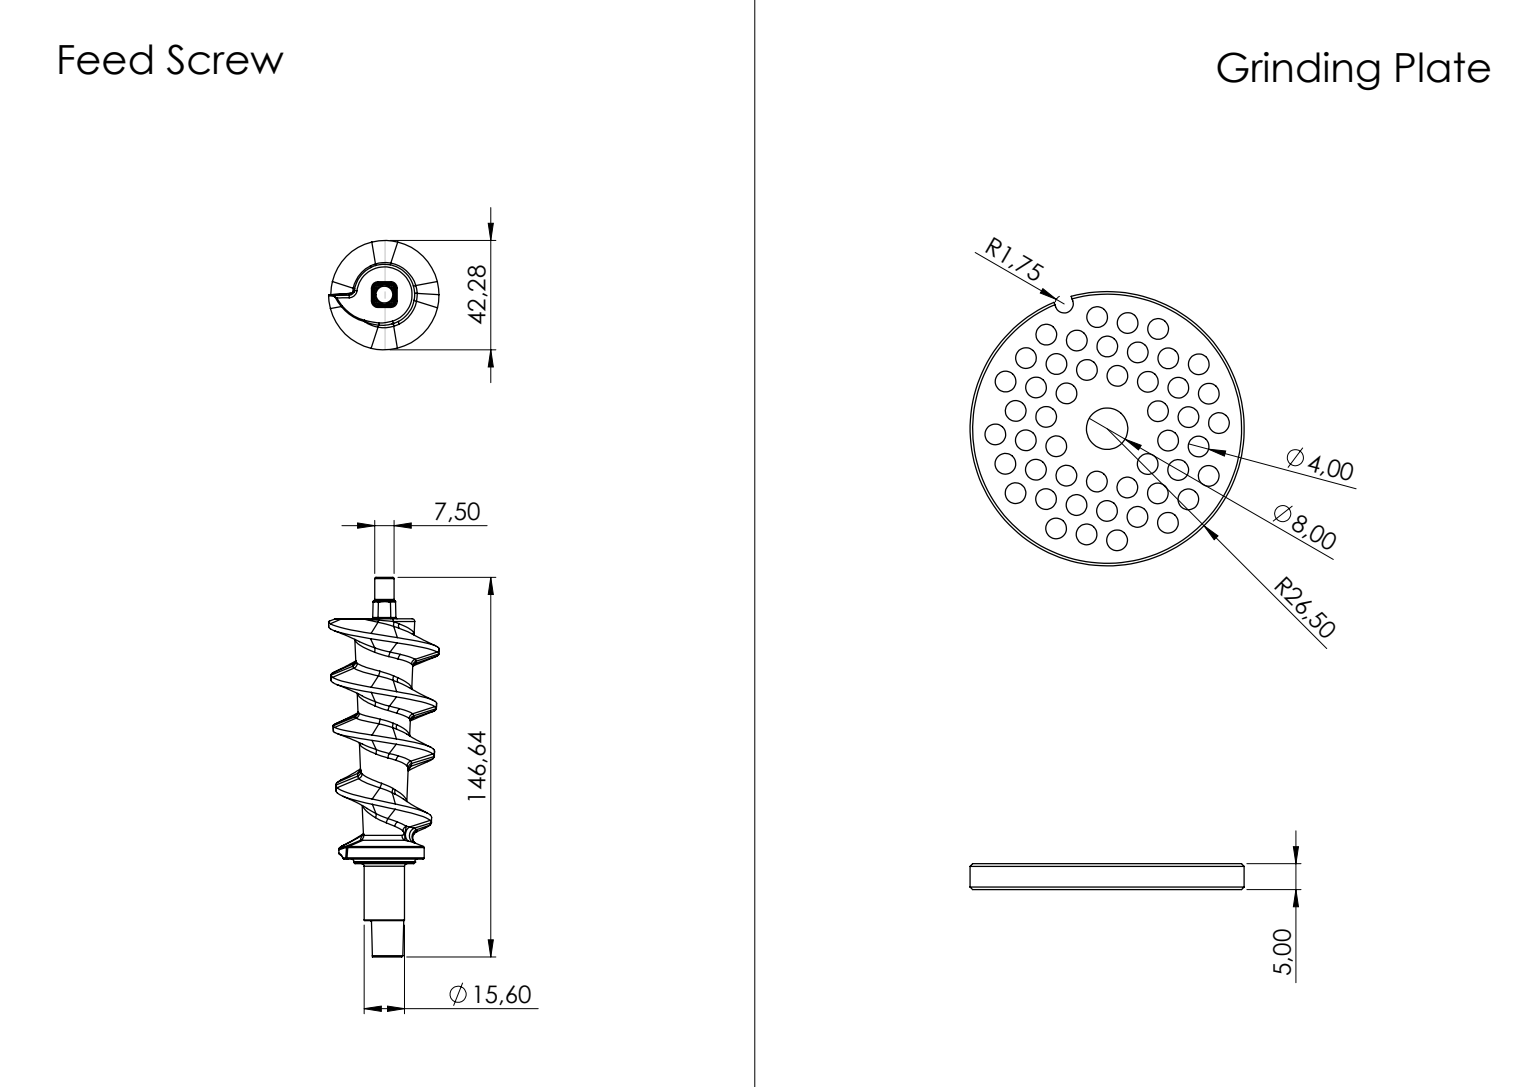
ISO-10303-21;
HEADER;
FILE_DESCRIPTION (('STEP AP214'),
    '1' );
FILE_NAME ('Feed Screw.step',
    '2026-10-06T09:49:54',
    ( '' ),
    ( '' ),
    'SwSTEP 2.0',
    'SolidWorks 2020',
    '' );
FILE_SCHEMA (( 'AUTOMOTIVE_DESIGN' ));
ENDSEC;

DATA;
#2=CIRCLE ( 'NONE', #35720, 101.7125698847119821 ) ;
#3=CARTESIAN_POINT ( 'NONE',  ( -1.842962214803815835, 1515.372048948338943, 213.3835825141717351 ) ) ;
#4=CARTESIAN_POINT ( 'NONE',  ( 9.183457267990059236, 1463.661210998930073, 215.2718514178839939 ) ) ;
#8=AXIS2_PLACEMENT_3D ( 'NONE', #3263, #37391, #36278 ) ;
#10=CARTESIAN_POINT ( 'NONE',  ( 0.5551898266394985626, 1477.809674746627479, 198.7211068470872135 ) ) ;
#12=CARTESIAN_POINT ( 'NONE',  ( -1.480872463509999903, 1515.456375364289897, 204.9462865469589872 ) ) ;
#15=CARTESIAN_POINT ( 'NONE',  ( 18.94656044352759849, 1455.761274322379904, 200.3458232381809694 ) ) ;
#17=CARTESIAN_POINT ( 'NONE',  ( -11.86274611122550127, 1422.387374207680068, 206.9860570071450070 ) ) ;
#28=CARTESIAN_POINT ( 'NONE',  ( -10.29516445159999982, 1471.669286221989978, 209.3797728120900103 ) ) ;
#29=DIRECTION ( 'NONE',  ( -3.697785493223495027E-32, -1.000000000000000000, 1.836970198721029688E-16 ) ) ;
#33=CARTESIAN_POINT ( 'NONE',  ( -4.766037424247389964, 1433.470086930039997, 216.3697912905370231 ) ) ;
#41=CARTESIAN_POINT ( 'NONE',  ( 11.68414648092010033, 1426.908524124409951, 207.1431733947370049 ) ) ;
#51=CARTESIAN_POINT ( 'NONE',  ( -6.833281637050000690, 1495.558145441189936, 200.1869151102389992 ) ) ;
#57=CARTESIAN_POINT ( 'NONE',  ( 5.798353088509999864, 1447.164911394289902, 201.8788308129090012 ) ) ;
#60=CARTESIAN_POINT ( 'NONE',  ( -2.894710226049999946, 1455.369075570189807, 200.0025452760189921 ) ) ;
#65=CARTESIAN_POINT ( 'NONE',  ( -1.064557613579999895, 1496.012454471690035, 220.6945835667989968 ) ) ;
#83=EDGE_CURVE ( 'NONE', #58839, #22042, #17431, .T. ) ;
#87=CARTESIAN_POINT ( 'NONE',  ( -4.994992778070000305, 1391.721842379389955, 214.6484993776389842 ) ) ;
#88=CARTESIAN_POINT ( 'NONE',  ( 15.23962836178434799, 1416.181292664740113, 211.4166089860522106 ) ) ;
#91=CARTESIAN_POINT ( 'NONE',  ( 9.827367186236088514, 1460.770885483560050, 206.7613957114989773 ) ) ;
#96=ORIENTED_EDGE ( 'NONE', *, *, #80068, .T. ) ;
#97=CARTESIAN_POINT ( 'NONE',  ( 2.803078862940000082, 1426.178365722219951, 191.2633630063989756 ) ) ;
#100=CARTESIAN_POINT ( 'NONE',  ( -12.21821484229520927, 1417.425190588804981, 199.7413714526001911 ) ) ;
#102=CARTESIAN_POINT ( 'NONE',  ( 4.324092179420000015, 1515.269353058490196, 209.1218459615519976 ) ) ;
#106=CARTESIAN_POINT ( 'NONE',  ( 9.417062327005512046, 1451.666586838229932, 209.4644760955090135 ) ) ;
#108=EDGE_CURVE ( 'NONE', #73608, #106056, #21407, .T. ) ;
#110=ORIENTED_EDGE ( 'NONE', *, *, #5630, .F. ) ;
#120=EDGE_CURVE ( 'NONE', #81793, #103948, #97600, .T. ) ;
#121=CARTESIAN_POINT ( 'NONE',  ( -9.628359219779209610, 1460.738556064009799, 208.1949697569470175 ) ) ;
#123=CARTESIAN_POINT ( 'NONE',  ( 10.94055631708340037, 1470.192781946979949, 206.9724510450730008 ) ) ;
#124=CARTESIAN_POINT ( 'NONE',  ( -3.048415848927723992, 1468.134006689671196, 219.8853015524805699 ) ) ;
#125=EDGE_CURVE ( 'NONE', #75164, #6066, #41467, .T. ) ;
#134=CARTESIAN_POINT ( 'NONE',  ( -17.39685236538799984, 1503.136637835580132, 222.8801028628849963 ) ) ;
#140=CARTESIAN_POINT ( 'NONE',  ( 0.7783252048321530614, 1515.125841190099891, 204.7939957918700316 ) ) ;
#144=CARTESIAN_POINT ( 'NONE',  ( -0.9578802547590020700, 1508.340034268889895, 220.7784182282989889 ) ) ;
#149=CARTESIAN_POINT ( 'NONE',  ( -5.649091365077420157, 1427.323616392150143, 201.6849725672220188 ) ) ;
#153=FACE_OUTER_BOUND ( 'NONE', #32956, .T. ) ;
#165=CARTESIAN_POINT ( 'NONE',  ( -14.80402621179999834, 1415.917690476640018, 204.7946628682890093 ) ) ;
#167=CARTESIAN_POINT ( 'NONE',  ( -4.911821946417970430, 1485.009740505319996, 198.2803573512069875 ) ) ;
#168=B_SPLINE_SURFACE_WITH_KNOTS ( 'NONE', 5, 5, ( 
 ( #106952, #71755, #28601, #29694, #97994, #64429 ),
 ( #81736, #88517, #89050, #98547, #97459, #20727 ),
 ( #54922, #21816, #107503, #56015, #12336, #105310 ),
 ( #90139, #13422, #62802, #46527, #11801, #45969 ),
 ( #80104, #37555, #80661, #98449, #4411, #47512 ),
 ( #96816, #3329, #28500, #89503, #82194, #106305 ),
 ( #97348, #37453, #12795, #72186, #90039, #21163 ),
 ( #90596, #62695, #38004, #13317, #4937, #12239 ),
 ( #72718, #45871, #80005, #29056, #106840, #63242 ) ),
 .UNSPECIFIED., .F., .F., .F.,
 ( 6, 3, 6 ),
 ( 6, 6 ),
 ( 14.29638737439180041, 25.07790639679999956, 35.02433850343369670 ),
 ( 0.000000000000000000, 2.000134677740009970 ),
 .UNSPECIFIED. ) ;
#169=CARTESIAN_POINT ( 'NONE',  ( -8.621279951388869378, 1436.974942194019832, 209.5887057810519991 ) ) ;
#170=CARTESIAN_POINT ( 'NONE',  ( -4.720696006799999900, 1497.300349750090163, 219.8012105612990013 ) ) ;
#172=CARTESIAN_POINT ( 'NONE',  ( 4.989246313819999834, 1471.909539260290103, 189.7082128665990126 ) ) ;
#175=CARTESIAN_POINT ( 'NONE',  ( -11.30102602861320094, 1508.425847713210032, 208.0120230822289784 ) ) ;
#193=CARTESIAN_POINT ( 'NONE',  ( 10.49733858283609855, 1480.659481621079976, 208.1380713321520091 ) ) ;
#195=CARTESIAN_POINT ( 'NONE',  ( -17.48499182319999790, 1442.494624508590050, 219.3180649765990040 ) ) ;
#197=CARTESIAN_POINT ( 'NONE',  ( -21.44637737161449920, 1506.412668956640118, 216.0243792029939982 ) ) ;
#202=CARTESIAN_POINT ( 'NONE',  ( 9.734438220109071338, 1436.124822200840072, 210.5259218765519620 ) ) ;
#203=CARTESIAN_POINT ( 'NONE',  ( -10.63028651890000020, 1491.023698122589849, 211.9405787866489845 ) ) ;
#204=CARTESIAN_POINT ( 'NONE',  ( 6.587579149753620023, 1448.214850730340004, 201.2521096501800173 ) ) ;
#214=ORIENTED_EDGE ( 'NONE', *, *, #74162, .T. ) ;
#220=CARTESIAN_POINT ( 'NONE',  ( -10.22078022364619976, 1448.827725899079724, 207.2905427559460065 ) ) ;
#221=CARTESIAN_POINT ( 'NONE',  ( -4.554962005479259446, 1508.731359867455467, 211.6097811027402713 ) ) ;
#230=CARTESIAN_POINT ( 'NONE',  ( 4.229167303610000594, 1436.983388288790138, 227.1518914930990150 ) ) ;
#234=VERTEX_POINT ( 'NONE', #57535 ) ;
#242=DIRECTION ( 'NONE',  ( -8.555280247707230573E-26, -1.000000000000000000, 1.836970198721029688E-16 ) ) ;
#245=EDGE_CURVE ( 'NONE', #43735, #91400, #105524, .T. ) ;
#249=ORIENTED_EDGE ( 'NONE', *, *, #87778, .F. ) ;
#257=CARTESIAN_POINT ( 'NONE',  ( 2.105736771246019767, 1423.442917612190058, 192.6277106367970191 ) ) ;
#258=EDGE_LOOP ( 'NONE', ( #43493, #77998, #28454, #11261 ) ) ;
#260=CARTESIAN_POINT ( 'NONE',  ( -17.51735096566159910, 1508.551704408389924, 210.4017072017840064 ) ) ;
#261=EDGE_CURVE ( 'NONE', #100109, #93900, #60124, .T. ) ;
#263=CARTESIAN_POINT ( 'NONE',  ( 5.082331142230000154, 1453.684120746589770, 217.0135184815189859 ) ) ;
#267=CARTESIAN_POINT ( 'NONE',  ( -2.999960124414019713, 1428.921094993090037, 200.2473963957619958 ) ) ;
#278=CARTESIAN_POINT ( 'NONE',  ( 10.93308164779909930, 1490.452501404730128, 209.9926135395130018 ) ) ;
#288=VERTEX_POINT ( 'NONE', #17119 ) ;
#290=CARTESIAN_POINT ( 'NONE',  ( -11.00800901137619903, 1508.439403004749920, 218.3132624233929846 ) ) ;
#293=CARTESIAN_POINT ( 'NONE',  ( -4.675540975309999681, 1462.620895424390028, 200.5633310686890241 ) ) ;
#301=CARTESIAN_POINT ( 'NONE',  ( 11.69460626421270000, 1479.933455554200009, 210.6357844716710019 ) ) ;
#302=CARTESIAN_POINT ( 'NONE',  ( 5.597778194180000888, 1506.679269386989972, 219.3685102149989916 ) ) ;
#308=EDGE_CURVE ( 'NONE', #12135, #84259, #7929, .T. ) ;
#312=CARTESIAN_POINT ( 'NONE',  ( 11.46319645939999887, 1501.893709296690076, 208.7006337201350163 ) ) ;
#318=DIRECTION ( 'NONE',  ( 0.000000000000000000, 1.000000000000000000, -1.836970198721029688E-16 ) ) ;
#320=CARTESIAN_POINT ( 'NONE',  ( -5.102340803919999779, 1483.010473641589897, 199.7820758705289848 ) ) ;
#328=VERTEX_POINT ( 'NONE', #27220 ) ;
#329=CARTESIAN_POINT ( 'NONE',  ( -2.217375791810000329, 1495.290970025190290, 217.2501089269190118 ) ) ;
#332=CARTESIAN_POINT ( 'NONE',  ( -0.6694169535389160597, 1457.182704574260015, 219.7360533319789795 ) ) ;
#336=CARTESIAN_POINT ( 'NONE',  ( 7.206186347910000123, 1424.944465238209887, 212.8420735846389960 ) ) ;
#337=CARTESIAN_POINT ( 'NONE',  ( -9.573037224950001089, 1423.427965722019962, 192.3355728592989919 ) ) ;
#345=VERTEX_POINT ( 'NONE', #33388 ) ;
#377=CARTESIAN_POINT ( 'NONE',  ( -3.070761075385165295, 1457.085219852218870, 218.1263196974262826 ) ) ;
#390=CARTESIAN_POINT ( 'NONE',  ( 10.73298406322840037, 1460.408024784029976, 207.0975327187530013 ) ) ;
#396=CARTESIAN_POINT ( 'NONE',  ( -18.69110324289999880, 1444.867398023490068, 206.3373603049990095 ) ) ;
#407=CARTESIAN_POINT ( 'NONE',  ( -10.75057650454519909, 1492.402834311169954, 203.1666067258980206 ) ) ;
#420=CARTESIAN_POINT ( 'NONE',  ( -16.94440841599999814, 1420.377411313550056, 203.4608118218089885 ) ) ;
#434=CARTESIAN_POINT ( 'NONE',  ( -13.41341432257899946, 1418.544055057069727, 200.5656092512240036 ) ) ;
#435=CARTESIAN_POINT ( 'NONE',  ( -5.015825127099213354, 1391.761757684846771, 203.5511880675617249 ) ) ;
#450=CARTESIAN_POINT ( 'NONE',  ( 10.56937681823290021, 1452.418559324240050, 209.1099374865879952 ) ) ;
#456=EDGE_LOOP ( 'NONE', ( #45426, #15333, #70007, #61987 ) ) ;
#458=FACE_OUTER_BOUND ( 'NONE', #93445, .T. ) ;
#462=CARTESIAN_POINT ( 'NONE',  ( 11.76667485211559949, 1479.372979666780111, 208.7507148262919827 ) ) ;
#470=CARTESIAN_POINT ( 'NONE',  ( -8.755578957433581166, 1424.773583938259890, 204.8410018134340191 ) ) ;
#475=CARTESIAN_POINT ( 'NONE',  ( 20.33642612138580219, 1475.138353456469986, 218.0161241308549904 ) ) ;
#479=DIRECTION ( 'NONE',  ( -1.699538841806929935E-33, 1.000000000000000000, -1.698192320643030073E-16 ) ) ;
#481=EDGE_CURVE ( 'NONE', #82285, #55990, #44994, .T. ) ;
#485=CARTESIAN_POINT ( 'NONE',  ( -2.314955559389999973, 1476.586284849689946, 199.0068122257989955 ) ) ;
#491=CARTESIAN_POINT ( 'NONE',  ( -7.514967970819999898, 1426.327999703259820, 205.9160403778789998 ) ) ;
#495=CARTESIAN_POINT ( 'NONE',  ( -7.863671303257509848, 1471.291298022706087, 215.5245834466820440 ) ) ;
#496=CARTESIAN_POINT ( 'NONE',  ( 7.537606959944939788, 1425.724147855899901, 212.1987702218239917 ) ) ;
#503=CARTESIAN_POINT ( 'NONE',  ( 1.205243432004479809, 1487.387165744484264, 219.8907050796039755 ) ) ;
#508=VERTEX_POINT ( 'NONE', #77503 ) ;
#515=ORIENTED_EDGE ( 'NONE', *, *, #31765, .T. ) ;
#529=CARTESIAN_POINT ( 'NONE',  ( -0.1150915766366530091, 1444.816874904579890, 199.0635159857669976 ) ) ;
#534=CARTESIAN_POINT ( 'NONE',  ( -3.384752634116700243, 1508.551704408389924, 213.9439043168609942 ) ) ;
#538=CARTESIAN_POINT ( 'NONE',  ( -3.774700670050000095, 1496.332844194289919, 198.4120365050989960 ) ) ;
#540=CARTESIAN_POINT ( 'NONE',  ( -1.514784269649715576, 1443.601484486217942, 218.3342104795610510 ) ) ;
#551=CARTESIAN_POINT ( 'NONE',  ( 9.575940986468468807, 1427.729431014379998, 211.3625234817539820 ) ) ;
#552=CARTESIAN_POINT ( 'NONE',  ( 1.154719254338330447, 1421.357514871522653, 193.7585151656728044 ) ) ;
#555=CARTESIAN_POINT ( 'NONE',  ( -9.252874484757731111, 1477.963449144112474, 214.0067384189093218 ) ) ;
#558=CARTESIAN_POINT ( 'NONE',  ( -11.02797255089159911, 1462.256692482700146, 209.5173753044250020 ) ) ;
#559=CARTESIAN_POINT ( 'NONE',  ( 18.24211828920000045, 1431.096497597789948, 200.8001355623590030 ) ) ;
#560=CARTESIAN_POINT ( 'NONE',  ( 10.45726464265210076, 1420.924558883679993, 198.4227429697920115 ) ) ;
#561=CARTESIAN_POINT ( 'NONE',  ( 4.780270616392929384, 1467.625973390280024, 217.8721612978610267 ) ) ;
#566=CARTESIAN_POINT ( 'NONE',  ( 0.3281250907512314741, 1477.756992672553451, 198.7115816712109506 ) ) ;
#568=CARTESIAN_POINT ( 'NONE',  ( -1.082449427729999858, 1515.225850744089939, 204.7966151436789914 ) ) ;
#570=CARTESIAN_POINT ( 'NONE',  ( -3.071477015947639888, 1470.850262397169899, 187.3986309147560121 ) ) ;
#572=CARTESIAN_POINT ( 'NONE',  ( -19.83550667398609946, 1418.664640197639983, 208.7685751368389901 ) ) ;
#578=DIRECTION ( 'NONE',  ( -0.000000000000000000, 1.836970198721029688E-16, 1.000000000000000000 ) ) ;
#582=CARTESIAN_POINT ( 'NONE',  ( -10.30263834680000024, 1471.732697784889979, 209.1299246244929861 ) ) ;
#583=B_SPLINE_CURVE_WITH_KNOTS ( 'NONE', 3,
 ( #94797, #754, #35441, #77995 ),
 .UNSPECIFIED., .F., .F.,
 ( 4, 4 ),
 ( 0.000000000000000000, 1.000000000000000000 ),
 .UNSPECIFIED. ) ;
#586=DIRECTION ( 'NONE',  ( -1.000000000000000000, 0.000000000000000000, 0.000000000000000000 ) ) ;
#587=CARTESIAN_POINT ( 'NONE',  ( -3.138770468918330003, 1433.097189459889933, 217.7316335566559928 ) ) ;
#589=CARTESIAN_POINT ( 'NONE',  ( 1.842963721827329815, 1515.551704300040001, 212.9514659606769840 ) ) ;
#594=CARTESIAN_POINT ( 'NONE',  ( 11.30421211722389963, 1422.134199828960163, 208.7798009037170175 ) ) ;
#599=CARTESIAN_POINT ( 'NONE',  ( 6.224950473385610472, 1466.920039123629977, 216.8753481341400118 ) ) ;
#601=CARTESIAN_POINT ( 'NONE',  ( 1.842962231260000028, 1515.064792882589927, 204.7923971856590128 ) ) ;
#603=CARTESIAN_POINT ( 'NONE',  ( -10.90040372089999998, 1492.525755917289871, 207.2558760794690045 ) ) ;
#608=CARTESIAN_POINT ( 'NONE',  ( 4.176540423850000572, 1446.483799824789912, 200.6257159222890039 ) ) ;
#611=CARTESIAN_POINT ( 'NONE',  ( -3.558358605100000016, 1455.955982659790152, 200.3550966547389862 ) ) ;
#615=CARTESIAN_POINT ( 'NONE',  ( -2.487213358930000062, 1495.883017016489930, 197.0235130655990190 ) ) ;
#616=CARTESIAN_POINT ( 'NONE',  ( -2.182814748220000212, 1496.366357223990008, 220.5334820124990074 ) ) ;
#618=CARTESIAN_POINT ( 'NONE',  ( -3.313501335607589748, 1397.551704408390151, 203.0565224509919915 ) ) ;
#633=EDGE_CURVE ( 'NONE', #14236, #26775, #48569, .T. ) ;
#635=CARTESIAN_POINT ( 'NONE',  ( 4.789026039587930050, 1508.551704408389924, 212.5881120909519950 ) ) ;
#639=CARTESIAN_POINT ( 'NONE',  ( 9.326151436081950408, 1460.944241195969880, 206.0386860876060098 ) ) ;
#640=CARTESIAN_POINT ( 'NONE',  ( -9.966727850805121136, 1439.480327375449860, 208.4309914983489875 ) ) ;
#642=VERTEX_POINT ( 'NONE', #25961 ) ;
#647=CARTESIAN_POINT ( 'NONE',  ( -11.16856291581570737, 1417.847332803086601, 198.5153517745319220 ) ) ;
#651=CARTESIAN_POINT ( 'NONE',  ( 9.418151193910370367, 1451.571079816670135, 209.2450735257419865 ) ) ;
#662=CARTESIAN_POINT ( 'NONE',  ( 6.537718912151950335, 1429.433188304760051, 215.9971499089490123 ) ) ;
#664=CARTESIAN_POINT ( 'NONE',  ( -8.182145408407338394, 1490.196931670758431, 216.4137635874354828 ) ) ;
#668=CARTESIAN_POINT ( 'NONE',  ( -8.211943818390000871, 1474.301007847190021, 202.7927141847590065 ) ) ;
#673=FACE_OUTER_BOUND ( 'NONE', #12560, .T. ) ;
#677=CARTESIAN_POINT ( 'NONE',  ( -19.73299507883049841, 1503.904988652430120, 218.6992329638289903 ) ) ;
#684=CARTESIAN_POINT ( 'NONE',  ( 0.4426438243888760060, 1515.147163425719782, 204.7945541343150069 ) ) ;
#690=CARTESIAN_POINT ( 'NONE',  ( -10.98255251702510016, 1462.120311678340158, 210.0436777776439783 ) ) ;
#692=FACE_OUTER_BOUND ( 'NONE', #109949, .T. ) ;
#694=CARTESIAN_POINT ( 'NONE',  ( 2.737811238710000428, 1478.658245750390051, 201.8858327187489863 ) ) ;
#696=CARTESIAN_POINT ( 'NONE',  ( -10.40955016854329962, 1480.514293831559826, 207.4814632850010128 ) ) ;
#703=EDGE_CURVE ( 'NONE', #94689, #56179, #31918, .T. ) ;
#707=CARTESIAN_POINT ( 'NONE',  ( -14.80403897610000108, 1417.086023134510015, 204.2975919913589848 ) ) ;
#710=CARTESIAN_POINT ( 'NONE',  ( -4.056355225345120274, 1485.204183987449824, 197.9328813784530041 ) ) ;
#712=CARTESIAN_POINT ( 'NONE',  ( 18.19395003950230105, 1429.625430537140119, 208.6624982699469797 ) ) ;
#713=CARTESIAN_POINT ( 'NONE',  ( -7.496170620820000075, 1497.189208763689976, 217.7743331409489826 ) ) ;
#714=VERTEX_POINT ( 'NONE', #62956 ) ;
#717=CARTESIAN_POINT ( 'NONE',  ( 10.57777681304790107, 1481.493442856720094, 209.1910062161780104 ) ) ;
#732=CARTESIAN_POINT ( 'NONE',  ( 3.609405579419999732, 1486.009611374690166, 219.2752556430990012 ) ) ;
#733=CARTESIAN_POINT ( 'NONE',  ( 10.89000033453339888, 1479.690907560379856, 208.0590789013299968 ) ) ;
#735=CARTESIAN_POINT ( 'NONE',  ( -17.57323599084560328, 1441.322512277789883, 219.0501625471149794 ) ) ;
#738=CARTESIAN_POINT ( 'NONE',  ( 20.56231132718039589, 1477.111355667389716, 217.7195232095880044 ) ) ;
#739=B_SPLINE_CURVE_WITH_KNOTS ( 'NONE', 5,
 ( #42585, #61612, #95745, #102472, #34730, #601 ),
 .UNSPECIFIED., .F., .F.,
 ( 6, 6 ),
 ( 0.000000000000000000, 1.000000000000000000 ),
 .UNSPECIFIED. ) ;
#744=CARTESIAN_POINT ( 'NONE',  ( -10.54543569900000044, 1491.422408008689899, 212.2964277208190254 ) ) ;
#745=CARTESIAN_POINT ( 'NONE',  ( 3.902982118626540320, 1446.676946215170119, 199.7493785281279770 ) ) ;
#751=CARTESIAN_POINT ( 'NONE',  ( 7.392112708435170099, 1434.232064116840093, 226.0537490036730048 ) ) ;
#753=CARTESIAN_POINT ( 'NONE',  ( 8.026470750289130152, 1504.708605097430109, 217.7675590729679982 ) ) ;
#754=CARTESIAN_POINT ( 'NONE',  ( -11.45094915626656018, 1505.046207261508243, 207.2314953572074785 ) ) ;
#761=ORIENTED_EDGE ( 'NONE', *, *, #76582, .F. ) ;
#763=CARTESIAN_POINT ( 'NONE',  ( -10.27580570860629905, 1448.659754571809799, 207.6397982481969962 ) ) ;
#764=CARTESIAN_POINT ( 'NONE',  ( 3.272146740929090303, 1515.551704204679936, 205.4774934054959772 ) ) ;
#769=CARTESIAN_POINT ( 'NONE',  ( 3.159262866049999730, 1466.676511916789877, 219.3004965968990234 ) ) ;
#777=VERTEX_POINT ( 'NONE', #27103 ) ;
#784=CARTESIAN_POINT ( 'NONE',  ( 20.96882344929999675, 1497.403700851489930, 212.2137616143489822 ) ) ;
#786=CARTESIAN_POINT ( 'NONE',  ( -0.9078489423485659460, 1465.209724574289794, 198.1556611775330055 ) ) ;
#788=CARTESIAN_POINT ( 'NONE',  ( 11.21656023086370091, 1422.137379126830183, 210.4074592674920154 ) ) ;
#791=ORIENTED_EDGE ( 'NONE', *, *, #108401, .F. ) ;
#795=DIRECTION ( 'NONE',  ( 0.9996573249755574819, 0.02617694830786557875, 0.000000000000000000 ) ) ;
#799=CARTESIAN_POINT ( 'NONE',  ( -1.400903968945880207, 1422.610669904860060, 192.5490106176209792 ) ) ;
#802=CARTESIAN_POINT ( 'NONE',  ( -17.67716118599750175, 1508.551704408389924, 210.4042409862270233 ) ) ;
#803=CARTESIAN_POINT ( 'NONE',  ( 1.779428963082609894, 1456.357349037730046, 198.6855221610310309 ) ) ;
#810=B_SPLINE_CURVE_WITH_KNOTS ( 'NONE', 3,
 ( #86877, #102007, #10171, #16338, #84662, #19666, #72306, #44910, #11292, #105900, #29721, #45460, #38124, #106437, #63371, #38670, #12366, #95830, #3999, #54953, #96390, #71782, #63906, #98021, #87442, #29180, #89079, #88010, #81220, #79601, #21293, #89626, #46553, #19098, #4536, #2905, #20755 ),
 .UNSPECIFIED., .F., .F.,
 ( 4, 3, 3, 3, 3, 3, 3, 3, 3, 3, 3, 3, 4 ),
 ( -12.02648877283809981, -11.71886065317380066, -11.10599023740059899, -10.45513282830309976, -9.768661030076680518, -9.016051782489549637, -8.113804059961630344, -7.249942693435659891, -6.491588414576360044, -5.633190057283429475, -4.895335684179899616, -4.254313181755179585, -3.650975912550000757 ),
 .UNSPECIFIED. ) ;
#811=FACE_OUTER_BOUND ( 'NONE', #80418, .T. ) ;
#818=ORIENTED_EDGE ( 'NONE', *, *, #64063, .F. ) ;
#820=CARTESIAN_POINT ( 'NONE',  ( 10.79932292162989960, 1490.768715835539979, 211.1233481957399931 ) ) ;
#839=B_SPLINE_CURVE_WITH_KNOTS ( 'NONE', 3,
 ( #94188, #26432, #95856, #96974, #60626, #95310, #44933, #10194, #44369, #79080, #712, #94749, #20238 ),
 .UNSPECIFIED., .F., .F.,
 ( 4, 3, 3, 3, 4 ),
 ( -1.599569173379999931, -0.7029132044934469636, 0.1891147555273189340, 1.073570521650659693, 1.599569173380000375 ),
 .UNSPECIFIED. ) ;
#840=CARTESIAN_POINT ( 'NONE',  ( 3.686065144790000137, 1468.106296616489999, 218.4108491294889802 ) ) ;
#841=CARTESIAN_POINT ( 'NONE',  ( 4.894570698429999922, 1447.010184225089915, 205.0316855332089858 ) ) ;
#847=CARTESIAN_POINT ( 'NONE',  ( 10.89269473999179993, 1480.433624861380167, 210.4306936963210148 ) ) ;
#849=CARTESIAN_POINT ( 'NONE',  ( -4.230955727593959104, 1446.180919742871311, 217.1469061245145724 ) ) ;
#857=CARTESIAN_POINT ( 'NONE',  ( 12.56213108819999924, 1501.082362947789989, 211.1229812159690198 ) ) ;
#861=CARTESIAN_POINT ( 'NONE',  ( 8.972723096110000185, 1427.878097284390151, 212.0837492402690145 ) ) ;
#866=CARTESIAN_POINT ( 'NONE',  ( -8.388361968899999965, 1483.465050472690109, 201.7385226000290004 ) ) ;
#874=ORIENTED_EDGE ( 'NONE', *, *, #74452, .T. ) ;
#876=CARTESIAN_POINT ( 'NONE',  ( -11.25637332900000054, 1500.624827952490023, 211.0037260121189888 ) ) ;
#877=CARTESIAN_POINT ( 'NONE',  ( -14.67979535943448255, 1416.151753477184002, 204.4125811959580972 ) ) ;
#880=CARTESIAN_POINT ( 'NONE',  ( -9.954564879586309090, 1438.994910147829842, 209.5496646517129875 ) ) ;
#881=EDGE_CURVE ( 'NONE', #44275, #39082, #97366, .T. ) ;
#884=CARTESIAN_POINT ( 'NONE',  ( 7.904651180169999236, 1423.075284537190100, 213.5785853047590024 ) ) ;
#885=CARTESIAN_POINT ( 'NONE',  ( -18.32377786700000399, 1464.077817829789865, 217.4721512913189940 ) ) ;
#890=CARTESIAN_POINT ( 'NONE',  ( 6.121126660120000729, 1455.402339941889750, 217.8370560331890147 ) ) ;
#894=CARTESIAN_POINT ( 'NONE',  ( -21.51338636340619814, 1505.551605034549766, 209.1218290568810119 ) ) ;
#896=CARTESIAN_POINT ( 'NONE',  ( 7.616929904139634999, 1500.300532160428247, 200.6431694768011482 ) ) ;
#898=CARTESIAN_POINT ( 'NONE',  ( -2.006862033407029955, 1475.288591552500066, 197.8580126313549954 ) ) ;
#925=B_SPLINE_SURFACE_WITH_KNOTS ( 'NONE', 5, 5, ( 
 ( #19475, #46376, #97294, #18912, #53676, #3824 ),
 ( #38484, #53110, #54765, #72133, #81042, #63188 ),
 ( #104039, #87819, #79951, #29002, #55317, #61517 ),
 ( #11106, #87247, #27891, #10538, #12182, #46923 ),
 ( #89449, #62074, #45268, #44712, #79406, #12741 ),
 ( #78863, #2717, #71032, #2170, #96760, #36285 ),
 ( #105153, #28445, #20030, #62639, #54224, #88351 ),
 ( #45818, #3268, #89993, #66483, #7097, #81581 ),
 ( #100045, #106789, #99478, #98393, #13268, #32299 ) ),
 .UNSPECIFIED., .F., .F., .F.,
 ( 6, 3, 6 ),
 ( 6, 6 ),
 ( 0.000000000000000000, 6.814644137399999302, 13.62928827480000038 ),
 ( 0.000000000000000000, 2.000000000000000000 ),
 .UNSPECIFIED. ) ;
#933=CARTESIAN_POINT ( 'NONE',  ( 5.983287317399999417, 1451.235340618889950, 210.0682002075799915 ) ) ;
#936=ADVANCED_FACE ( 'NONE', ( #76810 ), #40125, .T. ) ;
#940=CARTESIAN_POINT ( 'NONE',  ( -18.84544153430000080, 1444.454624232390188, 208.1911640471150235 ) ) ;
#950=EDGE_CURVE ( 'NONE', #36610, #45421, #18629, .T. ) ;
#951=CARTESIAN_POINT ( 'NONE',  ( -11.26811797368760004, 1492.006046055339993, 204.2379200572160016 ) ) ;
#961=CARTESIAN_POINT ( 'NONE',  ( -14.65245215464970130, 1420.119839417710182, 213.8659310620899987 ) ) ;
#964=ORIENTED_EDGE ( 'NONE', *, *, #29949, .T. ) ;
#966=CARTESIAN_POINT ( 'NONE',  ( 4.987078435459999071, 1509.051704408389924, 209.1218459616989946 ) ) ;
#971=CARTESIAN_POINT ( 'NONE',  ( 2.969165624449999541, 1442.252637987289972, 217.6050255308190060 ) ) ;
#976=EDGE_CURVE ( 'NONE', #32267, #2539, #49404, .T. ) ;
#978=CARTESIAN_POINT ( 'NONE',  ( 9253.086965755297570, 5182.654794667092574, 284.7734187413164477 ) ) ;
#980=CARTESIAN_POINT ( 'NONE',  ( -14.43176806938940082, 1417.361901689390152, 203.3004255274190086 ) ) ;
#983=CARTESIAN_POINT ( 'NONE',  ( -8.333035966500000669, 1508.478891882389917, 219.2689049391989897 ) ) ;
#991=CARTESIAN_POINT ( 'NONE',  ( -3.276363691050809823, 1486.691431019839911, 220.6577433852839931 ) ) ;
#992=CARTESIAN_POINT ( 'NONE',  ( -8.229021304010000648, 1439.448076410589920, 228.6152058856989697 ) ) ;
#998=CARTESIAN_POINT ( 'NONE',  ( 10.57159226293329901, 1452.549534872659933, 209.4522820094259714 ) ) ;
#1011=EDGE_CURVE ( 'NONE', #13254, #104898, #107740, .T. ) ;
#1020=CARTESIAN_POINT ( 'NONE',  ( 9.327660711791368797, 1434.415577812250149, 206.2244467992360057 ) ) ;
#1021=CARTESIAN_POINT ( 'NONE',  ( -15.14764113784119992, 1421.271689049209954, 203.4892272555310058 ) ) ;
#1024=ORIENTED_EDGE ( 'NONE', *, *, #4374, .T. ) ;
#1027=CARTESIAN_POINT ( 'NONE',  ( -4.249593083980000685, 1482.545674215690042, 231.1654941120989974 ) ) ;
#1034=CARTESIAN_POINT ( 'NONE',  ( -20.40544550950000158, 1484.240032026089921, 212.0770037828889940 ) ) ;
#1043=CARTESIAN_POINT ( 'NONE',  ( -7.987246895440000216, 1424.400859198919989, 210.3710278188289919 ) ) ;
#1048=CARTESIAN_POINT ( 'NONE',  ( 7.536498802507920480, 1425.740918852369987, 212.2034145707320079 ) ) ;
#1052=CARTESIAN_POINT ( 'NONE',  ( -10.95146640095969914, 1492.561632748999955, 207.2597909512799959 ) ) ;
#1055=CARTESIAN_POINT ( 'NONE',  ( -16.86741971048520128, 1508.492928484489994, 213.3340837003470085 ) ) ;
#1057=EDGE_LOOP ( 'NONE', ( #24193, #71471, #42216, #1770 ) ) ;
#1082=CARTESIAN_POINT ( 'NONE',  ( 4.303235405216580212, 1508.728291632010041, 205.3334392574930121 ) ) ;
#1085=CARTESIAN_POINT ( 'NONE',  ( -4.733838392061969991, 1508.551704408389924, 212.7087210097289756 ) ) ;
#1097=ORIENTED_EDGE ( 'NONE', *, *, #75681, .T. ) ;
#1102=CARTESIAN_POINT ( 'NONE',  ( 1.493039702043341022, 1421.445368576706869, 193.7871365012589706 ) ) ;
#1103=CARTESIAN_POINT ( 'NONE',  ( -4.326994892130199055, 1515.158502928330108, 209.0793308605450136 ) ) ;
#1106=CARTESIAN_POINT ( 'NONE',  ( -14.01525996361490023, 1415.677402202029953, 204.0303134510289738 ) ) ;
#1108=EDGE_CURVE ( 'NONE', #61133, #15891, #6544, .T. ) ;
#1110=FACE_OUTER_BOUND ( 'NONE', #108740, .T. ) ;
#1111=CARTESIAN_POINT ( 'NONE',  ( 18.25142110790000061, 1430.901022324190080, 200.8464198818790010 ) ) ;
#1113=CARTESIAN_POINT ( 'NONE',  ( 9.724852847713158610, 1462.948292999750265, 211.0616404486619899 ) ) ;
#1121=CARTESIAN_POINT ( 'NONE',  ( -1.448833437790000067, 1515.064791419390076, 204.7923971473389884 ) ) ;
#1122=CARTESIAN_POINT ( 'NONE',  ( -19.58884344854149973, 1465.811382644940068, 204.1485388013770148 ) ) ;
#1124=CARTESIAN_POINT ( 'NONE',  ( -13.94196614533020018, 1421.875924885620179, 203.6998106941310027 ) ) ;
#1125=CARTESIAN_POINT ( 'NONE',  ( 8.723134474349999223, 1451.781317889190177, 212.2855316608589931 ) ) ;
#1126=CARTESIAN_POINT ( 'NONE',  ( 17.96785475010000255, 1431.047211114990205, 205.7578563200790143 ) ) ;
#1130=CARTESIAN_POINT ( 'NONE',  ( -4.475591295720000140, 1474.980283356190057, 199.4186445563689745 ) ) ;
#1133=CARTESIAN_POINT ( 'NONE',  ( -5.469245208306690920, 1508.551704408389924, 219.5679309264459960 ) ) ;
#1135=FACE_OUTER_BOUND ( 'NONE', #76793, .T. ) ;
#1137=CARTESIAN_POINT ( 'NONE',  ( 5.104653541605128630, 1445.782371245855984, 201.6469468901138953 ) ) ;
#1148=ORIENTED_EDGE ( 'NONE', *, *, #73078, .F. ) ;
#1150=CARTESIAN_POINT ( 'NONE',  ( -4.378911555961889412, 1438.826708660780014, 227.2015615265439976 ) ) ;
#1151=ORIENTED_EDGE ( 'NONE', *, *, #27606, .F. ) ;
#1152=CARTESIAN_POINT ( 'NONE',  ( 5.622310450973170504, 1467.227804191469886, 217.3393949240599738 ) ) ;
#1155=CARTESIAN_POINT ( 'NONE',  ( 19.25039672899999843, 1455.004482529790039, 207.2621563279390102 ) ) ;
#1161=CARTESIAN_POINT ( 'NONE',  ( -10887.13479812350670, -2340.220200558883789, 7538.395907487779368 ) ) ;
#1165=CARTESIAN_POINT ( 'NONE',  ( 0.5801875626090010618, 1457.903154489290046, 199.5761716166789768 ) ) ;
#1169=CARTESIAN_POINT ( 'NONE',  ( -2.952024859200000240, 1496.639021482089902, 198.1365015686990034 ) ) ;
#1170=CARTESIAN_POINT ( 'NONE',  ( -2.178754852690000021, 1496.647359717190056, 220.9005516230989770 ) ) ;
#1185=CARTESIAN_POINT ( 'NONE',  ( -4.992439150849999230, 1391.624323207190173, 214.5505945479090144 ) ) ;
#1189=CARTESIAN_POINT ( 'NONE',  ( 10.02612625315829931, 1461.114985608630150, 207.7185774112350032 ) ) ;
#1191=ORIENTED_EDGE ( 'NONE', *, *, #89082, .F. ) ;
#1192=EDGE_LOOP ( 'NONE', ( #45908, #29426, #27970, #23465, #53686, #75685 ) ) ;
#1196=CARTESIAN_POINT ( 'NONE',  ( -7.680767148276910206, 1508.410451920919968, 219.5486563066939993 ) ) ;
#1197=CARTESIAN_POINT ( 'NONE',  ( -14.73343723154779994, 1508.551704405130067, 210.0752011545839935 ) ) ;
#1201=CARTESIAN_POINT ( 'NONE',  ( 9.592369369698889869, 1451.333035786799883, 207.7642936628679990 ) ) ;
#1202=CARTESIAN_POINT ( 'NONE',  ( 19.04547816490000045, 1456.669743087390088, 205.4226615881689781 ) ) ;
#1210=ORIENTED_EDGE ( 'NONE', *, *, #80921, .F. ) ;
#1214=CARTESIAN_POINT ( 'NONE',  ( -11.02689301977250125, 1462.508944275419935, 208.4529861560579889 ) ) ;
#1218=CARTESIAN_POINT ( 'NONE',  ( -7.027808362610000081, 1475.334978324289978, 201.5104037304890028 ) ) ;
#1219=CARTESIAN_POINT ( 'NONE',  ( 10.45331111600000185, 1492.246367015789929, 213.2054363916189743 ) ) ;
#1221=CARTESIAN_POINT ( 'NONE',  ( 8.995217975349083517, 1425.047741747077225, 195.6353441828489110 ) ) ;
#1222=CARTESIAN_POINT ( 'NONE',  ( -21.10523119420000171, 1505.940419546890098, 209.1830678612959957 ) ) ;
#1231=CARTESIAN_POINT ( 'NONE',  ( -14.75858115399999981, 1415.739699861750069, 212.8702772705990185 ) ) ;
#1232=CARTESIAN_POINT ( 'NONE',  ( -0.5056391281412709882, 1515.143808641139913, 204.7944662863439760 ) ) ;
#1234=CARTESIAN_POINT ( 'NONE',  ( -15.84297102958074532, 1415.885071821111978, 209.7209629398730328 ) ) ;
#1237=CARTESIAN_POINT ( 'NONE',  ( 19.96736869389999924, 1474.314440584889780, 212.0838811099789893 ) ) ;
#1238=CARTESIAN_POINT ( 'NONE',  ( -11.01732325727999928, 1462.230258711259921, 209.6174576145919843 ) ) ;
#1243=CARTESIAN_POINT ( 'NONE',  ( -11.63790511286740070, 1482.566214428189824, 206.5868431706369961 ) ) ;
#1255=CARTESIAN_POINT ( 'NONE',  ( -15.39978337890000049, 1415.475588077589919, 208.2578686251449938 ) ) ;
#1258=CARTESIAN_POINT ( 'NONE',  ( -3.792791800014749803, 1485.262872875560106, 197.8389773509790075 ) ) ;
#1260=DIRECTION ( 'NONE',  ( -0.1867376760110624201, -0.7251253628122718009, 0.6628138868222048785 ) ) ;
#1264=CARTESIAN_POINT ( 'NONE',  ( 14.60984432997775251, 1434.489065057944799, 221.3746616866943100 ) ) ;
#1277=CARTESIAN_POINT ( 'NONE',  ( 4.287908595200000228, 1515.369371658090131, 208.3885716294179815 ) ) ;
#1281=CARTESIAN_POINT ( 'NONE',  ( 5.027891267510000262, 1485.388390063490078, 218.6205902490090125 ) ) ;
#1282=CARTESIAN_POINT ( 'NONE',  ( 10.57494700539420052, 1480.041567197929908, 207.7444763255160183 ) ) ;
#1285=AXIS2_PLACEMENT_3D ( 'NONE', #34811, #68998, #94716 ) ;
#1286=CARTESIAN_POINT ( 'NONE',  ( 0.7066465098517540344, 1461.574489129789981, 230.4559209505140132 ) ) ;
#1288=CARTESIAN_POINT ( 'NONE',  ( 9.738308991446089635, 1493.400139332539993, 188.2659903719689680 ) ) ;
#1291=CARTESIAN_POINT ( 'NONE',  ( 9.815434228962379493, 1435.417726128900085, 208.8923042721449974 ) ) ;
#1292=CARTESIAN_POINT ( 'NONE',  ( -11.75194039070000152, 1490.261998080790136, 210.2102649680689979 ) ) ;
#1295=CARTESIAN_POINT ( 'NONE',  ( 4.180945349216710127, 1429.153325867737976, 216.2854025766479822 ) ) ;
#1299=CARTESIAN_POINT ( 'NONE',  ( 8.551703227357981163, 1503.794247392529996, 218.6779256640890026 ) ) ;
#1300=CARTESIAN_POINT ( 'NONE',  ( -10.04607665504151370, 1422.599490385782929, 210.6606566106900118 ) ) ;
#1315=CARTESIAN_POINT ( 'NONE',  ( 2.739535155620000051, 1466.840063050689878, 219.4352059655989819 ) ) ;
#1323=CARTESIAN_POINT ( 'NONE',  ( -18.26023438560000045, 1443.256148476890075, 213.5656046648789754 ) ) ;
#1331=CARTESIAN_POINT ( 'NONE',  ( -0.2723979594944390126, 1465.344599497509989, 198.1196121825180114 ) ) ;
#1336=CARTESIAN_POINT ( 'NONE',  ( 8.645456105984701267, 1437.915333935219905, 209.8214125568420059 ) ) ;
#1342=ORIENTED_EDGE ( 'NONE', *, *, #58015, .F. ) ;
#1346=CARTESIAN_POINT ( 'NONE',  ( -0.5495911971522959849, 1422.810403843149970, 192.5012090975810111 ) ) ;
#1355=CARTESIAN_POINT ( 'NONE',  ( -2.492811848245119588, 1429.200768276920144, 200.0866537460539973 ) ) ;
#1364=CARTESIAN_POINT ( 'NONE',  ( -4.987078442593329441, 1508.551704408389924, 211.6097810465890063 ) ) ;
#1377=AXIS2_PLACEMENT_3D ( 'NONE', #103027, #26324, #9531 ) ;
#1380=CARTESIAN_POINT ( 'NONE',  ( 3.466155636220000336, 1466.556171815189828, 219.1989959499990164 ) ) ;
#1387=CARTESIAN_POINT ( 'NONE',  ( 11.33822704553409899, 1479.770480605789999, 209.4503463167290249 ) ) ;
#1388=CARTESIAN_POINT ( 'NONE',  ( 3.529345253949999872, 1506.116810073189981, 220.6266478869990237 ) ) ;
#1396=CARTESIAN_POINT ( 'NONE',  ( 11.41988475489999999, 1502.185962516789914, 211.2997121632290032 ) ) ;
#1399=CARTESIAN_POINT ( 'NONE',  ( 8.877586941319998814, 1422.885318649510054, 212.4206501655689863 ) ) ;
#1404=ORIENTED_EDGE ( 'NONE', *, *, #13862, .F. ) ;
#1409=CARTESIAN_POINT ( 'NONE',  ( 1.850333291829999949, 1499.742999841690107, 230.3385376657990093 ) ) ;
#1410=CARTESIAN_POINT ( 'NONE',  ( -15.17407649454405139, 1416.062935498875049, 206.0915010440276660 ) ) ;
#1412=CARTESIAN_POINT ( 'NONE',  ( 0.2230871135786579862, 1456.931719161489809, 219.7455025295530220 ) ) ;
#1415=ADVANCED_FACE ( 'NONE', ( #58346 ), #55745, .F. ) ;
#1418=CARTESIAN_POINT ( 'NONE',  ( 7.494293556130000589, 1424.653638210349982, 212.2908972313289837 ) ) ;
#1419=CARTESIAN_POINT ( 'NONE',  ( 11.27339694790000024, 1433.557990534789951, 225.8166789514989716 ) ) ;
#1423=CARTESIAN_POINT ( 'NONE',  ( 6.708537208820000153, 1454.558820378589871, 216.3279882152490075 ) ) ;
#1432=CARTESIAN_POINT ( 'NONE',  ( 1.506981856204509862, 1476.106228118699846, 197.7392248870460207 ) ) ;
#1445=CARTESIAN_POINT ( 'NONE',  ( -4.060232945970000173, 1454.025412599190076, 199.8833095181790043 ) ) ;
#1457=EDGE_CURVE ( 'NONE', #35149, #76715, #34783, .T. ) ;
#1473=ORIENTED_EDGE ( 'NONE', *, *, #96056, .F. ) ;
#1483=CARTESIAN_POINT ( 'NONE',  ( -18.92739890465090014, 1503.345986874440086, 222.1981604764409894 ) ) ;
#1488=EDGE_CURVE ( 'NONE', #32360, #66058, #13266, .T. ) ;
#1492=CARTESIAN_POINT ( 'NONE',  ( -3.359680129360000045, 1429.147736159890201, 201.1390560926290050 ) ) ;
#1496=ADVANCED_FACE ( 'NONE', ( #9028 ), #7081, .T. ) ;
#1498=CARTESIAN_POINT ( 'NONE',  ( 3.830726099870000123, 1487.263094006890014, 197.7783884857990131 ) ) ;
#1510=VERTEX_POINT ( 'NONE', #35900 ) ;
#1511=EDGE_CURVE ( 'NONE', #61012, #77321, #48001, .T. ) ;
#1515=CARTESIAN_POINT ( 'NONE',  ( 2.613887865783830033, 1424.090078648330064, 191.3525227764439762 ) ) ;
#1522=CARTESIAN_POINT ( 'NONE',  ( -1.073559340110749938, 1444.993510080170154, 218.0402162255370229 ) ) ;
#1523=CARTESIAN_POINT ( 'NONE',  ( 10.57339846829999885, 1490.054618766489966, 202.8450963736189863 ) ) ;
#1526=ORIENTED_EDGE ( 'NONE', *, *, #72632, .T. ) ;
#1528=CARTESIAN_POINT ( 'NONE',  ( -4.833436873729840322, 1508.551704408090018, 212.3464058856069983 ) ) ;
#1532=CARTESIAN_POINT ( 'NONE',  ( 5.161277877375379575, 1424.205378946189967, 193.2953230041809718 ) ) ;
#1536=CARTESIAN_POINT ( 'NONE',  ( -2.731551787915110108, 1488.063880473559948, 219.6750998402769994 ) ) ;
#1537=CARTESIAN_POINT ( 'NONE',  ( 20.10527798697370017, 1430.877974082169885, 215.1856728963680041 ) ) ;
#1542=CARTESIAN_POINT ( 'NONE',  ( -5.034946147495399593, 1391.797004273162884, 214.6764752712134339 ) ) ;
#1544=CARTESIAN_POINT ( 'NONE',  ( 10.34950188612880062, 1451.639534178259964, 207.2650128704659949 ) ) ;
#1556=CARTESIAN_POINT ( 'NONE',  ( 8.983348777261449314, 1436.547473071500008, 210.1510915947499996 ) ) ;
#1565=CARTESIAN_POINT ( 'NONE',  ( -9.179291680683139276, 1449.804744045379948, 209.6468028662770280 ) ) ;
#1566=CARTESIAN_POINT ( 'NONE',  ( -10.52065382388829917, 1423.715440622650021, 204.4033256026779952 ) ) ;
#1571=CARTESIAN_POINT ( 'NONE',  ( 5.076297622210270255, 1469.790078878110080, 187.8425686012589892 ) ) ;
#1586=CARTESIAN_POINT ( 'NONE',  ( -9.227567128520000495, 1423.503386125029920, 208.4707392769450109 ) ) ;
#1587=ORIENTED_EDGE ( 'NONE', *, *, #48761, .T. ) ;
#1589=CARTESIAN_POINT ( 'NONE',  ( -9.088549428918609507, 1447.355647609609832, 212.1269012052750043 ) ) ;
#1592=CARTESIAN_POINT ( 'NONE',  ( 0.6958875083883689916, 1496.027399175239907, 221.4434803195429993 ) ) ;
#1602=CARTESIAN_POINT ( 'NONE',  ( -1.974748282550000011, 1461.153703759689961, 228.6317503212989948 ) ) ;
#1603=CARTESIAN_POINT ( 'NONE',  ( -8.888452916799840509, 1439.739375908359989, 206.8159864752560111 ) ) ;
#1604=ORIENTED_EDGE ( 'NONE', *, *, #54213, .T. ) ;
#1608=CARTESIAN_POINT ( 'NONE',  ( 2.157536728407479565, 1378.013060387289897, 207.9431782750405659 ) ) ;
#1611=ORIENTED_EDGE ( 'NONE', *, *, #77581, .F. ) ;
#1619=EDGE_CURVE ( 'NONE', #42338, #31705, #37819, .T. ) ;
#1626=ORIENTED_EDGE ( 'NONE', *, *, #36492, .T. ) ;
#1630=ORIENTED_EDGE ( 'NONE', *, *, #44015, .F. ) ;
#1637=CARTESIAN_POINT ( 'NONE',  ( -3.958123615280000784, 1496.263532292789932, 198.4814042619989891 ) ) ;
#1652=CARTESIAN_POINT ( 'NONE',  ( -9.414212789456051667, 1483.762164573529844, 201.8265950495219840 ) ) ;
#1653=CARTESIAN_POINT ( 'NONE',  ( 6.694559447547406172, 1420.584111001019892, 222.6458102056001565 ) ) ;
#1655=CARTESIAN_POINT ( 'NONE',  ( -4.329271545279450351, 1515.071561052280003, 207.5714932352460096 ) ) ;
#1661=CARTESIAN_POINT ( 'NONE',  ( -17.64133914897380251, 1419.302713979609962, 207.1869683601410088 ) ) ;
#1669=CARTESIAN_POINT ( 'NONE',  ( -15.57808073540140015, 1420.358152465259991, 210.5578313205389804 ) ) ;
#1672=CARTESIAN_POINT ( 'NONE',  ( 19.03958015586209740, 1453.804226984369734, 200.7927591122619901 ) ) ;
#1674=CARTESIAN_POINT ( 'NONE',  ( 1970.025574498409924, -8382.262153571269664, 413.0777247525010125 ) ) ;
#1675=( BOUNDED_SURFACE ( )  B_SPLINE_SURFACE ( 1, 2, ( 
 ( #51920, #17718, #978 ),
 ( #35102, #42398, #77665 ) ),
 .UNSPECIFIED., .F., .F., .F. ) 
 B_SPLINE_SURFACE_WITH_KNOTS ( ( 2, 2 ),
 ( 3, 3 ),
 ( -10000.00000000000000, 10000.00000000000000 ),
 ( 5.770213223686299742, 6.084699837289689661 ),
 .UNSPECIFIED. ) 
 GEOMETRIC_REPRESENTATION_ITEM ( )  RATIONAL_B_SPLINE_SURFACE ( (
 ( 0.8711730261270910214, 0.8915130006034900356, 0.9353332883307809986),
 ( 0.8711730261270910214, 0.8915130006034900356, 0.9353332883307809986) ) ) 
 REPRESENTATION_ITEM ( '' )  SURFACE ( )  );
#1678=VERTEX_POINT ( 'NONE', #59194 ) ;
#1679=DIRECTION ( 'NONE',  ( -6.922360974429999144E-17, -1.000000000000000000, 2.302693041820029802E-16 ) ) ;
#1681=CARTESIAN_POINT ( 'NONE',  ( -4.845900717560000182, 1475.703791084489922, 200.0054995007290017 ) ) ;
#1684=CARTESIAN_POINT ( 'NONE',  ( -5.312643570539870019, 1508.551704408389924, 219.6039287689250159 ) ) ;
#1686=B_SPLINE_SURFACE_WITH_KNOTS ( 'NONE', 5, 1, ( 
 ( #74996, #40266 ),
 ( #6664, #109145 ),
 ( #76630, #7225 ),
 ( #66606, #84478 ),
 ( #41384, #32960 ),
 ( #33500, #57097 ) ),
 .UNSPECIFIED., .F., .F., .F.,
 ( 6, 6 ),
 ( 2, 2 ),
 ( 0.000000000000000000, 3.644487327430000256 ),
 ( 0.000000000000000000, 14.00000000000000000 ),
 .UNSPECIFIED. ) ;
#1688=CARTESIAN_POINT ( 'NONE',  ( 7.124063054187752542, 1447.290098683538417, 203.4859220507082114 ) ) ;
#1692=CARTESIAN_POINT ( 'NONE',  ( 0.3570378922979989822, 1430.313573167290087, 217.4716923096189873 ) ) ;
#1693=CARTESIAN_POINT ( 'NONE',  ( -10.47820675957179937, 1471.893954719099838, 206.9970117854870182 ) ) ;
#1701=CARTESIAN_POINT ( 'NONE',  ( 11.15529992359070022, 1491.248582895630079, 209.3143910749519705 ) ) ;
#1704=CARTESIAN_POINT ( 'NONE',  ( 5.409313786005300884, 1467.330720308250193, 217.4825536316049863 ) ) ;
#1712=CARTESIAN_POINT ( 'NONE',  ( 11.41287573240554032, 1427.618782186570115, 209.6357587079445182 ) ) ;
#1716=CARTESIAN_POINT ( 'NONE',  ( 3.297786776830000210, 1446.227578061590066, 199.9593577526889874 ) ) ;
#1719=CARTESIAN_POINT ( 'NONE',  ( -17.04962538713110121, 1486.805668029350045, 197.2415639623459924 ) ) ;
#1724=B_SPLINE_SURFACE_WITH_KNOTS ( 'NONE', 5, 1, ( 
 ( #92066, #41669 ),
 ( #83658, #94260 ),
 ( #57933, #15338 ),
 ( #49533, #76934 ),
 ( #15879, #66891 ),
 ( #42221, #42773 ) ),
 .UNSPECIFIED., .F., .F., .F.,
 ( 6, 6 ),
 ( 2, 2 ),
 ( 0.000000000000000000, 3.703380931809999943 ),
 ( 0.000000000000000000, 14.00000000000000000 ),
 .UNSPECIFIED. ) ;
#1727=CARTESIAN_POINT ( 'NONE',  ( 0.1390463022569990159, 1495.976490991190076, 221.0825533988989946 ) ) ;
#1729=DIRECTION ( 'NONE',  ( 0.02091224828123159837, -0.9990482215818557998, 0.03827961371219689574 ) ) ;
#1742=CARTESIAN_POINT ( 'NONE',  ( 3.664296634863810187, 1508.551704408389924, 213.8143107331380008 ) ) ;
#1744=ORIENTED_EDGE ( 'NONE', *, *, #703, .T. ) ;
#1746=CARTESIAN_POINT ( 'NONE',  ( 10.57327070435720096, 1460.185313085440157, 206.4178343085929725 ) ) ;
#1752=CARTESIAN_POINT ( 'NONE',  ( 8.386023354940000729, 1423.866883236690001, 196.1572597689990118 ) ) ;
#1754=ORIENTED_EDGE ( 'NONE', *, *, #76872, .F. ) ;
#1758=EDGE_CURVE ( 'NONE', #70893, #20110, #58084, .T. ) ;
#1761=CARTESIAN_POINT ( 'NONE',  ( 10.12479509396839994, 1452.415778204070193, 209.5091751999849805 ) ) ;
#1770=ORIENTED_EDGE ( 'NONE', *, *, #81687, .F. ) ;
#1772=CARTESIAN_POINT ( 'NONE',  ( -7.764617407222809575, 1508.427764620530070, 219.4967056752809924 ) ) ;
#1774=CARTESIAN_POINT ( 'NONE',  ( -9.335957737771540366, 1471.828384389039911, 213.1700668700030121 ) ) ;
#1780=CARTESIAN_POINT ( 'NONE',  ( 10.26709333669999857, 1491.783873301489848, 213.2283046884589908 ) ) ;
#1788=VERTEX_POINT ( 'NONE', #48586 ) ;
#1793=CARTESIAN_POINT ( 'NONE',  ( 5.067689999509999765, 1506.887323632490052, 219.6537200326989989 ) ) ;
#1796=CARTESIAN_POINT ( 'NONE',  ( -1.107569330198709956, 1515.100382602269974, 204.7933291353800200 ) ) ;
#1798=CARTESIAN_POINT ( 'NONE',  ( -15.91585955922337980, 1416.028785253251044, 209.7484352619693198 ) ) ;
#1800=CARTESIAN_POINT ( 'NONE',  ( -16.16142260170000000, 1416.488921252410137, 208.6362116258320043 ) ) ;
#1801=CARTESIAN_POINT ( 'NONE',  ( 20.12874795999999833, 1473.837606016890049, 209.1218459616989946 ) ) ;
#1804=CARTESIAN_POINT ( 'NONE',  ( 1.124603181250000139, 1449.146011021990034, 189.9697284036990368 ) ) ;
#1805=FACE_OUTER_BOUND ( 'NONE', #29524, .T. ) ;
#1808=CARTESIAN_POINT ( 'NONE',  ( -10.50091854186509899, 1480.819183498580060, 208.0986103929409694 ) ) ;
#1818=CARTESIAN_POINT ( 'NONE',  ( 4.709520687179999499, 1480.407452823689937, 228.9869292435990076 ) ) ;
#1821=CARTESIAN_POINT ( 'NONE',  ( -15.39672782999999967, 1414.987016207339821, 208.1293397230249980 ) ) ;
#1847=CARTESIAN_POINT ( 'NONE',  ( 3.394586460100000203, 1484.752177863690122, 220.4731790066989845 ) ) ;
#1853=CARTESIAN_POINT ( 'NONE',  ( -9.960918163209999676, 1449.652119265389956, 190.8907471528989959 ) ) ;
#1855=CARTESIAN_POINT ( 'NONE',  ( 18.32583680416279748, 1473.764155899330035, 194.8973843979659932 ) ) ;
#1858=CARTESIAN_POINT ( 'NONE',  ( -5.076113882429999613, 1391.871667267490011, 203.5799967627289675 ) ) ;
#1861=CARTESIAN_POINT ( 'NONE',  ( -15.26258821600000104, 1420.451304246630116, 211.3041522489459965 ) ) ;
#1862=CARTESIAN_POINT ( 'NONE',  ( 9.538751646130227968, 1491.433371252692041, 189.9872483449992728 ) ) ;
#1869=CARTESIAN_POINT ( 'NONE',  ( 6.506813043129500151, 1504.727164751039936, 219.6746885927560129 ) ) ;
#1876=VERTEX_POINT ( 'NONE', #26095 ) ;
#1878=CARTESIAN_POINT ( 'NONE',  ( -10.29190872868499973, 1448.598814390959888, 207.7705778465489743 ) ) ;
#1881=CARTESIAN_POINT ( 'NONE',  ( 4.039020860156879777, 1467.562285101070074, 215.1688013428469901 ) ) ;
#1883=CARTESIAN_POINT ( 'NONE',  ( -1.713873510270000011, 1469.335086563190089, 219.0204275940589866 ) ) ;
#1885=ADVANCED_FACE ( 'NONE', ( #104481 ), #66090, .T. ) ;
#1888=CARTESIAN_POINT ( 'NONE',  ( -6.146133249640749696, 1425.318217922679878, 208.0573756490000221 ) ) ;
#1889=CARTESIAN_POINT ( 'NONE',  ( -20.61186923340000021, 1484.905403178689994, 208.1155942278690247 ) ) ;
#1892=DIRECTION ( 'NONE',  ( 0.4794255386042031719, 0.000000000000000000, 0.8775825618903726477 ) ) ;
#1901=CARTESIAN_POINT ( 'NONE',  ( 10.14837267200000070, 1461.673059420789968, 209.1843067467119965 ) ) ;
#1905=EDGE_CURVE ( 'NONE', #90721, #25072, #15288, .T. ) ;
#1907=VERTEX_POINT ( 'NONE', #61964 ) ;
#1909=ORIENTED_EDGE ( 'NONE', *, *, #65995, .T. ) ;
#1913=ORIENTED_EDGE ( 'NONE', *, *, #78321, .T. ) ;
#1922=CARTESIAN_POINT ( 'NONE',  ( -3.318767601309999815, 1508.056473026189906, 220.8617977084990116 ) ) ;
#1934=VERTEX_POINT ( 'NONE', #95529 ) ;
#1937=CARTESIAN_POINT ( 'NONE',  ( 5.939587785669203868, 1485.462588962051768, 218.1262196687094388 ) ) ;
#1940=CARTESIAN_POINT ( 'NONE',  ( -10.33299517979799909, 1447.717325788079961, 209.8084994951809961 ) ) ;
#1943=CARTESIAN_POINT ( 'NONE',  ( -9.135375560561769248, 1450.134946103599987, 207.9596124096709673 ) ) ;
#1952=CARTESIAN_POINT ( 'NONE',  ( 20.78416965899999980, 1496.368170310390042, 205.3334059301089951 ) ) ;
#1953=CARTESIAN_POINT ( 'NONE',  ( -0.3966884594078615711, 1469.475063426553106, 219.1656958591027831 ) ) ;
#1957=CARTESIAN_POINT ( 'NONE',  ( 1.248319727109999944, 1432.832940530890028, 200.7627304074090091 ) ) ;
#1959=CARTESIAN_POINT ( 'NONE',  ( 2.586184907469999850, 1507.324410716090142, 220.5577431766989775 ) ) ;
#1960=FACE_OUTER_BOUND ( 'NONE', #14772, .T. ) ;
#1965=CARTESIAN_POINT ( 'NONE',  ( -0.09132851563079860679, 1485.606224300089934, 197.9629336334990057 ) ) ;
#1966=CARTESIAN_POINT ( 'NONE',  ( 8.026943330234900031, 1467.154782912119799, 202.9971560891700051 ) ) ;
#1971=CARTESIAN_POINT ( 'NONE',  ( 8.528404547750000120, 1427.401138475999915, 211.7487601184689936 ) ) ;
#1976=CARTESIAN_POINT ( 'NONE',  ( -9.604374367299998383, 1481.821681780390008, 204.6246279580790031 ) ) ;
#1979=ORIENTED_EDGE ( 'NONE', *, *, #8655, .T. ) ;
#1980=CONICAL_SURFACE ( 'NONE', #64570, 0.9999999999999962252, 0.7853981633970000820 ) ;
#1984=CARTESIAN_POINT ( 'NONE',  ( -19.65008011549999978, 1466.825520213989876, 211.9829227778189988 ) ) ;
#1985=CARTESIAN_POINT ( 'NONE',  ( -15.29554544528689597, 1416.036841487845777, 206.5879621630117242 ) ) ;
#1988=CARTESIAN_POINT ( 'NONE',  ( -9.821317627027500663, 1438.502739476040233, 210.5947021706759870 ) ) ;
#1989=CARTESIAN_POINT ( 'NONE',  ( 0.1076058614650010070, 1458.116229757589963, 202.2619487776389917 ) ) ;
#1992=CARTESIAN_POINT ( 'NONE',  ( 7.540798545940000430, 1425.730109158910182, 212.1916703474689996 ) ) ;
#1993=CARTESIAN_POINT ( 'NONE',  ( 4.677562605459999467, 1434.889072344290071, 228.7640133631989841 ) ) ;
#1998=CARTESIAN_POINT ( 'NONE',  ( 5.588245553200000160, 1454.953086687389941, 217.2248557766390036 ) ) ;
#2008=CARTESIAN_POINT ( 'NONE',  ( -2.333876373187340203, 1475.197367001489965, 197.9245314158600024 ) ) ;
#2019=ORIENTED_EDGE ( 'NONE', *, *, #82259, .F. ) ;
#2021=CARTESIAN_POINT ( 'NONE',  ( -3.467945401910000225, 1455.040194281890081, 200.2251794624690149 ) ) ;
#2026=ORIENTED_EDGE ( 'NONE', *, *, #78076, .F. ) ;
#2036=CARTESIAN_POINT ( 'NONE',  ( 9.634908749268699779, 1462.534321465409903, 207.6260219664079898 ) ) ;
#2050=CARTESIAN_POINT ( 'NONE',  ( -21.46486317390879961, 1504.440058737759955, 215.6677353464210114 ) ) ;
#2056=ORIENTED_EDGE ( 'NONE', *, *, #95674, .T. ) ;
#2059=CARTESIAN_POINT ( 'NONE',  ( -4.858360392517085735, 1508.551704411667288, 206.6339107026657018 ) ) ;
#2080=CARTESIAN_POINT ( 'NONE',  ( 2.840612313169999847, 1441.622523712489965, 218.2291133001489811 ) ) ;
#2082=CARTESIAN_POINT ( 'NONE',  ( 740.1067050506055693, 11216.44053380570949, 2045.284436369865034 ) ) ;
#2086=CARTESIAN_POINT ( 'NONE',  ( -5.134146397328430922, 1464.447298219960203, 199.3723941709099847 ) ) ;
#2095=CARTESIAN_POINT ( 'NONE',  ( -2.205748714679999889, 1484.684221590389825, 198.4976517307989923 ) ) ;
#2096=CARTESIAN_POINT ( 'NONE',  ( -11.41675697748640061, 1482.775670443970057, 205.7339590229720159 ) ) ;
#2101=CARTESIAN_POINT ( 'NONE',  ( -11.28648375916229973, 1489.673514985999873, 212.4366478923779766 ) ) ;
#2102=CARTESIAN_POINT ( 'NONE',  ( 13.52267151192459949, 1497.923547478540286, 227.8730108396369758 ) ) ;
#2109=CARTESIAN_POINT ( 'NONE',  ( 10.56407631929999980, 1452.658139941989930, 209.7432180256290053 ) ) ;
#2116=EDGE_CURVE ( 'NONE', #42951, #41116, #80771, .T. ) ;
#2121=CARTESIAN_POINT ( 'NONE',  ( 9.001848782638129265, 1436.441033338579928, 209.9342506180670114 ) ) ;
#2127=CARTESIAN_POINT ( 'NONE',  ( -1.693092047772239983, 1443.235800395060096, 218.9922115469449864 ) ) ;
#2130=CARTESIAN_POINT ( 'NONE',  ( -9.184076889506968655, 1450.489465732099916, 208.2759141665609945 ) ) ;
#2131=CARTESIAN_POINT ( 'NONE',  ( -9.418568788532940772, 1424.364165527140131, 204.6686179336989824 ) ) ;
#2135=CARTESIAN_POINT ( 'NONE',  ( -3.176056732109739933, 1508.610720109290014, 213.8016369874950158 ) ) ;
#2136=CARTESIAN_POINT ( 'NONE',  ( 16.44572865500000347, 1495.267817486490003, 192.9050346917990169 ) ) ;
#2138=EDGE_CURVE ( 'NONE', #104484, #77864, #77374, .T. ) ;
#2143=CARTESIAN_POINT ( 'NONE',  ( 4.329407853939748918, 1515.066355634550064, 210.8164016152200020 ) ) ;
#2155=EDGE_CURVE ( 'NONE', #105726, #27470, #27209, .T. ) ;
#2162=CARTESIAN_POINT ( 'NONE',  ( -3.703568358935259930, 1497.311626042180023, 220.9591690318370070 ) ) ;
#2163=ORIENTED_EDGE ( 'NONE', *, *, #35189, .T. ) ;
#2168=CARTESIAN_POINT ( 'NONE',  ( 5.350728454891725328, 1427.748570762830695, 215.4189187839067188 ) ) ;
#2169=CARTESIAN_POINT ( 'NONE',  ( -17.00038391736149990, 1508.541898703860170, 212.8847129985989852 ) ) ;
#2170=CARTESIAN_POINT ( 'NONE',  ( 9.211869141260001115, 1471.980260610790083, 214.4234941383089961 ) ) ;
#2171=FACE_OUTER_BOUND ( 'NONE', #70001, .T. ) ;
#2175=FACE_OUTER_BOUND ( 'NONE', #89613, .T. ) ;
#2176=CARTESIAN_POINT ( 'NONE',  ( 8.468745670032260975, 1436.332250083529971, 207.5732686620520155 ) ) ;
#2195=VERTEX_POINT ( 'NONE', #5887 ) ;
#2196=CARTESIAN_POINT ( 'NONE',  ( 3.224549562455929941, 1508.551704408489968, 204.2884091523009999 ) ) ;
#2202=CARTESIAN_POINT ( 'NONE',  ( -3.983585865099999790, 1497.196993069489963, 198.5852023898990240 ) ) ;
#2208=CARTESIAN_POINT ( 'NONE',  ( 12.26870259150531872, 1428.415420825756428, 194.9349402552377057 ) ) ;
#2209=EDGE_CURVE ( 'NONE', #26627, #53103, #57965, .T. ) ;
#2213=CARTESIAN_POINT ( 'NONE',  ( -16.84534104709999980, 1417.257337058139910, 207.1240090553390019 ) ) ;
#2215=CARTESIAN_POINT ( 'NONE',  ( -6.267272736393399768, 1484.683887506470001, 198.9978965073320012 ) ) ;
#2216=CARTESIAN_POINT ( 'NONE',  ( -20.75777115397048433, 1507.865918544692931, 209.5048640109985172 ) ) ;
#2218=CARTESIAN_POINT ( 'NONE',  ( -4.327148319164989765, 1515.152643786279896, 208.8010119524350046 ) ) ;
#2225=CARTESIAN_POINT ( 'NONE',  ( -9.613516620566301185, 1460.231789534549989, 209.9813920803319718 ) ) ;
#2226=CARTESIAN_POINT ( 'NONE',  ( -9.292082803063870244, 1422.258564872340003, 192.2454125014830026 ) ) ;
#2231=CARTESIAN_POINT ( 'NONE',  ( -0.7790227543749990158, 1442.687262046989872, 200.2740145245590213 ) ) ;
#2232=CARTESIAN_POINT ( 'NONE',  ( -20.11385680769999951, 1487.601373209189887, 204.1067431612489997 ) ) ;
#2237=CARTESIAN_POINT ( 'NONE',  ( 8.454790733525280544, 1428.363638633589972, 213.4109935021670026 ) ) ;
#2239=EDGE_CURVE ( 'NONE', #10343, #12135, #19253, .T. ) ;
#2240=FACE_OUTER_BOUND ( 'NONE', #51460, .T. ) ;
#2243=CARTESIAN_POINT ( 'NONE',  ( 234.5897387251999930, 11221.53578756869865, -1757.702084499889907 ) ) ;
#2246=FACE_OUTER_BOUND ( 'NONE', #26866, .T. ) ;
#2253=CARTESIAN_POINT ( 'NONE',  ( -9.104767224130160486, 1421.478911732549932, 192.1853015429209961 ) ) ;
#2254=ORIENTED_EDGE ( 'NONE', *, *, #36492, .F. ) ;
#2260=CARTESIAN_POINT ( 'NONE',  ( -2.854504612459999979, 1433.072736100190014, 218.2391856586490064 ) ) ;
#2261=CARTESIAN_POINT ( 'NONE',  ( -10.39285233026310173, 1472.009416248819889, 207.0409344721679759 ) ) ;
#2266=CARTESIAN_POINT ( 'NONE',  ( 10.14173938847820189, 1422.829424262219845, 209.7691254332700055 ) ) ;
#2267=ORIENTED_EDGE ( 'NONE', *, *, #90513, .T. ) ;
#2269=CARTESIAN_POINT ( 'NONE',  ( 10.95672069168569962, 1490.579439969769965, 207.2253856564389878 ) ) ;
#2277=CARTESIAN_POINT ( 'NONE',  ( 12.32624855160359978, 1427.184147377119871, 207.2003428294259777 ) ) ;
#2288=CARTESIAN_POINT ( 'NONE',  ( 0.9541163229580019722, 1497.352948200390074, 197.4851080636989877 ) ) ;
#2289=CARTESIAN_POINT ( 'NONE',  ( -2.432658854300000062, 1495.143052030289937, 220.0417648853990045 ) ) ;
#2290=EDGE_CURVE ( 'NONE', #6066, #15508, #7175, .T. ) ;
#2293=DIRECTION ( 'NONE',  ( -9.152776640618289361E-47, 1.000000000000000000, -1.836970198721029688E-16 ) ) ;
#2303=CARTESIAN_POINT ( 'NONE',  ( -5.292247061280000331, 1391.913060387289988, 214.4361776263990009 ) ) ;
#2306=CARTESIAN_POINT ( 'NONE',  ( 6.225972109890000716, 1494.795958560490135, 219.7811165620990153 ) ) ;
#2310=VERTEX_POINT ( 'NONE', #53149 ) ;
#2311=CARTESIAN_POINT ( 'NONE',  ( 8.784510176764259270, 1452.237572000909950, 212.1743866200270077 ) ) ;
#2330=CARTESIAN_POINT ( 'NONE',  ( -2.188078410709979771, 1508.020976590390092, 220.9453026643990086 ) ) ;
#2333=CARTESIAN_POINT ( 'NONE',  ( -9.105445285308739756, 1471.726587830969947, 213.6544575909670129 ) ) ;
#2336=CARTESIAN_POINT ( 'NONE',  ( 9.221676543900459322, 1450.699204871009897, 209.5818517409399817 ) ) ;
#2337=CARTESIAN_POINT ( 'NONE',  ( -6.917540847650000657, 1474.438802919490172, 201.2803177021589818 ) ) ;
#2338=CARTESIAN_POINT ( 'NONE',  ( 9.489398001770000590, 1491.701139852389815, 214.8220554479490261 ) ) ;
#2340=CARTESIAN_POINT ( 'NONE',  ( 8.556778216962817041, 1424.669736104401181, 195.7159935075917474 ) ) ;
#2341=CARTESIAN_POINT ( 'NONE',  ( -20.26886524579999715, 1505.341425002289952, 209.1373927737770089 ) ) ;
#2355=CARTESIAN_POINT ( 'NONE',  ( -1.480922050758809894, 1515.075000927520023, 204.7926644938669938 ) ) ;
#2357=CARTESIAN_POINT ( 'NONE',  ( -15.87953847626955373, 1415.948856948393768, 209.7347139027639287 ) ) ;
#2361=CARTESIAN_POINT ( 'NONE',  ( 8.311307340579794811, 1438.191820051692957, 214.6582588010098220 ) ) ;
#2369=CARTESIAN_POINT ( 'NONE',  ( 9.756855720090040762, 1469.870621582290141, 211.6163541429820043 ) ) ;
#2382=CARTESIAN_POINT ( 'NONE',  ( -16.80421781410000293, 1416.570018552790089, 209.4889783200769955 ) ) ;
#2392=CARTESIAN_POINT ( 'NONE',  ( -12.56042467189510070, 1508.551704408300111, 210.1774334085390024 ) ) ;
#2396=CARTESIAN_POINT ( 'NONE',  ( -11.87618687435380060, 1481.834444412209905, 209.2076145084409973 ) ) ;
#2405=CARTESIAN_POINT ( 'NONE',  ( -10.06401538933667617, 1494.155344878688538, 204.3007335798515953 ) ) ;
#2408=CARTESIAN_POINT ( 'NONE',  ( 9.548870672246419389, 1470.075437067029952, 212.3439895025789781 ) ) ;
#2411=CARTESIAN_POINT ( 'NONE',  ( 3.296743891669999815, 1423.732652684919913, 192.8007254636989956 ) ) ;
#2414=CARTESIAN_POINT ( 'NONE',  ( 8.092055354027909431, 1461.514282906779954, 228.8774819441619854 ) ) ;
#2420=CARTESIAN_POINT ( 'NONE',  ( -15.57808073540140015, 1420.358152465259991, 210.5578313205389804 ) ) ;
#2433=VERTEX_POINT ( 'NONE', #33412 ) ;
#2448=CARTESIAN_POINT ( 'NONE',  ( -8.430248171497698451, 1423.638267348000227, 208.7623137433450040 ) ) ;
#2461=CARTESIAN_POINT ( 'NONE',  ( 10.95832423829999946, 1461.079497205190137, 209.0421603647289999 ) ) ;
#2466=VERTEX_POINT ( 'NONE', #101717 ) ;
#2478=CARTESIAN_POINT ( 'NONE',  ( 0.05881865638218039538, 1422.953928556980145, 192.4959481148550253 ) ) ;
#2493=VERTEX_POINT ( 'NONE', #74906 ) ;
#2497=CARTESIAN_POINT ( 'NONE',  ( -20.46002591053339970, 1487.323977817510013, 205.7581023369010040 ) ) ;
#2507=CARTESIAN_POINT ( 'NONE',  ( 1.448833437790000067, 1515.064791419390076, 213.4512947760589725 ) ) ;
#2515=CARTESIAN_POINT ( 'NONE',  ( -1.041670117440000043, 1431.845129037589913, 200.7519452021190034 ) ) ;
#2516=ADVANCED_FACE ( 'NONE', ( #76536 ), #83285, .T. ) ;
#2518=CARTESIAN_POINT ( 'NONE',  ( -1.441032304519999974, 1508.469141107589849, 220.8031696840990037 ) ) ;
#2523=CARTESIAN_POINT ( 'NONE',  ( 2.117784065689999995, 1485.870414137690204, 198.4209573190990170 ) ) ;
#2524=CARTESIAN_POINT ( 'NONE',  ( 5.461196333839980710, 1466.354709272569835, 200.5519884797059831 ) ) ;
#2530=EDGE_CURVE ( 'NONE', #53058, #98779, #37933, .T. ) ;
#2539=VERTEX_POINT ( 'NONE', #82737 ) ;
#2540=CARTESIAN_POINT ( 'NONE',  ( -11.38338690025777566, 1501.299005368582584, 207.9712302931637851 ) ) ;
#2541=CARTESIAN_POINT ( 'NONE',  ( -13.58182138314900023, 1508.547225165770215, 210.2471086096300041 ) ) ;
#2542=CARTESIAN_POINT ( 'NONE',  ( -19.67699484670000132, 1505.884115603990040, 219.0034652596590092 ) ) ;
#2544=CARTESIAN_POINT ( 'NONE',  ( -9.939836244837959356, 1438.908082076499795, 209.7414840783459908 ) ) ;
#2548=CARTESIAN_POINT ( 'NONE',  ( 7.508655101499999596, 1425.090260414829800, 212.1994906295190049 ) ) ;
#2549=CARTESIAN_POINT ( 'NONE',  ( -18.65941870309999828, 1468.219763198689861, 201.0822021908089994 ) ) ;
#2551=FACE_OUTER_BOUND ( 'NONE', #82195, .T. ) ;
#2554=EDGE_CURVE ( 'NONE', #73642, #32988, #47243, .T. ) ;
#2556=CARTESIAN_POINT ( 'NONE',  ( 4.492546581380000958, 1453.878649273890005, 217.3453973181289882 ) ) ;
#2558=ORIENTED_EDGE ( 'NONE', *, *, #1457, .F. ) ;
#2567=CARTESIAN_POINT ( 'NONE',  ( -2.765433514615380339, 1464.871865108300199, 198.4563297728979876 ) ) ;
#2579=CARTESIAN_POINT ( 'NONE',  ( -3.850432596239999672, 1454.142522157690109, 199.7891201249690027 ) ) ;
#2584=CARTESIAN_POINT ( 'NONE',  ( 7.892794852110000647, 1424.253103618490059, 211.9974886484589831 ) ) ;
#2605=CARTESIAN_POINT ( 'NONE',  ( 16.19637447162289945, 1427.902519050969886, 200.9814647519390007 ) ) ;
#2633=CARTESIAN_POINT ( 'NONE',  ( 3.255456066760000322, 1443.056962053689858, 217.4032295331390117 ) ) ;
#2641=CARTESIAN_POINT ( 'NONE',  ( 4.127868055549999582, 1487.366509936789953, 197.8725145131990075 ) ) ;
#2642=CARTESIAN_POINT ( 'NONE',  ( -4.996962189119175335, 1391.699467640956755, 203.5364589991260118 ) ) ;
#2647=CARTESIAN_POINT ( 'NONE',  ( -20.36287103150000277, 1507.711394158289977, 209.4617748114379765 ) ) ;
#2648=CARTESIAN_POINT ( 'NONE',  ( -2.721324782990000468, 1483.631500244790004, 198.7950877463990196 ) ) ;
#2649=CARTESIAN_POINT ( 'NONE',  ( -16.50171338560091883, 1417.502269239514590, 205.9477000315035582 ) ) ;
#2655=CARTESIAN_POINT ( 'NONE',  ( -11.02047842716129900, 1489.051096228969982, 214.3262357338399795 ) ) ;
#2656=CARTESIAN_POINT ( 'NONE',  ( 18.46111059403260057, 1471.786040807520067, 195.2229583357160152 ) ) ;
#2660=( BOUNDED_CURVE ( )  B_SPLINE_CURVE ( 3, ( #67670, #49211, #50851, #58160 ),
 .UNSPECIFIED., .F., .F. ) 
 B_SPLINE_CURVE_WITH_KNOTS ( ( 4, 4 ),
 ( 4.148177588089209777, 5.276600406385650643 ),
 .UNSPECIFIED. ) 
 CURVE ( )  GEOMETRIC_REPRESENTATION_ITEM ( )  RATIONAL_B_SPLINE_CURVE ( ( 1.000000000000000000, 0.8966737078530113703, 0.8966737078530113703, 1.000000000000000000 ) ) 
 REPRESENTATION_ITEM ( '' )  );
#2663=CARTESIAN_POINT ( 'NONE',  ( -18.65443362373700253, 1443.700676952599906, 211.5885854860179904 ) ) ;
#2669=ORIENTED_EDGE ( 'NONE', *, *, #55867, .F. ) ;
#2670=EDGE_LOOP ( 'NONE', ( #50814, #100737, #66353, #10024 ) ) ;
#2677=CARTESIAN_POINT ( 'NONE',  ( 9.820871455967859376, 1435.437962752369913, 208.9438784677120111 ) ) ;
#2679=CARTESIAN_POINT ( 'NONE',  ( 1.788309357509999975, 1480.920316621989969, 229.5180507505990022 ) ) ;
#2686=CARTESIAN_POINT ( 'NONE',  ( 1.959285310369999866, 1474.800623465989929, 220.3715843581990157 ) ) ;
#2687=CIRCLE ( 'NONE', #18699, 11.73843354579999954 ) ;
#2688=CARTESIAN_POINT ( 'NONE',  ( -10.99273638719279944, 1491.630725221910097, 209.8916735765129715 ) ) ;
#2691=CARTESIAN_POINT ( 'NONE',  ( -2.487924095911139943, 1509.038643251730036, 213.6090949890719912 ) ) ;
#2692=CARTESIAN_POINT ( 'NONE',  ( -21.57663945839999897, 1488.879494602689874, 202.2366601406689881 ) ) ;
#2694=CARTESIAN_POINT ( 'NONE',  ( 2.175409717514719593E-31, 1397.551704408390151, 209.1218459616989946 ) ) ;
#2699=CARTESIAN_POINT ( 'NONE',  ( -6.502638733110000402, 1458.675974398089920, 216.3652329231589704 ) ) ;
#2703=ORIENTED_EDGE ( 'NONE', *, *, #78909, .F. ) ;
#2711=CARTESIAN_POINT ( 'NONE',  ( -0.06724585139096760089, 1496.218926208830226, 221.4696802319550102 ) ) ;
#2713=AXIS2_PLACEMENT_3D ( 'NONE', #58056, #35038, #18772 ) ;
#2715=B_SPLINE_CURVE_WITH_KNOTS ( 'NONE', 3,
 ( #43010, #51962, #470, #87212, #28411, #2131, #36810, #19439, #17759, #69887, #1566, #52519, #44675, #10503, #53074, #95061, #86104, #53638, #43560, #18328, #44118, #102880, #61481, #27857, #78816, #104563, #34594, #62038, #96161, #85531, #9397, #77710, #1021, #35146, #71001, #9945, #8825, #78252, #62610, #95609, #87782, #11062, #45232, #68780, #27300, #26178, #35698, #79371, #18876 ),
 .UNSPECIFIED., .F., .F.,
 ( 4, 3, 3, 3, 3, 3, 3, 3, 3, 3, 3, 3, 3, 3, 3, 3, 4 ),
 ( 18.80849845009409904, 19.89523491153060064, 20.96856624117300072, 22.02675316388739901, 23.06319306041429940, 24.08912262180639985, 25.10114662952789999, 26.07035490390000021, 27.16676746860280289, 28.25787814313009960, 28.80892602879999842, 29.95369467953739928, 30.17821159120000019, 30.86285437239999752, 31.20517576310000152, 31.47730732964389944, 31.54749715370000018 ),
 .UNSPECIFIED. ) ;
#2716=CARTESIAN_POINT ( 'NONE',  ( -18.82283039985420103, 1508.494552192559922, 210.3700853329929998 ) ) ;
#2717=CARTESIAN_POINT ( 'NONE',  ( 8.720808663110000580, 1471.131229068790162, 214.3482137472890088 ) ) ;
#2718=CARTESIAN_POINT ( 'NONE',  ( -9.835408609723900852, 1439.978059041610095, 207.2081094720800252 ) ) ;
#2729=CARTESIAN_POINT ( 'NONE',  ( -0.9715543786848610530, 1467.707556206300069, 220.1856978582200099 ) ) ;
#2736=EDGE_CURVE ( 'NONE', #69095, #5037, #100762, .T. ) ;
#2744=CARTESIAN_POINT ( 'NONE',  ( 2.487922401834560038, 1508.551704408489968, 204.2892346663010130 ) ) ;
#2759=CARTESIAN_POINT ( 'NONE',  ( -17.00797534510000020, 1417.537219551289809, 207.7155427019889942 ) ) ;
#2761=CARTESIAN_POINT ( 'NONE',  ( -8.826538978809569613, 1481.764331815820015, 203.1249516821810062 ) ) ;
#2762=CARTESIAN_POINT ( 'NONE',  ( -9.233179502644661696, 1483.825061176979943, 201.6045247071639892 ) ) ;
#2766=CARTESIAN_POINT ( 'NONE',  ( -10.67290635632400075, 1462.958185458769776, 206.2378460151369950 ) ) ;
#2768=CARTESIAN_POINT ( 'NONE',  ( -14.48634920707452345, 1416.023439644662858, 203.8591738278827563 ) ) ;
#2770=CARTESIAN_POINT ( 'NONE',  ( -1.531246620494349863E-13, 1515.064792882589927, 204.7923971856590128 ) ) ;
#2771=B_SPLINE_SURFACE_WITH_KNOTS ( 'NONE', 5, 5, ( 
 ( #2231, #69988, #105217, #28505, #104656, #96824 ),
 ( #29062, #20093, #38010, #88952, #62136, #71660 ),
 ( #97895, #46433, #74934, #30701, #91159, #31251 ),
 ( #47518, #40756, #65434, #81640, #74388, #32363 ),
 ( #109082, #4417, #73265, #22827, #98993, #22268 ),
 ( #89507, #38544, #66544, #40206, #57032, #72723 ),
 ( #49180, #100647, #14434, #83310, #99543, #98453 ),
 ( #90602, #56470, #48632, #48066, #82200, #23933 ),
 ( #13325, #12798, #39086, #82762, #6054, #57585 ) ),
 .UNSPECIFIED., .F., .F., .F.,
 ( 6, 3, 6 ),
 ( 6, 6 ),
 ( 13.37707388139999942, 15.22166854640000011, 20.70300873780000117 ),
 ( 0.000000000000000000, 2.000000000000000000 ),
 .UNSPECIFIED. ) ;
#2772=CARTESIAN_POINT ( 'NONE',  ( -9.941270763631750995, 1461.322045364539918, 211.0756248058849849 ) ) ;
#2774=CARTESIAN_POINT ( 'NONE',  ( 14.37971982616849864, 1427.198226358100101, 195.4139261895699917 ) ) ;
#2775=ORIENTED_EDGE ( 'NONE', *, *, #42629, .T. ) ;
#2780=CARTESIAN_POINT ( 'NONE',  ( -9.445105015150314642, 1490.485136446142405, 189.9884643024701916 ) ) ;
#2782=DIRECTION ( 'NONE',  ( 9.500914144214121536E-47, -1.000000000000000000, 1.836970198721029688E-16 ) ) ;
#2785=CARTESIAN_POINT ( 'NONE',  ( 1.332267629549999902E-15, 1391.913060387289988, 209.1218459616989946 ) ) ;
#2788=CARTESIAN_POINT ( 'NONE',  ( 8.835383234542518949, 1451.659256596650039, 211.9451859889190075 ) ) ;
#2789=CARTESIAN_POINT ( 'NONE',  ( 3.584819811890000096, 1441.506325834089921, 217.6012887279890151 ) ) ;
#2790=VERTEX_POINT ( 'NONE', #961 ) ;
#2793=CARTESIAN_POINT ( 'NONE',  ( -4.683500221610000125, 1475.763858493990028, 199.9162038546990061 ) ) ;
#2796=ORIENTED_EDGE ( 'NONE', *, *, #85629, .T. ) ;
#2797=CARTESIAN_POINT ( 'NONE',  ( -13.97982192548539970, 1420.196024271650003, 195.9955606719640002 ) ) ;
#2804=CARTESIAN_POINT ( 'NONE',  ( -0.3695175741990010532, 1431.482447068790179, 217.8907632844189664 ) ) ;
#2810=CARTESIAN_POINT ( 'NONE',  ( 12.12282008797060051, 1491.484709589460181, 207.0783957174520253 ) ) ;
#2815=CARTESIAN_POINT ( 'NONE',  ( 0.1056718228839060025, 1496.587049647489948, 196.7558449521239936 ) ) ;
#2817=CARTESIAN_POINT ( 'NONE',  ( 11.91400850019820012, 1427.411956927870051, 208.4948976547729842 ) ) ;
#2824=EDGE_CURVE ( 'NONE', #27879, #39872, #55388, .T. ) ;
#2839=CARTESIAN_POINT ( 'NONE',  ( 2.581285063860000228, 1486.431383666189959, 219.6162510183990264 ) ) ;
#2843=ORIENTED_EDGE ( 'NONE', *, *, #95289, .T. ) ;
#2849=CARTESIAN_POINT ( 'NONE',  ( 9.582368326175020101, 1452.681705851589868, 210.9617576210509924 ) ) ;
#2850=CARTESIAN_POINT ( 'NONE',  ( 6.308047056989999568, 1423.705631131640075, 194.8804956342990238 ) ) ;
#2853=CARTESIAN_POINT ( 'NONE',  ( -8.689678022561432513, 1418.698340087812312, 196.3843397762474012 ) ) ;
#2859=EDGE_CURVE ( 'NONE', #36236, #24424, #73680, .T. ) ;
#2863=CARTESIAN_POINT ( 'NONE',  ( 10.93679547204000002, 1490.434980368090010, 209.9321327948960061 ) ) ;
#2868=EDGE_CURVE ( 'NONE', #92807, #71088, #52026, .T. ) ;
#2874=CARTESIAN_POINT ( 'NONE',  ( -4.733060768706960353, 1508.551704408389924, 219.7446302201209960 ) ) ;
#2878=CARTESIAN_POINT ( 'NONE',  ( -4.629079371760130179, 1468.688288304400203, 218.9163698581939741 ) ) ;
#2882=CARTESIAN_POINT ( 'NONE',  ( -12.69118497449169958, 1502.259178338380025, 210.4948179440679894 ) ) ;
#2883=CARTESIAN_POINT ( 'NONE',  ( 9.887380464539999636, 1491.508268245589989, 214.0815257268789935 ) ) ;
#2885=CARTESIAN_POINT ( 'NONE',  ( 8.814856031159362004, 1424.907964168706485, 195.6717967497336303 ) ) ;
#2887=CARTESIAN_POINT ( 'NONE',  ( -15.03612198640000130, 1503.549707945290038, 208.9024357440380015 ) ) ;
#2888=CARTESIAN_POINT ( 'NONE',  ( 10.38075141161009896, 1469.469397341999866, 204.6697731946910039 ) ) ;
#2899=EDGE_CURVE ( 'NONE', #36031, #103217, #14727, .T. ) ;
#2900=CARTESIAN_POINT ( 'NONE',  ( 12.69572402884860018, 1421.073347931960143, 203.4319052107520349 ) ) ;
#2902=CARTESIAN_POINT ( 'NONE',  ( -16.57704819438239952, 1418.510437161299933, 202.8789069828859795 ) ) ;
#2905=CARTESIAN_POINT ( 'NONE',  ( -2.381707907557049975, 1429.261286886310018, 200.0546762301680133 ) ) ;
#2914=CARTESIAN_POINT ( 'NONE',  ( -6.558658715760000035, 1477.685682757989753, 218.2637888529989993 ) ) ;
#2929=CARTESIAN_POINT ( 'NONE',  ( -15.42144792929999930, 1415.206394609319887, 209.1184241532129988 ) ) ;
#2952=CIRCLE ( 'NONE', #74470, 11.73460161499999899 ) ;
#2959=CARTESIAN_POINT ( 'NONE',  ( -1.920598319070000004, 1420.567467226830104, 193.8392728795989797 ) ) ;
#2962=CARTESIAN_POINT ( 'NONE',  ( -10.00816683080000047, 1449.847106855290122, 190.9047640032989932 ) ) ;
#2966=CARTESIAN_POINT ( 'NONE',  ( -5.093520080700000285, 1391.866578459589846, 203.7174121390089852 ) ) ;
#2968=CARTESIAN_POINT ( 'NONE',  ( 234.5897387251999930, 11221.53578756869865, -1757.702084499889907 ) ) ;
#2969=CARTESIAN_POINT ( 'NONE',  ( 19.30421002850018652, 1493.475027096192434, 199.7216057415594719 ) ) ;
#2975=CARTESIAN_POINT ( 'NONE',  ( -7179.982233247708791, -2339.246371527897281, 8259.998446794346819 ) ) ;
#2976=CARTESIAN_POINT ( 'NONE',  ( -13.81339225453198516, 1421.071880379611684, 210.6281576511377409 ) ) ;
#2979=VERTEX_POINT ( 'NONE', #83162 ) ;
#2981=ORIENTED_EDGE ( 'NONE', *, *, #46007, .F. ) ;
#2994=CARTESIAN_POINT ( 'NONE',  ( 2.487935123032369855, 1509.038615930399828, 204.6345961886270004 ) ) ;
#2997=CARTESIAN_POINT ( 'NONE',  ( -19.86622907060200305, 1443.388380008240119, 213.1207143647550311 ) ) ;
#3002=VERTEX_POINT ( 'NONE', #82614 ) ;
#3007=CARTESIAN_POINT ( 'NONE',  ( -2.031883580139580037, 1464.998375551469962, 198.3053770173009980 ) ) ;
#3027=CARTESIAN_POINT ( 'NONE',  ( -1.858949912414051386, 1455.785754466377284, 218.4293971133010359 ) ) ;
#3030=CARTESIAN_POINT ( 'NONE',  ( -6.690645534649999782, 1508.290528910890089, 219.9963685916989959 ) ) ;
#3032=CARTESIAN_POINT ( 'NONE',  ( 18.25280056480000113, 1432.153207019990077, 210.9297336666290050 ) ) ;
#3041=CARTESIAN_POINT ( 'NONE',  ( -4.853142760347620488, 1483.079447084539879, 199.6457431982469757 ) ) ;
#3053=CARTESIAN_POINT ( 'NONE',  ( -9.173772188490959323, 1450.560542621009972, 208.1432906865220218 ) ) ;
#3059=CARTESIAN_POINT ( 'NONE',  ( 0.7244299515159999814, 1515.369718807090067, 213.4098813832590054 ) ) ;
#3066=CARTESIAN_POINT ( 'NONE',  ( 3.322123243643906765, 1445.528383361184751, 200.7448775392205675 ) ) ;
#3070=CARTESIAN_POINT ( 'NONE',  ( -1.544604216069999980, 1508.025075525790044, 220.8982248008990155 ) ) ;
#3074=CARTESIAN_POINT ( 'NONE',  ( 2.315006021250000323, 1485.018218158490072, 198.6293828328989832 ) ) ;
#3075=CARTESIAN_POINT ( 'NONE',  ( 10.16195519437919970, 1469.411650742470101, 205.1025830150449849 ) ) ;
#3077=CARTESIAN_POINT ( 'NONE',  ( 3.092030599670000157, 1499.597189252489898, 201.0134171835890129 ) ) ;
#3079=CARTESIAN_POINT ( 'NONE',  ( 7.500055757779999333, 1423.184307743249974, 213.6185429247490219 ) ) ;
#3081=VECTOR ( 'NONE', #105652, 999.9999999999998863 ) ;
#3083=CARTESIAN_POINT ( 'NONE',  ( -11.10658002539999956, 1483.002145788689859, 204.7825228467889929 ) ) ;
#3090=CARTESIAN_POINT ( 'NONE',  ( -11.33134919748442471, 1502.978141622408202, 207.0767717826675209 ) ) ;
#3091=CARTESIAN_POINT ( 'NONE',  ( -13.58559797177369965, 1508.489012943990019, 209.9933550906049788 ) ) ;
#3098=CARTESIAN_POINT ( 'NONE',  ( 7.897123973650000295, 1424.702922360419961, 211.7415114879590021 ) ) ;
#3105=CARTESIAN_POINT ( 'NONE',  ( 7.892605823620001182, 1452.443926081389918, 214.1248619204189936 ) ) ;
#3129=CARTESIAN_POINT ( 'NONE',  ( -3.389499785119999942, 1455.558962287190070, 200.3052658018689840 ) ) ;
#3135=CARTESIAN_POINT ( 'NONE',  ( 7.901854723500001398, 1423.732064818020035, 212.4548200391890020 ) ) ;
#3143=EDGE_CURVE ( 'NONE', #8260, #27116, #82750, .T. ) ;
#3147=CARTESIAN_POINT ( 'NONE',  ( 4.326992699989999913, 1515.158586642790169, 209.1218459614979963 ) ) ;
#3156=ADVANCED_FACE ( 'NONE', ( #5221 ), #75032, .T. ) ;
#3161=ORIENTED_EDGE ( 'NONE', *, *, #108302, .T. ) ;
#3165=VERTEX_POINT ( 'NONE', #86883 ) ;
#3167=CARTESIAN_POINT ( 'NONE',  ( -4.730384175031817406, 1508.603735226452955, 206.6339107270123066 ) ) ;
#3176=CARTESIAN_POINT ( 'NONE',  ( 10.51972982329080075, 1470.321793319200196, 208.5210859618010204 ) ) ;
#3178=VERTEX_POINT ( 'NONE', #51640 ) ;
#3180=ADVANCED_FACE ( 'NONE', ( #153 ), #68846, .T. ) ;
#3181=EDGE_CURVE ( 'NONE', #93757, #70633, #100209, .T. ) ;
#3186=CARTESIAN_POINT ( 'NONE',  ( 4.771249618659999747, 1425.961663979450122, 210.6061160235690295 ) ) ;
#3187=EDGE_CURVE ( 'NONE', #62493, #65430, #7980, .T. ) ;
#3189=CARTESIAN_POINT ( 'NONE',  ( 2.967450459799999773, 1441.849466645390066, 217.8449471930090056 ) ) ;
#3199=CARTESIAN_POINT ( 'NONE',  ( 20.49831092009999978, 1496.178973653789853, 204.1013708937389879 ) ) ;
#3205=CARTESIAN_POINT ( 'NONE',  ( -3.235066836120000122, 1485.183772486390126, 198.0938001695989783 ) ) ;
#3210=CARTESIAN_POINT ( 'NONE',  ( -8.304037367963141847, 1489.233820626979877, 216.5016543136719918 ) ) ;
#3211=CARTESIAN_POINT ( 'NONE',  ( -21.51338718909140013, 1505.551624535830115, 209.1218323743090082 ) ) ;
#3214=CARTESIAN_POINT ( 'NONE',  ( -5.171974582749985672, 1391.896122674977278, 214.5527304933138737 ) ) ;
#3215=CARTESIAN_POINT ( 'NONE',  ( 6.732768143660000426, 1427.455436918209898, 213.9186140547390096 ) ) ;
#3241=ORIENTED_EDGE ( 'NONE', *, *, #26966, .F. ) ;
#3242=CARTESIAN_POINT ( 'NONE',  ( -3.961806501176829975, 1508.551704407889929, 213.6667149433449993 ) ) ;
#3244=CARTESIAN_POINT ( 'NONE',  ( -17.92831943059999844, 1489.596456395790028, 195.2426190332990075 ) ) ;
#3250=CARTESIAN_POINT ( 'NONE',  ( 4.328687482160760602, 1515.093865522929946, 210.3164017889689887 ) ) ;
#3252=CARTESIAN_POINT ( 'NONE',  ( -7.055457375169999601, 1459.495818635790101, 217.3326011958589845 ) ) ;
#3256=CARTESIAN_POINT ( 'NONE',  ( -8.818304860959999658, 1423.702314450679978, 208.5313052791129849 ) ) ;
#3261=DIRECTION ( 'NONE',  ( 0.000000000000000000, 4.493040424372315268E-15, -1.000000000000000000 ) ) ;
#3263=CARTESIAN_POINT ( 'NONE',  ( 4.163336342339999869E-15, 1416.177402202029953, 209.1218459616989946 ) ) ;
#3265=CARTESIAN_POINT ( 'NONE',  ( 3.628818056492709943, 1505.602008419380127, 221.3635114792730292 ) ) ;
#3268=CARTESIAN_POINT ( 'NONE',  ( 9.374255435350001164, 1470.737626183290104, 212.9758214168889765 ) ) ;
#3269=CARTESIAN_POINT ( 'NONE',  ( -9.907124821256790170, 1439.782531377399891, 207.6975214335770090 ) ) ;
#3274=CARTESIAN_POINT ( 'NONE',  ( 8.957671594842102181, 1435.649687873459925, 208.1941622349180250 ) ) ;
#3279=CARTESIAN_POINT ( 'NONE',  ( 2.170280451284099854, 1466.842894365370057, 219.9682480396010078 ) ) ;
#3285=EDGE_CURVE ( 'NONE', #96209, #14911, #48053, .T. ) ;
#3291=CARTESIAN_POINT ( 'NONE',  ( 0.5594537969809989519, 1444.672526988890013, 215.3952916019189843 ) ) ;
#3310=ORIENTED_EDGE ( 'NONE', *, *, #50885, .T. ) ;
#3312=CARTESIAN_POINT ( 'NONE',  ( -5.102340803919999779, 1483.010473641589897, 199.7820758705289848 ) ) ;
#3313=AXIS2_PLACEMENT_3D ( 'NONE', #66122, #56597, #100245 ) ;
#3329=CARTESIAN_POINT ( 'NONE',  ( 9.412245003297918799, 1500.377496655100003, 202.5220683207009813 ) ) ;
#3333=CARTESIAN_POINT ( 'NONE',  ( -1255.832924500349918, 1412.219004263330135, 209.0925205239309719 ) ) ;
#3340=CARTESIAN_POINT ( 'NONE',  ( -4.679790880385569452, 1508.610720271750097, 205.9457817814489715 ) ) ;
#3342=CARTESIAN_POINT ( 'NONE',  ( -14.75858115399999981, 1415.739699861750069, 212.8702772705990185 ) ) ;
#3351=CARTESIAN_POINT ( 'NONE',  ( -2.360343982743250191, 1508.551704408389924, 220.0510488555580082 ) ) ;
#3354=FACE_OUTER_BOUND ( 'NONE', #40201, .T. ) ;
#3357=CARTESIAN_POINT ( 'NONE',  ( -0.1306346743340009997, 1430.514091579490014, 217.4937112845890113 ) ) ;
#3360=CARTESIAN_POINT ( 'NONE',  ( 2.040878228339999989, 1454.390661367689972, 215.4849015426389940 ) ) ;
#3364=CARTESIAN_POINT ( 'NONE',  ( 12.33879830033670011, 1492.074832325789885, 209.1388286321879946 ) ) ;
#3369=CARTESIAN_POINT ( 'NONE',  ( -1.306867980634530024, 1496.219773069479970, 196.8427661518120146 ) ) ;
#3379=CARTESIAN_POINT ( 'NONE',  ( -3.156402467807082335, 1454.645949074940972, 199.8283705214046506 ) ) ;
#3381=CARTESIAN_POINT ( 'NONE',  ( 1.968601617930000103, 1498.935401861390119, 197.9561509160990056 ) ) ;
#3382=AXIS2_PLACEMENT_3D ( 'NONE', #13665, #16278, #50481 ) ;
#3383=B_SPLINE_CURVE_WITH_KNOTS ( 'NONE', 5,
 ( #71103, #62715, #96835, #77276, #34699, #11714 ),
 .UNSPECIFIED., .F., .F.,
 ( 6, 6 ),
 ( 0.000000000000000000, 1.000000000000000000 ),
 .UNSPECIFIED. ) ;
#3392=CARTESIAN_POINT ( 'NONE',  ( 2.918982678559999933, 1485.831548431689953, 219.6257443891990135 ) ) ;
#3402=CARTESIAN_POINT ( 'NONE',  ( 5.145309007309999849, 1422.426130173420006, 194.5914466168989918 ) ) ;
#3417=ORIENTED_EDGE ( 'NONE', *, *, #69223, .T. ) ;
#3420=ORIENTED_EDGE ( 'NONE', *, *, #96056, .T. ) ;
#3425=CARTESIAN_POINT ( 'NONE',  ( -7.120274244888039838, 1470.094334173359812, 216.5229890130249828 ) ) ;
#3428=CARTESIAN_POINT ( 'NONE',  ( -0.02549190311316479676, 1475.332589245109830, 220.5468605150740302 ) ) ;
#3429=DIRECTION ( 'NONE',  ( 4.465978680329379737E-17, 1.000000000000000000, -2.349386720892264891E-16 ) ) ;
#3432=CARTESIAN_POINT ( 'NONE',  ( -19.29649804419999981, 1504.799431328789979, 209.3162768295289879 ) ) ;
#3434=CARTESIAN_POINT ( 'NONE',  ( 12.45034049356619832, 1421.619540909540092, 207.5029415923690124 ) ) ;
#3443=CARTESIAN_POINT ( 'NONE',  ( 4.875706362549999895, 1506.017256195089885, 219.8452990541989891 ) ) ;
#3444=CARTESIAN_POINT ( 'NONE',  ( -15.41742678890000029, 1415.853057449160133, 210.9644741221289905 ) ) ;
#3445=CARTESIAN_POINT ( 'NONE',  ( -15.86086750622509989, 1419.980772078519976, 210.7345574348329933 ) ) ;
#3447=CARTESIAN_POINT ( 'NONE',  ( -16.78154512266720033, 1418.363846789659874, 203.4619184960750147 ) ) ;
#3448=CARTESIAN_POINT ( 'NONE',  ( 19.60792669039999936, 1475.100271358290229, 204.3343059087790152 ) ) ;
#3458=EDGE_CURVE ( 'NONE', #77864, #90721, #54814, .T. ) ;
#3459=CARTESIAN_POINT ( 'NONE',  ( -12.74982669920128941, 1462.837610516389304, 224.9934397671993054 ) ) ;
#3474=CARTESIAN_POINT ( 'NONE',  ( -16.80706507779999725, 1416.677443236529825, 209.1193462365459936 ) ) ;
#3479=DIRECTION ( 'NONE',  ( 1.273732310806389972E-11, 4.864864992887659796E-10, 1.000000000000000000 ) ) ;
#3496=CARTESIAN_POINT ( 'NONE',  ( 4.324478665330000027, 1515.254593745989951, 208.3983361640229930 ) ) ;
#3497=ORIENTED_EDGE ( 'NONE', *, *, #50233, .F. ) ;
#3503=CARTESIAN_POINT ( 'NONE',  ( -11.23368485119999960, 1500.117004219489900, 211.0002778243189994 ) ) ;
#3509=EDGE_CURVE ( 'NONE', #105125, #50173, #92804, .T. ) ;
#3510=CARTESIAN_POINT ( 'NONE',  ( 18.80805864981130071, 1458.321402826489930, 220.5644953607610148 ) ) ;
#3516=CARTESIAN_POINT ( 'NONE',  ( 1966.823930461590180, 11221.53578756869865, 443.7115846868979929 ) ) ;
#3522=CARTESIAN_POINT ( 'NONE',  ( 11.23549300526389949, 1502.543211738040100, 212.3416208334529927 ) ) ;
#3524=CARTESIAN_POINT ( 'NONE',  ( -13.70181463665861621, 1421.117064391099802, 210.6307364177106649 ) ) ;
#3531=DIRECTION ( 'NONE',  ( -0.9334681682710679329, 0.3057582888762500062, -0.1874807926378720124 ) ) ;
#3538=CARTESIAN_POINT ( 'NONE',  ( -1.044338232960000168, 1469.645465345889988, 219.1445103612989840 ) ) ;
#3540=CARTESIAN_POINT ( 'NONE',  ( 10.04557648923880109, 1482.796278672210065, 212.7028893834429937 ) ) ;
#3544=CARTESIAN_POINT ( 'NONE',  ( -20.55780381099999943, 1485.073231501690088, 207.1087988815990002 ) ) ;
#3548=CARTESIAN_POINT ( 'NONE',  ( -1.731903628061610023, 1431.483103224190017, 200.9088633058729840 ) ) ;
#3551=EDGE_CURVE ( 'NONE', #79909, #47729, #20081, .T. ) ;
#3557=CARTESIAN_POINT ( 'NONE',  ( 9.774667823450000625, 1462.791341090990045, 210.7173602730590005 ) ) ;
#3571=CARTESIAN_POINT ( 'NONE',  ( -17.98592010575266187, 1508.456915429008859, 211.9106567536674106 ) ) ;
#3582=B_SPLINE_SURFACE_WITH_KNOTS ( 'NONE', 5, 5, ( 
 ( #34061, #491, #33489, #34614, #51420, #58724 ),
 ( #68800, #76619, #74985, #91755, #109133, #67138 ),
 ( #32416, #84467, #68254, #66595, #100699, #83908 ),
 ( #25645, #93410, #67691, #8848, #101236, #58176 ),
 ( #41919, #50342, #92305, #15575, #101799, #49777 ),
 ( #50874, #7214, #75538, #109672, #24536, #92859 ),
 ( #16135, #7755, #76075, #59293, #110216, #25089 ),
 ( #16675, #85003, #44697, #20017, #3256, #1586 ),
 ( #51983, #94508, #103459, #17783, #27878, #79940 ),
 ( #88337, #71019, #69350, #10522, #53094, #104024 ),
 ( #60387, #26766, #60954, #45255, #95630, #11088 ),
 ( #79390, #37383, #9418, #43580, #36272, #77730 ),
 ( #105139, #1043, #27319, #61500, #70462, #96184 ),
 ( #86124, #54212, #28429, #35165, #95081, #18347 ),
 ( #11629, #62629, #52538, #86671, #9967, #44138 ) ),
 .UNSPECIFIED., .F., .F., .F.,
 ( 6, 3, 3, 3, 6 ),
 ( 6, 6 ),
 ( 10.77847743720000118, 25.90271913459999809, 41.12370487549999609, 56.51454383889999633, 65.55090256170001339 ),
 ( 0.000000000000000000, 2.000000000000000000 ),
 .UNSPECIFIED. ) ;
#3589=CARTESIAN_POINT ( 'NONE',  ( -2.646473796664690070, 1483.649213716789973, 198.7830764605120066 ) ) ;
#3596=CARTESIAN_POINT ( 'NONE',  ( -14.68065129330000040, 1415.999375028279928, 204.4212104945090118 ) ) ;
#3598=CARTESIAN_POINT ( 'NONE',  ( 12.23993107200000097, 1420.119835428209853, 199.7451907216789948 ) ) ;
#3599=EDGE_CURVE ( 'NONE', #23842, #58146, #11963, .T. ) ;
#3604=ORIENTED_EDGE ( 'NONE', *, *, #53028, .T. ) ;
#3608=CARTESIAN_POINT ( 'NONE',  ( -1.466212339980000001, 1515.204044912790096, 213.4476482949990270 ) ) ;
#3612=CARTESIAN_POINT ( 'NONE',  ( 21.13734888319999783, 1496.938803861589804, 209.1218459616989946 ) ) ;
#3617=CARTESIAN_POINT ( 'NONE',  ( 9.619198284380544806, 1463.334820347890400, 214.5538614071193706 ) ) ;
#3618=CARTESIAN_POINT ( 'NONE',  ( 3.246115288789999997, 1507.570166992290069, 220.3920571188990039 ) ) ;
#3631=CARTESIAN_POINT ( 'NONE',  ( 17.70437741359999961, 1453.580057579390086, 200.5051001409389926 ) ) ;
#3640=VERTEX_POINT ( 'NONE', #52483 ) ;
#3641=CARTESIAN_POINT ( 'NONE',  ( -11.32996165527507415, 1502.367014232210977, 207.2237320763624666 ) ) ;
#3646=CARTESIAN_POINT ( 'NONE',  ( -2.487934962309999776, 1508.551704408389924, 204.1347675205190058 ) ) ;
#3651=CARTESIAN_POINT ( 'NONE',  ( 7.436161634030000300, 1426.180031595399896, 212.4856801342990025 ) ) ;
#3652=CARTESIAN_POINT ( 'NONE',  ( 18.32584137559999959, 1473.764089050990151, 194.8973954003990059 ) ) ;
#3654=CARTESIAN_POINT ( 'NONE',  ( -21.12854634993719927, 1507.715432715349834, 209.4790063854959783 ) ) ;
#3660=ORIENTED_EDGE ( 'NONE', *, *, #109695, .T. ) ;
#3669=CARTESIAN_POINT ( 'NONE',  ( -1.720875739424750028, 1464.150623787119912, 199.3240472289820104 ) ) ;
#3676=ORIENTED_EDGE ( 'NONE', *, *, #21579, .F. ) ;
#3682=CARTESIAN_POINT ( 'NONE',  ( -4.360511100030000087, 1454.978814073790090, 200.7714291330290166 ) ) ;
#3687=ORIENTED_EDGE ( 'NONE', *, *, #36438, .F. ) ;
#3700=LINE ( 'NONE', #36174, #92569 ) ;
#3708=CARTESIAN_POINT ( 'NONE',  ( 13.54784204829999972, 1426.885522674909907, 197.1450391101479909 ) ) ;
#3717=CARTESIAN_POINT ( 'NONE',  ( -2.583034826040000009, 1429.324951399489919, 200.5039866108990054 ) ) ;
#3726=CARTESIAN_POINT ( 'NONE',  ( -16.11470690007832118, 1416.382804326506175, 208.7747741149743490 ) ) ;
#3728=CARTESIAN_POINT ( 'NONE',  ( 10.06225300309310100, 1469.716777501389970, 209.4998798077870106 ) ) ;
#3731=CARTESIAN_POINT ( 'NONE',  ( 10.52443147309969973, 1481.186296556219986, 208.2194658927409989 ) ) ;
#3733=CARTESIAN_POINT ( 'NONE',  ( 5.151075264148989419, 1490.744830062189976, 188.9005219498210124 ) ) ;
#3736=CARTESIAN_POINT ( 'NONE',  ( 2.583256299099999875, 1441.752764794789982, 218.3094755959190252 ) ) ;
#3743=CARTESIAN_POINT ( 'NONE',  ( -19.75595884730000051, 1465.302413857089959, 208.1547143399459685 ) ) ;
#3747=CARTESIAN_POINT ( 'NONE',  ( -9.903567409750580808, 1472.178920281909996, 211.4406132415489878 ) ) ;
#3751=CARTESIAN_POINT ( 'NONE',  ( -8.899549366109999582, 1508.515584743789987, 219.0073388492789945 ) ) ;
#3754=CARTESIAN_POINT ( 'NONE',  ( -3.082606035640000464, 1484.897200977490229, 198.4345628581990013 ) ) ;
#3759=CARTESIAN_POINT ( 'NONE',  ( 3.938385272561739647, 1493.417418013209954, 219.5392876527429848 ) ) ;
#3760=CARTESIAN_POINT ( 'NONE',  ( -10.29417939532470072, 1490.744234622979775, 212.9867478681659918 ) ) ;
#3761=CARTESIAN_POINT ( 'NONE',  ( 20.81805062950000362, 1457.016307409189949, 206.8942079858889826 ) ) ;
#3766=ORIENTED_EDGE ( 'NONE', *, *, #88002, .F. ) ;
#3778=CARTESIAN_POINT ( 'NONE',  ( 9.723333314712000686, 1436.167293238569982, 210.6196431544800021 ) ) ;
#3783=CARTESIAN_POINT ( 'NONE',  ( -19.84399396720000297, 1467.318719066990070, 208.1502282180090333 ) ) ;
#3786=CARTESIAN_POINT ( 'NONE',  ( 1.554992009126110020, 1515.071272245649880, 213.4511250689819803 ) ) ;
#3788=CARTESIAN_POINT ( 'NONE',  ( -5.864936813312239927, 1477.472823321480064, 219.0780053889600083 ) ) ;
#3796=CARTESIAN_POINT ( 'NONE',  ( -21.39151623717510020, 1487.103275126709832, 201.9631718257530224 ) ) ;
#3798=CARTESIAN_POINT ( 'NONE',  ( 7.516769032520000060, 1422.170349638209927, 195.6959265412990021 ) ) ;
#3803=CARTESIAN_POINT ( 'NONE',  ( -4.987078435459999071, 1508.551704408389924, 209.1218459616989946 ) ) ;
#3813=ORIENTED_EDGE ( 'NONE', *, *, #46047, .T. ) ;
#3817=EDGE_CURVE ( 'NONE', #106056, #88894, #75711, .T. ) ;
#3824=CARTESIAN_POINT ( 'NONE',  ( 5.826428076080000906, 1473.811884028689974, 218.9454251420289950 ) ) ;
#3825=CARTESIAN_POINT ( 'NONE',  ( -13.83457784759895937, 1504.369317328791112, 226.5199076315979312 ) ) ;
#3830=CARTESIAN_POINT ( 'NONE',  ( 8.536223301210858594, 1436.502018257360078, 207.9555195538749786 ) ) ;
#3835=CARTESIAN_POINT ( 'NONE',  ( 2.993162530245609965, 1466.561220909740086, 219.7621249222650022 ) ) ;
#3845=ORIENTED_EDGE ( 'NONE', *, *, #950, .F. ) ;
#3850=B_SPLINE_CURVE_WITH_KNOTS ( 'NONE', 3,
 ( #45604, #96535, #79746, #63518, #71375, #104375, #9757, #18148, #105487, #28778, #27125, #87592, #62978 ),
 .UNSPECIFIED., .F., .F.,
 ( 4, 3, 3, 3, 4 ),
 ( -7.154418212010000389, -6.085421029112350055, -5.016423846214689952, -3.988585745587499787, -2.933308256780000178 ),
 .UNSPECIFIED. ) ;
#3863=CARTESIAN_POINT ( 'NONE',  ( -17.23909798190000231, 1417.482756323010108, 206.7388844422490024 ) ) ;
#3866=CARTESIAN_POINT ( 'NONE',  ( -20.37344316928624721, 1508.015640753926164, 209.5635218970269023 ) ) ;
#3874=CARTESIAN_POINT ( 'NONE',  ( -10.32771419153329973, 1461.601508178220001, 211.2214880053600154 ) ) ;
#3886=CARTESIAN_POINT ( 'NONE',  ( -2.847678236428970333, 1430.845636561999981, 201.2564352187889938 ) ) ;
#3896=CARTESIAN_POINT ( 'NONE',  ( 4.001327954560360389, 1508.551704408389924, 204.6458544173759719 ) ) ;
#3898=VERTEX_POINT ( 'NONE', #40452 ) ;
#3899=CARTESIAN_POINT ( 'NONE',  ( 22.14278947725500402, 1473.984036977170035, 210.1089657997129905 ) ) ;
#3904=CARTESIAN_POINT ( 'NONE',  ( -6.404454395499999286, 1464.203453065390022, 200.1263287045289871 ) ) ;
#3913=CARTESIAN_POINT ( 'NONE',  ( 11.87221919846740015, 1491.806965132240066, 208.7302600617219923 ) ) ;
#3918=CARTESIAN_POINT ( 'NONE',  ( -18.69648219331439876, 1441.918081136590217, 210.3870465119969992 ) ) ;
#3919=CARTESIAN_POINT ( 'NONE',  ( -3.467940602053699806, 1495.562067921990092, 197.2905559617530002 ) ) ;
#3922=CARTESIAN_POINT ( 'NONE',  ( -14.46094609939999920, 1420.539308687509902, 213.8039270598989958 ) ) ;
#3934=CARTESIAN_POINT ( 'NONE',  ( 0.7572375962070010402, 1498.197839107489926, 197.8134798819990010 ) ) ;
#3935=CARTESIAN_POINT ( 'NONE',  ( -3.675448282928950317, 1497.092948350399865, 201.5013805017089794 ) ) ;
#3936=VERTEX_POINT ( 'NONE', #96380 ) ;
#3942=CARTESIAN_POINT ( 'NONE',  ( 2.086548178679999754, 1515.551704408389924, 205.2922258481490303 ) ) ;
#3944=CARTESIAN_POINT ( 'NONE',  ( 1.088119754170000064, 1486.968603087390193, 219.9165972894990091 ) ) ;
#3951=ORIENTED_EDGE ( 'NONE', *, *, #14255, .F. ) ;
#3954=CARTESIAN_POINT ( 'NONE',  ( 7.207469458989999467, 1424.355561564639856, 194.9835187250990032 ) ) ;
#3958=CARTESIAN_POINT ( 'NONE',  ( -10.57419901610000146, 1462.298693876490006, 208.7178814602820012 ) ) ;
#3975=CARTESIAN_POINT ( 'NONE',  ( -3.644778954545839778, 1508.551704408389924, 219.9243067801160123 ) ) ;
#3977=CARTESIAN_POINT ( 'NONE',  ( -7.960864549025298942, 1469.836596664489889, 216.0273995464790175 ) ) ;
#3979=CARTESIAN_POINT ( 'NONE',  ( 8.765728093939998189, 1421.055606564249956, 196.4760046562989828 ) ) ;
#3982=CARTESIAN_POINT ( 'NONE',  ( 11.12152504562100042, 1478.725870727130086, 205.8941487266770025 ) ) ;
#3984=CARTESIAN_POINT ( 'NONE',  ( -12.78476385600000143, 1502.707311016190033, 209.0177136757029928 ) ) ;
#3985=CARTESIAN_POINT ( 'NONE',  ( 12.26636271253249966, 1421.698877206780026, 207.4435041203790036 ) ) ;
#3993=CARTESIAN_POINT ( 'NONE',  ( 4.133200439670000392, 1506.299374241689975, 220.1647597449990030 ) ) ;
#3996=CARTESIAN_POINT ( 'NONE',  ( 2.022791977769999860, 1430.155356877590066, 217.3490746647090077 ) ) ;
#3998=CARTESIAN_POINT ( 'NONE',  ( -16.09575332200000020, 1416.289980099749982, 209.1849711052219902 ) ) ;
#3999=CARTESIAN_POINT ( 'NONE',  ( -0.1852938298213350210, 1430.295842153490185, 199.7081761581629848 ) ) ;
#4003=CARTESIAN_POINT ( 'NONE',  ( 7.679909121233859715, 1460.810760006640066, 203.1061546417070076 ) ) ;
#4006=CARTESIAN_POINT ( 'NONE',  ( 9.549000552458089430, 1470.075890067440014, 212.3436661921319910 ) ) ;
#4022=CARTESIAN_POINT ( 'NONE',  ( 2.554632337009709708, 1456.353935948870230, 219.4317766317170140 ) ) ;
#4028=CARTESIAN_POINT ( 'NONE',  ( -11.02808036529999924, 1492.177362994390023, 209.7513178175030077 ) ) ;
#4029=CARTESIAN_POINT ( 'NONE',  ( -3.660988608500000296, 1468.712036633390198, 189.5324782634990015 ) ) ;
#4037=CARTESIAN_POINT ( 'NONE',  ( -12.22358767350790032, 1490.666492278739724, 208.1734027058400045 ) ) ;
#4042=CARTESIAN_POINT ( 'NONE',  ( 2.183428632720000095, 1507.960443100289922, 217.8271517235889974 ) ) ;
#4045=DIRECTION ( 'NONE',  ( 1.000000000000000000, 0.000000000000000000, 0.000000000000000000 ) ) ;
#4047=CARTESIAN_POINT ( 'NONE',  ( -11.18708202009999830, 1500.025273076890244, 211.2389607902390196 ) ) ;
#4049=CARTESIAN_POINT ( 'NONE',  ( -0.5536948142769980707, 1422.303198269830091, 193.2759312063989796 ) ) ;
#4050=EDGE_CURVE ( 'NONE', #29796, #77481, #97817, .T. ) ;
#4053=CARTESIAN_POINT ( 'NONE',  ( -18.69626595349999931, 1468.616571719990134, 201.1221850591790030 ) ) ;
#4065=EDGE_LOOP ( 'NONE', ( #105815, #40794, #21686, #105689, #86561 ) ) ;
#4066=CARTESIAN_POINT ( 'NONE',  ( 3.281831459213320201, 1466.303209658950209, 198.5678429405679992 ) ) ;
#4067=CARTESIAN_POINT ( 'NONE',  ( -11.36636202294226727, 1422.064850992264837, 210.6381225563648911 ) ) ;
#4073=CARTESIAN_POINT ( 'NONE',  ( 2.563005697779590086, 1485.055789815510025, 220.6962468248860034 ) ) ;
#4074=LINE ( 'NONE', #62914, #42142 ) ;
#4077=CARTESIAN_POINT ( 'NONE',  ( 6.594885160195530283, 1463.733219486340204, 209.8009738102450115 ) ) ;
#4081=CARTESIAN_POINT ( 'NONE',  ( 12.52297189095030028, 1501.145799326159931, 211.3282646751150082 ) ) ;
#4083=B_SPLINE_CURVE_WITH_KNOTS ( 'NONE', 3,
 ( #106969, #5060, #39206, #89615, #73383, #22381, #31360, #49840, #26263 ),
 .UNSPECIFIED., .F., .F.,
 ( 4, 1, 2, 2, 4 ),
 ( 0.000000000000000000, 0.2500000000002982614, 0.3750000000003418932, 0.5000000000003855805, 1.000000000000000000 ),
 .UNSPECIFIED. ) ;
#4085=CARTESIAN_POINT ( 'NONE',  ( 2.824339754329999952, 1434.323903598489778, 204.0183183669190043 ) ) ;
#4086=ORIENTED_EDGE ( 'NONE', *, *, #51369, .T. ) ;
#4087=CARTESIAN_POINT ( 'NONE',  ( -17.51543818720000090, 1417.552356044260023, 206.7803260803289902 ) ) ;
#4099=CARTESIAN_POINT ( 'NONE',  ( 2.024278636110000029, 1464.636130398189835, 199.4774878893790060 ) ) ;
#4107=CARTESIAN_POINT ( 'NONE',  ( 11.31476318222129862, 1478.684671585819842, 206.0074932402150125 ) ) ;
#4129=CARTESIAN_POINT ( 'NONE',  ( -4.720855738540000068, 1427.997322581190019, 206.3545885669889799 ) ) ;
#4130=ORIENTED_EDGE ( 'NONE', *, *, #86035, .T. ) ;
#4134=CARTESIAN_POINT ( 'NONE',  ( 10.47511427260239891, 1482.040461736080033, 210.7458695605469927 ) ) ;
#4135=CARTESIAN_POINT ( 'NONE',  ( -14.79119396799999997, 1415.837009589480203, 205.0101417669090154 ) ) ;
#4145=CARTESIAN_POINT ( 'NONE',  ( 1.842963430059999963, 1515.219201257890063, 213.4472514052690144 ) ) ;
#4150=CARTESIAN_POINT ( 'NONE',  ( -5.931789999490000298, 1459.036866685989935, 218.1324649368089865 ) ) ;
#4155=EDGE_CURVE ( 'NONE', #24424, #77584, #66711, .T. ) ;
#4167=CARTESIAN_POINT ( 'NONE',  ( -3.328126825706799963, 1508.551704408389924, 204.2788038780209945 ) ) ;
#4171=CARTESIAN_POINT ( 'NONE',  ( -3.767256085520910514, 1436.652614717099823, 227.2392139179829940 ) ) ;
#4178=CARTESIAN_POINT ( 'NONE',  ( 7.763749353059999692, 1427.458563954329975, 212.5755154428889853 ) ) ;
#4179=CARTESIAN_POINT ( 'NONE',  ( -21.47379552819999660, 1487.892728108790152, 202.0847255913190281 ) ) ;
#4184=CARTESIAN_POINT ( 'NONE',  ( 8.768686371710000316, 1452.910156834589998, 212.7670267765590211 ) ) ;
#4190=CARTESIAN_POINT ( 'NONE',  ( 3.066583199566000534E-32, 1507.508085020990166, 209.1218459616989946 ) ) ;
#4192=CARTESIAN_POINT ( 'NONE',  ( -2.900859510217989268, 1441.812960597777874, 200.7451303979236741 ) ) ;
#4209=CARTESIAN_POINT ( 'NONE',  ( 11.45399678350000094, 1491.761485200589959, 209.6397955211830038 ) ) ;
#4227=ORIENTED_EDGE ( 'NONE', *, *, #87834, .F. ) ;
#4245=EDGE_CURVE ( 'NONE', #45310, #77584, #107936, .T. ) ;
#4253=CARTESIAN_POINT ( 'NONE',  ( 11.03115274839999849, 1422.777860647609941, 206.2455307242489937 ) ) ;
#4254=CARTESIAN_POINT ( 'NONE',  ( 0.5537922756022227722, 1498.600653688011789, 197.8120951424002385 ) ) ;
#4260=CARTESIAN_POINT ( 'NONE',  ( 11.39902737117300013, 1471.112819660780133, 209.6184962109379910 ) ) ;
#4268=( BOUNDED_CURVE ( )  B_SPLINE_CURVE ( 3, ( #41739, #8674, #52376, #75898 ),
 .UNSPECIFIED., .F., .F. ) 
 B_SPLINE_CURVE_WITH_KNOTS ( ( 4, 4 ),
 ( 5.498078030758629886, 7.068189173309639806 ),
 .UNSPECIFIED. ) 
 CURVE ( )  GEOMETRIC_REPRESENTATION_ITEM ( )  RATIONAL_B_SPLINE_CURVE ( ( 1.000000000000000000, 0.8048993259320535998, 0.8048993259320535998, 1.000000000000000000 ) ) 
 REPRESENTATION_ITEM ( '' )  );
#4269=FACE_OUTER_BOUND ( 'NONE', #9190, .T. ) ;
#4270=CARTESIAN_POINT ( 'NONE',  ( 8.544339041751733532, 1424.594794760930426, 195.7981282794199842 ) ) ;
#4272=CARTESIAN_POINT ( 'NONE',  ( 2.744355238500000294, 1442.847804213789914, 217.5784138281389914 ) ) ;
#4277=CARTESIAN_POINT ( 'NONE',  ( -5.268918391659049405, 1464.422126824970292, 199.4426748585790108 ) ) ;
#4286=CARTESIAN_POINT ( 'NONE',  ( -8.927975590540000894, 1508.479955638390038, 219.0952217288690065 ) ) ;
#4290=CARTESIAN_POINT ( 'NONE',  ( -2.572869546270000196, 1484.598564647389821, 198.5804750205990103 ) ) ;
#4295=CARTESIAN_POINT ( 'NONE',  ( 5.485830631332369478, 1494.971428724189991, 220.2122593298520030 ) ) ;
#4297=CARTESIAN_POINT ( 'NONE',  ( 16.50821402049999875, 1494.476688022989947, 193.0250027032990090 ) ) ;
#4298=CARTESIAN_POINT ( 'NONE',  ( -15.41756489359970139, 1415.677402202029953, 209.3686558232799939 ) ) ;
#4301=CARTESIAN_POINT ( 'NONE',  ( -18.83362749532000180, 1444.184359083290019, 209.4102611290639970 ) ) ;
#4318=CARTESIAN_POINT ( 'NONE',  ( -1.130521170243829809, 1515.098624608320051, 213.4504088227829754 ) ) ;
#4320=CARTESIAN_POINT ( 'NONE',  ( -10.91165881471389909, 1480.298603070810032, 213.5307502733419938 ) ) ;
#4323=EDGE_CURVE ( 'NONE', #104484, #82244, #102171, .T. ) ;
#4326=EDGE_LOOP ( 'NONE', ( #107604, #1626, #83708, #46078 ) ) ;
#4329=CARTESIAN_POINT ( 'NONE',  ( 9.763688521220180050, 1493.202298044959889, 188.2888330414619986 ) ) ;
#4331=CARTESIAN_POINT ( 'NONE',  ( 8.765535317279999461, 1421.152484001810080, 196.5454161687989938 ) ) ;
#4337=CARTESIAN_POINT ( 'NONE',  ( -6.617556317490000062, 1459.313145877689976, 217.6703565655190005 ) ) ;
#4346=EDGE_CURVE ( 'NONE', #91400, #14236, #53213, .T. ) ;
#4347=CARTESIAN_POINT ( 'NONE',  ( -8.759590148488889838, 1447.855092709829933, 212.1632990431340033 ) ) ;
#4348=CARTESIAN_POINT ( 'NONE',  ( -17.59976141832330043, 1419.797097700060021, 206.6695233765389901 ) ) ;
#4356=CARTESIAN_POINT ( 'NONE',  ( 1.110223024629999949E-15, 1377.913060387289988, 209.1218459616989946 ) ) ;
#4361=CARTESIAN_POINT ( 'NONE',  ( 9.634266010251048229, 1434.809772052239850, 207.3359404128959795 ) ) ;
#4365=ORIENTED_EDGE ( 'NONE', *, *, #2554, .F. ) ;
#4367=CARTESIAN_POINT ( 'NONE',  ( 11.39903530061180170, 1471.112746094619979, 209.6182361319149834 ) ) ;
#4369=CARTESIAN_POINT ( 'NONE',  ( -19.75056259240000145, 1465.177823603190063, 209.1218459616989946 ) ) ;
#4374=EDGE_CURVE ( 'NONE', #105852, #62493, #63928, .T. ) ;
#4394=EDGE_CURVE ( 'NONE', #92844, #75158, #90445, .T. ) ;
#4399=CARTESIAN_POINT ( 'NONE',  ( -3.739222493130000213, 1474.769836386989937, 198.3144648466990247 ) ) ;
#4400=FACE_OUTER_BOUND ( 'NONE', #92039, .T. ) ;
#4408=DIRECTION ( 'NONE',  ( -7.436362843295819681E-17, 1.000000000000000000, -1.457576885956999882E-16 ) ) ;
#4411=CARTESIAN_POINT ( 'NONE',  ( 8.452187789688819564, 1498.645326028860154, 200.1952072007560162 ) ) ;
#4415=CARTESIAN_POINT ( 'NONE',  ( 10.55222728675549959, 1481.276343967989988, 208.5110256208110115 ) ) ;
#4416=DIRECTION ( 'NONE',  ( 0.9990834534827314206, 0.04280481766341149436, 2.370275682555253978E-05 ) ) ;
#4417=CARTESIAN_POINT ( 'NONE',  ( -2.183147893290000585, 1442.593045501889947, 200.4930349953090172 ) ) ;
#4421=CARTESIAN_POINT ( 'NONE',  ( 0.000000000000000000, 1398.755125754900064, 209.1218459616989946 ) ) ;
#4426=CARTESIAN_POINT ( 'NONE',  ( -11.48593466557120024, 1501.387652528300123, 208.6966813591159848 ) ) ;
#4432=CARTESIAN_POINT ( 'NONE',  ( -3.544886644340000448, 1474.831256732490147, 198.2487847239990231 ) ) ;
#4435=CARTESIAN_POINT ( 'NONE',  ( -9.609618950303881135, 1464.248441293520273, 228.1966055971730043 ) ) ;
#4441=CARTESIAN_POINT ( 'NONE',  ( -5.670189958209999936, 1463.356297375389886, 200.9627545900790153 ) ) ;
#4451=EDGE_LOOP ( 'NONE', ( #99966, #90579, #89723, #10007 ) ) ;
#4454=CARTESIAN_POINT ( 'NONE',  ( -18.74447803847540328, 1442.135375080380072, 209.4108418761609869 ) ) ;
#4456=CARTESIAN_POINT ( 'NONE',  ( 12.89015451259809986, 1420.977333543979967, 203.3411088897940147 ) ) ;
#4458=CARTESIAN_POINT ( 'NONE',  ( -15.77822988280000160, 1420.228048065240046, 210.6636264438090222 ) ) ;
#4465=CARTESIAN_POINT ( 'NONE',  ( -9.901327976855469615, 1447.905481077269997, 209.8160867571170058 ) ) ;
#4471=CARTESIAN_POINT ( 'NONE',  ( 0.2116392608170009904, 1497.592233828489952, 197.6910041071990065 ) ) ;
#4480=CARTESIAN_POINT ( 'NONE',  ( -0.8226521178380009625, 1486.661073111190035, 220.2963016106990040 ) ) ;
#4494=CARTESIAN_POINT ( 'NONE',  ( 7.359652137679999484, 1491.427741686289892, 211.7193136839289878 ) ) ;
#4496=CARTESIAN_POINT ( 'NONE',  ( 2.895368129540000002, 1444.422959043590026, 200.6322053094490059 ) ) ;
#4497=VERTEX_POINT ( 'NONE', #81486 ) ;
#4503=CARTESIAN_POINT ( 'NONE',  ( 8.235190278047509693, 1482.696351514019852, 217.6054839274150083 ) ) ;
#4514=CARTESIAN_POINT ( 'NONE',  ( 10.39122783130000016, 1420.703789618900146, 197.9464487691990087 ) ) ;
#4516=CARTESIAN_POINT ( 'NONE',  ( -6.418176471656730442, 1494.502784414770076, 198.6080641912510032 ) ) ;
#4527=EDGE_CURVE ( 'NONE', #73491, #86829, #88950, .T. ) ;
#4530=CARTESIAN_POINT ( 'NONE',  ( -15.69169271700000046, 1415.996555271789930, 210.3616365314589984 ) ) ;
#4531=FACE_OUTER_BOUND ( 'NONE', #69074, .T. ) ;
#4533=CARTESIAN_POINT ( 'NONE',  ( 3.880613242430000387, 1429.881321868690065, 216.9307363606289982 ) ) ;
#4536=CARTESIAN_POINT ( 'NONE',  ( -2.282423313820620248, 1429.314140543729991, 200.0277053824169968 ) ) ;
#4539=CARTESIAN_POINT ( 'NONE',  ( 3.587171487853899610, 1458.048446730460000, 200.0260115809859940 ) ) ;
#4551=CARTESIAN_POINT ( 'NONE',  ( -14.21117982910179833, 1416.454926512799830, 203.1643232870270026 ) ) ;
#4557=CARTESIAN_POINT ( 'NONE',  ( -4.325231581420000637, 1515.225841049890050, 208.0340196748790049 ) ) ;
#4561=CARTESIAN_POINT ( 'NONE',  ( 8.565457501751716052, 1437.263446294652567, 210.3368058788049666 ) ) ;
#4563=CARTESIAN_POINT ( 'NONE',  ( 3.132736840369999776, 1477.411600225689881, 199.0056338034989949 ) ) ;
#4565=CARTESIAN_POINT ( 'NONE',  ( -12.23036328449999921, 1490.675422890390109, 208.1371813544890017 ) ) ;
#4566=CARTESIAN_POINT ( 'NONE',  ( -9.784003721936180398, 1438.410133247240083, 210.7787260446129949 ) ) ;
#4582=CARTESIAN_POINT ( 'NONE',  ( -11.24237508680000097, 1500.135314328090089, 210.9525305401789979 ) ) ;
#4583=B_SPLINE_CURVE_WITH_KNOTS ( 'NONE', 3,
 ( #10826, #104323, #103775, #45553, #36568, #86415, #95377, #95924, #104877, #1323 ),
 .UNSPECIFIED., .F., .F.,
 ( 4, 2, 2, 2, 4 ),
 ( 0.000000000000000000, 0.5154127766764070584, 1.031119021958050164, 1.547502715879019997, 2.064659070031829913 ),
 .UNSPECIFIED. ) ;
#4587=B_SPLINE_SURFACE_WITH_KNOTS ( 'NONE', 5, 1, ( 
 ( #31429, #39285 ),
 ( #65611, #55561 ),
 ( #22451, #73460 ),
 ( #74559, #56652 ),
 ( #31984, #4593 ),
 ( #30876, #99723 ) ),
 .UNSPECIFIED., .F., .F., .F.,
 ( 6, 6 ),
 ( 2, 2 ),
 ( 0.000000000000000000, 3.708546873389999998 ),
 ( 0.000000000000000000, 14.00000000000000000 ),
 .UNSPECIFIED. ) ;
#4588=CARTESIAN_POINT ( 'NONE',  ( 2.487935123020000194, 1509.038615934189920, 213.6090957346689834 ) ) ;
#4589=CARTESIAN_POINT ( 'NONE',  ( -20.38158083214809935, 1465.353255672800060, 211.0002992862519875 ) ) ;
#4593=CARTESIAN_POINT ( 'NONE',  ( 20.21058018289999936, 1475.708866082789882, 208.1563043901110177 ) ) ;
#4601=CARTESIAN_POINT ( 'NONE',  ( 11.66537932461100091, 1501.769425689289847, 211.4581373967929778 ) ) ;
#4602=CARTESIAN_POINT ( 'NONE',  ( -10.66799487405013558, 1422.348300139214871, 210.6394755018355909 ) ) ;
#4604=ORIENTED_EDGE ( 'NONE', *, *, #53075, .F. ) ;
#4607=ORIENTED_EDGE ( 'NONE', *, *, #90717, .T. ) ;
#4608=CARTESIAN_POINT ( 'NONE',  ( 2.061035136763549769, 1485.227510182900005, 220.8012168559289989 ) ) ;
#4617=CARTESIAN_POINT ( 'NONE',  ( -16.53125420670000167, 1418.541487540729804, 202.7561987471289910 ) ) ;
#4623=CARTESIAN_POINT ( 'NONE',  ( 11.69993711075939835, 1435.514582224059950, 225.6365368809329937 ) ) ;
#4629=CARTESIAN_POINT ( 'NONE',  ( -16.87622493273829960, 1508.451388730329882, 209.8247102120089949 ) ) ;
#4630=CARTESIAN_POINT ( 'NONE',  ( -18.98492718470860297, 1508.490463703670002, 210.0727590967670153 ) ) ;
#4632=CARTESIAN_POINT ( 'NONE',  ( 1.910178218220000002, 1465.721278390790076, 198.6655444000990087 ) ) ;
#4645=CARTESIAN_POINT ( 'NONE',  ( -17.97472709737555263, 1508.456906073600294, 211.9276151093460783 ) ) ;
#4661=CARTESIAN_POINT ( 'NONE',  ( 4.082779675200349345, 1515.071395204220153, 212.7082060777060235 ) ) ;
#4669=CARTESIAN_POINT ( 'NONE',  ( -14.70081393560000116, 1415.677402184240009, 205.6533923404689688 ) ) ;
#4670=CARTESIAN_POINT ( 'NONE',  ( 9.549927530160001510, 1420.582634806009992, 197.0246874367990131 ) ) ;
#4672=B_SPLINE_CURVE_WITH_KNOTS ( 'NONE', 5,
 ( #70814, #96528, #29312, #54008, #55095, #71368, #38258, #11427, #88139, #72442, #37172, #105481 ),
 .UNSPECIFIED., .F., .F.,
 ( 6, 3, 3, 6 ),
 ( 0.000000000000000000, 0.2399281645681053676, 0.6199640824044998499, 1.000000000000000000 ),
 .UNSPECIFIED. ) ;
#4679=CARTESIAN_POINT ( 'NONE',  ( -1.477486471839999815, 1515.342042115489903, 213.3960819243490050 ) ) ;
#4682=CARTESIAN_POINT ( 'NONE',  ( 3.106494988410000158, 1471.641399328589841, 189.2364613132990030 ) ) ;
#4683=CARTESIAN_POINT ( 'NONE',  ( 5.059013353549999259, 1501.257177412389865, 229.8390314845989906 ) ) ;
#4684=CARTESIAN_POINT ( 'NONE',  ( -7.748343491022634311, 1439.118950628315588, 205.0759599076347399 ) ) ;
#4698=CARTESIAN_POINT ( 'NONE',  ( 12.27851265883290033, 1491.806146454400050, 208.1629158539130060 ) ) ;
#4707=FACE_OUTER_BOUND ( 'NONE', #68624, .T. ) ;
#4711=CARTESIAN_POINT ( 'NONE',  ( -7.405436629479999588, 1451.940595730289942, 201.5764829818989767 ) ) ;
#4713=CARTESIAN_POINT ( 'NONE',  ( 8.454790768000000512, 1428.363638924389988, 213.4109941084990112 ) ) ;
#4714=CARTESIAN_POINT ( 'NONE',  ( 20.33643750519999926, 1475.138452888789971, 218.0161091832190152 ) ) ;
#4720=ORIENTED_EDGE ( 'NONE', *, *, #106335, .T. ) ;
#4731=CARTESIAN_POINT ( 'NONE',  ( -1.879441947317239903, 1463.200433190200101, 199.5207160416179875 ) ) ;
#4732=CARTESIAN_POINT ( 'NONE',  ( 12.45715143159750049, 1427.088322622419810, 206.6492473361469990 ) ) ;
#4742=CARTESIAN_POINT ( 'NONE',  ( -17.03470032699999948, 1420.297131032510151, 203.9213209310090065 ) ) ;
#4750=CARTESIAN_POINT ( 'NONE',  ( -18.45894773530089950, 1508.542100887300194, 210.6804767572419905 ) ) ;
#4778=B_SPLINE_CURVE_WITH_KNOTS ( 'NONE', 3,
 ( #95144, #52049, #36331, #61561, #68864, #17847, #18405, #95695, #26266, #94573, #78912, #9477, #86739, #59906, #87297, #43641, #16737, #52603, #18962, #99495, #26833, #552, #104088, #60456, #102968, #104643, #77793, #1102, #51486, #85069, #50944, #35231, #69419, #94027, #10591 ),
 .UNSPECIFIED., .F., .F.,
 ( 4, 2, 2, 1, 1, 2, 2, 2, 1, 2, 2, 1, 1, 1, 2, 2, 2, 1, 2, 2, 4 ),
 ( 0.000000000000000000, 0.1250000000000932032, 0.1875000000001283418, 0.2187500000001456890, 0.2343750000001545153, 0.2421875000001469658, 0.2500000000001393885, 0.3125000000000572320, 0.3437500000000050515, 0.3593749999999903411, 0.3749999999999756306, 0.4062499999999467093, 0.4218749999999321654, 0.4296874999999362177, 0.4335937499999382161, 0.4374999999999402145, 0.4687499999999615308, 0.4843749999999613642, 0.4921874999999606426, 0.4999999999999599209, 1.000000000000000000 ),
 .UNSPECIFIED. ) ;
#4783=CARTESIAN_POINT ( 'NONE',  ( 11.64657740540000042, 1421.681747358590201, 203.4365565939590113 ) ) ;
#4787=CARTESIAN_POINT ( 'NONE',  ( 1.779428963082609894, 1456.357349037730046, 198.6855221610310309 ) ) ;
#4788=CARTESIAN_POINT ( 'NONE',  ( 10.03573453041540020, 1469.254327712470058, 209.6255595403590064 ) ) ;
#4789=VERTEX_POINT ( 'NONE', #26554 ) ;
#4791=CARTESIAN_POINT ( 'NONE',  ( 10.19252854585250212, 1480.675633674519986, 206.4352025249530129 ) ) ;
#4792=ORIENTED_EDGE ( 'NONE', *, *, #110593, .F. ) ;
#4798=CARTESIAN_POINT ( 'NONE',  ( 2.380213422489999786, 1443.039342964089883, 217.6985620011490141 ) ) ;
#4807=CARTESIAN_POINT ( 'NONE',  ( -10.02128875133539943, 1472.300851888030138, 210.8937131631379884 ) ) ;
#4810=CARTESIAN_POINT ( 'NONE',  ( -14.48383822919999986, 1508.489289363889839, 215.9967763605189930 ) ) ;
#4815=FACE_OUTER_BOUND ( 'NONE', #54864, .T. ) ;
#4820=CARTESIAN_POINT ( 'NONE',  ( 6.225981071277309375, 1494.795956435949847, 219.7811113419710125 ) ) ;
#4822=CARTESIAN_POINT ( 'NONE',  ( -15.05902623708989907, 1415.677402202029953, 207.6815266051810056 ) ) ;
#4823=CARTESIAN_POINT ( 'NONE',  ( -9.544116702023510257, 1460.067049166229936, 210.4863253896969866 ) ) ;
#4825=CARTESIAN_POINT ( 'NONE',  ( 6.870558963890000648, 1491.940207589490001, 213.3945113296690010 ) ) ;
#4842=DIRECTION ( 'NONE',  ( 0.000000000000000000, 1.000000000000000000, -1.836970198721029688E-16 ) ) ;
#4846=CARTESIAN_POINT ( 'NONE',  ( -11.12097504240020029, 1480.502194893749902, 213.0088585123340010 ) ) ;
#4850=ORIENTED_EDGE ( 'NONE', *, *, #13319, .T. ) ;
#4854=ADVANCED_FACE ( 'NONE', ( #25430 ), #17830, .T. ) ;
#4855=CARTESIAN_POINT ( 'NONE',  ( -18.76196770059999963, 1505.911165295990031, 222.6390480598990109 ) ) ;
#4861=EDGE_CURVE ( 'NONE', #45216, #1907, #3850, .T. ) ;
#4865=CARTESIAN_POINT ( 'NONE',  ( -4.803286822639999620, 1458.496532453990085, 218.2603857696190062 ) ) ;
#4872=ORIENTED_EDGE ( 'NONE', *, *, #81477, .T. ) ;
#4874=CARTESIAN_POINT ( 'NONE',  ( -8.594767888845639803, 1448.338307337700144, 212.2585178878949819 ) ) ;
#4885=ADVANCED_FACE ( 'NONE', ( #56738 ), #76863, .T. ) ;
#4895=CARTESIAN_POINT ( 'NONE',  ( -1.978433376304360003, 1467.924323865460110, 220.0703243356560108 ) ) ;
#4896=CARTESIAN_POINT ( 'NONE',  ( 19.40350356789999964, 1457.232592156389956, 208.1907244810240059 ) ) ;
#4936=CARTESIAN_POINT ( 'NONE',  ( -11.33279196814429923, 1470.495430824379810, 210.3432187421609854 ) ) ;
#4937=CARTESIAN_POINT ( 'NONE',  ( 11.36889272073800150, 1499.667877637589982, 204.5284518008890302 ) ) ;
#4938=ORIENTED_EDGE ( 'NONE', *, *, #54341, .T. ) ;
#4940=CARTESIAN_POINT ( 'NONE',  ( -2.487935123034410445, 1508.909942010395071, 213.6124651809371642 ) ) ;
#4941=CIRCLE ( 'NONE', #44375, 10.71315034250000053 ) ;
#4945=CARTESIAN_POINT ( 'NONE',  ( 11.47870337641239935, 1502.276891194350128, 211.2824957803889845 ) ) ;
#4953=CARTESIAN_POINT ( 'NONE',  ( -11.46596297259700137, 1501.319154807139739, 208.6783501317359821 ) ) ;
#4960=CARTESIAN_POINT ( 'NONE',  ( 3.704457720059250114, 1508.551704408389924, 204.4495214305590025 ) ) ;
#4963=CARTESIAN_POINT ( 'NONE',  ( 20.81805316561590047, 1457.016391092229924, 206.8941893600089941 ) ) ;
#4966=CARTESIAN_POINT ( 'NONE',  ( -4.329415264797339624, 1515.068899375750107, 206.1637497075489875 ) ) ;
#4975=CARTESIAN_POINT ( 'NONE',  ( 0.000000000000000000, 1402.913060387289988, 209.1218459616989946 ) ) ;
#4979=ORIENTED_EDGE ( 'NONE', *, *, #69903, .F. ) ;
#4987=CARTESIAN_POINT ( 'NONE',  ( -15.33731769819999968, 1420.146962874850033, 211.9565886041989984 ) ) ;
#4994=ADVANCED_FACE ( 'NONE', ( #101454 ), #25875, .T. ) ;
#4996=AXIS2_PLACEMENT_3D ( 'NONE', #84298, #24379, #23278 ) ;
#4997=CARTESIAN_POINT ( 'NONE',  ( -9.178648612314900035, 1447.470203629239904, 211.6527240042640017 ) ) ;
#5006=CARTESIAN_POINT ( 'NONE',  ( -2.795964621609999590, 1422.864594294989956, 191.4386244948990168 ) ) ;
#5017=FACE_OUTER_BOUND ( 'NONE', #44553, .T. ) ;
#5021=CARTESIAN_POINT ( 'NONE',  ( 9.331306786325548330, 1452.122598230650055, 210.5717110549620088 ) ) ;
#5022=CARTESIAN_POINT ( 'NONE',  ( 5.450648847440000111, 1423.857684999099774, 194.2417023985990170 ) ) ;
#5025=CARTESIAN_POINT ( 'NONE',  ( 7.675506710379999653, 1490.901593261789913, 210.2162091181089920 ) ) ;
#5030=CARTESIAN_POINT ( 'NONE',  ( 0.2645430705366629831, 1443.121743617909942, 200.2023352529839997 ) ) ;
#5037=VERTEX_POINT ( 'NONE', #42683 ) ;
#5038=CARTESIAN_POINT ( 'NONE',  ( 7.375496855036300481, 1483.107846205720080, 218.3651359022439919 ) ) ;
#5042=CARTESIAN_POINT ( 'NONE',  ( -11.41699241967629952, 1481.865938852530235, 208.5945336717069836 ) ) ;
#5047=CARTESIAN_POINT ( 'NONE',  ( 12.23993107200000097, 1420.119835428209853, 199.7451907216789948 ) ) ;
#5048=CARTESIAN_POINT ( 'NONE',  ( 0.3127569488372759499, 1475.234939895219895, 220.5412273341300136 ) ) ;
#5054=CARTESIAN_POINT ( 'NONE',  ( 10.79561051538090055, 1423.418703670030027, 206.7986195382829919 ) ) ;
#5058=ORIENTED_EDGE ( 'NONE', *, *, #73390, .F. ) ;
#5059=CARTESIAN_POINT ( 'NONE',  ( 5.998951827550000004, 1470.912646799889899, 213.0429767062390169 ) ) ;
#5060=CARTESIAN_POINT ( 'NONE',  ( -16.76711878018801372, 1417.195629503265309, 207.2570596610230780 ) ) ;
#5063=CARTESIAN_POINT ( 'NONE',  ( 8.799694164910118133, 1425.068530136420122, 210.2036770632330160 ) ) ;
#5064=CARTESIAN_POINT ( 'NONE',  ( -16.50454912150300046, 1419.915473451730122, 209.2650646900050049 ) ) ;
#5065=ORIENTED_EDGE ( 'NONE', *, *, #74029, .T. ) ;
#5066=CARTESIAN_POINT ( 'NONE',  ( 3.663504462200000145, 1429.509591348389904, 216.7335040807589905 ) ) ;
#5068=CARTESIAN_POINT ( 'NONE',  ( -16.52561552909999776, 1416.917924532109964, 208.4225654288269993 ) ) ;
#5072=CARTESIAN_POINT ( 'NONE',  ( 2.357442550764540012, 1458.086361592170306, 199.7974089473029835 ) ) ;
#5073=FACE_OUTER_BOUND ( 'NONE', #35074, .T. ) ;
#5081=CARTESIAN_POINT ( 'NONE',  ( 1.955657237439999863, 1459.028687623489986, 202.4574169284290122 ) ) ;
#5083=CARTESIAN_POINT ( 'NONE',  ( 0.008119676858140530140, 1515.178500008189985, 204.7953747115290071 ) ) ;
#5084=CARTESIAN_POINT ( 'NONE',  ( 12.52897032537950217, 1427.032053915000006, 206.3112042049379795 ) ) ;
#5089=CARTESIAN_POINT ( 'NONE',  ( 8.727114281347018832, 1428.313213898079994, 213.1854654111380114 ) ) ;
#5092=CARTESIAN_POINT ( 'NONE',  ( 3.629220049600000220, 1485.493215689190038, 199.0019176958990101 ) ) ;
#5098=CARTESIAN_POINT ( 'NONE',  ( 9.293015197429999930, 1478.078892413390122, 202.6398356817990134 ) ) ;
#5100=CARTESIAN_POINT ( 'NONE',  ( -11.04294906800000042, 1491.966910088589884, 207.3598305497890237 ) ) ;
#5109=CARTESIAN_POINT ( 'NONE',  ( -4.301731299663230423, 1508.551704408389924, 204.9156561448070022 ) ) ;
#5117=CARTESIAN_POINT ( 'NONE',  ( 10.82166596142770132, 1471.344689967329941, 210.9651955021979859 ) ) ;
#5120=DIRECTION ( 'NONE',  ( -0.8907681516580484571, 1.273087901431153894E-31, 0.4544580288560254311 ) ) ;
#5121=CARTESIAN_POINT ( 'NONE',  ( -1.088650671229999922, 1420.780442655370052, 193.7338955114989858 ) ) ;
#5122=EDGE_CURVE ( 'NONE', #37608, #21803, #92536, .T. ) ;
#5125=CARTESIAN_POINT ( 'NONE',  ( -13.38188607319999868, 1469.919367367889890, 192.0112524093990203 ) ) ;
#5139=CARTESIAN_POINT ( 'NONE',  ( -9081.484824850398581, 5182.767774292099602, -1567.708540563249926 ) ) ;
#5147=CARTESIAN_POINT ( 'NONE',  ( -1.270117472468459852, 1486.209137599609903, 220.9629115624290137 ) ) ;
#5155=CARTESIAN_POINT ( 'NONE',  ( 7.231901239322829689, 1483.532524091059940, 217.6548318471419918 ) ) ;
#5160=CARTESIAN_POINT ( 'NONE',  ( 4.677562605459999467, 1434.889072344290071, 228.7640133631989841 ) ) ;
#5173=CARTESIAN_POINT ( 'NONE',  ( -1.347198969329999940, 1464.928942339390005, 198.6034036249990038 ) ) ;
#5178=ORIENTED_EDGE ( 'NONE', *, *, #63092, .T. ) ;
#5189=CARTESIAN_POINT ( 'NONE',  ( -10.11189522083689951, 1462.195248612440082, 207.9445251505729857 ) ) ;
#5190=CARTESIAN_POINT ( 'NONE',  ( -5.450781814275990733, 1434.502290401799883, 217.0838862464160002 ) ) ;
#5198=B_SPLINE_CURVE_WITH_KNOTS ( 'NONE', 3,
 ( #220, #42750, #69637, #18622, #51154, #763, #1878, #9149, #27061, #78562, #50602, #60119, #61247, #95361, #102621, #18080, #43313, #103181, #77461, #85850, #94805, #26483, #60679, #52275, #34892 ),
 .UNSPECIFIED., .F., .F.,
 ( 4, 3, 3, 3, 3, 3, 3, 3, 4 ),
 ( -7.454989583650000640, -7.295847338557649664, -6.603480943530409597, -5.920148531335569508, -5.256832802792740011, -4.983278890925820548, -4.387781186674780010, -3.607420121254749645, -3.058675454859999476 ),
 .UNSPECIFIED. ) ;
#5211=CARTESIAN_POINT ( 'NONE',  ( -7.649966233313090669, 1508.551704408389924, 219.0282755267929815 ) ) ;
#5212=CARTESIAN_POINT ( 'NONE',  ( 3.115880663340000023, 1508.551704408389924, 219.3718645306990140 ) ) ;
#5217=CARTESIAN_POINT ( 'NONE',  ( 7.345629923129999739, 1422.263538441430001, 195.5717800564989943 ) ) ;
#5219=CARTESIAN_POINT ( 'NONE',  ( -5.489226993980830471, 1448.625211997490169, 211.5470588731079715 ) ) ;
#5221=FACE_OUTER_BOUND ( 'NONE', #39014, .T. ) ;
#5222=CARTESIAN_POINT ( 'NONE',  ( 19.41979707700000191, 1457.606582239089903, 210.0704631242259950 ) ) ;
#5230=CARTESIAN_POINT ( 'NONE',  ( -1.551161424019060098, 1463.265709907049995, 199.4650991780359846 ) ) ;
#5232=CARTESIAN_POINT ( 'NONE',  ( -2.298816264069999615, 1486.462377070590037, 220.8289805453990198 ) ) ;
#5237=CARTESIAN_POINT ( 'NONE',  ( -3.906019471690000078, 1515.551703594190030, 210.6105386114290070 ) ) ;
#5249=B_SPLINE_SURFACE_WITH_KNOTS ( 'NONE', 5, 5, ( 
 ( #89479, #64859, #64302, #14404, #12774, #98967 ),
 ( #79980, #71628, #29565, #46951, #46405, #21694 ),
 ( #63749, #37980, #97863, #72693, #98422, #8208 ),
 ( #14952, #25555, #32334, #108485, #42374, #76529 ),
 ( #24454, #59747, #32862, #67601, #102275, #74357 ),
 ( #25002, #16586, #23902, #41826, #67054, #16051 ),
 ( #75457, #33972, #50254, #84383, #7670, #7127 ),
 ( #75982, #40176, #31768, #50783, #110133, #92228 ),
 ( #101160, #58642, #93323, #59205, #110681, #68168 ) ),
 .UNSPECIFIED., .F., .F., .F.,
 ( 6, 3, 6 ),
 ( 6, 6 ),
 ( 0.000000000000000000, 3.172668598669999618, 4.759002897999999426 ),
 ( 0.000000000000000000, 14.00000000000000000 ),
 .UNSPECIFIED. ) ;
#5255=CARTESIAN_POINT ( 'NONE',  ( 12.74090128278689882, 1421.413457440939965, 206.2481278393109960 ) ) ;
#5256=VECTOR ( 'NONE', #59809, 1000.000000000000000 ) ;
#5262=CARTESIAN_POINT ( 'NONE',  ( 10.75631864651809977, 1451.138109684059827, 190.3409053450899933 ) ) ;
#5267=CARTESIAN_POINT ( 'NONE',  ( 7.984273842250000364, 1426.916635774389988, 211.9701635203690273 ) ) ;
#5268=CARTESIAN_POINT ( 'NONE',  ( -21.44637799630000075, 1506.412602296789828, 216.0243671510289971 ) ) ;
#5270=CARTESIAN_POINT ( 'NONE',  ( -18.88624094756929850, 1419.246025400399958, 205.9308376352330185 ) ) ;
#5283=CARTESIAN_POINT ( 'NONE',  ( 2.329920886069499986, 1515.492270357839971, 204.9835198734710104 ) ) ;
#5299=CARTESIAN_POINT ( 'NONE',  ( 11.13894495610000135, 1491.363598464389952, 209.7173500882680059 ) ) ;
#5305=ORIENTED_EDGE ( 'NONE', *, *, #93194, .F. ) ;
#5306=CARTESIAN_POINT ( 'NONE',  ( -11.97066799919999980, 1502.729030670490147, 208.4344832896910020 ) ) ;
#5309=EDGE_CURVE ( 'NONE', #38904, #24522, #90458, .T. ) ;
#5312=ORIENTED_EDGE ( 'NONE', *, *, #10943, .T. ) ;
#5332=CARTESIAN_POINT ( 'NONE',  ( -3.271537981817990381, 1454.292002020450127, 199.1638778446669846 ) ) ;
#5344=CARTESIAN_POINT ( 'NONE',  ( 12.89505355770000072, 1420.989633701210096, 203.4267449422790150 ) ) ;
#5348=CARTESIAN_POINT ( 'NONE',  ( -4.772433264290000032, 1461.586210710390105, 228.1254610687989839 ) ) ;
#5352=CARTESIAN_POINT ( 'NONE',  ( 10.51581569650209858, 1481.161035245299900, 208.1366864954699736 ) ) ;
#5354=VECTOR ( 'NONE', #11730, 1000.000000000000114 ) ;
#5357=CARTESIAN_POINT ( 'NONE',  ( 10.93222784191639896, 1461.420118457989929, 209.9621245680470167 ) ) ;
#5359=CARTESIAN_POINT ( 'NONE',  ( 2.395822483399999925, 1441.661856669790041, 218.7568551047190226 ) ) ;
#5371=CARTESIAN_POINT ( 'NONE',  ( -15.53181541920000086, 1508.521255623489878, 214.8366523089289899 ) ) ;
#5379=B_SPLINE_SURFACE_WITH_KNOTS ( 'NONE', 5, 5, ( 
 ( #2759, #36879, #88393, #10586, #28488, #71074 ),
 ( #78338, #27376, #44757, #61558, #35785, #2213 ),
 ( #79991, #62680, #80548, #37441, #105758, #71638 ),
 ( #104082, #29043, #78905, #46416, #3863, #37991 ),
 ( #100092, #108495, #6033, #39641, #82741, #91687 ),
 ( #64868, #81622, #65413, #74367, #29574, #107939 ) ),
 .UNSPECIFIED., .F., .F., .F.,
 ( 6, 6 ),
 ( 6, 6 ),
 ( 22.07912247049999976, 26.44584043820000119 ),
 ( 0.000000000000000000, 0.5000000000000000000 ),
 .UNSPECIFIED. ) ;
#5381=CARTESIAN_POINT ( 'NONE',  ( 3.582189414718509823, 1494.866532486610140, 220.1463443050500075 ) ) ;
#5382=B_SPLINE_CURVE_WITH_KNOTS ( 'NONE', 3,
 ( #109925, #57883, #33204, #67394, #56217, #23698, #90347, #49479, #13627, #56772, #31551, #5255, #73587, #107718, #90910, #14193, #74133, #108265, #65728, #23141, #57346, #91470, #14750, #6358, #40507 ),
 .UNSPECIFIED., .F., .F.,
 ( 4, 3, 3, 3, 3, 3, 3, 3, 4 ),
 ( -25.30278126027359775, -25.08579948689999739, -24.77235297171529993, -24.14468077163109783, -23.20356205636220182, -22.54016880708680048, -21.81726924789879973, -20.86314243152489922, -19.77745610209999683 ),
 .UNSPECIFIED. ) ;
#5385=CARTESIAN_POINT ( 'NONE',  ( -9.599657450428111360, 1460.198427500139815, 210.0868860100479765 ) ) ;
#5395=CARTESIAN_POINT ( 'NONE',  ( 3.694265505850000242, 1454.607279123389844, 217.7787218116090173 ) ) ;
#5397=CARTESIAN_POINT ( 'NONE',  ( 8.958374100104808946, 1436.656241311369968, 210.3666130420500053 ) ) ;
#5399=CARTESIAN_POINT ( 'NONE',  ( 7.868158389100000427, 1422.937290482379922, 214.1570520181289794 ) ) ;
#5400=FACE_OUTER_BOUND ( 'NONE', #11486, .T. ) ;
#5402=CARTESIAN_POINT ( 'NONE',  ( -1.345088944733920044, 1515.083299843980058, 213.4508101154519863 ) ) ;
#5408=ORIENTED_EDGE ( 'NONE', *, *, #45670, .T. ) ;
#5409=VERTEX_POINT ( 'NONE', #41998 ) ;
#5412=CARTESIAN_POINT ( 'NONE',  ( 13.71656619866890026, 1499.109475169520010, 227.7998406596679786 ) ) ;
#5414=CARTESIAN_POINT ( 'NONE',  ( -0.9686567332709090650, 1473.830917872273858, 219.3200354843431228 ) ) ;
#5418=AXIS2_PLACEMENT_3D ( 'NONE', #37414, #12197, #105733 ) ;
#5422=CARTESIAN_POINT ( 'NONE',  ( 17.94074846905810006, 1431.033909182950083, 205.7008688429760070 ) ) ;
#5423=CARTESIAN_POINT ( 'NONE',  ( -6.210220977990000613, 1458.870741700389772, 216.9690521252790063 ) ) ;
#5432=CARTESIAN_POINT ( 'NONE',  ( -8.794092324118190973, 1447.789040521789957, 212.1549648291330072 ) ) ;
#5435=( LENGTH_UNIT ( ) NAMED_UNIT ( * ) SI_UNIT ( .MILLI., .METRE. ) );
#5447=ORIENTED_EDGE ( 'NONE', *, *, #74822, .T. ) ;
#5459=DIRECTION ( 'NONE',  ( -1.000000000000000000, 0.000000000000000000, 0.000000000000000000 ) ) ;
#5463=CARTESIAN_POINT ( 'NONE',  ( -7.544775971906443779, 1425.914422796234476, 205.6924955586506485 ) ) ;
#5464=CARTESIAN_POINT ( 'NONE',  ( -10.07154961049999820, 1473.228064888090103, 207.4129456781890326 ) ) ;
#5466=ORIENTED_EDGE ( 'NONE', *, *, #9215, .T. ) ;
#5475=CARTESIAN_POINT ( 'NONE',  ( 4.163336342339999869E-15, 1416.181292664740113, 209.1218459616989946 ) ) ;
#5484=EDGE_CURVE ( 'NONE', #26374, #63089, #67216, .T. ) ;
#5487=CARTESIAN_POINT ( 'NONE',  ( 1.029697549479999807, 1474.120255407390005, 219.4685556096990240 ) ) ;
#5509=CARTESIAN_POINT ( 'NONE',  ( -10.46250751532009993, 1491.356802638789986, 212.5409670664860187 ) ) ;
#5510=CARTESIAN_POINT ( 'NONE',  ( -1.452443133548009913, 1508.551704408389924, 220.0823312915929932 ) ) ;
#5512=CARTESIAN_POINT ( 'NONE',  ( -4.487249019397720140, 1509.038644351750008, 206.6339222935139901 ) ) ;
#5515=CARTESIAN_POINT ( 'NONE',  ( -11.72999038033949937, 1501.913969227260168, 208.8343572913619823 ) ) ;
#5521=CARTESIAN_POINT ( 'NONE',  ( -3.790930610359999786, 1476.560235432990112, 199.4766108674189979 ) ) ;
#5522=CARTESIAN_POINT ( 'NONE',  ( -10.22078085839999950, 1448.827725591389935, 207.2905425509590032 ) ) ;
#5524=CARTESIAN_POINT ( 'NONE',  ( -9.771943666833310616, 1448.872252160599828, 190.8346857363359845 ) ) ;
#5530=CARTESIAN_POINT ( 'NONE',  ( -9.941476446395858702, 1461.322233705820054, 211.0754656163810239 ) ) ;
#5533=CARTESIAN_POINT ( 'NONE',  ( -15.12493481535974738, 1420.059538282757785, 212.5153262450139096 ) ) ;
#5544=EDGE_LOOP ( 'NONE', ( #6050, #1024, #106130, #95629 ) ) ;
#5549=VECTOR ( 'NONE', #36638, 1000.000000000000114 ) ;
#5561=CARTESIAN_POINT ( 'NONE',  ( -9.853487827760540441, 1447.709311025530042, 210.2834318627940036 ) ) ;
#5566=CARTESIAN_POINT ( 'NONE',  ( 7.346206468657319633, 1425.063440261549886, 212.5639244028189978 ) ) ;
#5575=CARTESIAN_POINT ( 'NONE',  ( -4.638300726919323935, 1378.093220027633151, 214.4059711397904096 ) ) ;
#5585=CARTESIAN_POINT ( 'NONE',  ( 10.08587585095050088, 1452.694239366880083, 210.2353006364240002 ) ) ;
#5593=CARTESIAN_POINT ( 'NONE',  ( 2.487922177595819573, 1508.551704408389924, 213.9544573010300326 ) ) ;
#5600=VERTEX_POINT ( 'NONE', #39660 ) ;
#5601=CARTESIAN_POINT ( 'NONE',  ( 11.06169707739279851, 1480.845630662619897, 213.2313991462129934 ) ) ;
#5605=CARTESIAN_POINT ( 'NONE',  ( -10.51230281979400161, 1480.112285530560030, 208.7110773518720066 ) ) ;
#5610=CARTESIAN_POINT ( 'NONE',  ( -1.212018553542939969, 1475.694787048319995, 220.4957529374679837 ) ) ;
#5612=CARTESIAN_POINT ( 'NONE',  ( 10.99716211064770022, 1478.798203161799847, 205.9204684199630151 ) ) ;
#5616=CARTESIAN_POINT ( 'NONE',  ( 11.24378212487630080, 1426.078668191249790, 206.4971785593209859 ) ) ;
#5627=CARTESIAN_POINT ( 'NONE',  ( 10.47394328510990036, 1422.444227279350116, 210.3705285485489753 ) ) ;
#5628=CARTESIAN_POINT ( 'NONE',  ( 10.94161034597069992, 1423.824721436569689, 203.2068899696880067 ) ) ;
#5629=ORIENTED_EDGE ( 'NONE', *, *, #50004, .T. ) ;
#5630=EDGE_CURVE ( 'NONE', #22363, #63746, #55100, .T. ) ;
#5631=CARTESIAN_POINT ( 'NONE',  ( 3.346088552949999961, 1429.638897950889941, 216.8836957388089672 ) ) ;
#5639=CARTESIAN_POINT ( 'NONE',  ( 6.701030630508360453, 1458.780274625029961, 201.5154958855920029 ) ) ;
#5653=CARTESIAN_POINT ( 'NONE',  ( -14.61445746615800090, 1417.481753922669895, 203.2535310402599862 ) ) ;
#5659=CARTESIAN_POINT ( 'NONE',  ( -0.3534367268244609783, 1484.221040251851036, 198.4322127960935802 ) ) ;
#5663=ORIENTED_EDGE ( 'NONE', *, *, #26368, .F. ) ;
#5673=CARTESIAN_POINT ( 'NONE',  ( 9.217027833218040200, 1427.824330594879939, 211.8044439908819925 ) ) ;
#5677=MECHANICAL_DESIGN_GEOMETRIC_PRESENTATION_REPRESENTATION('',(#53993),#19966);
#5679=CARTESIAN_POINT ( 'NONE',  ( -3.890622774867280143, 1508.551704408389924, 204.5662182099170252 ) ) ;
#5686=CARTESIAN_POINT ( 'NONE',  ( 10.93373778070590063, 1471.043189543029939, 209.8922278286480037 ) ) ;
#5693=CARTESIAN_POINT ( 'NONE',  ( -20.36852751908510228, 1464.956532905599943, 210.9458057460080056 ) ) ;
#5695=CARTESIAN_POINT ( 'NONE',  ( 10.52384291159865626, 1498.970202591990983, 202.0357653132980431 ) ) ;
#5707=VERTEX_POINT ( 'NONE', #6604 ) ;
#5713=CARTESIAN_POINT ( 'NONE',  ( 11.27432879130000032, 1501.460240645189742, 207.0864724315690069 ) ) ;
#5725=ORIENTED_EDGE ( 'NONE', *, *, #76427, .F. ) ;
#5726=CARTESIAN_POINT ( 'NONE',  ( -18.92738905869999755, 1503.346139545890082, 222.1981867166989844 ) ) ;
#5734=CARTESIAN_POINT ( 'NONE',  ( -21.12854636069999970, 1507.715431485890122, 209.4790061967080135 ) ) ;
#5739=CARTESIAN_POINT ( 'NONE',  ( -0.02154542468749880146, 1464.515732093790120, 199.1359198071390040 ) ) ;
#5752=CARTESIAN_POINT ( 'NONE',  ( 8.413641089779510196, 1428.393608785230072, 213.4913874550600212 ) ) ;
#5756=ADVANCED_FACE ( 'NONE', ( #110165 ), #110817, .T. ) ;
#5779=CARTESIAN_POINT ( 'NONE',  ( -15.85591190879999779, 1415.880081504350073, 209.4912631162540038 ) ) ;
#5784=CARTESIAN_POINT ( 'NONE',  ( -12.22894430393720100, 1440.615615687460149, 224.1155035949470005 ) ) ;
#5798=CARTESIAN_POINT ( 'NONE',  ( -6.997399759229028682, 1439.698082657984287, 203.8640865756502194 ) ) ;
#5803=CARTESIAN_POINT ( 'NONE',  ( -12.03392632030000087, 1501.178862756489934, 213.6370645969589930 ) ) ;
#5824=CARTESIAN_POINT ( 'NONE',  ( -13.58963604942879932, 1508.337642800850062, 209.7220322380239850 ) ) ;
#5825=CARTESIAN_POINT ( 'NONE',  ( -16.83568192233699889, 1418.884533542789995, 201.2565368160369985 ) ) ;
#5826=CARTESIAN_POINT ( 'NONE',  ( -16.42987258731520228, 1416.947447175220077, 208.7386071577110158 ) ) ;
#5828=DIRECTION ( 'NONE',  ( 0.000000000000000000, -1.000000000000000000, 1.836970198721029688E-16 ) ) ;
#5832=CARTESIAN_POINT ( 'NONE',  ( 7.788969440409999834, 1427.187801883110069, 212.3321831630789802 ) ) ;
#5833=B_SPLINE_CURVE_WITH_KNOTS ( 'NONE', 3,
 ( #104519, #78771, #4277, #2086, #105638, #28923, #96115, #96681, #18836, #29454, #45187, #53032, #89373, #46844, #80429, #70959 ),
 .UNSPECIFIED., .F., .F.,
 ( 4, 3, 3, 3, 3, 4 ),
 ( -19.57721055789999909, -18.83699752252369919, -17.50138789245909976, -16.16248386776419821, -14.82273906699520083, -13.48402717865840117 ),
 .UNSPECIFIED. ) ;
#5839=CARTESIAN_POINT ( 'NONE',  ( 9.296940999030001151, 1453.078838425589993, 212.1081469227889897 ) ) ;
#5840=ORIENTED_EDGE ( 'NONE', *, *, #18175, .T. ) ;
#5851=CARTESIAN_POINT ( 'NONE',  ( -3.676358388133539989, 1464.513658476559840, 199.1740838259549946 ) ) ;
#5852=CARTESIAN_POINT ( 'NONE',  ( 3.839962655360000365, 1424.367742364450123, 191.5388040513990120 ) ) ;
#5857=ORIENTED_EDGE ( 'NONE', *, *, #43955, .T. ) ;
#5861=VERTEX_POINT ( 'NONE', #25590 ) ;
#5862=CARTESIAN_POINT ( 'NONE',  ( -9.975542809210001138, 1421.165924026620132, 193.6282031886989898 ) ) ;
#5868=CARTESIAN_POINT ( 'NONE',  ( -12.03574695270000028, 1503.040364855890175, 208.3824768740459774 ) ) ;
#5872=ORIENTED_EDGE ( 'NONE', *, *, #100359, .T. ) ;
#5887=CARTESIAN_POINT ( 'NONE',  ( 4.637787270109999582, 1462.124489585889933, 228.1829287868989979 ) ) ;
#5898=EDGE_CURVE ( 'NONE', #25016, #9292, #4941, .T. ) ;
#5902=CARTESIAN_POINT ( 'NONE',  ( 12.25880158789999896, 1421.301048178839892, 203.8561358684090123 ) ) ;
#5903=CARTESIAN_POINT ( 'NONE',  ( 1.968601690575629615, 1498.935401749600032, 197.9561509338619771 ) ) ;
#5906=CARTESIAN_POINT ( 'NONE',  ( -3.665756888920000289, 1508.551704408389924, 204.1347675262390169 ) ) ;
#5913=ADVANCED_FACE ( 'NONE', ( #1960 ), #93816, .T. ) ;
#5916=CARTESIAN_POINT ( 'NONE',  ( 10.89432528737160055, 1461.587524139910101, 210.3982013538480089 ) ) ;
#5919=CARTESIAN_POINT ( 'NONE',  ( 4.514829284230000184, 1467.261183020589897, 217.9965697402589910 ) ) ;
#5936=CARTESIAN_POINT ( 'NONE',  ( -8.992268003901459750, 1437.995299232369916, 210.5002298188580028 ) ) ;
#5937=FACE_OUTER_BOUND ( 'NONE', #15127, .T. ) ;
#5939=CARTESIAN_POINT ( 'NONE',  ( -15.14662681555729939, 1415.677402202029953, 208.0848883706039771 ) ) ;
#5949=CARTESIAN_POINT ( 'NONE',  ( -12.24556316650000021, 1502.082825312490058, 210.5128827789189927 ) ) ;
#5951=CARTESIAN_POINT ( 'NONE',  ( 5.215576331900000362, 1455.428525482890109, 217.8852023316690065 ) ) ;
#5953=CARTESIAN_POINT ( 'NONE',  ( -9.828024485749999428, 1446.801136681789785, 212.2328357390990163 ) ) ;
#5959=CARTESIAN_POINT ( 'NONE',  ( -4.314880714020009833, 1453.742010946499931, 199.5809203820919890 ) ) ;
#5967=CARTESIAN_POINT ( 'NONE',  ( -0.3156253571057110463, 1500.458247417000166, 233.1765627430370103 ) ) ;
#5969=CARTESIAN_POINT ( 'NONE',  ( -0.7525844464480936358, 1473.757687442616771, 219.3350183411363048 ) ) ;
#5974=CARTESIAN_POINT ( 'NONE',  ( 18.13470581173330132, 1431.285403419799877, 206.8618331735010258 ) ) ;
#5975=CARTESIAN_POINT ( 'NONE',  ( -3.286483335600000277, 1456.341186815189758, 218.0120298563990104 ) ) ;
#5981=ORIENTED_EDGE ( 'NONE', *, *, #31167, .F. ) ;
#5983=CARTESIAN_POINT ( 'NONE',  ( -8.561916019487169294, 1448.548092552390017, 212.3149918286959803 ) ) ;
#5999=ORIENTED_EDGE ( 'NONE', *, *, #85173, .T. ) ;
#6002=CARTESIAN_POINT ( 'NONE',  ( 3.959152859930000101, 1428.396642669490120, 216.3690266601789745 ) ) ;
#6009=CARTESIAN_POINT ( 'NONE',  ( 8.466507779077819151, 1437.781662910839941, 212.4976436764690106 ) ) ;
#6015=CARTESIAN_POINT ( 'NONE',  ( -10.28735288409999882, 1471.931396637590069, 208.3821031841859792 ) ) ;
#6017=ORIENTED_EDGE ( 'NONE', *, *, #89082, .T. ) ;
#6025=CARTESIAN_POINT ( 'NONE',  ( 7.898231641030000638, 1488.783166887790003, 199.9435678271790096 ) ) ;
#6028=CARTESIAN_POINT ( 'NONE',  ( -1.842963673760081633, 1515.499673572818438, 205.0355315610892717 ) ) ;
#6031=B_SPLINE_CURVE_WITH_KNOTS ( 'NONE', 5,
 ( #7132, #42378, #42946, #85465, #52460, #8765 ),
 .UNSPECIFIED., .F., .F.,
 ( 6, 6 ),
 ( -1.999999948112589854, 0.000000000000000000 ),
 .UNSPECIFIED. ) ;
#6033=CARTESIAN_POINT ( 'NONE',  ( -17.55052187609999592, 1417.724842222909956, 206.6897972996389967 ) ) ;
#6037=CARTESIAN_POINT ( 'NONE',  ( -14.62138543496649845, 1508.449146121320155, 215.8538878429280032 ) ) ;
#6040=CARTESIAN_POINT ( 'NONE',  ( -11.35660239823070050, 1471.035763858380051, 207.9971984677779915 ) ) ;
#6047=CARTESIAN_POINT ( 'NONE',  ( -11.08439360582739930, 1470.227138793769882, 211.7024792797219845 ) ) ;
#6048=CARTESIAN_POINT ( 'NONE',  ( -18.10730182580141090, 1463.999204004485136, 217.9814146746393533 ) ) ;
#6050=ORIENTED_EDGE ( 'NONE', *, *, #71943, .T. ) ;
#6051=ORIENTED_EDGE ( 'NONE', *, *, #14089, .F. ) ;
#6052=CARTESIAN_POINT ( 'NONE',  ( 10.56872017243719952, 1481.355203388010068, 208.7623620626110039 ) ) ;
#6054=CARTESIAN_POINT ( 'NONE',  ( -5.051845285050000633, 1442.712514107189918, 200.9272700336389903 ) ) ;
#6057=CARTESIAN_POINT ( 'NONE',  ( 11.00329356315880069, 1422.205372314400165, 210.7649067250879966 ) ) ;
#6058=CARTESIAN_POINT ( 'NONE',  ( -10.63964957199999972, 1491.500814366789882, 212.0075699686489941 ) ) ;
#6064=CARTESIAN_POINT ( 'NONE',  ( 10.77265657036890012, 1491.996909311660147, 212.1278075563569985 ) ) ;
#6065=CARTESIAN_POINT ( 'NONE',  ( -1.875564068250000105, 1457.387223672290020, 219.2073648825989949 ) ) ;
#6066=VERTEX_POINT ( 'NONE', #40489 ) ;
#6069=CARTESIAN_POINT ( 'NONE',  ( 4.692464771457559358, 1508.551704408389924, 205.4575493268739876 ) ) ;
#6073=CARTESIAN_POINT ( 'NONE',  ( -3.272123973762000038, 1515.551704204689941, 205.4774943669999914 ) ) ;
#6075=CARTESIAN_POINT ( 'NONE',  ( -4.958564224928870168, 1476.141795758730041, 200.0452580833139962 ) ) ;
#6077=CARTESIAN_POINT ( 'NONE',  ( 7.000867164840526513, 1506.106661430532313, 218.4736308527704978 ) ) ;
#6079=CARTESIAN_POINT ( 'NONE',  ( -15.40447533607079578, 1419.996928346919958, 211.7847516026819505 ) ) ;
#6080=CARTESIAN_POINT ( 'NONE',  ( -15.88879189127879954, 1508.551704408389924, 213.9582233978679824 ) ) ;
#6083=CARTESIAN_POINT ( 'NONE',  ( 15.69667967640000050, 1457.921467858090182, 221.7535892932990009 ) ) ;
#6084=CARTESIAN_POINT ( 'NONE',  ( 6.867528398042960447, 1434.820408621019851, 203.9336372596199851 ) ) ;
#6104=CARTESIAN_POINT ( 'NONE',  ( 7.499139530464689507, 1425.344745441989971, 212.2485671964089988 ) ) ;
#6114=EDGE_LOOP ( 'NONE', ( #16513, #45958, #99431, #72538 ) ) ;
#6116=CARTESIAN_POINT ( 'NONE',  ( 10.93419921699999975, 1501.146262457190005, 205.7756198371390042 ) ) ;
#6118=CARTESIAN_POINT ( 'NONE',  ( 11.23465321549999985, 1501.870423235890030, 206.7487909662190191 ) ) ;
#6120=EDGE_LOOP ( 'NONE', ( #66319, #26316, #34487, #78376 ) ) ;
#6128=B_SPLINE_CURVE_WITH_KNOTS ( 'NONE', 3,
 ( #46673, #65663, #88665, #11943, #21954, #72419, #39343, #46124, #3571, #4645, #80253, #107652, #56147, #30936, #47204, #71898, #98694, #13018, #106014, #72959, #29290, #63486, #59470, #100349, #32041, #40438, #101983 ),
 .UNSPECIFIED., .F., .F.,
 ( 4, 2, 1, 1, 1, 1, 1, 1, 2, 2, 2, 2, 1, 1, 1, 2, 2, 4 ),
 ( 0.000000000000000000, 0.2499999999978366749, 0.3749999999967544850, 0.4374999999962133623, 0.4687499999959512942, 0.4843749999958125163, 0.4921874999957430719, 0.4960937499957076557, 0.4980468749956977748, 0.4999999999956878938, 0.6249999999967579267, 0.6874999999973000486, 0.7187499999975709430, 0.7343749999977112752, 0.7421874999977768894, 0.7460937499978097520, 0.7499999999978425036, 1.000000000000000000 ),
 .UNSPECIFIED. ) ;
#6135=CARTESIAN_POINT ( 'NONE',  ( 11.38572442648590055, 1480.473707728230011, 212.2056756853490072 ) ) ;
#6138=ORIENTED_EDGE ( 'NONE', *, *, #91780, .F. ) ;
#6140=CARTESIAN_POINT ( 'NONE',  ( -11.66561531531410090, 1481.205695410650151, 211.1318747291790032 ) ) ;
#6144=CARTESIAN_POINT ( 'NONE',  ( 11.30339187070000051, 1420.292009770159893, 198.6214305233989990 ) ) ;
#6147=CARTESIAN_POINT ( 'NONE',  ( -3.670436697740000032, 1428.951561676790107, 201.2856072060390034 ) ) ;
#6148=CARTESIAN_POINT ( 'NONE',  ( -4.744745735780000473, 1495.278903626390047, 198.1817743977989892 ) ) ;
#6153=CARTESIAN_POINT ( 'NONE',  ( 11.86987523124740029, 1426.731981355150083, 206.5550359663369875 ) ) ;
#6155=CARTESIAN_POINT ( 'NONE',  ( -9.721984167771511309, 1440.173042851740092, 206.7023544724380031 ) ) ;
#6159=AXIS2_PLACEMENT_3D ( 'NONE', #30330, #55017, #46065 ) ;
#6162=B_SPLINE_SURFACE_WITH_KNOTS ( 'NONE', 5, 5, ( 
 ( #102167, #50677, #76426, #110580, #59641, #17029 ),
 ( #43392, #51792, #8654, #69153, #34426, #42832 ),
 ( #76993, #86477, #68599, #102703, #25997, #60195 ),
 ( #94314, #9773, #75349, #109489, #10323, #28236 ),
 ( #2515, #18707, #27139, #88707, #95989, #104391 ),
 ( #62993, #36095, #78642, #87034, #106052, #44497 ),
 ( #63531, #36639, #105502, #28794, #61325, #69721 ),
 ( #43938, #95443, #53460, #70835, #52904, #103839 ),
 ( #1957, #70281, #27687, #104945, #61871, #19255 ) ),
 .UNSPECIFIED., .F., .F., .F.,
 ( 6, 3, 6 ),
 ( 6, 6 ),
 ( 3.650975912550000313, 7.249943402570000472, 12.02648879740000076 ),
 ( 0.000000000000000000, 2.000000000000000000 ),
 .UNSPECIFIED. ) ;
#6164=CARTESIAN_POINT ( 'NONE',  ( 9.368003223766120158, 1423.587887591870185, 210.1931883339019862 ) ) ;
#6165=CARTESIAN_POINT ( 'NONE',  ( 11.02661629080069972, 1423.097658921510174, 203.2974929890660007 ) ) ;
#6167=CARTESIAN_POINT ( 'NONE',  ( 5.009886284249999377, 1430.069699660889910, 217.1776678749689893 ) ) ;
#6171=ADVANCED_FACE ( 'NONE', ( #66281 ), #59886, .T. ) ;
#6173=B_SPLINE_SURFACE_WITH_KNOTS ( 'NONE', 5, 1, ( 
 ( #60404, #94523 ),
 ( #68815, #85566 ),
 ( #78288, #102916 ),
 ( #17797, #1602 ),
 ( #77204, #51998 ),
 ( #86138, #35182 ),
 ( #103475, #26781 ),
 ( #60969, #18360 ),
 ( #52554, #9982 ) ),
 .UNSPECIFIED., .F., .F., .F.,
 ( 6, 3, 6 ),
 ( 2, 2 ),
 ( 0.000000000000000000, 3.619946782640000027, 7.224553348539999753 ),
 ( 0.000000000000000000, 14.00000000000000000 ),
 .UNSPECIFIED. ) ;
#6176=CARTESIAN_POINT ( 'NONE',  ( -7.362157615257188148, 1458.222784178867641, 215.2209630148805104 ) ) ;
#6182=CARTESIAN_POINT ( 'NONE',  ( -20.68581318029999849, 1486.599741798989953, 210.1122336357950076 ) ) ;
#6191=CARTESIAN_POINT ( 'NONE',  ( 3.350944662710000355, 1464.628126271390101, 199.8699733667390035 ) ) ;
#6197=CARTESIAN_POINT ( 'NONE',  ( 2.980241439829999894, 1451.608296861789995, 190.1062771521989987 ) ) ;
#6198=ORIENTED_EDGE ( 'NONE', *, *, #24711, .F. ) ;
#6199=CARTESIAN_POINT ( 'NONE',  ( -0.7146574492519990329, 1485.443249444889943, 197.9912040296989915 ) ) ;
#6202=CARTESIAN_POINT ( 'NONE',  ( -11.69964062410000061, 1491.144390090590150, 207.3445954516889742 ) ) ;
#6206=CARTESIAN_POINT ( 'NONE',  ( -16.91629849159999921, 1419.609072056739933, 208.4236488388899886 ) ) ;
#6210=CARTESIAN_POINT ( 'NONE',  ( -12.23540616512669921, 1490.610661065379873, 208.3569505650620215 ) ) ;
#6212=ORIENTED_EDGE ( 'NONE', *, *, #22433, .T. ) ;
#6218=CARTESIAN_POINT ( 'NONE',  ( 10.47535534418940095, 1470.915150549339842, 210.4403342155679866 ) ) ;
#6231=TOROIDAL_SURFACE ( 'NONE', #34846, 6.646318662569999702, 0.5000000000000000000 ) ;
#6245=CARTESIAN_POINT ( 'NONE',  ( 2.851735618451650023, 1484.953707064400078, 220.6267593247900152 ) ) ;
#6256=EDGE_CURVE ( 'NONE', #56179, #94930, #89025, .T. ) ;
#6259=ADVANCED_FACE ( 'NONE', ( #35399 ), #44934, .T. ) ;
#6262=CARTESIAN_POINT ( 'NONE',  ( 13.52268460260000005, 1497.923627545689897, 227.8730058995990078 ) ) ;
#6264=ORIENTED_EDGE ( 'NONE', *, *, #50747, .T. ) ;
#6265=ORIENTED_EDGE ( 'NONE', *, *, #94794, .T. ) ;
#6267=CARTESIAN_POINT ( 'NONE',  ( 3.637353868009999935, 1426.366397907009969, 191.4055625021989897 ) ) ;
#6270=CARTESIAN_POINT ( 'NONE',  ( -19.38312692761750000, 1508.551704424289937, 210.1488772976939856 ) ) ;
#6271=CARTESIAN_POINT ( 'NONE',  ( 2.330134126090001701, 1515.551704408337173, 205.1635078156689929 ) ) ;
#6288=CARTESIAN_POINT ( 'NONE',  ( 7.660102788296829779, 1428.868901441670005, 214.7109318833680049 ) ) ;
#6289=CARTESIAN_POINT ( 'NONE',  ( -18.75627164819999848, 1442.404900751590048, 208.2000273071639924 ) ) ;
#6301=B_SPLINE_SURFACE_WITH_KNOTS ( 'NONE', 5, 5, ( 
 ( #19936, #96665, #79314, #37308, #36750, #4260 ),
 ( #4788, #3728, #29987, #88808, #98300, #72569 ),
 ( #79866, #46829, #54682, #71503, #53576, #63637 ),
 ( #29438, #55784, #97198, #3176, #27795, #106696 ),
 ( #80958, #28906, #97751, #64179, #88260, #87723 ),
 ( #55226, #70942, #21576, #89900, #13171, #47360 ),
 ( #63101, #37858, #72044, #28349, #12091, #38934 ),
 ( #11001, #106161, #73114, #80414, #61982, #45173 ),
 ( #105059, #62544, #91564, #92653, #22115, #90998 ) ),
 .UNSPECIFIED., .F., .F., .F.,
 ( 6, 3, 6 ),
 ( 6, 6 ),
 ( 3.061701835029610130, 6.405260106299999201, 7.456840382068469886 ),
 ( -0.0004170354784579379903, 2.000000000000000000 ),
 .UNSPECIFIED. ) ;
#6309=CARTESIAN_POINT ( 'NONE',  ( 3.542288683788520132, 1515.375307391110027, 213.1422521534840087 ) ) ;
#6311=CARTESIAN_POINT ( 'NONE',  ( -12.28882577965210032, 1501.802949440490011, 211.5612507580339923 ) ) ;
#6312=ORIENTED_EDGE ( 'NONE', *, *, #80921, .T. ) ;
#6317=CARTESIAN_POINT ( 'NONE',  ( -4.553191091878280083, 1442.065269977319986, 201.3752770252120001 ) ) ;
#6319=CARTESIAN_POINT ( 'NONE',  ( 20.74641727850000095, 1496.330958597389781, 205.0865742704490060 ) ) ;
#6323=CARTESIAN_POINT ( 'NONE',  ( 6.537728378210000635, 1462.897344095490098, 208.5037906403959767 ) ) ;
#6324=ORIENTED_EDGE ( 'NONE', *, *, #69262, .F. ) ;
#6328=CARTESIAN_POINT ( 'NONE',  ( -3.703568344589999839, 1497.311626104689822, 220.9591690177990131 ) ) ;
#6332=EDGE_CURVE ( 'NONE', #29958, #5600, #105800, .T. ) ;
#6335=CARTESIAN_POINT ( 'NONE',  ( -10.29908310198690025, 1447.573334503160140, 210.1662163023220273 ) ) ;
#6340=CARTESIAN_POINT ( 'NONE',  ( -10.49383960940000016, 1500.045019812190276, 215.0277856566890193 ) ) ;
#6358=CARTESIAN_POINT ( 'NONE',  ( 12.91118672957320079, 1421.030139935020088, 203.7088207097539794 ) ) ;
#6359=EDGE_CURVE ( 'NONE', #45310, #61133, #86480, .T. ) ;
#6363=CARTESIAN_POINT ( 'NONE',  ( -13.59378551342209818, 1507.992802046239831, 209.4432269169830079 ) ) ;
#6365=CARTESIAN_POINT ( 'NONE',  ( -17.51543818711899902, 1417.552356043139980, 206.7803260800679936 ) ) ;
#6370=CARTESIAN_POINT ( 'NONE',  ( -14.68773312159869882, 1420.564508854909946, 212.7973254087889927 ) ) ;
#6375=DIRECTION ( 'NONE',  ( 1.000000000000000000, 0.000000000000000000, 0.000000000000000000 ) ) ;
#6377=CARTESIAN_POINT ( 'NONE',  ( -18.98074344019839899, 1419.205094861039925, 205.9182421121359994 ) ) ;
#6386=ORIENTED_EDGE ( 'NONE', *, *, #46636, .T. ) ;
#6388=EDGE_CURVE ( 'NONE', #98779, #18748, #109124, .T. ) ;
#6390=CARTESIAN_POINT ( 'NONE',  ( 15.32773529925650102, 1420.119835273649869, 210.6256678854140034 ) ) ;
#6396=CARTESIAN_POINT ( 'NONE',  ( -3.509040552655700029, 1464.225060470080052, 199.5119554303080065 ) ) ;
#6403=EDGE_LOOP ( 'NONE', ( #42198, #100667, #76778, #6422 ) ) ;
#6407=EDGE_CURVE ( 'NONE', #34770, #20056, #82557, .T. ) ;
#6413=ADVANCED_FACE ( 'NONE', ( #46581 ), #72905, .T. ) ;
#6415=EDGE_LOOP ( 'NONE', ( #96, #24588, #23195, #31135 ) ) ;
#6416=CARTESIAN_POINT ( 'NONE',  ( -11.62340356170000000, 1502.516964898590004, 208.1148589984090052 ) ) ;
#6422=ORIENTED_EDGE ( 'NONE', *, *, #25350, .F. ) ;
#6424=CARTESIAN_POINT ( 'NONE',  ( -7.156442445803939734, 1453.513166831520039, 203.0923578546739918 ) ) ;
#6442=CARTESIAN_POINT ( 'NONE',  ( 9.788553136239070085, 1435.243871060430138, 208.4607419252359932 ) ) ;
#6446=VERTEX_POINT ( 'NONE', #15668 ) ;
#6451=CARTESIAN_POINT ( 'NONE',  ( 6.554685473989913191, 1473.611172115990030, 218.5142022801588553 ) ) ;
#6452=CARTESIAN_POINT ( 'NONE',  ( 12.23498997169999924, 1421.239601672929894, 203.4474965640889934 ) ) ;
#6453=CARTESIAN_POINT ( 'NONE',  ( -2.214263094331805348, 1497.815544588951980, 198.0520811483251293 ) ) ;
#6463=CARTESIAN_POINT ( 'NONE',  ( 10.90371891546730154, 1461.552474635850103, 210.3079516580219774 ) ) ;
#6464=CARTESIAN_POINT ( 'NONE',  ( 8.297169622465377259, 1424.294093603346710, 195.8426830675071244 ) ) ;
#6465=CARTESIAN_POINT ( 'NONE',  ( 4.639337580630000346, 1465.928856497889910, 219.1434977748990036 ) ) ;
#6474=EDGE_LOOP ( 'NONE', ( #65988, #17906, #105704, #13012, #63697 ) ) ;
#6477=CARTESIAN_POINT ( 'NONE',  ( 9.799878764200000703, 1423.431745859970079, 209.4822081458350169 ) ) ;
#6481=CARTESIAN_POINT ( 'NONE',  ( -9.905282292037359326, 1438.748818913890091, 210.0876870654180095 ) ) ;
#6484=CARTESIAN_POINT ( 'NONE',  ( -14.16774589291680009, 1415.677402201999939, 204.4588472394289624 ) ) ;
#6498=CARTESIAN_POINT ( 'NONE',  ( -2.391931473960000165, 1445.002411567389800, 217.8135387986989997 ) ) ;
#6504=CARTESIAN_POINT ( 'NONE',  ( -3.857685964098449993, 1453.986003452039995, 199.3820233995429874 ) ) ;
#6509=DIRECTION ( 'NONE',  ( -1.224646799147350002E-16, 1.836970198721029688E-16, 1.000000000000000000 ) ) ;
#6511=EDGE_LOOP ( 'NONE', ( #88904, #102526, #2843, #100300, #31212, #65315, #24732, #81040, #110198, #45270, #29478, #100457, #15424, #79597 ) ) ;
#6514=CARTESIAN_POINT ( 'NONE',  ( 19.17904245640259830, 1497.230174812279984, 221.9978027818679891 ) ) ;
#6521=CARTESIAN_POINT ( 'NONE',  ( -20.59722728060000208, 1484.571346146590031, 210.1121776662889999 ) ) ;
#6522=CARTESIAN_POINT ( 'NONE',  ( 18.27180342219620002, 1431.618699553079978, 208.4181533866990037 ) ) ;
#6523=CARTESIAN_POINT ( 'NONE',  ( -3.597719018270000291, 1458.022133392390060, 218.7636985456790057 ) ) ;
#6529=CARTESIAN_POINT ( 'NONE',  ( -4.328142686769930414, 1515.114670419599861, 210.0487672904759791 ) ) ;
#6535=CARTESIAN_POINT ( 'NONE',  ( 8.854488364011938728, 1425.207168016459946, 194.9722730769710211 ) ) ;
#6540=CARTESIAN_POINT ( 'NONE',  ( 2.175409717514719593E-31, 1397.551704408390151, 209.1218459616989946 ) ) ;
#6544=B_SPLINE_CURVE_WITH_KNOTS ( 'NONE', 3,
 ( #52853, #18108, #78028, #1336, #61274, #44446, #45565, #78590, #79706, #36044, #27630, #19199, #61816, #53401, #87552, #10840 ),
 .UNSPECIFIED., .F., .F.,
 ( 4, 3, 3, 3, 3, 4 ),
 ( -14.84820554333979992, -14.42705417563930048, -13.45967978722200087, -12.49597291703340041, -11.53390232449759978, -10.57397516620000033 ),
 .UNSPECIFIED. ) ;
#6553=ORIENTED_EDGE ( 'NONE', *, *, #89960, .T. ) ;
#6559=EDGE_CURVE ( 'NONE', #18694, #34842, #10344, .T. ) ;
#6564=CARTESIAN_POINT ( 'NONE',  ( 9.377625631454941768, 1436.953526060589866, 212.2519149868810189 ) ) ;
#6567=ADVANCED_FACE ( 'NONE', ( #79489 ), #77777, .F. ) ;
#6568=ORIENTED_EDGE ( 'NONE', *, *, #83590, .T. ) ;
#6570=CARTESIAN_POINT ( 'NONE',  ( -9.978326636743720002, 1439.380423524790103, 208.6695145202539834 ) ) ;
#6580=CARTESIAN_POINT ( 'NONE',  ( 5.281945572889999774, 1487.428016119789845, 199.2096035253390198 ) ) ;
#6588=CARTESIAN_POINT ( 'NONE',  ( -16.87841318179999917, 1420.387307786450037, 203.7287732364889905 ) ) ;
#6589=CARTESIAN_POINT ( 'NONE',  ( -16.36323254953610373, 1508.551704408389924, 213.3980841489470208 ) ) ;
#6590=CARTESIAN_POINT ( 'NONE',  ( -2.119623532050000314, 1475.831458439090056, 219.9786267809990079 ) ) ;
#6595=CARTESIAN_POINT ( 'NONE',  ( -1.615118886346869953, 1455.072079523880120, 198.7395845362720195 ) ) ;
#6598=CARTESIAN_POINT ( 'NONE',  ( -11.01233496866419870, 1470.178673701140042, 211.9709904787150094 ) ) ;
#6604=CARTESIAN_POINT ( 'NONE',  ( -4.958564224928870168, 1476.141795758730041, 200.0452580833139962 ) ) ;
#6607=CARTESIAN_POINT ( 'NONE',  ( 11.41298749625700104, 1502.480512559349791, 211.2134296033459862 ) ) ;
#6608=CARTESIAN_POINT ( 'NONE',  ( -762.4595216451192528, -8387.357407334291565, -1619.875998970129785 ) ) ;
#6610=CARTESIAN_POINT ( 'NONE',  ( 1.289688745822530125, 1508.551704408389924, 219.8224770426249677 ) ) ;
#6614=DIRECTION ( 'NONE',  ( -0.8907681516580507886, 0.000000000000000000, 0.4544580288560209347 ) ) ;
#6615=CARTESIAN_POINT ( 'NONE',  ( 10.96547367623530000, 1490.901970238939839, 209.8192269860039971 ) ) ;
#6618=CARTESIAN_POINT ( 'NONE',  ( -20.60448988230000111, 1484.737042837089803, 209.1218459616989946 ) ) ;
#6627=CARTESIAN_POINT ( 'NONE',  ( 3.666164899629999585, 1486.466096722590009, 219.2737630301990066 ) ) ;
#6628=CARTESIAN_POINT ( 'NONE',  ( -7.996087907170001507, 1462.263563461390049, 203.4213808977189899 ) ) ;
#6630=CARTESIAN_POINT ( 'NONE',  ( 4.760896992130000172, 1449.971761959190189, 190.6385172635989704 ) ) ;
#6631=CARTESIAN_POINT ( 'NONE',  ( -10.80382370743670073, 1508.551704408389924, 217.9004706025669975 ) ) ;
#6635=CARTESIAN_POINT ( 'NONE',  ( 3.967425320557659507, 1431.784486675220023, 200.3531835805560206 ) ) ;
#6658=CARTESIAN_POINT ( 'NONE',  ( 7.509953471767339295, 1425.386002328900076, 212.2272222051859956 ) ) ;
#6659=ORIENTED_EDGE ( 'NONE', *, *, #18790, .T. ) ;
#6664=CARTESIAN_POINT ( 'NONE',  ( -6.208076407620000126, 1461.436029833090060, 207.2638656286190155 ) ) ;
#6666=CARTESIAN_POINT ( 'NONE',  ( -4.646147438016499542, 1378.399971910029990, 214.5514622210689879 ) ) ;
#6670=ORIENTED_EDGE ( 'NONE', *, *, #80171, .T. ) ;
#6674=CARTESIAN_POINT ( 'NONE',  ( 10.08490127059999963, 1462.177701891290099, 210.4147059520890082 ) ) ;
#6682=CARTESIAN_POINT ( 'NONE',  ( 7.468436490899999392, 1491.313758626190065, 211.3467155923090104 ) ) ;
#6694=CARTESIAN_POINT ( 'NONE',  ( 4.343364931220000003, 1426.780599525880007, 211.8480867413289843 ) ) ;
#6697=CARTESIAN_POINT ( 'NONE',  ( 7.302416004457981558, 1435.594922686310838, 204.5677890833769652 ) ) ;
#6699=CARTESIAN_POINT ( 'NONE',  ( 6.966807131377220408, 1504.412568754190033, 219.8081154884820023 ) ) ;
#6700=CARTESIAN_POINT ( 'NONE',  ( 7.455473913919999696, 1422.775276769710217, 195.6452099806990077 ) ) ;
#6701=CARTESIAN_POINT ( 'NONE',  ( 1.233474458951280051, 1431.395778057770031, 218.5319384325650276 ) ) ;
#6702=CARTESIAN_POINT ( 'NONE',  ( -5.254485968520000050, 1494.936664904289955, 197.9757700040989903 ) ) ;
#6706=CARTESIAN_POINT ( 'NONE',  ( 11.56989304032649812, 1426.466096579750001, 206.5199424030009823 ) ) ;
#6715=CARTESIAN_POINT ( 'NONE',  ( 9.362767939971719855, 1424.864447360270105, 209.3171238155310050 ) ) ;
#6716=CARTESIAN_POINT ( 'NONE',  ( 11.53900508938759906, 1422.010879093899803, 203.4012210850169993 ) ) ;
#6717=CARTESIAN_POINT ( 'NONE',  ( -11.01004492055549910, 1462.557516207839853, 208.2324619591759927 ) ) ;
#6723=CARTESIAN_POINT ( 'NONE',  ( 4.487249773072029768, 1509.038615930399828, 211.6097810847319920 ) ) ;
#6725=CARTESIAN_POINT ( 'NONE',  ( 5.544572127002579620, 1465.561989329190055, 218.7012434299869881 ) ) ;
#6730=CARTESIAN_POINT ( 'NONE',  ( 5.550896940410000369, 1461.183176948789878, 205.2452863306889981 ) ) ;
#6733=CARTESIAN_POINT ( 'NONE',  ( 12.74509880840539999, 1426.619167131859967, 203.6612177353580080 ) ) ;
#6736=CARTESIAN_POINT ( 'NONE',  ( 9.762629409768241118, 1468.224221565797279, 206.7965198539660321 ) ) ;
#6748=CARTESIAN_POINT ( 'NONE',  ( 1.894388308689999967, 1506.148290744889891, 221.7829938216989945 ) ) ;
#6751=CARTESIAN_POINT ( 'NONE',  ( -16.22868724909999827, 1418.857858964219986, 209.4919173468780116 ) ) ;
#6756=CARTESIAN_POINT ( 'NONE',  ( 10.31871872550729918, 1424.391353036610099, 207.1214719758330034 ) ) ;
#6760=CARTESIAN_POINT ( 'NONE',  ( 1.886382439867170024, 1437.487153458199828, 227.5670087340569978 ) ) ;
#6762=CARTESIAN_POINT ( 'NONE',  ( 4.972072924729999954, 1472.535148281390093, 218.0116174414390002 ) ) ;
#6763=CARTESIAN_POINT ( 'NONE',  ( 9.690921760896669568, 1469.947179451500006, 211.8829996226070023 ) ) ;
#6766=DIRECTION ( 'NONE',  ( -7.436362843295819681E-17, 1.000000000000000000, -1.457576885956999882E-16 ) ) ;
#6771=CARTESIAN_POINT ( 'NONE',  ( 9.698381235350000296, 1450.963213650890111, 206.3010183936889916 ) ) ;
#6775=CARTESIAN_POINT ( 'NONE',  ( -1.100379444789999939, 1455.838357077089768, 199.3345172646990022 ) ) ;
#6777=B_SPLINE_CURVE_WITH_KNOTS ( 'NONE', 5,
 ( #85214, #77388, #61174, #1804, #84664, #50539 ),
 .UNSPECIFIED., .F., .F.,
 ( 6, 6 ),
 ( 141.1642459979999842, 150.6560418210000023 ),
 .UNSPECIFIED. ) ;
#6789=CARTESIAN_POINT ( 'NONE',  ( 11.36630642249999923, 1502.069393327289845, 207.5140256288290175 ) ) ;
#6794=B_SPLINE_CURVE_WITH_KNOTS ( 'NONE', 3,
 ( #34593, #60364, #2130, #95060, #51961, #35697, #85530, #44117, #36254, #8824, #18327, #1565, #94486, #69886, #35145, #105118 ),
 .UNSPECIFIED., .F., .F.,
 ( 4, 3, 3, 3, 3, 4 ),
 ( -7.454956845832920287, -7.041679458493519839, -6.041855899781880090, -5.045615715417369529, -4.051023835724380184, -3.058675454860000364 ),
 .UNSPECIFIED. ) ;
#6797=CARTESIAN_POINT ( 'NONE',  ( 12.64308048353610126, 1500.885237595450008, 210.4353653217530109 ) ) ;
#6801=CARTESIAN_POINT ( 'NONE',  ( -16.61337445550000069, 1463.629612651790012, 220.4655171657990138 ) ) ;
#6803=ORIENTED_EDGE ( 'NONE', *, *, #2824, .T. ) ;
#6804=ORIENTED_EDGE ( 'NONE', *, *, #56458, .F. ) ;
#6805=B_SPLINE_CURVE_WITH_KNOTS ( 'NONE', 3,
 ( #71080, #44201, #20079, #11156, #1655, #18406, #18963, #78346, #86740, #10032, #105205, #96809, #52051, #54273, #35791, #68865, #11690, #102969, #103532, #95145, #27941, #26267, #62122, #2218, #45317, #96249, #69975, #19523, #1103, #60457, #88398 ),
 .UNSPECIFIED., .F., .F.,
 ( 4, 3, 3, 3, 3, 3, 3, 3, 3, 3, 4 ),
 ( 2.324858856890000158, 2.629659992475509966, 2.924842188867320392, 3.130565735668509930, 3.432172540442299802, 3.731439316943959916, 4.025646101810540500, 4.318556006757110488, 4.608870342396969910, 4.895817133586150227, 4.991117563610000474 ),
 .UNSPECIFIED. ) ;
#6810=CARTESIAN_POINT ( 'NONE',  ( -21.11329577064019958, 1508.551704414039932, 210.1840812171020048 ) ) ;
#6812=CARTESIAN_POINT ( 'NONE',  ( 3.401541474470889614, 1468.225229937070026, 218.5224292273400124 ) ) ;
#6819=ORIENTED_EDGE ( 'NONE', *, *, #51369, .F. ) ;
#6822=EDGE_LOOP ( 'NONE', ( #50881, #56359, #102236, #102265 ) ) ;
#6829=CARTESIAN_POINT ( 'NONE',  ( -9.343473286536170264, 1461.635954483039995, 206.4705841331299894 ) ) ;
#6831=CARTESIAN_POINT ( 'NONE',  ( 9.908749694887600157, 1468.699217298059921, 207.6203599669360074 ) ) ;
#6832=CARTESIAN_POINT ( 'NONE',  ( -6.488994010384053546, 1468.824241490008717, 218.3969213443690762 ) ) ;
#6837=CARTESIAN_POINT ( 'NONE',  ( 9.079024693347159669, 1468.625100210450000, 202.5093681977309927 ) ) ;
#6842=CARTESIAN_POINT ( 'NONE',  ( -15.77149559868386675, 1420.276057766250915, 210.6539470928313165 ) ) ;
#6847=CARTESIAN_POINT ( 'NONE',  ( -11.87651332576620078, 1501.535165843179811, 211.4045997421629863 ) ) ;
#6850=CARTESIAN_POINT ( 'NONE',  ( -1.568956603680000006, 1508.180600514190019, 220.9064527986990072 ) ) ;
#6852=CARTESIAN_POINT ( 'NONE',  ( 1.557255085340000011, 1435.511706276389987, 227.5437143207990118 ) ) ;
#6855=CARTESIAN_POINT ( 'NONE',  ( -6.544710712048379619, 1426.691555418079815, 202.4711062780949931 ) ) ;
#6859=CARTESIAN_POINT ( 'NONE',  ( -10.71539411164560107, 1482.205790377970288, 206.4284175877959910 ) ) ;
#6867=CARTESIAN_POINT ( 'NONE',  ( 10.94830312428359953, 1490.380690179980093, 209.7447272360980151 ) ) ;
#6876=DIRECTION ( 'NONE',  ( 9.261055619630009070E-47, -1.000000000000000000, 1.836970198721029688E-16 ) ) ;
#6877=CARTESIAN_POINT ( 'NONE',  ( -15.56126507649999979, 1417.814061455979981, 204.2177041305290004 ) ) ;
#6882=CARTESIAN_POINT ( 'NONE',  ( -16.15556852644305863, 1419.752504305882894, 210.0532078212941940 ) ) ;
#6883=CARTESIAN_POINT ( 'NONE',  ( -4.212749018120000244, 1497.360448316590009, 220.3810617930989793 ) ) ;
#6888=CIRCLE ( 'NONE', #22938, 975.0211406871101190 ) ;
#6889=CARTESIAN_POINT ( 'NONE',  ( -7.980162481601299262, 1424.786834349992887, 210.5240428619318322 ) ) ;
#6896=CARTESIAN_POINT ( 'NONE',  ( 4.038582018749999669, 1515.598601288590089, 209.1218459616989946 ) ) ;
#6902=CARTESIAN_POINT ( 'NONE',  ( 10.53834095255740166, 1479.220444398180007, 206.2733528961080083 ) ) ;
#6905=CARTESIAN_POINT ( 'NONE',  ( -9.488417199124221213, 1447.702184401620116, 190.7505744106450152 ) ) ;
#6920=CARTESIAN_POINT ( 'NONE',  ( -22.90642118200990041, 1417.395382955499826, 209.8927238903939951 ) ) ;
#6929=ORIENTED_EDGE ( 'NONE', *, *, #3181, .T. ) ;
#6937=CARTESIAN_POINT ( 'NONE',  ( -17.34523078839999854, 1417.790224563129868, 207.1689930853989949 ) ) ;
#6957=CARTESIAN_POINT ( 'NONE',  ( -11.40807687090000044, 1502.267969405689882, 207.7237911178790171 ) ) ;
#6963=ORIENTED_EDGE ( 'NONE', *, *, #69228, .F. ) ;
#6965=CARTESIAN_POINT ( 'NONE',  ( -7.977617884082539135, 1452.731462069070176, 204.2954127766810188 ) ) ;
#6981=CARTESIAN_POINT ( 'NONE',  ( 16.69693468393730029, 1428.155315606670001, 202.0365457747359699 ) ) ;
#6992=DIRECTION ( 'NONE',  ( 0.000000000000000000, -1.000000000000000000, 0.000000000000000000 ) ) ;
#6993=CARTESIAN_POINT ( 'NONE',  ( -2.361220391463635160, 1495.123712929674411, 220.0409822458833844 ) ) ;
#6994=CARTESIAN_POINT ( 'NONE',  ( 6.104420695803289831, 1484.441873671279836, 218.1702592719159952 ) ) ;
#6995=FACE_OUTER_BOUND ( 'NONE', #19469, .T. ) ;
#6999=CARTESIAN_POINT ( 'NONE',  ( -10.35382106464290075, 1447.820467530350015, 209.5541548230679894 ) ) ;
#7001=VERTEX_POINT ( 'NONE', #8186 ) ;
#7008=CARTESIAN_POINT ( 'NONE',  ( 10.80995225166140017, 1461.830262730540198, 211.0065464265690025 ) ) ;
#7020=CARTESIAN_POINT ( 'NONE',  ( 3.775314256393730084, 1507.374707593759922, 220.2027404254530154 ) ) ;
#7022=ORIENTED_EDGE ( 'NONE', *, *, #26100, .F. ) ;
#7023=CARTESIAN_POINT ( 'NONE',  ( -8.377772372675931223, 1439.624752306900064, 206.1459263295090238 ) ) ;
#7028=CARTESIAN_POINT ( 'NONE',  ( -5.192567649020000786, 1483.459673190490093, 199.8090161968289635 ) ) ;
#7031=CARTESIAN_POINT ( 'NONE',  ( -8.589403565197139656, 1436.797923814430078, 209.9038308123180059 ) ) ;
#7046=B_SPLINE_CURVE_WITH_KNOTS ( 'NONE', 3,
 ( #68412, #102515, #67306, #25252, #7916, #109841, #58890, #93023, #16295, #84621, #51041, #50499, #42087, #110383, #76236, #59455, #16840, #101966, #57943, #6424, #23205, #48444, #14808, #31611, #109442, #6965, #73082, #82583, #57404, #15348, #38899, #39473, #90966, #101009, #92075, #40016, #107222, #107774, #30511, #64700, #74196, #98818, #49543 ),
 .UNSPECIFIED., .F., .F.,
 ( 4, 3, 3, 3, 3, 3, 3, 3, 3, 3, 3, 3, 3, 3, 4 ),
 ( -31.90163827269670094, -31.43425787619030132, -29.98858318685319801, -28.53496177318270099, -27.07797101134740103, -26.89876598673080110, -25.44723142269879901, -23.99928790089909825, -22.55496867767820035, -21.04730123312180012, -19.61770596032359748, -18.19541948610630300, -16.78105471453919861, -15.31006667213799943, -13.91937871329999865 ),
 .UNSPECIFIED. ) ;
#7048=CARTESIAN_POINT ( 'NONE',  ( 2.216729547819999979, 1455.498911564990067, 218.4410051553589938 ) ) ;
#7050=CARTESIAN_POINT ( 'NONE',  ( -2.090539597859999876, 1443.965784278489764, 218.2184972947390236 ) ) ;
#7056=CARTESIAN_POINT ( 'NONE',  ( 7.535764321409999411, 1423.202263985780064, 213.6586556354689890 ) ) ;
#7067=CARTESIAN_POINT ( 'NONE',  ( 14.00740487959999925, 1500.888346221290021, 227.6900866534990087 ) ) ;
#7069=CARTESIAN_POINT ( 'NONE',  ( -10.76610293753739889, 1461.751116445120033, 211.3389343603909936 ) ) ;
#7075=CARTESIAN_POINT ( 'NONE',  ( 9.919384991629041082, 1468.593841060750037, 207.7518384896150110 ) ) ;
#7081=B_SPLINE_SURFACE_WITH_KNOTS ( 'NONE', 5, 1, ( 
 ( #86287, #79020 ),
 ( #19626, #1202 ),
 ( #96349, #35335 ),
 ( #10133, #62790 ),
 ( #11257, #44305 ),
 ( #19059, #78448 ) ),
 .UNSPECIFIED., .F., .F., .F.,
 ( 6, 6 ),
 ( 2, 2 ),
 ( 0.000000000000000000, 3.595663933400000012 ),
 ( 0.000000000000000000, 14.00000000000000000 ),
 .UNSPECIFIED. ) ;
#7086=CARTESIAN_POINT ( 'NONE',  ( 7.705921152320070355, 1424.884187513139977, 194.3337803165900084 ) ) ;
#7097=CARTESIAN_POINT ( 'NONE',  ( 10.27486387009999902, 1471.877390917489947, 213.0768048428889756 ) ) ;
#7100=B_SPLINE_CURVE_WITH_KNOTS ( 'NONE', 3,
 ( #67459, #93175, #16445, #8069 ),
 .UNSPECIFIED., .F., .F.,
 ( 4, 4 ),
 ( 0.000000000000000000, 1.000000000000000000 ),
 .UNSPECIFIED. ) ;
#7106=CARTESIAN_POINT ( 'NONE',  ( 5.826685344680000433, 1451.766759332889933, 210.9235202141190086 ) ) ;
#7108=CARTESIAN_POINT ( 'NONE',  ( 1.353590696506990154, 1425.853514710840045, 191.1378424660090047 ) ) ;
#7113=CARTESIAN_POINT ( 'NONE',  ( 5.398404081564367019, 1459.746910339853230, 201.1147253787919169 ) ) ;
#7115=FACE_OUTER_BOUND ( 'NONE', #38780, .T. ) ;
#7120=CARTESIAN_POINT ( 'NONE',  ( -11.27244568259999902, 1471.218590734589952, 207.2933119717289969 ) ) ;
#7123=CARTESIAN_POINT ( 'NONE',  ( 7.331631502509999621, 1481.335631838190011, 208.7201577476780017 ) ) ;
#7127=CARTESIAN_POINT ( 'NONE',  ( -17.64296983559999887, 1417.255069634780057, 208.0149687280789976 ) ) ;
#7130=CARTESIAN_POINT ( 'NONE',  ( 7.000551371890000318, 1488.139301625489907, 200.2663657335290281 ) ) ;
#7132=CARTESIAN_POINT ( 'NONE',  ( 10.92857032808210072, 1460.888924644350027, 208.5047758900509791 ) ) ;
#7136=CARTESIAN_POINT ( 'NONE',  ( 18.25280056480000113, 1432.153207019990077, 210.9297336666290050 ) ) ;
#7139=DIRECTION ( 'NONE',  ( -9.462326934583649054E-47, 1.000000000000000000, -1.836970198721029688E-16 ) ) ;
#7144=CARTESIAN_POINT ( 'NONE',  ( -2.023054527036900030, 1423.041924723330112, 191.3215604683840070 ) ) ;
#7145=CARTESIAN_POINT ( 'NONE',  ( -11.36893632117620001, 1470.999913913189857, 208.1399306574149932 ) ) ;
#7146=CARTESIAN_POINT ( 'NONE',  ( -6.565194752462199190, 1508.347353571651638, 219.9240066229079105 ) ) ;
#7150=CARTESIAN_POINT ( 'NONE',  ( -3.958338178574812627, 1515.551704408389696, 210.9648098108357033 ) ) ;
#7152=CARTESIAN_POINT ( 'NONE',  ( -10.13174304484510024, 1472.026935049100075, 209.9584671908849884 ) ) ;
#7153=CARTESIAN_POINT ( 'NONE',  ( 4.328426199472190206, 1515.103843506339899, 208.0564445731249918 ) ) ;
#7156=ADVANCED_FACE ( 'NONE', ( #40572 ), #63763, .T. ) ;
#7158=EDGE_CURVE ( 'NONE', #36610, #41661, #55585, .T. ) ;
#7161=FACE_OUTER_BOUND ( 'NONE', #10061, .T. ) ;
#7170=CARTESIAN_POINT ( 'NONE',  ( 12.27488635486660051, 1492.418620469620009, 210.4946640001330138 ) ) ;
#7171=CARTESIAN_POINT ( 'NONE',  ( 0.3560709500229989888, 1455.537836849089899, 218.5814834089789827 ) ) ;
#7175=B_SPLINE_CURVE_WITH_KNOTS ( 'NONE', 5,
 ( #103520, #18953, #2208, #105192, #28484, #62676 ),
 .UNSPECIFIED., .F., .F.,
 ( 6, 6 ),
 ( 0.000000000000000000, 1.000000000000000000 ),
 .UNSPECIFIED. ) ;
#7178=CARTESIAN_POINT ( 'NONE',  ( 8.319417205733840248, 1436.545527341170100, 206.8831545614739866 ) ) ;
#7181=CARTESIAN_POINT ( 'NONE',  ( -21.43625278670000256, 1505.201739750890056, 211.1850546088390104 ) ) ;
#7182=CARTESIAN_POINT ( 'NONE',  ( -2.801044513574019845, 1515.551704203360032, 205.2926231456509925 ) ) ;
#7187=CARTESIAN_POINT ( 'NONE',  ( -9.025098172850000822, 1462.934938264289940, 204.1976517399190243 ) ) ;
#7189=CARTESIAN_POINT ( 'NONE',  ( 1.378013107889999977, 1443.686999423290217, 202.9879073201189783 ) ) ;
#7194=CARTESIAN_POINT ( 'NONE',  ( 2.166404729989209965, 1486.720363920270074, 197.3876830102489919 ) ) ;
#7195=EDGE_CURVE ( 'NONE', #74194, #51048, #27605, .T. ) ;
#7208=CARTESIAN_POINT ( 'NONE',  ( 1.698736666709999898, 1476.148439429189921, 197.7469619067989868 ) ) ;
#7214=CARTESIAN_POINT ( 'NONE',  ( -8.053805599429999518, 1425.213684849519950, 208.0209531150689770 ) ) ;
#7220=CARTESIAN_POINT ( 'NONE',  ( 7.519426757291130414, 1425.430319809400089, 212.2093128352389897 ) ) ;
#7222=VERTEX_POINT ( 'NONE', #91409 ) ;
#7225=CARTESIAN_POINT ( 'NONE',  ( -19.58933252839999994, 1465.550215966989981, 206.2255664879889991 ) ) ;
#7230=EDGE_LOOP ( 'NONE', ( #76055, #38360, #105301, #16877, #105249, #74565 ) ) ;
#7231=CARTESIAN_POINT ( 'NONE',  ( 11.07826983750000061, 1500.667907230989840, 205.8218841770989798 ) ) ;
#7233=CARTESIAN_POINT ( 'NONE',  ( 11.52816659857622383, 1414.661898229710005, 211.3132496073693005 ) ) ;
#7242=CARTESIAN_POINT ( 'NONE',  ( 3.176066407067710262, 1508.610720099250102, 213.8016370287309655 ) ) ;
#7250=CARTESIAN_POINT ( 'NONE',  ( -0.7827245234523669826, 1444.561379792319940, 199.0971546026119938 ) ) ;
#7252=CARTESIAN_POINT ( 'NONE',  ( 13.03846733632719790, 1432.812993616249969, 222.4048857007069842 ) ) ;
#7254=CARTESIAN_POINT ( 'NONE',  ( -10.37371817630540072, 1479.852997517780068, 210.7819975190230082 ) ) ;
#7256=CARTESIAN_POINT ( 'NONE',  ( -2.564245648394030130, 1508.551704408389924, 214.1089243555790063 ) ) ;
#7257=CARTESIAN_POINT ( 'NONE',  ( 11.80702251126379920, 1501.961501625749861, 213.8659162354030059 ) ) ;
#7258=CARTESIAN_POINT ( 'NONE',  ( 7.340164244669999505, 1422.546863311710013, 195.5659725453989779 ) ) ;
#7259=CARTESIAN_POINT ( 'NONE',  ( -1.860813652961599951, 1432.605433200009884, 218.4608168085190130 ) ) ;
#7260=CARTESIAN_POINT ( 'NONE',  ( 10.07826753830500088, 1480.104525031030107, 205.9543300576330012 ) ) ;
#7270=CARTESIAN_POINT ( 'NONE',  ( 5.161034791280000533, 1485.814572579490005, 218.5690567784690188 ) ) ;
#7273=CARTESIAN_POINT ( 'NONE',  ( -15.92986207429999901, 1416.139014782290133, 209.7537124246929920 ) ) ;
#7274=CARTESIAN_POINT ( 'NONE',  ( 11.47825147261290013, 1422.092222879909968, 203.3953002428119987 ) ) ;
#7275=CARTESIAN_POINT ( 'NONE',  ( -10.86989658753349985, 1462.792704963670076, 207.1137526030339870 ) ) ;
#7280=CARTESIAN_POINT ( 'NONE',  ( 6.648507829046476303, 1432.796636465103802, 201.9740417089893185 ) ) ;
#7281=CARTESIAN_POINT ( 'NONE',  ( -9.651319794912328831, 1460.367258809480063, 209.5401502381419903 ) ) ;
#7283=CARTESIAN_POINT ( 'NONE',  ( -16.92750792760880074, 1420.371514553650059, 203.6344363212050155 ) ) ;
#7284=CARTESIAN_POINT ( 'NONE',  ( 11.60899603973430061, 1420.226618356180097, 197.9003279743849930 ) ) ;
#7285=CARTESIAN_POINT ( 'NONE',  ( 7.901747246281610515, 1464.504505592670057, 216.3084624029710028 ) ) ;
#7288=CARTESIAN_POINT ( 'NONE',  ( 3.533737149336580341, 1474.412271694010087, 219.9835368386560219 ) ) ;
#7290=CARTESIAN_POINT ( 'NONE',  ( -8.080362626630025247, 1425.655864844915413, 208.1442273905381910 ) ) ;
#7295=CARTESIAN_POINT ( 'NONE',  ( 12.74442039725110121, 1426.727524945199775, 204.3806995420410146 ) ) ;
#7296=CARTESIAN_POINT ( 'NONE',  ( -8.229021131380180876, 1439.448077257160094, 228.6152060057279982 ) ) ;
#7298=CARTESIAN_POINT ( 'NONE',  ( -16.75443776603389878, 1420.334096955099994, 204.7363179042169747 ) ) ;
#7300=CARTESIAN_POINT ( 'NONE',  ( 7.151487810977736892, 1466.240892066645756, 202.2032590110584067 ) ) ;
#7301=ORIENTED_EDGE ( 'NONE', *, *, #23300, .T. ) ;
#7304=DIRECTION ( 'NONE',  ( 0.9112835967509683721, 0.3049192395332191996, -0.2767425945804181109 ) ) ;
#7308=CARTESIAN_POINT ( 'NONE',  ( -1.726831718310000152, 1484.334257313489843, 198.5613320218990054 ) ) ;
#7310=CARTESIAN_POINT ( 'NONE',  ( 10.17891481550000066, 1479.588126538789766, 206.0283001565290135 ) ) ;
#7313=CARTESIAN_POINT ( 'NONE',  ( -4.834465893738980391, 1433.076913074690083, 216.1502409442880150 ) ) ;
#7321=CARTESIAN_POINT ( 'NONE',  ( 10.46737987522440072, 1424.278786533029916, 206.5800728862719779 ) ) ;
#7327=CARTESIAN_POINT ( 'NONE',  ( 3.883237672519999517, 1472.390963103490094, 218.5418498176989885 ) ) ;
#7335=CARTESIAN_POINT ( 'NONE',  ( 5.972707271129999107, 1446.365007016290065, 202.2403774837590049 ) ) ;
#7338=CARTESIAN_POINT ( 'NONE',  ( -3.205905787939999918, 1454.493866239789895, 199.5427767106090187 ) ) ;
#7341=ORIENTED_EDGE ( 'NONE', *, *, #91494, .F. ) ;
#7347=CARTESIAN_POINT ( 'NONE',  ( -17.45404115237240106, 1417.661807274269904, 206.3269853752529741 ) ) ;
#7363=CARTESIAN_POINT ( 'NONE',  ( 13.84583968663999798, 1499.900157016389812, 227.7510566287420204 ) ) ;
#7372=CARTESIAN_POINT ( 'NONE',  ( -14.15554687228640063, 1508.551704408389924, 210.3501763792300210 ) ) ;
#7373=CARTESIAN_POINT ( 'NONE',  ( 4.045211208830000515, 1515.528099018290050, 210.6101754513790070 ) ) ;
#7385=CIRCLE ( 'NONE', #16307, 15.41143114519999990 ) ;
#7388=DIRECTION ( 'NONE',  ( -0.8907681516580484571, 1.273087901431153894E-31, 0.4544580288560254311 ) ) ;
#7394=CARTESIAN_POINT ( 'NONE',  ( 11.04934308535739973, 1470.239499499950171, 206.9398480105810165 ) ) ;
#7395=CARTESIAN_POINT ( 'NONE',  ( -10.93363683719999813, 1471.692480041690033, 205.6467075678189929 ) ) ;
#7396=CARTESIAN_POINT ( 'NONE',  ( 7.630292994640000437, 1493.382908296590131, 217.4308410871590240 ) ) ;
#7405=DIRECTION ( 'NONE',  ( -1.000000000000000000, 0.000000000000000000, 0.000000000000000000 ) ) ;
#7408=CARTESIAN_POINT ( 'NONE',  ( 5.416019587700000137, 1505.806237347190063, 219.5704354396989970 ) ) ;
#7411=ORIENTED_EDGE ( 'NONE', *, *, #85629, .F. ) ;
#7412=CARTESIAN_POINT ( 'NONE',  ( -15.60757908461217269, 1415.701611827778834, 209.6322609307934499 ) ) ;
#7413=CARTESIAN_POINT ( 'NONE',  ( -1.561170263100000177, 1508.551704408389924, 220.0946958077990132 ) ) ;
#7415=CARTESIAN_POINT ( 'NONE',  ( -15.64577121609999821, 1415.699210022930174, 209.5376526706779998 ) ) ;
#7416=CARTESIAN_POINT ( 'NONE',  ( -7.332216129953320838, 1441.976895380970063, 202.1891949145530134 ) ) ;
#7418=FACE_OUTER_BOUND ( 'NONE', #13238, .T. ) ;
#7421=CARTESIAN_POINT ( 'NONE',  ( -15.05898902610000079, 1503.430790790689798, 209.1800621844290049 ) ) ;
#7429=LINE ( 'NONE', #85226, #80320 ) ;
#7430=CARTESIAN_POINT ( 'NONE',  ( 2.713367651848939577, 1454.423712428280169, 218.1168998963650267 ) ) ;
#7434=CARTESIAN_POINT ( 'NONE',  ( -14.83256633360000087, 1416.408364792800057, 204.9070730081490126 ) ) ;
#7437=CARTESIAN_POINT ( 'NONE',  ( -3.556250521940888198, 1497.014257045862678, 220.2466743886169240 ) ) ;
#7438=CARTESIAN_POINT ( 'NONE',  ( -16.55781857232240384, 1419.635042661685247, 209.2150186604269209 ) ) ;
#7439=CARTESIAN_POINT ( 'NONE',  ( -4.351525890989999645, 1495.862468678689993, 219.4621222446990316 ) ) ;
#7443=CARTESIAN_POINT ( 'NONE',  ( -14.20981385350011017, 1419.004818489330546, 200.1611769720297502 ) ) ;
#7446=FACE_OUTER_BOUND ( 'NONE', #29816, .T. ) ;
#7453=CARTESIAN_POINT ( 'NONE',  ( 7.480280153066277471, 1471.188496245784791, 215.9764434431355085 ) ) ;
#7459=CARTESIAN_POINT ( 'NONE',  ( 11.42820171992390144, 1478.773761690850051, 206.4058094161790109 ) ) ;
#7461=CARTESIAN_POINT ( 'NONE',  ( -8.548024229050710687, 1437.883693539470187, 228.3934038729859708 ) ) ;
#7463=CARTESIAN_POINT ( 'NONE',  ( -17.65533443933999891, 1419.497285706960156, 207.2321711664930035 ) ) ;
#7464=CARTESIAN_POINT ( 'NONE',  ( -16.12185590881189867, 1416.489668067350067, 209.3435334434090009 ) ) ;
#7466=CARTESIAN_POINT ( 'NONE',  ( -4.992349863779999453, 1391.620913471789891, 203.8075142969990168 ) ) ;
#7469=CARTESIAN_POINT ( 'NONE',  ( 9.922759194041839592, 1450.941995602500128, 205.8041822776330037 ) ) ;
#7484=ORIENTED_EDGE ( 'NONE', *, *, #54478, .T. ) ;
#7488=CARTESIAN_POINT ( 'NONE',  ( -0.3986462593559989553, 1443.308886971090260, 200.2051758347389807 ) ) ;
#7493=CARTESIAN_POINT ( 'NONE',  ( 0.9889191132270008788, 1418.023982291090078, 204.0456544364789977 ) ) ;
#7495=CARTESIAN_POINT ( 'NONE',  ( 4.329448776274299249, 1515.064792882709980, 211.4519800890089982 ) ) ;
#7499=ORIENTED_EDGE ( 'NONE', *, *, #98330, .F. ) ;
#7509=CARTESIAN_POINT ( 'NONE',  ( -12.08541892319999889, 1503.227962273290132, 208.3926044072909747 ) ) ;
#7521=EDGE_CURVE ( 'NONE', #82285, #43603, #44875, .T. ) ;
#7538=DIRECTION ( 'NONE',  ( -1.000000000000000000, 0.000000000000000000, 0.000000000000000000 ) ) ;
#7553=CARTESIAN_POINT ( 'NONE',  ( -9.156505819859109607, 1449.262359179090026, 209.6968860301970210 ) ) ;
#7575=CARTESIAN_POINT ( 'NONE',  ( 5.234983244518070400, 1455.659623156430143, 218.3679346420140064 ) ) ;
#7576=CARTESIAN_POINT ( 'NONE',  ( 642.7360634221799955, 11220.04953453920098, 2085.137448048184979 ) ) ;
#7580=CARTESIAN_POINT ( 'NONE',  ( -9.030488842750038714, 1438.110210707299984, 210.2927785181310014 ) ) ;
#7581=CARTESIAN_POINT ( 'NONE',  ( -2.329898843064519998, 1515.219291385629958, 213.4472495155459910 ) ) ;
#7587=VERTEX_POINT ( 'NONE', #101843 ) ;
#7592=CARTESIAN_POINT ( 'NONE',  ( -3.300826323869999968, 1500.561897259590069, 230.1976133252990167 ) ) ;
#7594=CARTESIAN_POINT ( 'NONE',  ( 1.878980900259999975, 1455.587583919590088, 218.5151519414690142 ) ) ;
#7596=CARTESIAN_POINT ( 'NONE',  ( -7.374483111930000057, 1447.147829244589957, 214.6826825380690025 ) ) ;
#7601=CARTESIAN_POINT ( 'NONE',  ( 7.224319591869999613, 1424.601783486629984, 212.7752974582190291 ) ) ;
#7620=CARTESIAN_POINT ( 'NONE',  ( -9.409898537430208876, 1446.992683627339829, 212.1329179144990178 ) ) ;
#7624=CARTESIAN_POINT ( 'NONE',  ( -4.327230971739010279, 1515.149487411890050, 209.5135165373189921 ) ) ;
#7628=CARTESIAN_POINT ( 'NONE',  ( 9.651063919191019025, 1425.440657924460083, 195.4941620015079877 ) ) ;
#7630=CARTESIAN_POINT ( 'NONE',  ( 0.1315954949189999945, 1432.375264448149892, 200.6910518521459892 ) ) ;
#7635=ADVANCED_FACE ( 'NONE', ( #107115 ), #7859, .T. ) ;
#7637=EDGE_CURVE ( 'NONE', #104222, #32267, #106325, .T. ) ;
#7641=EDGE_CURVE ( 'NONE', #69447, #63442, #51603, .T. ) ;
#7650=EDGE_CURVE ( 'NONE', #35149, #2466, #36912, .T. ) ;
#7657=FACE_OUTER_BOUND ( 'NONE', #70071, .T. ) ;
#7662=CARTESIAN_POINT ( 'NONE',  ( -8.825147375033820296, 1438.586940765240115, 208.4641837083139819 ) ) ;
#7663=EDGE_CURVE ( 'NONE', #10365, #32988, #103765, .T. ) ;
#7665=EDGE_LOOP ( 'NONE', ( #61933, #6659, #56431, #22841 ) ) ;
#7666=FACE_OUTER_BOUND ( 'NONE', #38525, .T. ) ;
#7670=CARTESIAN_POINT ( 'NONE',  ( -14.96473955119999921, 1416.430699836160102, 207.9564624935089796 ) ) ;
#7672=CARTESIAN_POINT ( 'NONE',  ( 3.965821128770000481, 1486.919029566390009, 198.6437641315989993 ) ) ;
#7674=CARTESIAN_POINT ( 'NONE',  ( 1.468816372564279993, 1431.317999364719981, 218.4991881548640151 ) ) ;
#7682=CARTESIAN_POINT ( 'NONE',  ( -16.99051315430000386, 1420.323703249610162, 203.8408267910690199 ) ) ;
#7683=EDGE_CURVE ( 'NONE', #61362, #88484, #60942, .T. ) ;
#7685=CARTESIAN_POINT ( 'NONE',  ( 0.6307243961899989815, 1474.949842634390052, 220.1414127045989915 ) ) ;
#7694=CARTESIAN_POINT ( 'NONE',  ( -7.015951070247499644, 1421.061870212209897, 194.1995972353730053 ) ) ;
#7701=DIRECTION ( 'NONE',  ( 1.158258077154680071E-09, -1.836970198721029688E-16, -1.000000000000000000 ) ) ;
#7705=EDGE_CURVE ( 'NONE', #21410, #10141, #52835, .T. ) ;
#7710=ADVANCED_FACE ( 'NONE', ( #4531 ), #40008, .F. ) ;
#7711=CARTESIAN_POINT ( 'NONE',  ( 10.01013843233299916, 1469.369181467840008, 209.9819040969830155 ) ) ;
#7712=CARTESIAN_POINT ( 'NONE',  ( 11.86092065826349895, 1492.895007130480053, 212.5849778500719935 ) ) ;
#7713=CARTESIAN_POINT ( 'NONE',  ( 1.776582264570000014, 1456.341121776589716, 219.1753798333990062 ) ) ;
#7717=CARTESIAN_POINT ( 'NONE',  ( 8.062587302181759341, 1436.235894220949831, 206.1282943059349861 ) ) ;
#7725=CARTESIAN_POINT ( 'NONE',  ( 11.55221588404359956, 1480.217597516799970, 211.4789165460060190 ) ) ;
#7727=EDGE_CURVE ( 'NONE', #18777, #102315, #26187, .T. ) ;
#7730=CARTESIAN_POINT ( 'NONE',  ( -15.66330071820020287, 1508.551704408389924, 214.2112499943270052 ) ) ;
#7731=CARTESIAN_POINT ( 'NONE',  ( -1.240189040380000218, 1457.347231108689812, 202.3619262432189885 ) ) ;
#7734=CARTESIAN_POINT ( 'NONE',  ( 6.343729916319600370, 1432.997535027899858, 202.2534603803919993 ) ) ;
#7736=B_SPLINE_CURVE_WITH_KNOTS ( 'NONE', 3,
 ( #63392, #97507, #38689, #5089, #20776, #39242, #54977, #12390, #38145, #59384 ),
 .UNSPECIFIED., .F., .F.,
 ( 4, 3, 3, 4 ),
 ( -12.93235455439439896, -12.28324979274049866, -11.03322287909449884, -9.791994790430690543 ),
 .UNSPECIFIED. ) ;
#7739=CARTESIAN_POINT ( 'NONE',  ( -20.40768745807410056, 1466.146701207289880, 211.1092863667410029 ) ) ;
#7744=EDGE_CURVE ( 'NONE', #45421, #75670, #4778, .T. ) ;
#7747=CARTESIAN_POINT ( 'NONE',  ( -13.13536861894177576, 1507.686078928800043, 209.3105439034022197 ) ) ;
#7748=CARTESIAN_POINT ( 'NONE',  ( -2.851018948600000158, 1476.884648983389980, 199.1362811694189929 ) ) ;
#7755=CARTESIAN_POINT ( 'NONE',  ( -8.082242560709998358, 1425.089483080600075, 208.3127043135090162 ) ) ;
#7759=CARTESIAN_POINT ( 'NONE',  ( 7.513965249524710011, 1425.915627064070122, 212.2777243754379981 ) ) ;
#7765=EDGE_CURVE ( 'NONE', #109440, #5037, #65514, .T. ) ;
#7768=CARTESIAN_POINT ( 'NONE',  ( 8.454790733525280544, 1428.363638633589972, 213.4109935021670026 ) ) ;
#7781=CARTESIAN_POINT ( 'NONE',  ( -5.062155874537689115, 1439.003721114779864, 206.7420737057830138 ) ) ;
#7795=FACE_OUTER_BOUND ( 'NONE', #48962, .T. ) ;
#7797=CARTESIAN_POINT ( 'NONE',  ( -3.780333225011479836, 1508.551704408389924, 213.7482560551979986 ) ) ;
#7798=CARTESIAN_POINT ( 'NONE',  ( 12.33991424210799970, 1501.419616770270068, 212.2020435037020150 ) ) ;
#7799=CARTESIAN_POINT ( 'NONE',  ( 8.135441375949998388, 1421.256651981180084, 196.0379973919989709 ) ) ;
#7802=CARTESIAN_POINT ( 'NONE',  ( -4.867399450039999742, 1495.075882605090101, 197.7983437550990118 ) ) ;
#7808=ADVANCED_FACE ( 'NONE', ( #109605 ), #23912, .T. ) ;
#7813=CARTESIAN_POINT ( 'NONE',  ( -10.45913315801519872, 1483.337912596790147, 203.4298690767190010 ) ) ;
#7816=CARTESIAN_POINT ( 'NONE',  ( 11.85965305928869995, 1425.934783538740021, 202.8481194454130048 ) ) ;
#7817=CARTESIAN_POINT ( 'NONE',  ( -11.03352341481849841, 1462.446812322350070, 208.7213867630900097 ) ) ;
#7819=CARTESIAN_POINT ( 'NONE',  ( -10.37617513879240150, 1479.403831811299824, 210.6295454707710064 ) ) ;
#7823=CARTESIAN_POINT ( 'NONE',  ( -17.54341085149529889, 1417.941250412889985, 206.8706738254780078 ) ) ;
#7824=CARTESIAN_POINT ( 'NONE',  ( 12.90319585266200164, 1420.986560144630175, 203.4264861624149887 ) ) ;
#7826=CARTESIAN_POINT ( 'NONE',  ( 8.179457570200950656, 1464.307649058119978, 216.6184750703820043 ) ) ;
#7832=CARTESIAN_POINT ( 'NONE',  ( 0.5996034049719994874, 1477.819945573845416, 198.7231221488051744 ) ) ;
#7837=CARTESIAN_POINT ( 'NONE',  ( -17.55008883411199960, 1487.029577352629758, 194.9701233786059902 ) ) ;
#7839=CARTESIAN_POINT ( 'NONE',  ( -22.46469623289999618, 1417.574324945069975, 209.9387869133350080 ) ) ;
#7844=DIRECTION ( 'NONE',  ( -1.156023075842281927E-31, 1.000000000000000000, -1.698192320643030073E-16 ) ) ;
#7852=CARTESIAN_POINT ( 'NONE',  ( 7.835755939781712698, 1447.918173471444334, 204.3989379467183198 ) ) ;
#7855=CARTESIAN_POINT ( 'NONE',  ( -8.284402606713660688, 1436.555342802109863, 212.1856797791610063 ) ) ;
#7856=CARTESIAN_POINT ( 'NONE',  ( -15.70179666829999832, 1415.698136594249945, 210.0629521891549985 ) ) ;
#7859=B_SPLINE_SURFACE_WITH_KNOTS ( 'NONE', 5, 1, ( 
 ( #89218, #38254 ),
 ( #98713, #21430 ),
 ( #4129, #56165 ),
 ( #64041, #55642 ),
 ( #89763, #13034 ),
 ( #106031, #97079 ) ),
 .UNSPECIFIED., .F., .F., .F.,
 ( 6, 6 ),
 ( 2, 2 ),
 ( 3.552713678800000397E-15, 14.76708736389999999 ),
 ( 0.000000000000000000, 14.00000000000000000 ),
 .UNSPECIFIED. ) ;
#7863=CARTESIAN_POINT ( 'NONE',  ( 10.54782078997249961, 1426.750615647500126, 208.6717185375519819 ) ) ;
#7864=ORIENTED_EDGE ( 'NONE', *, *, #109531, .T. ) ;
#7867=CARTESIAN_POINT ( 'NONE',  ( 3.346707516019999940, 1443.005054410889898, 217.3642451189890323 ) ) ;
#7869=CARTESIAN_POINT ( 'NONE',  ( 2.252978874640000129, 1474.529339387290065, 219.9022295252989920 ) ) ;
#7876=CARTESIAN_POINT ( 'NONE',  ( 9.709932644140000235, 1450.584296204089924, 205.0446109545989941 ) ) ;
#7879=CARTESIAN_POINT ( 'NONE',  ( -10.22078022364619976, 1448.827725899079724, 207.2905427559460065 ) ) ;
#7883=FACE_OUTER_BOUND ( 'NONE', #6114, .T. ) ;
#7888=ORIENTED_EDGE ( 'NONE', *, *, #110593, .T. ) ;
#7902=CARTESIAN_POINT ( 'NONE',  ( 2.674013553562669898, 1508.551704408389924, 214.1019878693419969 ) ) ;
#7905=CARTESIAN_POINT ( 'NONE',  ( -21.26810766760000249, 1485.919195121089842, 201.7808564926190229 ) ) ;
#7911=CARTESIAN_POINT ( 'NONE',  ( 10.36757158123830003, 1453.224707006280141, 211.3662413356020124 ) ) ;
#7913=CARTESIAN_POINT ( 'NONE',  ( -12.37112953626025735, 1417.358968133092048, 199.9426545053605651 ) ) ;
#7914=CARTESIAN_POINT ( 'NONE',  ( 4.324092172210000307, 1515.269353063089966, 209.4835653193450185 ) ) ;
#7916=CARTESIAN_POINT ( 'NONE',  ( -4.933290692019969725, 1455.123182729209930, 201.0873875226590144 ) ) ;
#7917=ADVANCED_FACE ( 'NONE', ( #26124 ), #14964, .T. ) ;
#7920=B_SPLINE_SURFACE_WITH_KNOTS ( 'NONE', 5, 5, ( 
 ( #51803, #85371, #69164, #95453, #26009, #67511 ),
 ( #110590, #312, #102180, #101614, #103268, #26577 ),
 ( #60206, #50689, #93233, #18718, #33876, #87046 ),
 ( #52370, #69731, #34984, #77554, #10334, #68612 ),
 ( #52914, #110043, #77006, #9785, #16500, #17603 ),
 ( #86490, #8120, #85944, #24901, #94325, #18173 ),
 ( #44506, #9245, #76437, #60774, #42287, #857 ),
 ( #68068, #43951, #33316, #25460, #94899, #61334 ),
 ( #59655, #78094, #1396, #27149, #93763, #17041 ) ),
 .UNSPECIFIED., .F., .F., .F.,
 ( 6, 3, 6 ),
 ( 6, 6 ),
 ( 3.257013150990000216, 5.599849328569999507, 7.942685506149999242 ),
 ( 0.000000000000000000, 2.000000000000000000 ),
 .UNSPECIFIED. ) ;
#7928=CARTESIAN_POINT ( 'NONE',  ( 19.32263322520000060, 1455.378559704889767, 209.1218459616989946 ) ) ;
#7929=B_SPLINE_CURVE_WITH_KNOTS ( 'NONE', 5,
 ( #110661, #52989, #87122, #59187, #18243, #95523, #94975, #33954, #59728 ),
 .UNSPECIFIED., .F., .F.,
 ( 6, 3, 6 ),
 ( 0.000000000000000000, 0.3844850474641056115, 1.000000000000000000 ),
 .UNSPECIFIED. ) ;
#7931=ORIENTED_EDGE ( 'NONE', *, *, #70625, .T. ) ;
#7934=CARTESIAN_POINT ( 'NONE',  ( -17.24773937279860192, 1420.120834743239811, 204.7828160326650107 ) ) ;
#7935=CARTESIAN_POINT ( 'NONE',  ( -9.851064782010787724, 1490.933270807075132, 214.0922473749026267 ) ) ;
#7940=CARTESIAN_POINT ( 'NONE',  ( -10.46250751532009993, 1491.356802638789986, 212.5409670664860187 ) ) ;
#7943=CARTESIAN_POINT ( 'NONE',  ( -3.807470111109999777, 1497.262881795189742, 198.5198641202990189 ) ) ;
#7944=CARTESIAN_POINT ( 'NONE',  ( 2.487935142314050108, 1509.038615934839981, 213.6090957367470082 ) ) ;
#7948=EDGE_LOOP ( 'NONE', ( #80381, #71777, #45644, #14878 ) ) ;
#7955=TOROIDAL_SURFACE ( 'NONE', #68811, 3.250000000000000000, 0.5000000000000000000 ) ;
#7959=CARTESIAN_POINT ( 'NONE',  ( -0.9720884905540009280, 1508.551704159290011, 220.3304486672990095 ) ) ;
#7964=CARTESIAN_POINT ( 'NONE',  ( 21.06331657220000153, 1496.634916824290030, 207.0954909778190256 ) ) ;
#7965=CARTESIAN_POINT ( 'NONE',  ( 18.54783228039999798, 1474.422996780290077, 200.1179429635390079 ) ) ;
#7967=CARTESIAN_POINT ( 'NONE',  ( -10.78800201790000024, 1480.681111995489800, 211.1294777214090175 ) ) ;
#7972=B_SPLINE_SURFACE_WITH_KNOTS ( 'NONE', 5, 1, ( 
 ( #38084, #106391 ),
 ( #29675, #30777 ),
 ( #21242, #55455 ),
 ( #89581, #12874 ),
 ( #47053, #60418 ),
 ( #7781, #93989 ) ),
 .UNSPECIFIED., .F., .F., .F.,
 ( 6, 6 ),
 ( 2, 2 ),
 ( -2.253879340347439943E-05, 15.90092593249339892 ),
 ( 0.000000000000000000, 14.00002253879340053 ),
 .UNSPECIFIED. ) ;
#7979=CARTESIAN_POINT ( 'NONE',  ( -15.44336791849999990, 1417.906189380320029, 203.8647015642989970 ) ) ;
#7980=B_SPLINE_CURVE_WITH_KNOTS ( 'NONE', 5,
 ( #70681, #88016, #3459, #28637, #6048, #104794 ),
 .UNSPECIFIED., .F., .F.,
 ( 6, 6 ),
 ( 0.000000000000000000, 1.000000000000000000 ),
 .UNSPECIFIED. ) ;
#7983=CARTESIAN_POINT ( 'NONE',  ( -8.601854796231091171, 1436.861797634760023, 209.7917467578280082 ) ) ;
#7984=CARTESIAN_POINT ( 'NONE',  ( -4.234183914609999988, 1496.289481068690066, 219.5317350564990022 ) ) ;
#7988=CARTESIAN_POINT ( 'NONE',  ( -11.14967447845340054, 1508.551708988489963, 208.5621525772319842 ) ) ;
#7995=CARTESIAN_POINT ( 'NONE',  ( -3.152270363119999974, 1474.954422145789977, 198.1306181043989909 ) ) ;
#8000=CARTESIAN_POINT ( 'NONE',  ( -15.85591190879999779, 1415.880081504350073, 209.4912631162540038 ) ) ;
#8004=CARTESIAN_POINT ( 'NONE',  ( 4.702020435729999726, 1486.019901504789914, 218.8180113132190172 ) ) ;
#8005=CARTESIAN_POINT ( 'NONE',  ( 10.35218644306529967, 1480.376106472589981, 207.1666581537910190 ) ) ;
#8008=CARTESIAN_POINT ( 'NONE',  ( -8.109401236050000961, 1440.034690421490041, 228.6983774484990022 ) ) ;
#8051=CARTESIAN_POINT ( 'NONE',  ( -8.343905337393612953, 1474.683381955320783, 203.1186823195534146 ) ) ;
#8061=CARTESIAN_POINT ( 'NONE',  ( -2.330134126090000368, 1515.064792882589927, 204.7923971856590128 ) ) ;
#8069=CARTESIAN_POINT ( 'NONE',  ( 4.253777714910000007, 1442.471859903390168, 216.9083338397390150 ) ) ;
#8074=CARTESIAN_POINT ( 'NONE',  ( -3.738592038228889969, 1428.502628658499816, 200.5405866258459753 ) ) ;
#8078=AXIS2_PLACEMENT_3D ( 'NONE', #87900, #59943, #35267 ) ;
#8084=VERTEX_POINT ( 'NONE', #12100 ) ;
#8086=B_SPLINE_SURFACE_WITH_KNOTS ( 'NONE', 5, 5, ( 
 ( #73398, #30825, #65000, #99118, #82884, #109742, #17300, #102431, #50411 ),
 ( #69427, #101871, #33565, #76144, #33024, #24602, #59916, #68323, #17861 ),
 ( #16746, #41447, #67213, #34685, #8369, #68876, #560, #101309, #7284 ),
 ( #85627, #42538, #18413, #34137, #102977, #95154, #8928, #103541, #25714 ),
 ( #94036, #75612, #51495, #9485, #110289, #77261, #52611, #58796, #93476 ),
 ( #50953, #60464, #92936, #43650, #16207, #43101, #52060, #84536, #7824 ) ),
 .UNSPECIFIED., .F., .F., .F.,
 ( 6, 6 ),
 ( 6, 3, 6 ),
 ( 8.238698527393529147, 19.77813405259999868 ),
 ( -8.198479471770259521E-05, 1.500000000000000000, 3.003699267706470000 ),
 .UNSPECIFIED. ) ;
#8089=CARTESIAN_POINT ( 'NONE',  ( -0.6331911303215019826, 1494.577966063601252, 220.2613815778443893 ) ) ;
#8094=CARTESIAN_POINT ( 'NONE',  ( -9.103435472426211206, 1449.500063809829953, 210.3012238382719943 ) ) ;
#8096=EDGE_LOOP ( 'NONE', ( #35184, #91254, #33714, #76928 ) ) ;
#8120=CARTESIAN_POINT ( 'NONE',  ( 11.42883607589999961, 1502.384062944689958, 210.3441498915189811 ) ) ;
#8123=CARTESIAN_POINT ( 'NONE',  ( 7.254058142540000809, 1424.158195616359990, 212.5403795493589882 ) ) ;
#8124=CARTESIAN_POINT ( 'NONE',  ( -4.329448802513499395, 1515.064791340959800, 211.4517443289939820 ) ) ;
#8127=CARTESIAN_POINT ( 'NONE',  ( -6.103113815119999508, 1482.731685980090106, 200.3426744219489990 ) ) ;
#8135=CARTESIAN_POINT ( 'NONE',  ( -1.017068913289999932, 1494.761373610690043, 217.4896306674490063 ) ) ;
#8137=CARTESIAN_POINT ( 'NONE',  ( 1.875671966999999940, 1456.514202392889956, 219.5762891471990201 ) ) ;
#8139=CARTESIAN_POINT ( 'NONE',  ( -5.213813250899999474, 1445.091437330390136, 217.1001509711090023 ) ) ;
#8143=CARTESIAN_POINT ( 'NONE',  ( 7.103763521679999471, 1424.020716665080045, 213.1883901192190081 ) ) ;
#8145=CARTESIAN_POINT ( 'NONE',  ( -4.017758734575580526, 1453.901170738600058, 199.4485904977269684 ) ) ;
#8146=CARTESIAN_POINT ( 'NONE',  ( 1.702416261868870073, 1493.957958506549858, 220.1113518634800243 ) ) ;
#8150=EDGE_LOOP ( 'NONE', ( #18826, #78483, #60221, #9433 ) ) ;
#8162=CARTESIAN_POINT ( 'NONE',  ( -9.105453163054910704, 1449.059532022529993, 210.1349288613230044 ) ) ;
#8171=CARTESIAN_POINT ( 'NONE',  ( 6.960583431767130236, 1424.680772738690166, 193.9777372977509913 ) ) ;
#8174=CARTESIAN_POINT ( 'NONE',  ( 0.000000000000000000, 1420.119835273649869, 209.1218459616989946 ) ) ;
#8186=CARTESIAN_POINT ( 'NONE',  ( -4.646147438016499542, 1378.399971910029990, 214.5514622210689879 ) ) ;
#8188=CARTESIAN_POINT ( 'NONE',  ( 12.26470395605226571, 1426.140792135694483, 200.3478462435150504 ) ) ;
#8191=CARTESIAN_POINT ( 'NONE',  ( -11.60387536552270049, 1481.105535834539978, 211.4044418330699955 ) ) ;
#8196=CARTESIAN_POINT ( 'NONE',  ( 7.227136201815060446, 1482.982132909030042, 211.7482587894230051 ) ) ;
#8204=CARTESIAN_POINT ( 'NONE',  ( -12.02051106306990036, 1491.153688555679992, 206.6632162730240054 ) ) ;
#8208=CARTESIAN_POINT ( 'NONE',  ( -17.06814468720000377, 1418.145817546499984, 204.3351068018390038 ) ) ;
#8210=CARTESIAN_POINT ( 'NONE',  ( 10.20885384580000022, 1489.898602996290037, 203.1012352018590263 ) ) ;
#8215=CARTESIAN_POINT ( 'NONE',  ( -1.842963333050206209, 1515.193466796482426, 204.7957666306796796 ) ) ;
#8220=CARTESIAN_POINT ( 'NONE',  ( -16.83270678099999884, 1420.441345669400107, 203.3485545991589731 ) ) ;
#8221=ORIENTED_EDGE ( 'NONE', *, *, #30760, .T. ) ;
#8222=CARTESIAN_POINT ( 'NONE',  ( -18.39846574424100112, 1508.551704408389924, 210.4158962701780240 ) ) ;
#8226=CARTESIAN_POINT ( 'NONE',  ( -11.40193393769130026, 1470.847406381370092, 208.7670122399519812 ) ) ;
#8227=CARTESIAN_POINT ( 'NONE',  ( -7.280829216295649609, 1508.396933602414720, 219.6675365539373388 ) ) ;
#8230=CARTESIAN_POINT ( 'NONE',  ( -8.340003444863377524, 1458.803746027120042, 213.9233038274046237 ) ) ;
#8233=CARTESIAN_POINT ( 'NONE',  ( -11.38244087966499940, 1470.612899495130023, 209.7950405083470002 ) ) ;
#8236=ORIENTED_EDGE ( 'NONE', *, *, #13923, .T. ) ;
#8243=LINE ( 'NONE', #74390, #53842 ) ;
#8244=CARTESIAN_POINT ( 'NONE',  ( -4.636368232763167008, 1378.015684711496988, 203.9444611951153377 ) ) ;
#8246=CARTESIAN_POINT ( 'NONE',  ( 19.03958390842529980, 1453.804148033969796, 200.7927771423659919 ) ) ;
#8248=ADVANCED_FACE ( 'NONE', ( #4269 ), #40913, .T. ) ;
#8252=CARTESIAN_POINT ( 'NONE',  ( 12.31939201916519977, 1492.268456928650039, 209.8911822630940094 ) ) ;
#8253=CARTESIAN_POINT ( 'NONE',  ( 0.6519600591489990160, 1456.622952327490111, 219.3373220789989944 ) ) ;
#8260=VERTEX_POINT ( 'NONE', #91572 ) ;
#8261=EDGE_CURVE ( 'NONE', #105125, #43735, #18050, .T. ) ;
#8267=CARTESIAN_POINT ( 'NONE',  ( 11.55681713461770066, 1480.209600850990000, 211.4560790503059877 ) ) ;
#8271=CARTESIAN_POINT ( 'NONE',  ( -10.52263122030180043, 1508.551704408389924, 218.0322449975469681 ) ) ;
#8274=FACE_OUTER_BOUND ( 'NONE', #53660, .T. ) ;
#8281=CARTESIAN_POINT ( 'NONE',  ( -3.130661101029999838, 1471.246791520290117, 187.3882170434989973 ) ) ;
#8291=CARTESIAN_POINT ( 'NONE',  ( -0.9759527017809989102, 1477.437381222690192, 198.7358441459990104 ) ) ;
#8297=CARTESIAN_POINT ( 'NONE',  ( 1.833097954248699812, 1429.276494549819972, 217.2158816865839981 ) ) ;
#8298=CARTESIAN_POINT ( 'NONE',  ( -2.048534905309999932, 1444.110401950890036, 199.2775038477390126 ) ) ;
#8303=CARTESIAN_POINT ( 'NONE',  ( -9.699660872752350116, 1472.030908259890111, 212.1562907213800031 ) ) ;
#8304=CARTESIAN_POINT ( 'NONE',  ( 7.520380367349810413, 1425.880113479670172, 212.2583774670760022 ) ) ;
#8311=B_SPLINE_CURVE_WITH_KNOTS ( 'NONE', 5,
 ( #17192, #58151, #16645, #24508, #32919, #110187 ),
 .UNSPECIFIED., .F., .F.,
 ( 6, 6 ),
 ( 265.9669962020000185, 275.7680412249999904 ),
 .UNSPECIFIED. ) ;
#8312=FACE_OUTER_BOUND ( 'NONE', #106646, .T. ) ;
#8314=CARTESIAN_POINT ( 'NONE',  ( 3.892080479029999651, 1421.098424262469962, 205.7437050486190060 ) ) ;
#8320=CARTESIAN_POINT ( 'NONE',  ( 8.197348291215568850, 1436.381065636019912, 206.4883948098359951 ) ) ;
#8328=CARTESIAN_POINT ( 'NONE',  ( 3.117403407738490007, 1508.880976867409800, 213.6144879028050241 ) ) ;
#8335=CARTESIAN_POINT ( 'NONE',  ( 0.6746223769683330485, 1445.135766336949928, 199.0746255971319840 ) ) ;
#8338=CARTESIAN_POINT ( 'NONE',  ( -11.16939613673820020, 1480.956201967079778, 211.2843442006090129 ) ) ;
#8339=CARTESIAN_POINT ( 'NONE',  ( 5.401943384969776218, 1434.552886126495196, 202.5243240070273032 ) ) ;
#8340=CARTESIAN_POINT ( 'NONE',  ( 2.487935123032369855, 1509.038615930399828, 204.6345961886270004 ) ) ;
#8342=CARTESIAN_POINT ( 'NONE',  ( 7.417144106380000323, 1422.547346766210012, 195.6244150781990072 ) ) ;
#8344=CARTESIAN_POINT ( 'NONE',  ( -3.801318561300000010, 1497.265417599789998, 198.5158051468989981 ) ) ;
#8356=CARTESIAN_POINT ( 'NONE',  ( -10.94871860470700042, 1483.088542335439797, 204.4306030440669986 ) ) ;
#8360=CARTESIAN_POINT ( 'NONE',  ( -11.03223536238590086, 1462.458870289319975, 208.6692969917750133 ) ) ;
#8369=CARTESIAN_POINT ( 'NONE',  ( 9.555970081965631024, 1422.926917982770192, 198.6394148135399860 ) ) ;
#8370=CARTESIAN_POINT ( 'NONE',  ( 9.559796994581459373, 1464.142862108780264, 211.4021333761209860 ) ) ;
#8374=B_SPLINE_CURVE_WITH_KNOTS ( 'NONE', 3,
 ( #14974, #7150, #40746, #57575, #100637, #13870 ),
 .UNSPECIFIED., .F., .F.,
 ( 4, 2, 4 ),
 ( 0.000000000000000000, 0.5000000000000000000, 1.000000000000000000 ),
 .UNSPECIFIED. ) ;
#8375=CARTESIAN_POINT ( 'NONE',  ( -8.044681560367203943, 1424.920053392873342, 210.1656137535678397 ) ) ;
#8377=CARTESIAN_POINT ( 'NONE',  ( 2.752776352959999784, 1478.720949088489988, 229.3133615295990069 ) ) ;
#8382=CARTESIAN_POINT ( 'NONE',  ( 10.59813984854799962, 1477.524079690600047, 229.9254213654089938 ) ) ;
#8384=CARTESIAN_POINT ( 'NONE',  ( -21.93836957199999915, 1417.787473855720009, 209.9936763310599872 ) ) ;
#8389=CARTESIAN_POINT ( 'NONE',  ( -16.65376764594610037, 1508.454796205149933, 213.7212175226700026 ) ) ;
#8393=ORIENTED_EDGE ( 'NONE', *, *, #55867, .T. ) ;
#8395=CARTESIAN_POINT ( 'NONE',  ( 9.664166848750001648, 1480.267612727490132, 204.8064600242389872 ) ) ;
#8397=CARTESIAN_POINT ( 'NONE',  ( 9.520297885996999554, 1500.537487524489961, 228.7174115261980205 ) ) ;
#8398=CARTESIAN_POINT ( 'NONE',  ( -8.242357959885127983, 1435.730723328530075, 211.7688826979850205 ) ) ;
#8400=CARTESIAN_POINT ( 'NONE',  ( -15.16741077070000188, 1418.509014818010201, 212.0774864640089845 ) ) ;
#8405=CARTESIAN_POINT ( 'NONE',  ( 10.54001418240659937, 1422.676165995590054, 209.0262571849499977 ) ) ;
#8412=CARTESIAN_POINT ( 'NONE',  ( 2.356071275890000205, 1473.765556327289914, 219.2284513104989685 ) ) ;
#8415=CARTESIAN_POINT ( 'NONE',  ( -9.086012908930001686, 1493.639819928789848, 201.8509011471290080 ) ) ;
#8420=CARTESIAN_POINT ( 'NONE',  ( 9.005061041439999414, 1450.163101882289993, 205.4957679819289922 ) ) ;
#8421=CARTESIAN_POINT ( 'NONE',  ( -8.603573955260001682, 1512.656901503689824, 210.4681710982189884 ) ) ;
#8430=CARTESIAN_POINT ( 'NONE',  ( -1.982554037259999902, 1496.032958330690008, 196.9258813337989977 ) ) ;
#8431=CARTESIAN_POINT ( 'NONE',  ( 1.157103504880000022, 1494.548177158689896, 220.2271105453990003 ) ) ;
#8446=CARTESIAN_POINT ( 'NONE',  ( 2.487935084889999704, 1508.551704408389924, 214.1089244042930204 ) ) ;
#8455=FACE_OUTER_BOUND ( 'NONE', #84829, .T. ) ;
#8456=CARTESIAN_POINT ( 'NONE',  ( 8.813958094369999330, 1425.194329715850017, 194.9377351523990001 ) ) ;
#8458=CARTESIAN_POINT ( 'NONE',  ( -13.21112480721102500, 1416.964352618932935, 201.1890931735370032 ) ) ;
#8459=CARTESIAN_POINT ( 'NONE',  ( 4.329448776040000446, 1515.064792882589927, 210.5737005773590056 ) ) ;
#8464=CARTESIAN_POINT ( 'NONE',  ( 9.346483001066818730, 1451.068298621479926, 208.1598608262460175 ) ) ;
#8470=ORIENTED_EDGE ( 'NONE', *, *, #28567, .F. ) ;
#8477=CARTESIAN_POINT ( 'NONE',  ( -10.13499527144800005, 1462.137798843650216, 208.1879751690069895 ) ) ;
#8480=CARTESIAN_POINT ( 'NONE',  ( 10.01091973119789991, 1469.175247106300048, 207.4504093468829922 ) ) ;
#8485=CARTESIAN_POINT ( 'NONE',  ( -3.834487992390000155, 1497.252746959389924, 198.5300765076990217 ) ) ;
#8486=CARTESIAN_POINT ( 'NONE',  ( 6.945936638575799904, 1467.632090493969827, 200.3893422253750032 ) ) ;
#8496=CARTESIAN_POINT ( 'NONE',  ( -14.93837056410000130, 1416.023439710309958, 212.9159407817990086 ) ) ;
#8498=EDGE_LOOP ( 'NONE', ( #86653, #59052, #102105, #67868, #39334 ) ) ;
#8500=CARTESIAN_POINT ( 'NONE',  ( 1.821641572679999932, 1508.445828156189918, 220.3212548158989819 ) ) ;
#8501=ADVANCED_FACE ( 'NONE', ( #10234 ), #25749, .F. ) ;
#8504=CARTESIAN_POINT ( 'NONE',  ( 2.793296738545309577, 1446.096199209579936, 199.4004782075479909 ) ) ;
#8506=LINE ( 'NONE', #110429, #28813 ) ;
#8509=CARTESIAN_POINT ( 'NONE',  ( -11.41709147838199989, 1481.865887416040096, 208.5948008914320155 ) ) ;
#8511=CARTESIAN_POINT ( 'NONE',  ( -5.260591405550000488, 1471.234187460190242, 214.2384833057390097 ) ) ;
#8522=CARTESIAN_POINT ( 'NONE',  ( -15.77133688790000043, 1418.153097379740075, 203.3734809581490026 ) ) ;
#8524=ADVANCED_FACE ( 'NONE', ( #81834 ), #36444, .F. ) ;
#8525=CARTESIAN_POINT ( 'NONE',  ( -4.107751809467400150, 1485.192704402420077, 197.9515937704389898 ) ) ;
#8526=CARTESIAN_POINT ( 'NONE',  ( -16.60289890951143121, 1419.621976417301084, 209.1245877213969777 ) ) ;
#8529=EDGE_CURVE ( 'NONE', #97755, #71088, #78645, .T. ) ;
#8537=CARTESIAN_POINT ( 'NONE',  ( -18.76586283470000183, 1443.851548150590133, 210.9125287142690013 ) ) ;
#8547=FACE_OUTER_BOUND ( 'NONE', #65768, .T. ) ;
#8552=CARTESIAN_POINT ( 'NONE',  ( 3.747879590680000206, 1486.431719912689914, 219.2436390487989968 ) ) ;
#8553=CARTESIAN_POINT ( 'NONE',  ( 11.69055014891650046, 1479.114015910159878, 207.7900583562500003 ) ) ;
#8555=CARTESIAN_POINT ( 'NONE',  ( -19.44024196839999874, 1446.691694840189939, 200.1268145916089907 ) ) ;
#8557=CARTESIAN_POINT ( 'NONE',  ( -17.84104529106779680, 1489.004166502169937, 195.1797425130460226 ) ) ;
#8563=CARTESIAN_POINT ( 'NONE',  ( 6.984146249619830549, 1448.464884018210114, 201.5728536464569913 ) ) ;
#8564=CARTESIAN_POINT ( 'NONE',  ( 11.16717556649999921, 1414.661898229710005, 205.5169791222290030 ) ) ;
#8568=DIRECTION ( 'NONE',  ( -0.9990022738941407576, 0.04465933583335028600, -2.184628763019654698E-05 ) ) ;
#8570=CARTESIAN_POINT ( 'NONE',  ( 1.969186904083861878, 1477.306100694335782, 198.9158131895061388 ) ) ;
#8571=EDGE_CURVE ( 'NONE', #28705, #56028, #36712, .T. ) ;
#8572=CARTESIAN_POINT ( 'NONE',  ( 7.440231166432099030, 1504.359119642949963, 219.0606402491349911 ) ) ;
#8587=CARTESIAN_POINT ( 'NONE',  ( 2.580208331920000209, 1468.552870077789976, 218.8097162688989670 ) ) ;
#8596=VERTEX_POINT ( 'NONE', #11899 ) ;
#8611=CARTESIAN_POINT ( 'NONE',  ( 0.3878997263335109968, 1423.031706118989860, 192.4974707188740126 ) ) ;
#8612=ORIENTED_EDGE ( 'NONE', *, *, #75587, .F. ) ;
#8614=CARTESIAN_POINT ( 'NONE',  ( -14.16375222470900219, 1508.551704408389924, 210.3503176839390107 ) ) ;
#8621=CONICAL_SURFACE ( 'NONE', #76567, 6.911399307709998219, 0.04363323129990067523 ) ;
#8622=CARTESIAN_POINT ( 'NONE',  ( -2.768293557658910053, 1429.049511582360083, 200.1700803755659877 ) ) ;
#8627=CARTESIAN_POINT ( 'NONE',  ( -11.74702494663919872, 1482.400884356720098, 207.2154382537309800 ) ) ;
#8635=B_SPLINE_CURVE_WITH_KNOTS ( 'NONE', 5,
 ( #19447, #78827, #104570, #54200, #72635, #80480, #3798, #89424, #12714, #21641, #81022, #88326, #27865, #4331, #30055, #62045, #79930, #105129, #64246, #62618, #55846 ),
 .UNSPECIFIED., .F., .F.,
 ( 6, 3, 3, 3, 3, 3, 6 ),
 ( 0.000000000000000000, 0.05351524642481629568, 0.1243167101037662425, 0.1849540613865951477, 0.2691738040383257480, 0.5436324044764058172, 1.000000000000000000 ),
 .UNSPECIFIED. ) ;
#8637=CARTESIAN_POINT ( 'NONE',  ( -12.71559489689999900, 1467.455103516190093, 192.9444858715990279 ) ) ;
#8641=CARTESIAN_POINT ( 'NONE',  ( -9.545666265298249797, 1448.964112459540047, 208.2525275868840140 ) ) ;
#8644=ORIENTED_EDGE ( 'NONE', *, *, #84525, .T. ) ;
#8650=CARTESIAN_POINT ( 'NONE',  ( -19.48953932349999718, 1466.720370645889943, 212.7779717757290143 ) ) ;
#8651=CARTESIAN_POINT ( 'NONE',  ( 2.765840192760000260, 1444.819550295790123, 203.5022050451889868 ) ) ;
#8654=CARTESIAN_POINT ( 'NONE',  ( -2.210109237099999735, 1430.259655991189902, 200.9461818968590023 ) ) ;
#8655=EDGE_CURVE ( 'NONE', #26067, #25916, #97915, .T. ) ;
#8657=CARTESIAN_POINT ( 'NONE',  ( 8.179408651070591674, 1464.307684099787593, 216.6184067479095745 ) ) ;
#8659=CARTESIAN_POINT ( 'NONE',  ( -9.521904627593841042, 1448.210782710000103, 209.8760350557079732 ) ) ;
#8670=CARTESIAN_POINT ( 'NONE',  ( -2.329906352152919968, 1515.372228416590133, 213.3835081558460161 ) ) ;
#8674=CARTESIAN_POINT ( 'NONE',  ( 3.208637323091700022, 1515.551704408389696, 212.9514660497620184 ) ) ;
#8678=DIRECTION ( 'NONE',  ( -1.699538841806929935E-33, 1.000000000000000000, -1.698192320643030073E-16 ) ) ;
#8683=CARTESIAN_POINT ( 'NONE',  ( -12.60557393880000099, 1502.061266880889889, 211.1128455371190000 ) ) ;
#8692=CARTESIAN_POINT ( 'NONE',  ( 7.096850047520000260, 1424.506042705289929, 213.0086243585190005 ) ) ;
#8693=CARTESIAN_POINT ( 'NONE',  ( -9.609628710759999137, 1464.248356776189894, 228.1965957863990013 ) ) ;
#8698=B_SPLINE_CURVE_WITH_KNOTS ( 'NONE', 3,
 ( #100651, #107408, #31809, #65998, #49733, #21726, #14988, #82204, #13331, #66549, #55928, #5510, #39666, #109087, #81644, #107961, #49185, #23937, #31258, #74940, #32368, #83314, #40212, #30704, #74392, #91165, #14440, #6610, #108518, #58132, #47522, #64890, #98997, #22274, #93361, #86622, #16626, #85501, #25596, #84953 ),
 .UNSPECIFIED., .F., .F.,
 ( 4, 3, 3, 3, 3, 3, 3, 3, 3, 3, 3, 3, 3, 4 ),
 ( -10.41361588720000064, -10.13063035700000114, -9.847644826829998976, -9.281676235200000846, -8.963578704315109391, -8.116477003980460125, -7.172239364826979546, -6.079724662395450174, -4.751561961960000247, -3.666469461290509990, -2.567348413909280147, -1.622951925397099870, -0.7893940661170741890, 0.000000000000000000 ),
 .UNSPECIFIED. ) ;
#8702=CARTESIAN_POINT ( 'NONE',  ( -19.83859993069999916, 1467.194195006989958, 209.1218459616989946 ) ) ;
#8710=CARTESIAN_POINT ( 'NONE',  ( -2.758550930766380027, 1475.074343013350017, 198.0237746611490195 ) ) ;
#8748=CARTESIAN_POINT ( 'NONE',  ( 9.001872265064569945, 1479.644900270570133, 227.9349562530539970 ) ) ;
#8757=CARTESIAN_POINT ( 'NONE',  ( -11.75527373628579930, 1491.528794388550068, 205.5782633857490111 ) ) ;
#8760=B_SPLINE_SURFACE_WITH_KNOTS ( 'NONE', 5, 1, ( 
 ( #100559, #92710 ),
 ( #110071, #67542 ),
 ( #84847, #83029 ),
 ( #108223, #89771 ),
 ( #108778, #57310 ),
 ( #73547, #13042 ) ),
 .UNSPECIFIED., .F., .F., .F.,
 ( 6, 6 ),
 ( 2, 2 ),
 ( -9.032913087590760002E-05, 17.14253593653090135 ),
 ( 0.000000000000000000, 14.00009032913090046 ),
 .UNSPECIFIED. ) ;
#8765=CARTESIAN_POINT ( 'NONE',  ( 9.698064461892839105, 1462.705242386489999, 208.0596150282290182 ) ) ;
#8767=CARTESIAN_POINT ( 'NONE',  ( 6.826200034800000260, 1424.874072630889941, 213.4902541782590220 ) ) ;
#8771=CARTESIAN_POINT ( 'NONE',  ( -16.65468421539999966, 1420.515480522079770, 203.5047434824589914 ) ) ;
#8773=CIRCLE ( 'NONE', #71429, 14.91144628110000170 ) ;
#8774=CARTESIAN_POINT ( 'NONE',  ( 19.30423710177419849, 1493.475036102569902, 199.7216101148530072 ) ) ;
#8776=CARTESIAN_POINT ( 'NONE',  ( -8.493714061740000432, 1509.017688834789851, 209.4777728399689920 ) ) ;
#8783=CARTESIAN_POINT ( 'NONE',  ( 6.225972109890000716, 1494.795958560490135, 219.7811165620990153 ) ) ;
#8784=CARTESIAN_POINT ( 'NONE',  ( -7.254007743607123970, 1458.163048246020253, 215.3456065187994852 ) ) ;
#8787=CARTESIAN_POINT ( 'NONE',  ( -11.39447792757199984, 1470.674147238439900, 209.5206840692040089 ) ) ;
#8793=CARTESIAN_POINT ( 'NONE',  ( -4.326992699989999913, 1515.158586642889986, 209.4787185339210112 ) ) ;
#8798=CARTESIAN_POINT ( 'NONE',  ( -4.636493443397069036, 1378.021649596855468, 203.9344422422949776 ) ) ;
#8799=CARTESIAN_POINT ( 'NONE',  ( -4.226426730560000067, 1515.477082009289916, 209.1218459617439862 ) ) ;
#8805=CARTESIAN_POINT ( 'NONE',  ( 10.53451941872170039, 1452.171317966529841, 208.4890148705030128 ) ) ;
#8809=CARTESIAN_POINT ( 'NONE',  ( -3.430374836980000008, 1431.708658569990121, 216.7924588047190184 ) ) ;
#8810=EDGE_CURVE ( 'NONE', #106272, #105229, #63629, .T. ) ;
#8811=ORIENTED_EDGE ( 'NONE', *, *, #22923, .T. ) ;
#8817=CARTESIAN_POINT ( 'NONE',  ( 11.76014171143800091, 1479.338753478690023, 208.6264959333659874 ) ) ;
#8822=CARTESIAN_POINT ( 'NONE',  ( -0.2329096773732799996, 1486.060289406110087, 197.2204110355460216 ) ) ;
#8823=CARTESIAN_POINT ( 'NONE',  ( 9.975222784249348607, 1470.060250684319954, 210.5865425885360196 ) ) ;
#8824=CARTESIAN_POINT ( 'NONE',  ( -9.197582055050311567, 1449.962432854769986, 209.3192927283980111 ) ) ;
#8825=CARTESIAN_POINT ( 'NONE',  ( -15.54139885464740090, 1421.077970550840064, 203.4236906915260192 ) ) ;
#8830=CARTESIAN_POINT ( 'NONE',  ( 22.14279220764339939, 1473.984090239060151, 210.1089564727559775 ) ) ;
#8841=CARTESIAN_POINT ( 'NONE',  ( -0.8775662281799990749, 1477.001762535890066, 198.7462694420989919 ) ) ;
#8846=CARTESIAN_POINT ( 'NONE',  ( 1.435735496894300134, 1429.431631213589981, 217.3000859563380232 ) ) ;
#8848=CARTESIAN_POINT ( 'NONE',  ( -8.075931970399999216, 1424.985315206749874, 206.4140305923890253 ) ) ;
#8853=CARTESIAN_POINT ( 'NONE',  ( 7.538390275667609330, 1425.596513388789845, 212.1820638689150087 ) ) ;
#8862=CARTESIAN_POINT ( 'NONE',  ( 2.589235753919999445E-16, 1524.551704408390151, 209.1218459616989946 ) ) ;
#8873=CARTESIAN_POINT ( 'NONE',  ( -10.68991641760000100, 1481.192726480790043, 208.4620359433729959 ) ) ;
#8875=TOROIDAL_SURFACE ( 'NONE', #71529, 4.250000000000000000, 0.5000000000000000000 ) ;
#8880=ADVANCED_FACE ( 'NONE', ( #7883 ), #99522, .F. ) ;
#8882=CARTESIAN_POINT ( 'NONE',  ( -3.710825910270000083, 1429.315763641489866, 201.5588532669389963 ) ) ;
#8884=ORIENTED_EDGE ( 'NONE', *, *, #69223, .F. ) ;
#8894=CARTESIAN_POINT ( 'NONE',  ( -2.801140078490090168, 1508.551704408389924, 214.0906714726369842 ) ) ;
#8897=CARTESIAN_POINT ( 'NONE',  ( 7.367316997829999714, 1422.547007707180001, 195.5834347947990182 ) ) ;
#8900=CARTESIAN_POINT ( 'NONE',  ( -3.671863939699999690, 1495.492710535389961, 197.3513011073989958 ) ) ;
#8915=CARTESIAN_POINT ( 'NONE',  ( 8.331628387504050437, 1425.215661044880108, 210.8086245623740069 ) ) ;
#8917=CARTESIAN_POINT ( 'NONE',  ( -10.90853107422250012, 1462.746370323140127, 207.3438040333890058 ) ) ;
#8926=CARTESIAN_POINT ( 'NONE',  ( 18.27002674530000093, 1430.510071776790028, 200.9389885209290014 ) ) ;
#8928=CARTESIAN_POINT ( 'NONE',  ( 11.16314367537479946, 1421.171381915769871, 200.1196691949539854 ) ) ;
#8929=CARTESIAN_POINT ( 'NONE',  ( 6.531329447192200099, 1466.275421158679819, 216.6368425205710082 ) ) ;
#8933=AXIS2_PLACEMENT_3D ( 'NONE', #6540, #38479, #64265 ) ;
#8935=CARTESIAN_POINT ( 'NONE',  ( 1.644415622395181353, 1478.048958850599092, 198.8242942082682418 ) ) ;
#8937=CARTESIAN_POINT ( 'NONE',  ( -1.842963900900000063, 1515.551704191689851, 205.2922257884789872 ) ) ;
#8939=CARTESIAN_POINT ( 'NONE',  ( 16.50821395286810045, 1494.476688879279891, 193.0250025734499957 ) ) ;
#8942=CARTESIAN_POINT ( 'NONE',  ( -18.95612632361009631, 1419.023425851569982, 208.8707427548719977 ) ) ;
#8944=CARTESIAN_POINT ( 'NONE',  ( 3.414905379839999977, 1441.318761073790029, 218.0249493360389863 ) ) ;
#8948=CARTESIAN_POINT ( 'NONE',  ( 12.03449236470000017, 1491.353386475389925, 206.6667661057590237 ) ) ;
#8956=CARTESIAN_POINT ( 'NONE',  ( 13.68046382411920092, 1499.825599652919891, 226.3926818705750179 ) ) ;
#8957=B_SPLINE_CURVE_WITH_KNOTS ( 'NONE', 3,
 ( #23154, #101503, #42182, #83077, #6370, #86382, #87505, #27041, #77443, #68505, #1861, #53930, #78546, #103741, #61229, #2420 ),
 .UNSPECIFIED., .F., .F.,
 ( 4, 3, 3, 3, 3, 4 ),
 ( 4.019724148039999889, 6.150493503467039602, 8.416124416742510661, 10.70624330608290009, 12.92002759199360007, 13.77031185580000106 ),
 .UNSPECIFIED. ) ;
#8959=CARTESIAN_POINT ( 'NONE',  ( -6.860676238782120073, 1434.586309434399936, 214.3896270283869967 ) ) ;
#8962=CARTESIAN_POINT ( 'NONE',  ( -17.97414461820000042, 1423.929594390560169, 208.2618829023350031 ) ) ;
#8967=CARTESIAN_POINT ( 'NONE',  ( 11.52984783759620058, 1422.027592033300152, 208.2049052604949964 ) ) ;
#8971=EDGE_LOOP ( 'NONE', ( #100836, #92993, #66469, #85333 ) ) ;
#8972=CARTESIAN_POINT ( 'NONE',  ( -19.78987248279999989, 1467.442824718890051, 207.1782906715690160 ) ) ;
#8982=CARTESIAN_POINT ( 'NONE',  ( 4.439133174170000196, 1445.351637362389738, 201.2425731753489799 ) ) ;
#8983=FACE_OUTER_BOUND ( 'NONE', #35747, .T. ) ;
#8985=CARTESIAN_POINT ( 'NONE',  ( -2.009517772400000180, 1455.098376589789950, 199.1884203155790090 ) ) ;
#8990=CARTESIAN_POINT ( 'NONE',  ( -1.776356839399999804E-15, 1414.661898229710005, 209.1218459616989946 ) ) ;
#8992=CARTESIAN_POINT ( 'NONE',  ( -0.01467710756120139959, 1495.315433949589988, 220.4548505147990056 ) ) ;
#8995=EDGE_LOOP ( 'NONE', ( #65890, #56124, #29561, #106090 ) ) ;
#9007=CARTESIAN_POINT ( 'NONE',  ( 4.106634628316339963, 1508.551704408389924, 213.5130254241009879 ) ) ;
#9011=CARTESIAN_POINT ( 'NONE',  ( 9.762886224428157789, 1460.688233213919830, 206.5243166130410088 ) ) ;
#9015=COLOUR_RGB ( '', 0.40784314, 0.44705882, 0.49803922) ;
#9016=ORIENTED_EDGE ( 'NONE', *, *, #2859, .F. ) ;
#9020=CARTESIAN_POINT ( 'NONE',  ( -10.88843716487655122, 1417.951816079329774, 198.2287934583217179 ) ) ;
#9026=EDGE_CURVE ( 'NONE', #27470, #42229, #53227, .T. ) ;
#9027=CARTESIAN_POINT ( 'NONE',  ( 9.970943783957169515, 1451.601728650610085, 207.6130147570040094 ) ) ;
#9028=FACE_OUTER_BOUND ( 'NONE', #12738, .T. ) ;
#9039=CARTESIAN_POINT ( 'NONE',  ( 7.053034928242810864, 1429.189209343189987, 215.4664347411579968 ) ) ;
#9045=CARTESIAN_POINT ( 'NONE',  ( 5.989307772389999229, 1494.629795928590056, 219.4239502688990058 ) ) ;
#9048=EDGE_CURVE ( 'NONE', #50471, #21520, #10100, .T. ) ;
#9054=B_SPLINE_SURFACE_WITH_KNOTS ( 'NONE', 5, 5, ( 
 ( #99432, #75374, #66973, #23281, #101084, #24382 ),
 ( #57477, #22710, #30594, #64782, #14879, #39551 ),
 ( #98892, #22160, #56360, #90492, #13767, #47951 ),
 ( #73725, #56908, #91041, #82658, #5949, #74276 ),
 ( #52386, #76454, #51254, #77023, #94916, #8683 ),
 ( #27164, #876, #95468, #61348, #18732, #93248 ) ),
 .UNSPECIFIED., .F., .F., .F.,
 ( 6, 6 ),
 ( 6, 6 ),
 ( 44.26078367470000074, 48.30090647720000163 ),
 ( 0.000000000000000000, 2.000000000000000000 ),
 .UNSPECIFIED. ) ;
#9061=CARTESIAN_POINT ( 'NONE',  ( -14.62523883179999906, 1415.865102022439942, 213.8037711709790187 ) ) ;
#9063=CARTESIAN_POINT ( 'NONE',  ( -0.6915095762680909530, 1515.131927850350166, 204.7941551768030308 ) ) ;
#9067=CARTESIAN_POINT ( 'NONE',  ( -2.140640208939999845, 1508.551704408389924, 220.0635243260990137 ) ) ;
#9070=CARTESIAN_POINT ( 'NONE',  ( 2.915041327195820209, 1446.157008382559980, 199.4325186832650161 ) ) ;
#9071=EDGE_CURVE ( 'NONE', #77131, #81034, #56940, .T. ) ;
#9078=CARTESIAN_POINT ( 'NONE',  ( -10.85282564929999971, 1480.164835466490103, 213.9155123631190065 ) ) ;
#9079=CARTESIAN_POINT ( 'NONE',  ( -2.519788581729999866, 1470.392735159189897, 216.0597033484689860 ) ) ;
#9086=CARTESIAN_POINT ( 'NONE',  ( -15.60330020924029881, 1418.235805516329947, 203.0264043510670149 ) ) ;
#9090=CARTESIAN_POINT ( 'NONE',  ( -16.16040309870000158, 1417.154526695929917, 206.7693472903190184 ) ) ;
#9093=B_SPLINE_SURFACE_WITH_KNOTS ( 'NONE', 5, 5, ( 
 ( #100123, #109093, #49191, #92820, #84958, #7712 ),
 ( #67649, #91719, #6064, #23407, #48643, #109632 ),
 ( #40217, #74398, #92271, #32375, #110176, #75498 ),
 ( #49740, #16091, #74946, #50298, #31815, #108523 ),
 ( #83867, #66555, #101757, #100659, #14993, #58687 ),
 ( #66003, #84426, #23943, #57598, #40768, #7170 ),
 ( #32905, #83320, #76026, #67098, #41871, #101201 ),
 ( #42418, #24497, #76575, #33448, #82771, #8252 ),
 ( #58139, #6615, #25045, #110727, #59247, #93366 ) ),
 .UNSPECIFIED., .F., .F., .F.,
 ( 6, 3, 6 ),
 ( 6, 6 ),
 ( 3.230686157760149779, 5.552647417019999310, 7.874608676279850172 ),
 ( -0.0004440811798492790030, 2.000000000000000000 ),
 .UNSPECIFIED. ) ;
#9094=CARTESIAN_POINT ( 'NONE',  ( -8.646868171490730504, 1437.292463641849736, 208.9934304095080222 ) ) ;
#9096=EDGE_LOOP ( 'NONE', ( #21527, #43332, #22041, #56274, #86967, #11281, #70964, #12579, #104621, #8811, #66466, #53503, #23609, #20853, #13401 ) ) ;
#9099=CARTESIAN_POINT ( 'NONE',  ( 10.55886014504109838, 1481.314177749799910, 208.6326544899590090 ) ) ;
#9112=CARTESIAN_POINT ( 'NONE',  ( 8.648576441527131564, 1470.685138533134250, 214.4961241725896741 ) ) ;
#9119=CARTESIAN_POINT ( 'NONE',  ( 10.47542077232779967, 1481.052741024980151, 207.7774047151940238 ) ) ;
#9120=CARTESIAN_POINT ( 'NONE',  ( -6.112144431844329873, 1451.758908031599958, 207.3773668546839986 ) ) ;
#9121=CARTESIAN_POINT ( 'NONE',  ( 11.52930592674979948, 1434.731876196460007, 225.7086000943210138 ) ) ;
#9122=CARTESIAN_POINT ( 'NONE',  ( -3.945788320325708032, 1515.565606825038003, 210.3713667179344782 ) ) ;
#9123=CARTESIAN_POINT ( 'NONE',  ( 16.50820874103769853, 1494.476754866449937, 193.0249925670599964 ) ) ;
#9129=CARTESIAN_POINT ( 'NONE',  ( -10.98820255369999899, 1490.057925297589918, 212.1172194307789880 ) ) ;
#9130=CARTESIAN_POINT ( 'NONE',  ( 5.964116108761399637, 1447.836085667069938, 200.8032929224230259 ) ) ;
#9140=CARTESIAN_POINT ( 'NONE',  ( 6.510813747272850449, 1506.316984162309836, 218.8516934173640323 ) ) ;
#9147=ORIENTED_EDGE ( 'NONE', *, *, #481, .F. ) ;
#9149=CARTESIAN_POINT ( 'NONE',  ( -10.30780163688080009, 1448.538669356370065, 207.8996510353259737 ) ) ;
#9150=CARTESIAN_POINT ( 'NONE',  ( 3.982959088878939902, 1515.551843419129909, 206.2722828609170165 ) ) ;
#9164=VERTEX_POINT ( 'NONE', #64387 ) ;
#9166=ADVANCED_FACE ( 'NONE', ( #89559 ), #106905, .T. ) ;
#9171=CARTESIAN_POINT ( 'NONE',  ( -8.046540862050292731, 1474.840790622590930, 202.7137200846936196 ) ) ;
#9184=FACE_OUTER_BOUND ( 'NONE', #30103, .T. ) ;
#9190=EDGE_LOOP ( 'NONE', ( #3813, #84021, #28525, #19183 ) ) ;
#9192=CARTESIAN_POINT ( 'NONE',  ( -15.59788086836899978, 1508.551704408389924, 210.3719525949329920 ) ) ;
#9197=CARTESIAN_POINT ( 'NONE',  ( 19.55988977460000200, 1474.636381753090063, 214.0184790771390055 ) ) ;
#9201=CARTESIAN_POINT ( 'NONE',  ( -2.620874085839509871, 1429.130643781209983, 200.1242597526310192 ) ) ;
#9215=EDGE_CURVE ( 'NONE', #106390, #59861, #28790, .T. ) ;
#9220=CARTESIAN_POINT ( 'NONE',  ( -10.32568877401340224, 1448.475227332080067, 208.0351690947539964 ) ) ;
#9224=CARTESIAN_POINT ( 'NONE',  ( -11.86647391014470010, 1508.441731521209931, 217.8507656475659928 ) ) ;
#9241=CARTESIAN_POINT ( 'NONE',  ( 3.560575673166030075, 1456.106869275790132, 219.1309344377709749 ) ) ;
#9245=CARTESIAN_POINT ( 'NONE',  ( 11.40024098090000138, 1502.471351942989941, 210.6161612907290248 ) ) ;
#9253=CARTESIAN_POINT ( 'NONE',  ( -7.851774706560000539, 1482.164398796690193, 201.8541463733390060 ) ) ;
#9256=ORIENTED_EDGE ( 'NONE', *, *, #66126, .F. ) ;
#9258=CARTESIAN_POINT ( 'NONE',  ( -4.440280304591389893, 1489.606077279609735, 216.0962888374899933 ) ) ;
#9260=ORIENTED_EDGE ( 'NONE', *, *, #18756, .T. ) ;
#9261=CARTESIAN_POINT ( 'NONE',  ( -0.1973361429370009967, 1494.452141646590007, 217.5167685628690037 ) ) ;
#9262=CARTESIAN_POINT ( 'NONE',  ( -15.26295761389349792, 1416.044054022097953, 206.4503499115064926 ) ) ;
#9264=CARTESIAN_POINT ( 'NONE',  ( 1.250280881337970218, 1456.664103658099975, 219.6692350580109974 ) ) ;
#9268=CARTESIAN_POINT ( 'NONE',  ( 2.740701793870000014, 1426.136123009330049, 188.7843822941989913 ) ) ;
#9276=CARTESIAN_POINT ( 'NONE',  ( -21.54678038960369690, 1506.340315034190098, 209.2559991757600244 ) ) ;
#9278=CARTESIAN_POINT ( 'NONE',  ( 7.900179536920721723, 1500.382728750624892, 200.8993804518913748 ) ) ;
#9281=CARTESIAN_POINT ( 'NONE',  ( -0.9866390672850040566, 1475.553619744739990, 197.7149975239109949 ) ) ;
#9292=VERTEX_POINT ( 'NONE', #31303 ) ;
#9322=CARTESIAN_POINT ( 'NONE',  ( -6.076016578960000913, 1450.645075640589994, 208.7037629494849966 ) ) ;
#9327=DIRECTION ( 'NONE',  ( 0.02091224828123190022, 0.9990482215818557998, 0.03827961371219716635 ) ) ;
#9333=CARTESIAN_POINT ( 'NONE',  ( -9.983110113756229254, 1492.881261275560064, 201.9487339551459968 ) ) ;
#9346=EDGE_CURVE ( 'NONE', #75555, #49951, #75400, .T. ) ;
#9349=CARTESIAN_POINT ( 'NONE',  ( 17.00812965271749988, 1492.794527032730002, 195.6196781557690088 ) ) ;
#9353=CARTESIAN_POINT ( 'NONE',  ( 2.993128258680000098, 1442.239305041489843, 217.5960754105989849 ) ) ;
#9370=CARTESIAN_POINT ( 'NONE',  ( -11.23993869538120016, 1470.374453574730069, 210.9407000820530129 ) ) ;
#9371=CARTESIAN_POINT ( 'NONE',  ( -2.993067780513550158, 1487.214450571009820, 219.9661333581329927 ) ) ;
#9372=CARTESIAN_POINT ( 'NONE',  ( -16.83567051276560278, 1418.884454701650156, 201.2565205294370116 ) ) ;
#9377=CARTESIAN_POINT ( 'NONE',  ( 10.52289893411149890, 1452.116717517039888, 208.3553807036720116 ) ) ;
#9388=CARTESIAN_POINT ( 'NONE',  ( 4.896309118140000471, 1485.934254991190073, 218.7196314378989825 ) ) ;
#9389=CARTESIAN_POINT ( 'NONE',  ( 8.561878008634579373, 1436.589096639300124, 208.1469354389350030 ) ) ;
#9397=CARTESIAN_POINT ( 'NONE',  ( -14.65253846807509852, 1421.518381437140079, 203.5747437415320178 ) ) ;
#9398=AXIS2_PLACEMENT_3D ( 'NONE', #36338, #70531, #71649 ) ;
#9402=CARTESIAN_POINT ( 'NONE',  ( -13.48707387329999818, 1506.009490401690073, 209.0918298080249826 ) ) ;
#9403=CARTESIAN_POINT ( 'NONE',  ( -4.284681050939999736, 1482.348681575889941, 231.1486602034989915 ) ) ;
#9407=CARTESIAN_POINT ( 'NONE',  ( -6.733221321159999384, 1470.315040358090073, 190.1905927392990066 ) ) ;
#9408=CARTESIAN_POINT ( 'NONE',  ( 4.329338606958539337, 1515.069000070079937, 210.7431442201590244 ) ) ;
#9410=CARTESIAN_POINT ( 'NONE',  ( -11.60674135321730027, 1507.508082919659955, 207.5537295141489835 ) ) ;
#9418=CARTESIAN_POINT ( 'NONE',  ( -8.131798216469999119, 1423.938023408190020, 210.2346984346590091 ) ) ;
#9423=CARTESIAN_POINT ( 'NONE',  ( 7.534131688341251021, 1425.533913774680059, 212.1852849544380035 ) ) ;
#9425=ORIENTED_EDGE ( 'NONE', *, *, #21553, .T. ) ;
#9429=CARTESIAN_POINT ( 'NONE',  ( 6.768867072198900381, 1426.907320758384230, 213.7789536137680386 ) ) ;
#9430=CARTESIAN_POINT ( 'NONE',  ( -4.325405441727872002, 1515.219201590508419, 207.2788837474028014 ) ) ;
#9433=ORIENTED_EDGE ( 'NONE', *, *, #74106, .F. ) ;
#9439=ORIENTED_EDGE ( 'NONE', *, *, #63060, .T. ) ;
#9450=CARTESIAN_POINT ( 'NONE',  ( -4.989533930479999491, 1429.437332217889889, 202.3857892670889953 ) ) ;
#9457=CARTESIAN_POINT ( 'NONE',  ( 2.487921644133460397, 1508.551704408389924, 204.1347675643650348 ) ) ;
#9461=CARTESIAN_POINT ( 'NONE',  ( 12.37893659083640152, 1501.369140013739980, 212.0434529887650115 ) ) ;
#9462=CARTESIAN_POINT ( 'NONE',  ( 7.500748375389999723, 1423.062354593270129, 195.6521519453989697 ) ) ;
#9472=EDGE_LOOP ( 'NONE', ( #17245, #79198, #16852, #33950, #105720, #69505, #60397, #79187, #106401 ) ) ;
#9477=CARTESIAN_POINT ( 'NONE',  ( 0.02783439897821873149, 1421.066780746317590, 193.7160764248625071 ) ) ;
#9484=CARTESIAN_POINT ( 'NONE',  ( -9.666683979049999209, 1423.817746360030014, 192.3656247972989775 ) ) ;
#9485=CARTESIAN_POINT ( 'NONE',  ( 10.94894508182309956, 1424.836538624790137, 201.4990293608930187 ) ) ;
#9494=CARTESIAN_POINT ( 'NONE',  ( -16.61337446934520301, 1463.629612318100044, 220.4655171191939758 ) ) ;
#9496=CARTESIAN_POINT ( 'NONE',  ( -13.96277354420170091, 1421.421066752219986, 206.6487300726359990 ) ) ;
#9498=CARTESIAN_POINT ( 'NONE',  ( 8.883945244656709761, 1451.594843122180009, 211.7725949629070215 ) ) ;
#9500=CARTESIAN_POINT ( 'NONE',  ( 4.124127541549999165, 1440.791920158089852, 218.1322488136489994 ) ) ;
#9506=CARTESIAN_POINT ( 'NONE',  ( 20.33509540109970004, 1432.834541216450134, 214.7556705994980177 ) ) ;
#9513=CARTESIAN_POINT ( 'NONE',  ( 1.842963787330042180, 1515.551704408389469, 213.0801841379113455 ) ) ;
#9518=CARTESIAN_POINT ( 'NONE',  ( 10.42928995599340070, 1426.801324560409967, 208.9238221840179790 ) ) ;
#9521=CARTESIAN_POINT ( 'NONE',  ( -0.2285350204260230278, 1437.936383516839896, 227.6814155838589784 ) ) ;
#9522=ORIENTED_EDGE ( 'NONE', *, *, #65731, .F. ) ;
#9531=DIRECTION ( 'NONE',  ( 1.000000000000000000, 0.000000000000000000, 0.000000000000000000 ) ) ;
#9539=CARTESIAN_POINT ( 'NONE',  ( -3.163205911649999980, 1497.502928199090093, 198.2885394267989909 ) ) ;
#9540=CARTESIAN_POINT ( 'NONE',  ( -1.029084866039999824, 1496.468087385590024, 221.4697290446989939 ) ) ;
#9541=VERTEX_POINT ( 'NONE', #105144 ) ;
#9554=CARTESIAN_POINT ( 'NONE',  ( 2.759035106590659758, 1508.551704408389924, 214.0956385152369990 ) ) ;
#9558=CARTESIAN_POINT ( 'NONE',  ( 10.49207437818910016, 1461.076854184230115, 208.4973394663880129 ) ) ;
#9567=CARTESIAN_POINT ( 'NONE',  ( -9.360141924177080242, 1418.479953072925355, 196.8921625633495012 ) ) ;
#9571=CARTESIAN_POINT ( 'NONE',  ( 9.251643635294589885, 1451.133743409539875, 209.4001945862339937 ) ) ;
#9578=CARTESIAN_POINT ( 'NONE',  ( 18.72979941119999836, 1454.437773883689943, 204.5413093961989830 ) ) ;
#9585=CARTESIAN_POINT ( 'NONE',  ( -1.713536632167919960, 1469.335432983970122, 219.0203854141810211 ) ) ;
#9588=CARTESIAN_POINT ( 'NONE',  ( 4.487249775049700240, 1509.038615934839981, 206.6339108193819811 ) ) ;
#9589=CARTESIAN_POINT ( 'NONE',  ( -12.78943302956389871, 1502.708798875820094, 209.0180534851929792 ) ) ;
#9595=CARTESIAN_POINT ( 'NONE',  ( 9.468383857098320533, 1468.845280592710196, 203.0453074138920044 ) ) ;
#9599=ORIENTED_EDGE ( 'NONE', *, *, #78365, .T. ) ;
#9603=CARTESIAN_POINT ( 'NONE',  ( -14.44692751430000044, 1415.677402202029953, 213.4243480473190289 ) ) ;
#9604=CARTESIAN_POINT ( 'NONE',  ( 1.842962231260000028, 1515.064792882589927, 204.7923971856590128 ) ) ;
#9610=B_SPLINE_CURVE_WITH_KNOTS ( 'NONE', 3,
 ( #71338, #96498, #19778, #53979, #27635, #11939, #18659, #37691, #106546, #87557, #55067, #71894, #80801, #95944, #97601, #46119, #88112, #4107, #20871 ),
 .UNSPECIFIED., .F., .F.,
 ( 4, 3, 3, 3, 3, 3, 4 ),
 ( -7.430926493242850484, -7.167859904195459819, -6.108952779777689912, -5.238805666324060084, -4.533344564236309715, -3.758780901387599460, -3.046684027039999521 ),
 .UNSPECIFIED. ) ;
#9616=EDGE_CURVE ( 'NONE', #16269, #20056, #63179, .T. ) ;
#9617=CARTESIAN_POINT ( 'NONE',  ( -9.861282131150000296, 1479.534343986590102, 214.8159920528989915 ) ) ;
#9626=CARTESIAN_POINT ( 'NONE',  ( 19.64599270300000100, 1476.662575758389949, 214.0395835971089866 ) ) ;
#9630=CARTESIAN_POINT ( 'NONE',  ( -5.906252883828099876, 1484.773058574589868, 198.7863962546840071 ) ) ;
#9636=CARTESIAN_POINT ( 'NONE',  ( -11.77719994041109963, 1507.564759742010210, 208.2431318171160228 ) ) ;
#9649=DIRECTION ( 'NONE',  ( 0.4794255386042031719, 0.000000000000000000, 0.8775825618903726477 ) ) ;
#9654=ADVANCED_FACE ( 'NONE', ( #89442 ), #28434, .F. ) ;
#9656=CARTESIAN_POINT ( 'NONE',  ( 4.389420737370000047, 1486.156988616190120, 218.9715652691990044 ) ) ;
#9657=CARTESIAN_POINT ( 'NONE',  ( 10.43856162392300035, 1480.982005454859973, 207.5364568915489940 ) ) ;
#9660=EDGE_CURVE ( 'NONE', #27509, #15707, #23201, .T. ) ;
#9661=CARTESIAN_POINT ( 'NONE',  ( 19.14951757210000238, 1460.484328893590146, 220.2380389338990199 ) ) ;
#9663=CARTESIAN_POINT ( 'NONE',  ( 9.992001554966840615, 1491.422527301840319, 188.4943246010310247 ) ) ;
#9666=CARTESIAN_POINT ( 'NONE',  ( -4.993299335669999728, 1391.657172340389934, 203.5222458180090257 ) ) ;
#9668=CARTESIAN_POINT ( 'NONE',  ( -11.24552814110000121, 1490.344885738790026, 211.0486739485690180 ) ) ;
#9669=CARTESIAN_POINT ( 'NONE',  ( 9.735382849826228480, 1450.705275490849999, 205.3287227118019871 ) ) ;
#9677=CARTESIAN_POINT ( 'NONE',  ( 2.326513286163319538, 1476.258183507229887, 197.8633931498989966 ) ) ;
#9678=CARTESIAN_POINT ( 'NONE',  ( 6.386763885830579746, 1505.038503483219984, 219.3374787946009974 ) ) ;
#9679=CARTESIAN_POINT ( 'NONE',  ( -9.315479902914303167, 1422.891722004452731, 210.7235706083796458 ) ) ;
#9682=ORIENTED_EDGE ( 'NONE', *, *, #65339, .F. ) ;
#9689=CARTESIAN_POINT ( 'NONE',  ( 2.898098007870020254, 1515.492902828930028, 204.9850961497120352 ) ) ;
#9697=B_SPLINE_SURFACE_WITH_KNOTS ( 'NONE', 5, 5, ( 
 ( #26931, #2311, #62779, #86276, #19050, #62212 ),
 ( #18499, #36422, #44857, #27468, #53253, #87393 ),
 ( #104735, #85719, #79009, #52695, #51587, #86831 ),
 ( #95783, #70615, #28024, #19617, #35889, #11246 ),
 ( #53818, #45407, #79547, #2849, #36973, #71165 ),
 ( #43189, #77341, #5021, #38080, #71733, #80083 ),
 ( #96893, #38621, #45944, #22346, #5585, #21239 ),
 ( #63316, #97436, #64953, #99067, #54899, #20703 ),
 ( #13402, #97970, #89578, #89026, #72257, #12870 ) ),
 .UNSPECIFIED., .F., .F., .F.,
 ( 6, 3, 6 ),
 ( 6, 6 ),
 ( 3.012462719602379657, 5.172868947549999596, 7.333275175507620425 ),
 ( -0.0004258868076247550446, 2.000000000000000000 ),
 .UNSPECIFIED. ) ;
#9701=CARTESIAN_POINT ( 'NONE',  ( -8.466661967441870829, 1424.048519636140099, 207.5723062640520027 ) ) ;
#9713=CARTESIAN_POINT ( 'NONE',  ( 9.720721973410000771, 1462.346955765789971, 208.4427505688250051 ) ) ;
#9717=CARTESIAN_POINT ( 'NONE',  ( 2.949954862130000244, 1464.477966747790106, 199.7317119218890014 ) ) ;
#9719=ORIENTED_EDGE ( 'NONE', *, *, #12532, .F. ) ;
#9722=EDGE_LOOP ( 'NONE', ( #100361, #31184, #38666, #29350, #80475, #97891, #7341 ) ) ;
#9729=CARTESIAN_POINT ( 'NONE',  ( 5.161277877375379575, 1424.205378946189967, 193.2953230041809718 ) ) ;
#9734=CARTESIAN_POINT ( 'NONE',  ( -2.409034624560000282, 1511.999350511789999, 211.5308805862590020 ) ) ;
#9744=CARTESIAN_POINT ( 'NONE',  ( -11.81773885611420027, 1482.251074316360018, 207.7669157962629924 ) ) ;
#9749=CARTESIAN_POINT ( 'NONE',  ( 10.93679547204000002, 1490.434980368090010, 209.9321327948960061 ) ) ;
#9757=CARTESIAN_POINT ( 'NONE',  ( -8.884856068493249381, 1449.032530459529880, 211.3463590648900094 ) ) ;
#9773=CARTESIAN_POINT ( 'NONE',  ( -1.682023246740000033, 1431.030650798590159, 200.9066206319189973 ) ) ;
#9774=CARTESIAN_POINT ( 'NONE',  ( 10.60784606965410148, 1480.939836828909847, 210.5430849895140284 ) ) ;
#9777=ORIENTED_EDGE ( 'NONE', *, *, #25491, .T. ) ;
#9778=MANIFOLD_SOLID_BREP ( 'Stock-MAS-682-1', #44953 ) ;
#9780=ADVANCED_FACE ( 'NONE', ( #88094 ), #59760, .T. ) ;
#9782=CARTESIAN_POINT ( 'NONE',  ( 3.629220049600000220, 1485.493215689190038, 199.0019176958990101 ) ) ;
#9785=CARTESIAN_POINT ( 'NONE',  ( 11.85479774020000043, 1501.321054691989957, 210.0448065485869904 ) ) ;
#9790=CARTESIAN_POINT ( 'NONE',  ( -7.027952441359999192, 1482.449581481789892, 201.0380530320790058 ) ) ;
#9800=ORIENTED_EDGE ( 'NONE', *, *, #74922, .T. ) ;
#9801=CARTESIAN_POINT ( 'NONE',  ( -1.821463311390000062, 1495.107949858190068, 217.3487309858989818 ) ) ;
#9802=CARTESIAN_POINT ( 'NONE',  ( -14.93413738244312228, 1416.108689801689025, 205.2226948075607709 ) ) ;
#9804=CARTESIAN_POINT ( 'NONE',  ( -9.977180581269040616, 1439.208816910850146, 209.0674583647880240 ) ) ;
#9809=CARTESIAN_POINT ( 'NONE',  ( 7.618847152659999900, 1425.153911876999928, 211.9847758557390023 ) ) ;
#9810=FACE_OUTER_BOUND ( 'NONE', #68119, .T. ) ;
#9815=CARTESIAN_POINT ( 'NONE',  ( 5.082331142230000154, 1453.684120746589770, 217.0135184815189859 ) ) ;
#9817=EDGE_LOOP ( 'NONE', ( #71992, #5466, #79082, #2669 ) ) ;
#9825=CARTESIAN_POINT ( 'NONE',  ( -2.890649542061729971, 1475.035107952139924, 198.0572108960010098 ) ) ;
#9839=CARTESIAN_POINT ( 'NONE',  ( -4.172050517839999806, 1455.094832059689907, 200.6673091711190011 ) ) ;
#9842=EDGE_CURVE ( 'NONE', #3898, #73081, #4583, .T. ) ;
#9845=ORIENTED_EDGE ( 'NONE', *, *, #74031, .T. ) ;
#9854=CARTESIAN_POINT ( 'NONE',  ( 9.691985945171570194, 1462.686535208950090, 208.0124194077490074 ) ) ;
#9864=CARTESIAN_POINT ( 'NONE',  ( 9.273172440071220990, 1436.467920671469983, 210.7384122601949912 ) ) ;
#9867=CARTESIAN_POINT ( 'NONE',  ( 13.84584525154450141, 1499.900191053290200, 227.7510545287100001 ) ) ;
#9892=CARTESIAN_POINT ( 'NONE',  ( -8.331757017630000206, 1505.205016750989898, 208.8972188790260134 ) ) ;
#9897=FACE_OUTER_BOUND ( 'NONE', #68520, .T. ) ;
#9898=EDGE_CURVE ( 'NONE', #5600, #34770, #37901, .T. ) ;
#9904=CARTESIAN_POINT ( 'NONE',  ( -2.140897214623600053, 1421.480990132170064, 193.7252737798519888 ) ) ;
#9911=CARTESIAN_POINT ( 'NONE',  ( 9.651066088509999474, 1425.440658930580184, 195.4941615409990163 ) ) ;
#9916=CARTESIAN_POINT ( 'NONE',  ( -4.038582019099999698, 1515.598601288489817, 209.1218459616829932 ) ) ;
#9918=AXIS2_PLACEMENT_3D ( 'NONE', #31273, #23417, #33456 ) ;
#9919=DIRECTION ( 'NONE',  ( -0.9126757963125582407, 0.3056501852620481241, 0.2712947752436700721 ) ) ;
#9922=CARTESIAN_POINT ( 'NONE',  ( 10.35952170215530010, 1451.661118394300047, 207.3115203362889929 ) ) ;
#9931=CARTESIAN_POINT ( 'NONE',  ( -4.772349923247530157, 1461.586223916219978, 228.1255533131570132 ) ) ;
#9934=CARTESIAN_POINT ( 'NONE',  ( 5.161034791280000533, 1485.814572579490005, 218.5690567784690188 ) ) ;
#9935=ADVANCED_FACE ( 'NONE', ( #107073 ), #37671, .T. ) ;
#9944=CARTESIAN_POINT ( 'NONE',  ( 8.249347533650759345, 1435.329610800189812, 206.3473214876380268 ) ) ;
#9945=CARTESIAN_POINT ( 'NONE',  ( -15.49276695593840181, 1421.101837051059874, 203.4317233017570175 ) ) ;
#9946=EDGE_CURVE ( 'NONE', #60953, #95904, #32538, .T. ) ;
#9948=CARTESIAN_POINT ( 'NONE',  ( 3.535327672168380175, 1487.160996015089950, 197.6951163816430039 ) ) ;
#9951=CARTESIAN_POINT ( 'NONE',  ( 18.27173588000000137, 1474.555276297389810, 194.7671755014989969 ) ) ;
#9958=CARTESIAN_POINT ( 'NONE',  ( -11.65521739912845156, 1507.535655403029295, 207.9035470747624004 ) ) ;
#9962=CARTESIAN_POINT ( 'NONE',  ( -9.082109893440000192, 1460.473744250790105, 214.5004399023289920 ) ) ;
#9967=CARTESIAN_POINT ( 'NONE',  ( -8.754460142190000127, 1423.123606144270070, 210.6600973048190042 ) ) ;
#9973=CARTESIAN_POINT ( 'NONE',  ( 7.503182177443590284, 1425.966042803340088, 212.3089147954889881 ) ) ;
#9974=CARTESIAN_POINT ( 'NONE',  ( 0.5135640108309369456, 1496.071902881799815, 221.4546726054459782 ) ) ;
#9977=CARTESIAN_POINT ( 'NONE',  ( 5.068064628910000202, 1505.106222020589939, 220.8372522273990057 ) ) ;
#9981=CARTESIAN_POINT ( 'NONE',  ( -16.85913248346849969, 1508.551704408389924, 212.7777254685370281 ) ) ;
#9982=CARTESIAN_POINT ( 'NONE',  ( 4.617353517619999792, 1460.098150474590057, 228.0971968620989969 ) ) ;
#9983=CARTESIAN_POINT ( 'NONE',  ( -9.526124601274780446, 1440.436526369470130, 205.9994947568980024 ) ) ;
#9991=ORIENTED_EDGE ( 'NONE', *, *, #87778, .T. ) ;
#10003=ORIENTED_EDGE ( 'NONE', *, *, #22726, .F. ) ;
#10004=CARTESIAN_POINT ( 'NONE',  ( 1.167418783940000093, 1444.307247415689972, 215.3110397704089962 ) ) ;
#10007=ORIENTED_EDGE ( 'NONE', *, *, #58613, .F. ) ;
#10008=CARTESIAN_POINT ( 'NONE',  ( 3.865424752145830034, 1508.610338626970133, 204.7110934638159847 ) ) ;
#10010=B_SPLINE_SURFACE_WITH_KNOTS ( 'NONE', 5, 5, ( 
 ( #44122, #44679, #104007, #27304, #79375, #20003 ),
 ( #103441, #54195, #36814, #28973, #71570, #105691 ),
 ( #78257, #88322, #79927, #51967, #86108, #9402 ),
 ( #63698, #98911, #91060, #88872, #89965, #48537 ),
 ( #30615, #64802, #21638, #90512, #73176, #55291 ),
 ( #81019, #29504, #47429, #21087, #97809, #81552 ) ),
 .UNSPECIFIED., .F., .F., .F.,
 ( 6, 6 ),
 ( 6, 6 ),
 ( 7.080340024990000813, 12.74512986790000113 ),
 ( 0.000000000000000000, 2.000000000000000000 ),
 .UNSPECIFIED. ) ;
#10015=CARTESIAN_POINT ( 'NONE',  ( -3.490466736259999703, 1496.905313612590135, 198.4270292345989901 ) ) ;
#10017=CARTESIAN_POINT ( 'NONE',  ( -3.208637323093683769, 1515.551704408389924, 205.2922258736341519 ) ) ;
#10024=ORIENTED_EDGE ( 'NONE', *, *, #50153, .F. ) ;
#10025=CARTESIAN_POINT ( 'NONE',  ( -17.37965410361753982, 1465.838514868465154, 219.1858979602013164 ) ) ;
#10026=CARTESIAN_POINT ( 'NONE',  ( -2.940338105849999994, 1463.323050212790122, 228.6636231251989955 ) ) ;
#10029=AXIS2_PLACEMENT_3D ( 'NONE', #12417, #46602, #4045 ) ;
#10030=CARTESIAN_POINT ( 'NONE',  ( -21.12854634993719927, 1507.715432715349834, 209.4790063854959783 ) ) ;
#10032=CARTESIAN_POINT ( 'NONE',  ( -4.328818125147580353, 1515.088876468550097, 207.8567422199149917 ) ) ;
#10037=DIRECTION ( 'NONE',  ( 0.9980318515193558060, 0.000000000000000000, 0.06270903725019710828 ) ) ;
#10039=CARTESIAN_POINT ( 'NONE',  ( -17.69729716890000049, 1420.080679157370014, 207.3677048410189911 ) ) ;
#10040=CARTESIAN_POINT ( 'NONE',  ( 9.627620378001870094, 1463.988716367230154, 211.0622702830050059 ) ) ;
#10045=CARTESIAN_POINT ( 'NONE',  ( -15.99542386634146851, 1420.238047865418366, 209.6726076052734982 ) ) ;
#10048=CARTESIAN_POINT ( 'NONE',  ( 22.24401333792100033, 1475.958618154809983, 209.7631869422630189 ) ) ;
#10050=CARTESIAN_POINT ( 'NONE',  ( 2173.981453289206911, -8382.262153571264207, -1556.947849745907888 ) ) ;
#10051=CARTESIAN_POINT ( 'NONE',  ( 9.173643782033812144, 1450.994954104630096, 210.2665090766199683 ) ) ;
#10052=CARTESIAN_POINT ( 'NONE',  ( 3.991437517280000513, 1441.662116857989986, 217.1481707352390060 ) ) ;
#10056=EDGE_CURVE ( 'NONE', #76758, #20056, #98578, .T. ) ;
#10060=CARTESIAN_POINT ( 'NONE',  ( 3.217406951622789890, 1424.184472523990053, 188.9579968088540056 ) ) ;
#10061=EDGE_LOOP ( 'NONE', ( #103361, #87408, #19164 ) ) ;
#10066=CARTESIAN_POINT ( 'NONE',  ( -0.7593982673170009967, 1430.316802068590050, 217.4503154216889982 ) ) ;
#10067=CARTESIAN_POINT ( 'NONE',  ( -10.52582819352379850, 1471.840167648990018, 206.9753088315659966 ) ) ;
#10073=ORIENTED_EDGE ( 'NONE', *, *, #7158, .T. ) ;
#10074=CARTESIAN_POINT ( 'NONE',  ( 11.26469520917990152, 1491.013796966650261, 207.1901082836730268 ) ) ;
#10076=CARTESIAN_POINT ( 'NONE',  ( -3.381226883360950008, 1438.609729080699935, 227.4063576580390134 ) ) ;
#10077=ORIENTED_EDGE ( 'NONE', *, *, #19715, .T. ) ;
#10082=CARTESIAN_POINT ( 'NONE',  ( -2.599202470067710102, 1495.843114574169931, 197.0638286399839672 ) ) ;
#10091=CARTESIAN_POINT ( 'NONE',  ( -19.58495063083499943, 1485.885833950319920, 202.2948491896230223 ) ) ;
#10095=DIRECTION ( 'NONE',  ( -0.9990982087154917091, 0.04245902717575712748, -1.878255039611807006E-05 ) ) ;
#10097=CARTESIAN_POINT ( 'NONE',  ( -3.156992497350000093, 1496.318815817190170, 220.0352492536989928 ) ) ;
#10098=ORIENTED_EDGE ( 'NONE', *, *, #17104, .F. ) ;
#10100=CIRCLE ( 'NONE', #80187, 830.3529813948301808 ) ;
#10102=ORIENTED_EDGE ( 'NONE', *, *, #29058, .F. ) ;
#10114=CARTESIAN_POINT ( 'NONE',  ( -5.263807122380000258, 1391.914765277889956, 214.5215612962889793 ) ) ;
#10118=CARTESIAN_POINT ( 'NONE',  ( 9.146190246725058870, 1461.862305004799964, 205.8338018421410140 ) ) ;
#10119=AXIS2_PLACEMENT_3D ( 'NONE', #88643, #64001, #56680 ) ;
#10124=CARTESIAN_POINT ( 'NONE',  ( -2.298816259811510054, 1486.462377102800019, 220.8289805423670202 ) ) ;
#10132=( BOUNDED_CURVE ( )  B_SPLINE_CURVE ( 3, ( #94748, #7437, #58406, #33728 ),
 .UNSPECIFIED., .F., .F. ) 
 B_SPLINE_CURVE_WITH_KNOTS ( ( 4, 4 ),
 ( 4.152341638222174502, 5.272436418961190085 ),
 .UNSPECIFIED. ) 
 CURVE ( )  GEOMETRIC_REPRESENTATION_ITEM ( )  RATIONAL_B_SPLINE_CURVE ( ( 1.000000000000000000, 0.8981532913012172381, 0.8981532913012172381, 1.000000000000000000 ) ) 
 REPRESENTATION_ITEM ( '' )  );
#10133=CARTESIAN_POINT ( 'NONE',  ( 6.361972252410000195, 1462.343751617889893, 207.5519484895090159 ) ) ;
#10141=VERTEX_POINT ( 'NONE', #75142 ) ;
#10143=CARTESIAN_POINT ( 'NONE',  ( -7.116759930024330494, 1508.500068961840043, 219.5125775166329731 ) ) ;
#10145=CARTESIAN_POINT ( 'NONE',  ( -3.774544273728137611, 1488.811965616022462, 219.3433275354165062 ) ) ;
#10148=CARTESIAN_POINT ( 'NONE',  ( 9.167247559838790139, 1450.084797855079842, 208.2842279015860072 ) ) ;
#10149=CARTESIAN_POINT ( 'NONE',  ( -12.71213581786250124, 1502.313795877750181, 210.3224788360479920 ) ) ;
#10150=CARTESIAN_POINT ( 'NONE',  ( 11.16440858570000039, 1492.931605700189948, 213.3458366114890055 ) ) ;
#10153=CARTESIAN_POINT ( 'NONE',  ( -21.15335024929999719, 1505.792763867390022, 209.1590586292889782 ) ) ;
#10156=CARTESIAN_POINT ( 'NONE',  ( -9.966727850805121136, 1439.480327375449860, 208.4309914983489875 ) ) ;
#10163=CARTESIAN_POINT ( 'NONE',  ( 4.253676957470000630, 1505.389161788490128, 221.1607250897990014 ) ) ;
#10166=CARTESIAN_POINT ( 'NONE',  ( 0.1187972039649769912, 1515.157712620099801, 204.7948303746160263 ) ) ;
#10168=CARTESIAN_POINT ( 'NONE',  ( -15.86842751682814701, 1415.926969301026702, 209.7305162940345440 ) ) ;
#10170=CARTESIAN_POINT ( 'NONE',  ( -16.28210776099999890, 1416.583347678280006, 208.7674903396639934 ) ) ;
#10171=CARTESIAN_POINT ( 'NONE',  ( 1.804110352077529900, 1431.051163599219990, 199.8239164788810172 ) ) ;
#10177=CARTESIAN_POINT ( 'NONE',  ( -10.12886798639999952, 1479.735562891690051, 213.4664817790389861 ) ) ;
#10194=CARTESIAN_POINT ( 'NONE',  ( 18.13448186070239743, 1429.411014922339973, 207.6636477268740180 ) ) ;
#10199=CARTESIAN_POINT ( 'NONE',  ( -13.36486944082299999, 1507.695946242639820, 209.3487293561690024 ) ) ;
#10204=CARTESIAN_POINT ( 'NONE',  ( -16.43158050010680071, 1420.644938884899830, 203.2808245233400157 ) ) ;
#10216=CARTESIAN_POINT ( 'NONE',  ( 3.305606196530000318, 1485.263013345289892, 219.7395598687990059 ) ) ;
#10217=CARTESIAN_POINT ( 'NONE',  ( 4.461246620899999904, 1423.870484961680177, 193.5243008840990058 ) ) ;
#10219=CARTESIAN_POINT ( 'NONE',  ( 10.26657504319999958, 1453.676195443890037, 189.9132845388990063 ) ) ;
#10221=CARTESIAN_POINT ( 'NONE',  ( 4.803828466469020064, 1471.771541183390127, 187.6888343885629808 ) ) ;
#10224=CARTESIAN_POINT ( 'NONE',  ( -4.992905603179999652, 1391.642136302990139, 203.5786559967189930 ) ) ;
#10226=CARTESIAN_POINT ( 'NONE',  ( -12.07474050270000099, 1489.840319478090123, 211.0992678051489690 ) ) ;
#10234=FACE_OUTER_BOUND ( 'NONE', #84043, .T. ) ;
#10243=CARTESIAN_POINT ( 'NONE',  ( -1.682067311822292632, 1456.930731614571641, 199.7658281152051529 ) ) ;
#10249=CARTESIAN_POINT ( 'NONE',  ( -1.811578048269999908, 1468.887281251189961, 219.1129677655590058 ) ) ;
#10253=CARTESIAN_POINT ( 'NONE',  ( -4.507044386543670456, 1426.351334971300048, 208.6001660766199848 ) ) ;
#10255=VERTEX_POINT ( 'NONE', #31459 ) ;
#10263=AXIS2_PLACEMENT_3D ( 'NONE', #19096, #70671, #79055 ) ;
#10264=CARTESIAN_POINT ( 'NONE',  ( -4.240938962173256499, 1509.032014554845546, 205.3774795649941893 ) ) ;
#10265=CARTESIAN_POINT ( 'NONE',  ( 9.878689728610000387, 1462.081439766189987, 209.0598259307259923 ) ) ;
#10266=CARTESIAN_POINT ( 'NONE',  ( 11.27370387821760112, 1422.118576165349850, 210.3076253712490029 ) ) ;
#10272=ORIENTED_EDGE ( 'NONE', *, *, #73711, .F. ) ;
#10279=CARTESIAN_POINT ( 'NONE',  ( 2.950090637770019786, 1423.648712310149904, 192.7546880243370140 ) ) ;
#10285=DIRECTION ( 'NONE',  ( -3.884000507300682969E-06, 0.9999999999895848868, -2.396820608630749728E-06 ) ) ;
#10288=CARTESIAN_POINT ( 'NONE',  ( -3.035907725099100229, 1428.901055825690037, 200.2600137390959958 ) ) ;
#10294=CARTESIAN_POINT ( 'NONE',  ( -11.76331282408339973, 1482.371198147200175, 207.3261823526030128 ) ) ;
#10307=LINE ( 'NONE', #44480, #82344 ) ;
#10311=VERTEX_POINT ( 'NONE', #109289 ) ;
#10313=CARTESIAN_POINT ( 'NONE',  ( -9.821428347282159521, 1508.436132293389846, 218.8451730364450043 ) ) ;
#10318=CARTESIAN_POINT ( 'NONE',  ( 3.826592460210000102, 1468.046643628590118, 218.3510257011089948 ) ) ;
#10319=CARTESIAN_POINT ( 'NONE',  ( -0.5374665116262267173, 1469.511926925009675, 219.1609941224751879 ) ) ;
#10323=CARTESIAN_POINT ( 'NONE',  ( -1.393502785639999964, 1429.966547008989892, 200.2027313623789837 ) ) ;
#10325=CARTESIAN_POINT ( 'NONE',  ( 2.994526374120000334, 1506.310361900689941, 220.7972505012990041 ) ) ;
#10326=EDGE_CURVE ( 'NONE', #62781, #95904, #82969, .T. ) ;
#10332=CARTESIAN_POINT ( 'NONE',  ( 10.32070371839930090, 1469.846300739589879, 207.1845276051559779 ) ) ;
#10334=CARTESIAN_POINT ( 'NONE',  ( 12.26027809410000025, 1500.839094156290230, 209.5442590651630326 ) ) ;
#10342=B_SPLINE_CURVE_WITH_KNOTS ( 'NONE', 5,
 ( #57880, #75231, #42721, #33200, #66836, #68489 ),
 .UNSPECIFIED., .F., .F.,
 ( 6, 6 ),
 ( 0.000000000000000000, 1.000000000000000000 ),
 .UNSPECIFIED. ) ;
#10343=VERTEX_POINT ( 'NONE', #640 ) ;
#10344=B_SPLINE_CURVE_WITH_KNOTS ( 'NONE', 3,
 ( #102451, #59939, #94056, #17324, #61592, #27969, #105235, #70008, #27410, #11722, #95725, #19557, #103565, #20111, #87330, #60487, #62153, #62723, #43672, #70557, #96844, #77825, #104675, #78377, #1133, #1684, #104122, #95177, #54304, #26867, #35825, #45350, #18990, #35263, #71111, #69448, #96280, #53763, #88432, #61055, #87897, #3351, #18433, #11188, #53188, #52633 ),
 .UNSPECIFIED., .F., .F.,
 ( 4, 3, 3, 3, 3, 3, 3, 3, 3, 3, 3, 3, 3, 3, 3, 4 ),
 ( 8.670147881838009580E-05, 0.4789285211775260453, 0.9744792269830828690, 1.259346753059999990, 1.776261645606839856, 2.325059878702980143, 2.711818916799999979, 3.323520562006709866, 4.028423604586089724, 4.918128909075430322, 5.564709931820000399, 7.179393063629159855, 8.369582197274629820, 9.352558316332389765, 10.31444422860000110, 10.41999860509999998 ),
 .UNSPECIFIED. ) ;
#10348=CARTESIAN_POINT ( 'NONE',  ( -6.753153240240000521, 1472.181002690289915, 210.7318518582290210 ) ) ;
#10355=CARTESIAN_POINT ( 'NONE',  ( -8.635302540649998804, 1451.543452603389824, 205.3798752934189906 ) ) ;
#10358=CARTESIAN_POINT ( 'NONE',  ( 7.574305215059999874, 1424.934277763670025, 212.0912061558890116 ) ) ;
#10359=CARTESIAN_POINT ( 'NONE',  ( 20.10528729609999843, 1430.878053336090034, 215.1856554784289983 ) ) ;
#10365=VERTEX_POINT ( 'NONE', #87390 ) ;
#10372=CARTESIAN_POINT ( 'NONE',  ( -3.152270375085599596, 1474.954422185709745, 198.1306180807430053 ) ) ;
#10380=ORIENTED_EDGE ( 'NONE', *, *, #84388, .F. ) ;
#10387=CARTESIAN_POINT ( 'NONE',  ( -3.757047865440000134, 1455.840493388089953, 200.4411851703590060 ) ) ;
#10389=AXIS2_PLACEMENT_3D ( 'NONE', #106748, #40100, #64790 ) ;
#10395=ORIENTED_EDGE ( 'NONE', *, *, #108900, .F. ) ;
#10413=CARTESIAN_POINT ( 'NONE',  ( -14.47516141776405618, 1416.049748536053812, 214.4146204850279673 ) ) ;
#10421=EDGE_CURVE ( 'NONE', #67895, #11716, #87271, .T. ) ;
#10430=CARTESIAN_POINT ( 'NONE',  ( -3.246589359020000121, 1430.595539088089936, 201.4224038467990283 ) ) ;
#10434=CARTESIAN_POINT ( 'NONE',  ( 3.436085222180000454, 1486.341472188189982, 198.7604664416990090 ) ) ;
#10435=CARTESIAN_POINT ( 'NONE',  ( 11.09565341729999943, 1425.086740399749942, 203.0248198978989933 ) ) ;
#10437=ADVANCED_FACE ( 'NONE', ( #5017 ), #13194, .T. ) ;
#10450=CARTESIAN_POINT ( 'NONE',  ( 3.087555757030000070, 1443.150514725890162, 217.4716940151990059 ) ) ;
#10463=CARTESIAN_POINT ( 'NONE',  ( -4.487359741654690204, 1509.034536824670113, 212.2379826147090114 ) ) ;
#10469=ADVANCED_FACE ( 'NONE', ( #40273 ), #66061, .T. ) ;
#10471=CARTESIAN_POINT ( 'NONE',  ( -11.24296408042640039, 1470.377897305100078, 210.9233862662850072 ) ) ;
#10474=CARTESIAN_POINT ( 'NONE',  ( -10.90534521260189926, 1489.991766825829927, 212.3803483885259880 ) ) ;
#10475=CARTESIAN_POINT ( 'NONE',  ( -4.326992699989999913, 1515.158586642790169, 209.1218459619010162 ) ) ;
#10487=EDGE_LOOP ( 'NONE', ( #50130, #15215, #12191, #47685 ) ) ;
#10494=CARTESIAN_POINT ( 'NONE',  ( 8.644428848947828925, 1437.072346058449739, 209.1799678029250060 ) ) ;
#10496=CARTESIAN_POINT ( 'NONE',  ( -0.1934954855810029906, 1481.263391716890055, 229.6341570919989863 ) ) ;
#10499=CARTESIAN_POINT ( 'NONE',  ( -2.363918620589999797, 1443.448698872290151, 218.8950620034389942 ) ) ;
#10503=CARTESIAN_POINT ( 'NONE',  ( -11.17515840243070002, 1423.345794038340046, 204.2560692912300055 ) ) ;
#10508=CARTESIAN_POINT ( 'NONE',  ( 18.40700370933230090, 1472.577248366799722, 195.0927350935599804 ) ) ;
#10513=CARTESIAN_POINT ( 'NONE',  ( 4.329448776040000446, 1515.064792882589927, 210.9648081929590262 ) ) ;
#10517=CARTESIAN_POINT ( 'NONE',  ( -7.649433525730000127, 1459.248781285089990, 215.2925678204190092 ) ) ;
#10520=CARTESIAN_POINT ( 'NONE',  ( -11.87328871660000118, 1482.014094933990009, 208.6022274357210051 ) ) ;
#10522=CARTESIAN_POINT ( 'NONE',  ( -8.467016979619998551, 1423.717407386009882, 209.4627668193359966 ) ) ;
#10526=CARTESIAN_POINT ( 'NONE',  ( -11.16643434163729864, 1471.372555858320084, 206.7508257846899937 ) ) ;
#10534=CARTESIAN_POINT ( 'NONE',  ( 10.13545575494789830, 1453.511789163979984, 212.2748783515349942 ) ) ;
#10535=CARTESIAN_POINT ( 'NONE',  ( 1.925781382208645587, 1487.138807670421329, 219.7730072395593766 ) ) ;
#10536=CARTESIAN_POINT ( 'NONE',  ( -19.02872918048390005, 1508.494693425979904, 209.9678762690199960 ) ) ;
#10538=CARTESIAN_POINT ( 'NONE',  ( 7.261898129199999552, 1472.764678900990020, 216.9089656813590068 ) ) ;
#10539=CARTESIAN_POINT ( 'NONE',  ( 17.68711869539999881, 1428.828027849089949, 204.9896315466789929 ) ) ;
#10544=CARTESIAN_POINT ( 'NONE',  ( 9.357230663576631358, 1435.432546474700075, 208.4556945073640009 ) ) ;
#10548=ORIENTED_EDGE ( 'NONE', *, *, #16459, .F. ) ;
#10566=ORIENTED_EDGE ( 'NONE', *, *, #4155, .F. ) ;
#10568=ADVANCED_FACE ( 'NONE', ( #2175 ), #41838, .T. ) ;
#10581=VECTOR ( 'NONE', #36414, 1000.000000000000114 ) ;
#10586=CARTESIAN_POINT ( 'NONE',  ( -16.91437751779999843, 1417.214263006909960, 207.5096583893090099 ) ) ;
#10589=EDGE_CURVE ( 'NONE', #100027, #45257, #41257, .T. ) ;
#10591=CARTESIAN_POINT ( 'NONE',  ( 5.145309177750649887, 1422.426130283250131, 194.5914460530619863 ) ) ;
#10594=CARTESIAN_POINT ( 'NONE',  ( -14.48519483975229960, 1416.181292564900104, 203.8595933512790168 ) ) ;
#10598=CARTESIAN_POINT ( 'NONE',  ( -14.50129934600000148, 1422.728001101090058, 196.3816483097989760 ) ) ;
#10602=CARTESIAN_POINT ( 'NONE',  ( -11.60387536552270049, 1481.105535834539978, 211.4044418330699955 ) ) ;
#10606=B_SPLINE_CURVE_WITH_KNOTS ( 'NONE', 3,
 ( #105241, #35272, #104131, #27976, #44801, #61066, #44240, #87337, #62160, #18997, #17333, #69458, #10067, #1693, #53196, #2261, #51528, #60497, #36375, #70564, #105806, #29086, #107982, #21191, #12822, #88441, #38570, #80592, #47545, #72747, #56499, #81665, #37484, #11732 ),
 .UNSPECIFIED., .F., .F.,
 ( 4, 3, 3, 3, 3, 3, 3, 3, 3, 3, 3, 4 ),
 ( -1.999999989989980076, -1.861718069389969976, -1.678534718961790073, -1.493099238245260141, -1.306486601231749978, -1.118423644982459830, -0.9299498955213489904, -0.7415292143806480052, -0.5536198130809719675, -0.3674063791434580839, -0.1827794707570640220, 0.000000000000000000 ),
 .UNSPECIFIED. ) ;
#10610=CARTESIAN_POINT ( 'NONE',  ( -16.46732193653928533, 1420.114675349507934, 208.7316782250878191 ) ) ;
#10616=CARTESIAN_POINT ( 'NONE',  ( -234.5897387251999930, 11221.53578756869865, 2175.945776423289772 ) ) ;
#10618=CARTESIAN_POINT ( 'NONE',  ( 4.253777714910000007, 1442.471859903390168, 216.9083338397390150 ) ) ;
#10626=CARTESIAN_POINT ( 'NONE',  ( -16.83566012920760002, 1418.884382950350073, 201.2565057074210131 ) ) ;
#10629=CARTESIAN_POINT ( 'NONE',  ( 5.440512190109999757, 1424.738065781850082, 191.9794586101990319 ) ) ;
#10632=CARTESIAN_POINT ( 'NONE',  ( -14.65245215464970130, 1420.119839417710182, 213.8659310620899987 ) ) ;
#10641=CARTESIAN_POINT ( 'NONE',  ( 12.32715944251560103, 1492.190983864200007, 209.5901420063510159 ) ) ;
#10664=CARTESIAN_POINT ( 'NONE',  ( 0.2999317787290010084, 1497.191549081989933, 197.4584646491989872 ) ) ;
#10678=CARTESIAN_POINT ( 'NONE',  ( 2.931762418139999937, 1484.928921319690062, 220.6147940381989940 ) ) ;
#10684=CARTESIAN_POINT ( 'NONE',  ( 10.08864075595840148, 1461.294693056749793, 208.2010832468129991 ) ) ;
#10689=CARTESIAN_POINT ( 'NONE',  ( 7.184880219700001014, 1423.497618239299982, 195.4521118202989953 ) ) ;
#10696=CARTESIAN_POINT ( 'NONE',  ( 9.201640575826802504, 1450.639316510839990, 208.3453033095780143 ) ) ;
#10706=ORIENTED_EDGE ( 'NONE', *, *, #89828, .F. ) ;
#10709=CARTESIAN_POINT ( 'NONE',  ( -3.523962699983150149, 1476.511731499819916, 220.0526012347959863 ) ) ;
#10710=CARTESIAN_POINT ( 'NONE',  ( -9.959969825530610166, 1470.547643313240087, 212.5949768734770089 ) ) ;
#10715=CARTESIAN_POINT ( 'NONE',  ( -7.192114391989999689, 1473.717433820989982, 200.7095979941090036 ) ) ;
#10716=CARTESIAN_POINT ( 'NONE',  ( 11.01187558969999891, 1492.459055990190109, 212.4069249470189789 ) ) ;
#10718=CARTESIAN_POINT ( 'NONE',  ( 8.708214553643372824, 1424.815002788605398, 195.6916425196928913 ) ) ;
#10719=CARTESIAN_POINT ( 'NONE',  ( -14.29847877429999947, 1503.225636699989991, 208.9837668400270161 ) ) ;
#10720=CARTESIAN_POINT ( 'NONE',  ( 10.59718513049560151, 1469.650899207149905, 205.1638397631170108 ) ) ;
#10728=EDGE_CURVE ( 'NONE', #41661, #42951, #49671, .T. ) ;
#10732=CARTESIAN_POINT ( 'NONE',  ( -1.379638663386490105, 1515.081065330719866, 204.7928232953929921 ) ) ;
#10734=DIRECTION ( 'NONE',  ( -0.02616798426450838572, -0.9993150019883944024, 0.02616798426450848286 ) ) ;
#10737=CARTESIAN_POINT ( 'NONE',  ( -19.75056259240000145, 1465.177823603190063, 209.1218459616989946 ) ) ;
#10744=CARTESIAN_POINT ( 'NONE',  ( 9.799773730352699275, 1469.816546466489854, 211.4317690604339930 ) ) ;
#10745=DIRECTION ( 'NONE',  ( -7.363503285428202099E-05, 3.211508572083940804E-06, 0.9999999972837841922 ) ) ;
#10754=CARTESIAN_POINT ( 'NONE',  ( 0.7941283559409979542, 1479.063403849489987, 229.6081502463990205 ) ) ;
#10756=CARTESIAN_POINT ( 'NONE',  ( -11.33475729453610192, 1500.341569088609958, 210.4138246906279903 ) ) ;
#10760=CARTESIAN_POINT ( 'NONE',  ( -16.32619598790000026, 1416.471320734319988, 209.2727045491550086 ) ) ;
#10770=CARTESIAN_POINT ( 'NONE',  ( -11.60387536552270049, 1481.105535834539978, 211.4044418330699955 ) ) ;
#10777=CARTESIAN_POINT ( 'NONE',  ( -5.387811863060000483, 1496.648312753189884, 199.2595355468089906 ) ) ;
#10784=CARTESIAN_POINT ( 'NONE',  ( 3.226607219819999539, 1423.257519486769979, 193.6078189732990040 ) ) ;
#10787=B_SPLINE_SURFACE_WITH_KNOTS ( 'NONE', 5, 5, ( 
 ( #109416, #22597, #59015, #39440, #99323, #24811 ),
 ( #101523, #41090, #107744, #32141, #57374, #74165 ),
 ( #92047, #56800, #14224, #48410, #100981, #75267 ),
 ( #84736, #50062, #82554, #91501, #109957, #108295 ),
 ( #73616, #23174, #93142, #33235, #58457, #48966 ),
 ( #108845, #100445, #66872, #84189, #66327, #23728 ),
 ( #24276, #57914, #15319, #49513, #83637, #92585 ),
 ( #15856, #7488, #41649, #94807, #52823, #59561 ),
 ( #17514, #51156, #18625, #95363, #51712, #26486 ) ),
 .UNSPECIFIED., .F., .F., .F.,
 ( 6, 3, 6 ),
 ( 6, 6 ),
 ( 3.918736331710000353, 7.747513759300000302, 12.84118059900000119 ),
 ( 0.000000000000000000, 2.000000000000000000 ),
 .UNSPECIFIED. ) ;
#10789=CARTESIAN_POINT ( 'NONE',  ( 19.03958482845590083, 1453.804128677390054, 200.7927815628769963 ) ) ;
#10795=CARTESIAN_POINT ( 'NONE',  ( -10.94181931979999867, 1491.470369003389806, 210.4086029903089923 ) ) ;
#10798=CARTESIAN_POINT ( 'NONE',  ( 10.36616749849999941, 1462.084512446189819, 211.0499673381089849 ) ) ;
#10802=CARTESIAN_POINT ( 'NONE',  ( 6.392991367490600041, 1505.880701581259927, 218.9074644499650049 ) ) ;
#10803=CARTESIAN_POINT ( 'NONE',  ( -9.710888762612963632, 1422.734008549482496, 210.6841274085994655 ) ) ;
#10809=ORIENTED_EDGE ( 'NONE', *, *, #43900, .T. ) ;
#10815=FACE_OUTER_BOUND ( 'NONE', #97138, .T. ) ;
#10826=CARTESIAN_POINT ( 'NONE',  ( -4.682234856550000046, 1438.893385222290135, 227.1256850459990062 ) ) ;
#10832=CIRCLE ( 'NONE', #87719, 0.5000000000000032196 ) ;
#10835=B_SPLINE_CURVE_WITH_KNOTS ( 'NONE', 3,
 ( #51786, #33300, #15935, #34419, #83715, #85925, #67495, #101599, #66396, #16481, #58535, #25441, #50671, #68592, #59634, #15395, #100516, #57984, #293 ),
 .UNSPECIFIED., .F., .F.,
 ( 4, 2, 2, 2, 1, 1, 1, 2, 2, 2, 4 ),
 ( 0.000000000000000000, 0.2500000000001726952, 0.3750000000002590150, 0.4375000000003022027, 0.4687500000003208545, 0.4843750000003272937, 0.4921875000003335665, 0.4960937500003307354, 0.5000000000003279599, 0.7500000000001639799, 1.000000000000000000 ),
 .UNSPECIFIED. ) ;
#10836=CARTESIAN_POINT ( 'NONE',  ( 0.8459567068543710766, 1465.606436347200088, 198.1403988231419930 ) ) ;
#10840=CARTESIAN_POINT ( 'NONE',  ( 8.559858904628349308, 1437.030483964089854, 207.9845584131589931 ) ) ;
#10853=CARTESIAN_POINT ( 'NONE',  ( 3.654206417870119683, 1423.822803498439953, 192.8935211664289966 ) ) ;
#10863=EDGE_CURVE ( 'NONE', #109438, #104137, #99132, .T. ) ;
#10874=CARTESIAN_POINT ( 'NONE',  ( 10.19356100915574714, 1482.603900002795854, 212.2173956555756149 ) ) ;
#10886=B_SPLINE_CURVE_WITH_KNOTS ( 'NONE', 5,
 ( #83929, #90670, #82824, #7231, #6116, #75556 ),
 .UNSPECIFIED., .F., .F.,
 ( 6, 6 ),
 ( -2.000000000000000000, 0.000000000000000000 ),
 .UNSPECIFIED. ) ;
#10889=CARTESIAN_POINT ( 'NONE',  ( -19.37335128149999974, 1466.648676094589746, 213.3177732612090267 ) ) ;
#10894=CARTESIAN_POINT ( 'NONE',  ( 0.6849490657429989637, 1506.697984446489954, 221.5403866999990043 ) ) ;
#10895=CARTESIAN_POINT ( 'NONE',  ( -4.324092179320000007, 1515.269353058490196, 209.1218459616989946 ) ) ;
#10896=VECTOR ( 'NONE', #60189, 999.9999999999998863 ) ;
#10897=EDGE_LOOP ( 'NONE', ( #99101, #24826, #21650, #92396 ) ) ;
#10899=FACE_OUTER_BOUND ( 'NONE', #23564, .T. ) ;
#10900=CARTESIAN_POINT ( 'NONE',  ( 3.281448589401000149, 1466.303082592839928, 198.5677341052449947 ) ) ;
#10914=CARTESIAN_POINT ( 'NONE',  ( -5.832233384169380308, 1490.191062745069985, 214.8994725848050109 ) ) ;
#10916=CARTESIAN_POINT ( 'NONE',  ( -11.41143408916500412, 1500.995514667651150, 208.5044259995214588 ) ) ;
#10918=CARTESIAN_POINT ( 'NONE',  ( -8.190304664959999315, 1512.060957492389889, 212.0841603871389793 ) ) ;
#10922=CARTESIAN_POINT ( 'NONE',  ( -8.154782393420001441, 1452.666828378989749, 204.3290871732590119 ) ) ;
#10924=CARTESIAN_POINT ( 'NONE',  ( 7.528870192820000362, 1425.840869188159786, 212.2336632603989983 ) ) ;
#10925=CARTESIAN_POINT ( 'NONE',  ( -16.53114558859999761, 1465.611456236089907, 220.7423132190989747 ) ) ;
#10930=CARTESIAN_POINT ( 'NONE',  ( 6.261024423890000357, 1453.731044942389872, 216.1357478295089720 ) ) ;
#10937=CARTESIAN_POINT ( 'NONE',  ( 5.514426304880457153, 1499.747148894430666, 199.1702447789172652 ) ) ;
#10943=EDGE_CURVE ( 'NONE', #23318, #17806, #103106, .T. ) ;
#10949=CARTESIAN_POINT ( 'NONE',  ( -14.01525996361490023, 1415.677402202029953, 204.0303134510289738 ) ) ;
#10951=DIRECTION ( 'NONE',  ( -0.6147312344637360093, -0.2401348534948875013, -0.7512927269125400098 ) ) ;
#10955=CARTESIAN_POINT ( 'NONE',  ( -3.866699731040000199, 1454.806985439190157, 200.4000761353790097 ) ) ;
#10961=CARTESIAN_POINT ( 'NONE',  ( 7.868158389100000427, 1422.937290482379922, 214.1570520181289794 ) ) ;
#10965=CARTESIAN_POINT ( 'NONE',  ( -11.76016211164009917, 1489.518188874960060, 212.3895637392580227 ) ) ;
#10980=CARTESIAN_POINT ( 'NONE',  ( 11.84876590452089928, 1426.365912190949985, 195.4914265713040038 ) ) ;
#10989=CIRCLE ( 'NONE', #100415, 0.9999999999998898659 ) ;
#11001=CARTESIAN_POINT ( 'NONE',  ( 9.922877777048348946, 1468.601600206289959, 207.7732624088289981 ) ) ;
#11010=CARTESIAN_POINT ( 'NONE',  ( 2.234896868229169886, 1424.004436568589881, 191.3087619182109904 ) ) ;
#11018=CARTESIAN_POINT ( 'NONE',  ( 12.03449227190490056, 1491.353386486839781, 206.6667661091970274 ) ) ;
#11021=ORIENTED_EDGE ( 'NONE', *, *, #56328, .T. ) ;
#11024=ORIENTED_EDGE ( 'NONE', *, *, #5309, .F. ) ;
#11027=CARTESIAN_POINT ( 'NONE',  ( -2.363461299099999913, 1483.719072616789845, 198.7034185567990221 ) ) ;
#11034=CARTESIAN_POINT ( 'NONE',  ( -11.30600794628579919, 1470.458368520040040, 210.5249131588269904 ) ) ;
#11035=CARTESIAN_POINT ( 'NONE',  ( -9.980182751213080294, 1489.983213112079738, 214.0086324331080050 ) ) ;
#11036=CARTESIAN_POINT ( 'NONE',  ( 18.32584137559999959, 1473.764089050990151, 194.8973954003990059 ) ) ;
#11043=CARTESIAN_POINT ( 'NONE',  ( 4.709520687179999499, 1480.407452823689937, 228.9869292435990076 ) ) ;
#11053=CARTESIAN_POINT ( 'NONE',  ( 8.701117752674768724, 1436.141255594499853, 208.2914523929980248 ) ) ;
#11056=CARTESIAN_POINT ( 'NONE',  ( 2.801507340699999737, 1486.711793625290056, 216.6331940948190038 ) ) ;
#11062=CARTESIAN_POINT ( 'NONE',  ( -16.13494021775330367, 1420.788389406239958, 203.3274822485300035 ) ) ;
#11069=CARTESIAN_POINT ( 'NONE',  ( -21.26809730078759841, 1485.919095653640170, 201.7808411774039996 ) ) ;
#11082=CARTESIAN_POINT ( 'NONE',  ( -8.372769162319999126, 1460.069700419990113, 216.1743697456390123 ) ) ;
#11088=CARTESIAN_POINT ( 'NONE',  ( -9.241005602170000444, 1423.079004508810158, 209.8534315543390107 ) ) ;
#11098=VERTEX_POINT ( 'NONE', #36370 ) ;
#11105=CARTESIAN_POINT ( 'NONE',  ( -17.20083043329730188, 1508.455239297279832, 213.0365388520800138 ) ) ;
#11106=CARTESIAN_POINT ( 'NONE',  ( 6.734691585760000265, 1471.477077836790158, 216.7572454896890122 ) ) ;
#11113=CARTESIAN_POINT ( 'NONE',  ( 9.102815358048328420, 1434.837644414159968, 206.9573682008849858 ) ) ;
#11119=CARTESIAN_POINT ( 'NONE',  ( 2.015156349838810090, 1466.892420976849962, 219.9987159044960094 ) ) ;
#11132=ORIENTED_EDGE ( 'NONE', *, *, #70737, .T. ) ;
#11133=CARTESIAN_POINT ( 'NONE',  ( 4.038582018736556201, 1515.598601288561440, 208.8110691765281217 ) ) ;
#11153=EDGE_CURVE ( 'NONE', #34173, #67299, #90728, .T. ) ;
#11156=CARTESIAN_POINT ( 'NONE',  ( -4.329338606958669011, 1515.069000070069933, 207.5005477031000112 ) ) ;
#11162=CARTESIAN_POINT ( 'NONE',  ( -10.76604721355800010, 1461.751042529569986, 211.3391729738050060 ) ) ;
#11164=CARTESIAN_POINT ( 'NONE',  ( 14.09839856069999975, 1429.347419047090170, 194.9681440372989982 ) ) ;
#11167=CARTESIAN_POINT ( 'NONE',  ( 9.797638205384430421, 1462.858754388850002, 211.9411891193020097 ) ) ;
#11171=CARTESIAN_POINT ( 'NONE',  ( 12.35389624737000069, 1501.312344378229909, 211.6968100630580238 ) ) ;
#11174=CARTESIAN_POINT ( 'NONE',  ( -4.227540919128129460, 1441.218328383909920, 201.3833897788859986 ) ) ;
#11177=CARTESIAN_POINT ( 'NONE',  ( -4.240941581556870510, 1509.032042628840145, 205.3774810555430008 ) ) ;
#11179=CARTESIAN_POINT ( 'NONE',  ( -1970.025574498409924, -8382.262153571269664, 5.165967170900809258 ) ) ;
#11181=CARTESIAN_POINT ( 'NONE',  ( 3.962702341850000032, 1441.289781348989891, 217.4194346338989874 ) ) ;
#11184=EDGE_CURVE ( 'NONE', #81034, #76431, #2952, .T. ) ;
#11188=CARTESIAN_POINT ( 'NONE',  ( -2.176911324350150334, 1508.551704408389924, 220.0615420812520142 ) ) ;
#11194=CARTESIAN_POINT ( 'NONE',  ( 1.245014951509999968, 1431.187215948689982, 218.1259614198890233 ) ) ;
#11195=CARTESIAN_POINT ( 'NONE',  ( 1.842963446620166756, 1515.320037063702557, 213.3925623524362720 ) ) ;
#11197=CARTESIAN_POINT ( 'NONE',  ( 15.69667967640000050, 1457.921467858090182, 221.7535892932990009 ) ) ;
#11201=CARTESIAN_POINT ( 'NONE',  ( 10.97216364479129780, 1490.548997753850244, 208.6390587469809930 ) ) ;
#11202=CARTESIAN_POINT ( 'NONE',  ( -2.603171510209300266, 1438.442375251419890, 227.5216627168830144 ) ) ;
#11217=EDGE_CURVE ( 'NONE', #44333, #50492, #100541, .T. ) ;
#11224=EDGE_CURVE ( 'NONE', #36047, #86670, #46999, .T. ) ;
#11225=EDGE_CURVE ( 'NONE', #642, #5707, #71494, .T. ) ;
#11235=CARTESIAN_POINT ( 'NONE',  ( 2.713049553179999851, 1486.854776021489897, 219.6015362787990171 ) ) ;
#11237=CARTESIAN_POINT ( 'NONE',  ( -5.445054425793269814, 1494.866999379700246, 198.0707246423999948 ) ) ;
#11240=CARTESIAN_POINT ( 'NONE',  ( 11.59635154200000251, 1493.084219504590010, 213.4865999382489861 ) ) ;
#11246=CARTESIAN_POINT ( 'NONE',  ( 10.33893311465990017, 1453.276181934919805, 211.5205973212629829 ) ) ;
#11255=ORIENTED_EDGE ( 'NONE', *, *, #17225, .T. ) ;
#11257=CARTESIAN_POINT ( 'NONE',  ( 6.430565326490000011, 1462.522017996690010, 207.8657408012490180 ) ) ;
#11261=ORIENTED_EDGE ( 'NONE', *, *, #72032, .F. ) ;
#11264=ORIENTED_EDGE ( 'NONE', *, *, #34941, .F. ) ;
#11266=CARTESIAN_POINT ( 'NONE',  ( -5.996344191627310138, 1508.294791148050081, 220.1442991035219734 ) ) ;
#11268=CARTESIAN_POINT ( 'NONE',  ( -6.984424792645270053, 1470.560553081000307, 216.4904170223669837 ) ) ;
#11273=CARTESIAN_POINT ( 'NONE',  ( -2.225173971327330413, 1421.719837958959943, 193.4847570808190085 ) ) ;
#11276=CARTESIAN_POINT ( 'NONE',  ( -17.70278889250000276, 1504.268309054989913, 209.3612281098589847 ) ) ;
#11281=ORIENTED_EDGE ( 'NONE', *, *, #95346, .T. ) ;
#11286=CARTESIAN_POINT ( 'NONE',  ( -15.60316731140000002, 1415.677402317759970, 209.6305779890419956 ) ) ;
#11287=CARTESIAN_POINT ( 'NONE',  ( 12.89505231660000106, 1420.989630775359956, 203.4267439564690108 ) ) ;
#11292=CARTESIAN_POINT ( 'NONE',  ( 1.185810694231899998, 1430.833857439850135, 199.7444253494500117 ) ) ;
#11297=CARTESIAN_POINT ( 'NONE',  ( 1.332267629549999902E-15, 1412.913060387329779, 209.1218459616989946 ) ) ;
#11313=CARTESIAN_POINT ( 'NONE',  ( -15.57527174580000029, 1415.800173951010038, 208.9182627945979789 ) ) ;
#11322=CARTESIAN_POINT ( 'NONE',  ( -13.58464396841030108, 1508.551708197639755, 210.0579433922160035 ) ) ;
#11338=LINE ( 'NONE', #72354, #71257 ) ;
#11340=CARTESIAN_POINT ( 'NONE',  ( -0.2498415990399980025, 1420.995056578739877, 193.6850923126989983 ) ) ;
#11344=CARTESIAN_POINT ( 'NONE',  ( -3.152135748510000113, 1450.885091632490003, 188.5439271930990230 ) ) ;
#11348=CARTESIAN_POINT ( 'NONE',  ( -5.022927195390000321, 1391.808119929889926, 203.5626871977489998 ) ) ;
#11351=CARTESIAN_POINT ( 'NONE',  ( -11.80269316780000111, 1489.550427191690005, 212.2530852381789828 ) ) ;
#11359=CARTESIAN_POINT ( 'NONE',  ( 12.44781172279570036, 1501.268274303350154, 211.7240488200220341 ) ) ;
#11360=CARTESIAN_POINT ( 'NONE',  ( -11.56191713950926925, 1421.985365140208387, 210.6398819361144206 ) ) ;
#11373=CARTESIAN_POINT ( 'NONE',  ( -0.1544838608760010223, 1468.067337115490091, 219.5125637271989945 ) ) ;
#11377=CARTESIAN_POINT ( 'NONE',  ( -5.314640358949040078, 1425.825096639779986, 208.2911617466580196 ) ) ;
#11380=CARTESIAN_POINT ( 'NONE',  ( 5.140106207186420306, 1436.845544181910100, 228.7442480593620076 ) ) ;
#11382=ORIENTED_EDGE ( 'NONE', *, *, #2209, .F. ) ;
#11389=CARTESIAN_POINT ( 'NONE',  ( 2.632111276144470047, 1466.096714734490206, 198.4011313589680015 ) ) ;
#11397=ORIENTED_EDGE ( 'NONE', *, *, #633, .T. ) ;
#11413=CARTESIAN_POINT ( 'NONE',  ( -3.606501271529999997, 1507.464096719490044, 221.5253835883989950 ) ) ;
#11415=CARTESIAN_POINT ( 'NONE',  ( 5.469059239369999936, 1437.444982562589985, 208.6508151085089935 ) ) ;
#11421=CARTESIAN_POINT ( 'NONE',  ( -11.65753171920430020, 1482.533532356269916, 206.7098060248759737 ) ) ;
#11427=CARTESIAN_POINT ( 'NONE',  ( -6.944001484987491146, 1487.611668854129675, 219.0757229943065454 ) ) ;
#11428=CARTESIAN_POINT ( 'NONE',  ( -14.98950744470000096, 1415.677402218840143, 206.7597182584589746 ) ) ;
#11433=CARTESIAN_POINT ( 'NONE',  ( -10.22074380055929943, 1448.827829969109871, 207.2903289465359933 ) ) ;
#11438=CARTESIAN_POINT ( 'NONE',  ( -1.106162138419999996, 1515.349603040190004, 213.4044250793790241 ) ) ;
#11444=CARTESIAN_POINT ( 'NONE',  ( 3.601839739459999912, 1444.840594719589944, 200.9001243581789993 ) ) ;
#11451=VECTOR ( 'NONE', #64101, 1000.000000000000114 ) ;
#11452=CARTESIAN_POINT ( 'NONE',  ( 1.159696500349999937, 1485.109384876889862, 198.4167286540990176 ) ) ;
#11453=CARTESIAN_POINT ( 'NONE',  ( 9.406701834158939235, 1468.782307090909853, 204.4388643328819910 ) ) ;
#11460=B_SPLINE_SURFACE_WITH_KNOTS ( 'NONE', 5, 5, ( 
 ( #70864, #45652, #53490, #52934, #78672, #71421 ),
 ( #105537, #37777, #72488, #29903, #64095, #98217 ),
 ( #87070, #10355, #44526, #36125, #70309, #104422 ),
 ( #10922, #109397, #39419, #48391, #100426, #92029 ),
 ( #47824, #98769, #107726, #21485, #89819, #4711 ),
 ( #39969, #15300, #83078, #30463, #81959, #56228 ),
 ( #32124, #13092, #91481, #47276, #81399, #23709 ),
 ( #65191, #22578, #74146, #56782, #23155, #108276 ),
 ( #49493, #38854, #90920, #31564, #57893, #73033 ) ),
 .UNSPECIFIED., .F., .F., .F.,
 ( 6, 3, 6 ),
 ( 6, 6 ),
 ( 13.91937871330000043, 27.07797103040000053, 31.90163864219999823 ),
 ( 0.000000000000000000, 2.000000000000000000 ),
 .UNSPECIFIED. ) ;
#11462=CARTESIAN_POINT ( 'NONE',  ( -9.878263419269998735, 1481.129257303990016, 205.3617022385789994 ) ) ;
#11469=VERTEX_POINT ( 'NONE', #109644 ) ;
#11470=CARTESIAN_POINT ( 'NONE',  ( -4.364633595095840590, 1436.783259246580201, 227.1130992530970047 ) ) ;
#11478=CARTESIAN_POINT ( 'NONE',  ( 7.438538526529999473, 1425.192287214430053, 212.3736570440989908 ) ) ;
#11479=CARTESIAN_POINT ( 'NONE',  ( -18.92738905869999755, 1503.346139545890082, 222.1981867166989844 ) ) ;
#11486=EDGE_LOOP ( 'NONE', ( #66428, #28430, #29144, #64257, #109709, #71857, #74015, #1744 ) ) ;
#11492=CARTESIAN_POINT ( 'NONE',  ( -3.551846384670535262, 1441.533148028869391, 200.9985935998525974 ) ) ;
#11496=LINE ( 'NONE', #96602, #101489 ) ;
#11509=CARTESIAN_POINT ( 'NONE',  ( -3.271537977250000395, 1454.292002038190049, 199.1638778798389922 ) ) ;
#11514=CARTESIAN_POINT ( 'NONE',  ( 7.957350483939999108, 1425.611849966230011, 211.5358269577189958 ) ) ;
#11516=EDGE_CURVE ( 'NONE', #49433, #63638, #8311, .T. ) ;
#11519=CARTESIAN_POINT ( 'NONE',  ( -12.15405767247520075, 1489.994125339409948, 210.5239156192949963 ) ) ;
#11544=CARTESIAN_POINT ( 'NONE',  ( -3.119872722899999840, 1429.296741504189868, 201.0353256376990316 ) ) ;
#11548=CARTESIAN_POINT ( 'NONE',  ( -9.519812938348620079, 1460.017558366200092, 210.6311618255110147 ) ) ;
#11554=ORIENTED_EDGE ( 'NONE', *, *, #99292, .T. ) ;
#11557=ORIENTED_EDGE ( 'NONE', *, *, #37123, .F. ) ;
#11562=CARTESIAN_POINT ( 'NONE',  ( 2.911424594440000124, 1441.585781036189928, 218.2054819051689947 ) ) ;
#11565=CARTESIAN_POINT ( 'NONE',  ( 2.326513307799999986, 1476.258183369789776, 197.8633931413990013 ) ) ;
#11571=CARTESIAN_POINT ( 'NONE',  ( 4.329358020582290578, 1515.068258693859889, 207.4791162324520144 ) ) ;
#11572=CARTESIAN_POINT ( 'NONE',  ( -9.756549938588090498, 1472.065839394849945, 211.9795509805560130 ) ) ;
#11577=CARTESIAN_POINT ( 'NONE',  ( -3.817423482790000211, 1484.725631220790092, 198.6719352447990161 ) ) ;
#11582=DIRECTION ( 'NONE',  ( -1.224646799147350002E-16, 1.836970198721029688E-16, 1.000000000000000000 ) ) ;
#11584=CARTESIAN_POINT ( 'NONE',  ( -10.44425495210050059, 1490.271910750019970, 212.9366649069719983 ) ) ;
#11585=CARTESIAN_POINT ( 'NONE',  ( -18.65941870309999828, 1468.219763198689861, 201.0822021908089994 ) ) ;
#11588=CARTESIAN_POINT ( 'NONE',  ( -5.124785876484846625, 1391.876141467484103, 214.5965346519774926 ) ) ;
#11601=CIRCLE ( 'NONE', #54557, 10.71315034250000053 ) ;
#11602=CARTESIAN_POINT ( 'NONE',  ( 9.396366832618360476, 1435.725902782769936, 209.1467788222589945 ) ) ;
#11608=VECTOR ( 'NONE', #106016, 1000.000000000000000 ) ;
#11611=CARTESIAN_POINT ( 'NONE',  ( -9.656448545818989260, 1479.372503699150002, 215.7269582878559788 ) ) ;
#11614=DIRECTION ( 'NONE',  ( 0.1867471702549220458, -2.391457216852619248E-16, -0.9824080081115885710 ) ) ;
#11615=EDGE_LOOP ( 'NONE', ( #99012, #47048, #100284, #53687 ) ) ;
#11618=CARTESIAN_POINT ( 'NONE',  ( 9.662212368149999620, 1493.993336057090119, 188.1975001349989896 ) ) ;
#11625=CARTESIAN_POINT ( 'NONE',  ( -8.539526853489999070, 1458.917133117889762, 213.6780174602090199 ) ) ;
#11629=CARTESIAN_POINT ( 'NONE',  ( -7.982037141949999359, 1424.874072662569915, 210.5243721551090061 ) ) ;
#11641=CARTESIAN_POINT ( 'NONE',  ( -9.293376658228730491, 1440.013600069829863, 206.7969830623249834 ) ) ;
#11653=CARTESIAN_POINT ( 'NONE',  ( 0.9773820611809029835, 1467.205418092640002, 220.1532616540179959 ) ) ;
#11656=B_SPLINE_SURFACE_WITH_KNOTS ( 'NONE', 5, 1, ( 
 ( #28199, #62386 ),
 ( #105466, #88126 ),
 ( #11415, #3032 ),
 ( #54540, #106023 ),
 ( #19217, #37158 ),
 ( #53419, #28755 ) ),
 .UNSPECIFIED., .F., .F., .F.,
 ( 6, 6 ),
 ( 2, 2 ),
 ( 0.000000000000000000, 3.472809815250000209 ),
 ( 0.000000000000000000, 14.00000000000000000 ),
 .UNSPECIFIED. ) ;
#11664=CARTESIAN_POINT ( 'NONE',  ( 3.357570129570000450, 1437.173063345790069, 227.3648210081989873 ) ) ;
#11675=CARTESIAN_POINT ( 'NONE',  ( 11.30915027500000036, 1490.769366722990071, 205.5036971762389726 ) ) ;
#11680=ORIENTED_EDGE ( 'NONE', *, *, #13962, .T. ) ;
#11690=CARTESIAN_POINT ( 'NONE',  ( -4.327853128026350582, 1515.125728221830059, 208.3398689723839823 ) ) ;
#11698=CARTESIAN_POINT ( 'NONE',  ( 2.086548178679999754, 1515.551704408389924, 212.9514660752490158 ) ) ;
#11699=ORIENTED_EDGE ( 'NONE', *, *, #42172, .F. ) ;
#11706=CARTESIAN_POINT ( 'NONE',  ( -16.29090474523583154, 1420.160629993541534, 209.0771752386399953 ) ) ;
#11710=CARTESIAN_POINT ( 'NONE',  ( -3.273040579383169835, 1508.551704408389924, 204.1347629179929868 ) ) ;
#11713=CARTESIAN_POINT ( 'NONE',  ( -14.93718008229999938, 1416.181292664740113, 212.9156384192889959 ) ) ;
#11714=CARTESIAN_POINT ( 'NONE',  ( -2.330134126090000368, 1515.064792882589927, 204.7923971856590128 ) ) ;
#11716=VERTEX_POINT ( 'NONE', #102327 ) ;
#11722=CARTESIAN_POINT ( 'NONE',  ( -6.951511259182890257, 1508.551704405770124, 219.1997712163169751 ) ) ;
#11724=EDGE_CURVE ( 'NONE', #67299, #62781, #37687, .T. ) ;
#11727=CARTESIAN_POINT ( 'NONE',  ( 4.172675962690000517, 1490.591284869190076, 188.6582191385990086 ) ) ;
#11728=CARTESIAN_POINT ( 'NONE',  ( 3.340336038346551906, 1485.759119865504999, 219.3558821538616996 ) ) ;
#11730=DIRECTION ( 'NONE',  ( -0.3026086614614409420, 0.3677779883867259847, -0.8792993513398769112 ) ) ;
#11731=CARTESIAN_POINT ( 'NONE',  ( -1.602167524609999782, 1430.706703968889997, 217.3531761583190018 ) ) ;
#11732=CARTESIAN_POINT ( 'NONE',  ( -10.07154918488590134, 1473.228065907060000, 207.4129428866500007 ) ) ;
#11737=CARTESIAN_POINT ( 'NONE',  ( 9.912698782267559849, 1426.220931725540140, 209.0671000446980088 ) ) ;
#11738=CARTESIAN_POINT ( 'NONE',  ( 11.21226529693919893, 1490.925921770189916, 206.9374627972229916 ) ) ;
#11742=CARTESIAN_POINT ( 'NONE',  ( -2.750440272224420113, 1495.796400148049997, 197.0976659292670092 ) ) ;
#11749=CARTESIAN_POINT ( 'NONE',  ( -6.025152189795589308, 1484.743689720570046, 198.8560543189699956 ) ) ;
#11755=CARTESIAN_POINT ( 'NONE',  ( -7.071828507238460126, 1490.865216771150017, 189.3536562381210047 ) ) ;
#11762=AXIS2_PLACEMENT_3D ( 'NONE', #58510, #24327, #15914 ) ;
#11769=EDGE_LOOP ( 'NONE', ( #74157, #48865, #37120, #29459 ) ) ;
#11772=CARTESIAN_POINT ( 'NONE',  ( -4.270716320095258922, 1515.320037165259464, 206.7917118365956242 ) ) ;
#11776=CARTESIAN_POINT ( 'NONE',  ( 5.982479193689999697, 1424.279491935699980, 194.0293373055990003 ) ) ;
#11777=EDGE_CURVE ( 'NONE', #92278, #108598, #77743, .T. ) ;
#11784=CARTESIAN_POINT ( 'NONE',  ( 1.668736474052739949, 1443.775022403490084, 200.3211312882999948 ) ) ;
#11797=ORIENTED_EDGE ( 'NONE', *, *, #95331, .F. ) ;
#11800=CARTESIAN_POINT ( 'NONE',  ( -4.802733161482000135, 1508.515565345379855, 220.0795834517809908 ) ) ;
#11801=CARTESIAN_POINT ( 'NONE',  ( 6.266043415252799953, 1498.127554395540074, 198.6678067497960001 ) ) ;
#11803=CARTESIAN_POINT ( 'NONE',  ( -2.651145353956480211, 1469.068394821650145, 218.9699912446779990 ) ) ;
#11806=CARTESIAN_POINT ( 'NONE',  ( 9.203495734806530493, 1450.275870452079971, 208.6687953531569804 ) ) ;
#11807=CARTESIAN_POINT ( 'NONE',  ( -5.584029160970000127, 1475.430779401290010, 200.4113593926190049 ) ) ;
#11808=CARTESIAN_POINT ( 'NONE',  ( -2.418619436219159979, 1422.249129387939774, 192.8987411397049812 ) ) ;
#11811=CARTESIAN_POINT ( 'NONE',  ( -13.54316952090000115, 1502.948981525290037, 209.0729592470459863 ) ) ;
#11820=CARTESIAN_POINT ( 'NONE',  ( 18.29188182340000068, 1431.768652859389704, 209.1218459616989946 ) ) ;
#11821=EDGE_CURVE ( 'NONE', #51048, #10343, #96385, .T. ) ;
#11822=CARTESIAN_POINT ( 'NONE',  ( 4.664268937930000192, 1505.247554523090002, 221.0077437511990013 ) ) ;
#11823=CARTESIAN_POINT ( 'NONE',  ( -14.75858103010000022, 1415.739699867389845, 212.8702772392690292 ) ) ;
#11824=CARTESIAN_POINT ( 'NONE',  ( -16.66302441916570132, 1420.069697476050123, 208.3115331456619970 ) ) ;
#11827=CARTESIAN_POINT ( 'NONE',  ( -15.75920964212049569, 1415.789874363079662, 209.6894149795170961 ) ) ;
#11834=CARTESIAN_POINT ( 'NONE',  ( 2.672403418599419656, 1457.264926085269963, 199.5268423672170286 ) ) ;
#11838=CARTESIAN_POINT ( 'NONE',  ( -7.982037141949999359, 1424.874072662569915, 210.5243721551090061 ) ) ;
#11847=CARTESIAN_POINT ( 'NONE',  ( 4.687651746879999415, 1478.378160227390254, 228.9010599218989910 ) ) ;
#11849=CARTESIAN_POINT ( 'NONE',  ( 12.59194315185039947, 1426.976044800900127, 205.9677913843619876 ) ) ;
#11852=CARTESIAN_POINT ( 'NONE',  ( -16.28543887299999682, 1416.852015342750065, 207.9358373243390190 ) ) ;
#11862=EDGE_CURVE ( 'NONE', #27986, #92844, #105715, .T. ) ;
#11868=EDGE_CURVE ( 'NONE', #27986, #58087, #58434, .T. ) ;
#11878=CARTESIAN_POINT ( 'NONE',  ( 6.610761729033765022, 1420.121162737279974, 222.4765268707103303 ) ) ;
#11884=CARTESIAN_POINT ( 'NONE',  ( 0.3865936853360019687, 1422.115159822240230, 193.5453889049990153 ) ) ;
#11887=CARTESIAN_POINT ( 'NONE',  ( 19.00237509055349960, 1454.586986596490078, 200.6139983104000066 ) ) ;
#11891=CARTESIAN_POINT ( 'NONE',  ( -5.030623454749999723, 1391.799616574489846, 203.7592715847190163 ) ) ;
#11893=CARTESIAN_POINT ( 'NONE',  ( 203.9558787908000284, -8382.262153571269664, -1760.903728536709878 ) ) ;
#11894=LINE ( 'NONE', #97010, #58684 ) ;
#11899=CARTESIAN_POINT ( 'NONE',  ( -10.94209231895430179, 1492.979988125699947, 207.3926202358989883 ) ) ;
#11900=CARTESIAN_POINT ( 'NONE',  ( -11.30108578371440586, 1422.091378380982405, 210.6376354647668734 ) ) ;
#11912=CARTESIAN_POINT ( 'NONE',  ( -0.2597432229320009722, 1467.543909054789992, 220.2373604048989932 ) ) ;
#11914=CARTESIAN_POINT ( 'NONE',  ( 10.99603037215820045, 1480.661475631009807, 212.0619901542429773 ) ) ;
#11918=CARTESIAN_POINT ( 'NONE',  ( 20.75865325819999896, 1455.056399776190119, 207.3304373729289978 ) ) ;
#11919=CARTESIAN_POINT ( 'NONE',  ( -2.187180277853430166, 1431.234802153099963, 201.0301937506220042 ) ) ;
#11924=CARTESIAN_POINT ( 'NONE',  ( 4.671899514437313883, 1454.661148777524886, 217.2862335604198165 ) ) ;
#11926=CARTESIAN_POINT ( 'NONE',  ( 20.78751799560000180, 1497.558923099089952, 213.2307807641690260 ) ) ;
#11928=CARTESIAN_POINT ( 'NONE',  ( 3.281831459213320201, 1466.303209658950209, 198.5678429405679992 ) ) ;
#11930=CARTESIAN_POINT ( 'NONE',  ( -18.39846574424100112, 1508.551704408389924, 210.4158962701780240 ) ) ;
#11932=CARTESIAN_POINT ( 'NONE',  ( 3.281831498710000350, 1466.303209520490100, 198.5678428718989892 ) ) ;
#11939=CARTESIAN_POINT ( 'NONE',  ( 11.71326577039419981, 1479.172152660740039, 208.0100838261020044 ) ) ;
#11943=CARTESIAN_POINT ( 'NONE',  ( -18.46075352249601664, 1508.457339376852588, 211.1564294638567958 ) ) ;
#11948=DIRECTION ( 'NONE',  ( -3.909897602534546929E-05, -1.707468113285530796E-06, 0.9999999992341774835 ) ) ;
#11950=CARTESIAN_POINT ( 'NONE',  ( -7.138635338890000348, 1509.224971056590221, 218.8819033035289863 ) ) ;
#11959=CARTESIAN_POINT ( 'NONE',  ( -3.143710964241499983, 1483.525783009509951, 198.9295231152539998 ) ) ;
#11963=B_SPLINE_CURVE_WITH_KNOTS ( 'NONE', 3,
 ( #35105, #61999, #2642, #69847, #435, #26135, #78212, #27819, #95569, #96118, #34554, #28366, #77668, #68737 ),
 .UNSPECIFIED., .F., .F.,
 ( 4, 2, 2, 1, 1, 2, 2, 4 ),
 ( 0.000000000000000000, 0.1250000000000179579, 0.2500000000000359157, 0.3750000000000538458, 0.4374999999996236344, 0.4687499999994085287, 0.4999999999991934230, 1.000000000000000000 ),
 .UNSPECIFIED. ) ;
#11966=CARTESIAN_POINT ( 'NONE',  ( 10.37397012400595919, 1482.317496542443223, 211.4772094469874162 ) ) ;
#11971=B_SPLINE_CURVE_WITH_KNOTS ( 'NONE', 3,
 ( #106863, #100129, #91176, #22844, #56486, #30154, #48084, #40222, #38025, #39104, #108530, #82219, #90617, #39677, #81654, #73844, #64346, #4960, #107971, #63795, #21737, #3896, #14456, #55939, #90060, #29610, #48649, #13341, #47533, #30715, #31268, #99008, #82776, #6069, #74403, #31820, #57607, #80580, #50834, #66562, #83874, #41877, #110181, #16638, #51380, #32380, #59254, #85513, #32912 ),
 .UNSPECIFIED., .F., .F.,
 ( 4, 3, 3, 3, 3, 3, 3, 3, 3, 3, 3, 3, 3, 3, 3, 3, 4 ),
 ( -12.57638456940000005, -12.28317881097320097, -11.95680856205710008, -11.62570944449999999, -11.51472436910320063, -11.17721019326580034, -10.83638269494210071, -10.49376598036129948, -10.14927727058690010, -9.804494080889758933, -9.458815399600899454, -9.117616601269459053, -8.780289088706128453, -8.445887015288109367, -8.114782774046028990, -7.787209585599999428, -7.548674336869999557 ),
 .UNSPECIFIED. ) ;
#11980=CARTESIAN_POINT ( 'NONE',  ( 1.485593186740000071, 1515.527915486090023, 213.1675302385690145 ) ) ;
#11989=B_SPLINE_CURVE_WITH_KNOTS ( 'NONE', 5,
 ( #54804, #27935, #61014, #79449, #2761, #20074, #88935, #88394, #3312 ),
 .UNSPECIFIED., .F., .F.,
 ( 6, 3, 6 ),
 ( -26.06148575846079751, -22.14719212230000167, -12.02292824550000105 ),
 .UNSPECIFIED. ) ;
#11990=CARTESIAN_POINT ( 'NONE',  ( -1.653204953259999943, 1507.621692541890070, 221.1218351714989865 ) ) ;
#11994=CARTESIAN_POINT ( 'NONE',  ( 9.104904664964859506, 1467.958063039340004, 204.8661130570050091 ) ) ;
#12011=CARTESIAN_POINT ( 'NONE',  ( -11.33033813286753677, 1502.925034412118521, 207.0842279942457083 ) ) ;
#12013=CARTESIAN_POINT ( 'NONE',  ( -20.87069991009999725, 1506.658021081189872, 214.5368842940590071 ) ) ;
#12016=CARTESIAN_POINT ( 'NONE',  ( -3.558358604862239982, 1455.955982659530036, 200.3550966546550001 ) ) ;
#12019=CARTESIAN_POINT ( 'NONE',  ( 7.783524595000000268, 1424.818165691749982, 211.8233307128890033 ) ) ;
#12020=AXIS2_PLACEMENT_3D ( 'NONE', #47074, #3429, #81198 ) ;
#12023=CARTESIAN_POINT ( 'NONE',  ( -11.16717556649999921, 1414.661898229710005, 212.7267128011690147 ) ) ;
#12026=DIRECTION ( 'NONE',  ( 0.02091224828123190022, 0.9990482215818557998, 0.03827961371219716635 ) ) ;
#12027=ORIENTED_EDGE ( 'NONE', *, *, #88452, .F. ) ;
#12049=CARTESIAN_POINT ( 'NONE',  ( -15.62861149524349891, 1418.244676918490086, 203.0179538217920197 ) ) ;
#12050=CARTESIAN_POINT ( 'NONE',  ( 20.87949000879999772, 1495.383548355589937, 212.2163053943189936 ) ) ;
#12065=VECTOR ( 'NONE', #91135, 1000.000000000000114 ) ;
#12074=CARTESIAN_POINT ( 'NONE',  ( 9.992021184015209556, 1491.422374287340062, 188.4943422680200058 ) ) ;
#12082=CARTESIAN_POINT ( 'NONE',  ( -2.532956463620000154, 1430.062184787290107, 201.0558268371090094 ) ) ;
#12090=CARTESIAN_POINT ( 'NONE',  ( -3.467940602053699806, 1495.562067921990092, 197.2905559617530002 ) ) ;
#12091=CARTESIAN_POINT ( 'NONE',  ( 10.75551144678770044, 1470.210679328900142, 207.2751881891400103 ) ) ;
#12097=CARTESIAN_POINT ( 'NONE',  ( 7.499999999999999112, 1392.213060387289943, 209.1218459616989946 ) ) ;
#12100=CARTESIAN_POINT ( 'NONE',  ( 3.750000000000000000, 1516.051704408390151, 209.1218459616989946 ) ) ;
#12103=CARTESIAN_POINT ( 'NONE',  ( 1.542378980109999853, 1442.042834985789796, 218.9497927206290058 ) ) ;
#12109=DIRECTION ( 'NONE',  ( -9.341989762165448955E-47, 1.000000000000000000, -1.836970198721029688E-16 ) ) ;
#12112=CARTESIAN_POINT ( 'NONE',  ( -1.748905610829809998, 1488.269106374019884, 219.8524659745219765 ) ) ;
#12115=CARTESIAN_POINT ( 'NONE',  ( -15.40297484210000079, 1508.551704408389924, 214.7119267552490101 ) ) ;
#12120=CARTESIAN_POINT ( 'NONE',  ( -16.24600786016249643, 1417.782917922866091, 204.8292002259562707 ) ) ;
#12125=CARTESIAN_POINT ( 'NONE',  ( -6.435172845517500129, 1488.130694331340237, 218.4885078549579873 ) ) ;
#12126=CARTESIAN_POINT ( 'NONE',  ( -4.354856984870000502, 1481.954696296189923, 231.1149923864989830 ) ) ;
#12135=VERTEX_POINT ( 'NONE', #26185 ) ;
#12137=CARTESIAN_POINT ( 'NONE',  ( -7.762930123710000352, 1492.073939571090023, 209.9113589376980258 ) ) ;
#12159=CARTESIAN_POINT ( 'NONE',  ( -11.67226624329999929, 1483.956261651290106, 228.3627183349989878 ) ) ;
#12166=CARTESIAN_POINT ( 'NONE',  ( -8.776085081250000641, 1460.194150302089838, 214.2375442011990003 ) ) ;
#12174=CARTESIAN_POINT ( 'NONE',  ( -5.062212390315069754, 1474.342205398819942, 198.8731691453010058 ) ) ;
#12176=DIRECTION ( 'NONE',  ( 0.02091224828123159837, -0.9990482215818557998, 0.03827961371219689574 ) ) ;
#12179=ORIENTED_EDGE ( 'NONE', *, *, #1011, .F. ) ;
#12180=CARTESIAN_POINT ( 'NONE',  ( 3.838475640130000421, 1505.530984303090008, 221.3004008607989874 ) ) ;
#12182=CARTESIAN_POINT ( 'NONE',  ( 7.567873768730000172, 1473.049319849490075, 217.1534710516689870 ) ) ;
#12183=B_SPLINE_CURVE_WITH_KNOTS ( 'NONE', 5,
 ( #58373, #15234, #108207, #30397, #65126, #64588, #98707, #31495, #39909 ),
 .UNSPECIFIED., .F., .F.,
 ( 6, 3, 6 ),
 ( 0.000000000000000000, 0.2682459062916608961, 1.000000000000000000 ),
 .UNSPECIFIED. ) ;
#12184=CARTESIAN_POINT ( 'NONE',  ( -8.106549357737529604, 1438.741334074130009, 205.9368686404189930 ) ) ;
#12185=ORIENTED_EDGE ( 'NONE', *, *, #43802, .T. ) ;
#12191=ORIENTED_EDGE ( 'NONE', *, *, #43900, .F. ) ;
#12193=CARTESIAN_POINT ( 'NONE',  ( -2.029307951927409981, 1467.934477929960167, 220.0622926176330054 ) ) ;
#12197=DIRECTION ( 'NONE',  ( 7.303600220002790452E-17, 1.000000000000000000, -3.615388577796539518E-17 ) ) ;
#12210=FACE_OUTER_BOUND ( 'NONE', #93558, .T. ) ;
#12239=CARTESIAN_POINT ( 'NONE',  ( 11.78397860869369929, 1499.475900767659823, 204.3830586676889993 ) ) ;
#12255=EDGE_LOOP ( 'NONE', ( #5840, #72953, #99202, #55030 ) ) ;
#12258=CARTESIAN_POINT ( 'NONE',  ( -3.444563290230000074, 1476.680507959189981, 199.3428731527990010 ) ) ;
#12259=DIRECTION ( 'NONE',  ( -0.8742006210163753011, -0.3833097456314917273, -0.2980719931803466616 ) ) ;
#12261=CARTESIAN_POINT ( 'NONE',  ( 10.59810956035219753, 1477.523927547069889, 229.9254287524879885 ) ) ;
#12262=VERTEX_POINT ( 'NONE', #93397 ) ;
#12266=CARTESIAN_POINT ( 'NONE',  ( -1.189318188510000152, 1432.130355740389859, 218.1858096881190079 ) ) ;
#12267=CARTESIAN_POINT ( 'NONE',  ( 20.65879167559999985, 1494.308160183190012, 205.1000562319489973 ) ) ;
#12269=CARTESIAN_POINT ( 'NONE',  ( 12.55979069370000012, 1458.679714032590027, 224.9161459441990019 ) ) ;
#12278=CARTESIAN_POINT ( 'NONE',  ( 1.049829441584229750, 1496.809906337439998, 196.7866365865189948 ) ) ;
#12286=DIRECTION ( 'NONE',  ( 8.727810504445229884E-47, -1.000000000000000000, 1.836970198721029688E-16 ) ) ;
#12288=AXIS2_PLACEMENT_3D ( 'NONE', #43017, #59278, #76060 ) ;
#12303=DIRECTION ( 'NONE',  ( -1.000000000000000000, -2.657783323254384930E-32, -1.224646799147351975E-16 ) ) ;
#12305=CARTESIAN_POINT ( 'NONE',  ( 3.305605061710000125, 1485.263013822589983, 219.7395602488990107 ) ) ;
#12318=ORIENTED_EDGE ( 'NONE', *, *, #7705, .F. ) ;
#12329=ORIENTED_EDGE ( 'NONE', *, *, #103785, .F. ) ;
#12332=ORIENTED_EDGE ( 'NONE', *, *, #81136, .F. ) ;
#12334=CARTESIAN_POINT ( 'NONE',  ( -10.51558556386050114, 1480.736735032730166, 208.3484430820659838 ) ) ;
#12336=CARTESIAN_POINT ( 'NONE',  ( 5.024924619706210294, 1497.858354990089992, 198.0416419176340241 ) ) ;
#12338=CARTESIAN_POINT ( 'NONE',  ( -2.779626312165170088, 1468.659898279970093, 219.1847641695690072 ) ) ;
#12340=CARTESIAN_POINT ( 'NONE',  ( 9.213396914969999685, 1420.767274165939853, 196.7655569023989983 ) ) ;
#12342=CARTESIAN_POINT ( 'NONE',  ( -5.693783788968350912, 1494.776061667409977, 198.1946402388329886 ) ) ;
#12345=CARTESIAN_POINT ( 'NONE',  ( -19.19558940460000329, 1505.173093966990109, 209.0368464700519837 ) ) ;
#12348=B_SPLINE_CURVE_WITH_KNOTS ( 'NONE', 3,
 ( #110559, #58516, #101036, #41701, #56861, #84250, #41150, #66382, #76404, #100501, #8089, #24336, #49569, #40045, #74227, #83697, #6993, #92646, #15920, #50122, #24870, #82609 ),
 .UNSPECIFIED., .F., .F.,
 ( 4, 2, 1, 1, 2, 2, 2, 2, 1, 1, 2, 2, 4 ),
 ( 0.000000000000000000, 0.1250000000000019151, 0.1874999999999887867, 0.2187499999999827360, 0.2343749999999658884, 0.2499999999999490685, 0.4999999999998919198, 0.6249999999998638867, 0.6874999999998662181, 0.7187499999998674394, 0.7343749999998693268, 0.7499999999998712141, 1.000000000000000000 ),
 .UNSPECIFIED. ) ;
#12356=B_SPLINE_SURFACE_WITH_KNOTS ( 'NONE', 5, 1, ( 
 ( #68568, #59059 ),
 ( #76392, #102130 ),
 ( #51761, #103226 ),
 ( #19220, #20338 ),
 ( #96514, #36603 ),
 ( #63498, #105470 ),
 ( #38247, #70249 ),
 ( #62390, #46684 ),
 ( #89757, #19793 ) ),
 .UNSPECIFIED., .F., .F., .F.,
 ( 6, 3, 6 ),
 ( 2, 2 ),
 ( 0.000000000000000000, 3.688278477100000341, 7.358176137350000090 ),
 ( 0.000000000000000000, 14.00000000000000000 ),
 .UNSPECIFIED. ) ;
#12358=CARTESIAN_POINT ( 'NONE',  ( 4.507890822339999382, 1506.158184558590165, 220.0129750286989747 ) ) ;
#12360=CARTESIAN_POINT ( 'NONE',  ( -17.78871670860239718, 1419.650462417609788, 206.8064655431160190 ) ) ;
#12366=CARTESIAN_POINT ( 'NONE',  ( 0.1351882977586719992, 1430.428589182629821, 199.6983684263929888 ) ) ;
#12371=CARTESIAN_POINT ( 'NONE',  ( 8.340772919400350816, 1460.715584676179787, 204.0670572953980013 ) ) ;
#12375=CARTESIAN_POINT ( 'NONE',  ( 10.00676819928309946, 1469.384229055800233, 210.0288051735269903 ) ) ;
#12381=AXIS2_PLACEMENT_3D ( 'NONE', #108747, #32039, #7388 ) ;
#12386=CARTESIAN_POINT ( 'NONE',  ( -14.22077585328280058, 1416.525864124620057, 203.1782020047139952 ) ) ;
#12390=CARTESIAN_POINT ( 'NONE',  ( 9.402787699681429245, 1428.181318586850011, 212.5511139594050007 ) ) ;
#12401=CARTESIAN_POINT ( 'NONE',  ( -13.58042247833220095, 1508.551704408300111, 210.3416305655150040 ) ) ;
#12410=CARTESIAN_POINT ( 'NONE',  ( -12.20257788280040145, 1490.746699033079949, 207.9129267422960083 ) ) ;
#12411=CARTESIAN_POINT ( 'NONE',  ( -3.490046645198510156, 1508.551704408389924, 204.3447946308859855 ) ) ;
#12417=CARTESIAN_POINT ( 'NONE',  ( 0.000000000000000000, 1412.913060387329779, 209.1218459616989946 ) ) ;
#12420=CARTESIAN_POINT ( 'NONE',  ( -17.54273015099310129, 1417.931783278020021, 206.8684746656099946 ) ) ;
#12424=CARTESIAN_POINT ( 'NONE',  ( -18.64099322077279908, 1468.021338938559893, 201.0622087414649855 ) ) ;
#12440=CARTESIAN_POINT ( 'NONE',  ( -10.67342804297004655, 1422.346099354243051, 210.6393889615464730 ) ) ;
#12451=CARTESIAN_POINT ( 'NONE',  ( 10.92766316885620093, 1501.618323021010156, 205.6861136770480130 ) ) ;
#12452=( BOUNDED_CURVE ( )  B_SPLINE_CURVE ( 3, ( #97901, #55380, #62712, #3886 ),
 .UNSPECIFIED., .F., .T. ) 
 B_SPLINE_CURVE_WITH_KNOTS ( ( 4, 4 ),
 ( 4.173463862610059749, 5.251314181851939544 ),
 .UNSPECIFIED. ) 
 CURVE ( )  GEOMETRIC_REPRESENTATION_ITEM ( )  RATIONAL_B_SPLINE_CURVE ( ( 1.000000000000000000, 0.9055071999559949347, 0.9055071999559949347, 1.000000000000000000 ) ) 
 REPRESENTATION_ITEM ( '' )  );
#12456=CARTESIAN_POINT ( 'NONE',  ( -1.335546054589999976, 1468.359610537590015, 219.4358368445990095 ) ) ;
#12458=CARTESIAN_POINT ( 'NONE',  ( 7.311558199926071033, 1484.801511308949785, 217.1227323129160141 ) ) ;
#12462=VERTEX_POINT ( 'NONE', #36687 ) ;
#12463=CARTESIAN_POINT ( 'NONE',  ( 0.9103496401472069843, 1462.760058940530143, 230.5111392918950060 ) ) ;
#12494=CARTESIAN_POINT ( 'NONE',  ( -6.625178543776530482, 1435.234561983659887, 216.2082763422070286 ) ) ;
#12503=B_SPLINE_SURFACE_WITH_KNOTS ( 'NONE', 5, 5, ( 
 ( #63286, #3922, #70581, #55964, #15024, #99586 ),
 ( #73310, #22313, #39702, #38586, #73868, #109127 ),
 ( #21763, #90087, #74430, #107446, #66032, #47559 ),
 ( #32408, #81681, #14483, #31293, #4987, #57078 ),
 ( #30180, #56516, #90643, #22869, #48676, #72765 ),
 ( #49222, #100155, #4458, #64372, #39131, #12838 ) ),
 .UNSPECIFIED., .F., .F., .F.,
 ( 6, 6 ),
 ( 6, 6 ),
 ( 4.019724148039999889, 13.77031185580000106 ),
 ( 0.000000000000000000, 0.5000000000000000000 ),
 .UNSPECIFIED. ) ;
#12506=CARTESIAN_POINT ( 'NONE',  ( 4.329448781177520189, 1515.064792686469900, 207.2788827064790098 ) ) ;
#12518=CARTESIAN_POINT ( 'NONE',  ( -14.48634919999999937, 1416.023439645540066, 203.8591738074189834 ) ) ;
#12526=EDGE_LOOP ( 'NONE', ( #41663, #19881, #26058, #74795 ) ) ;
#12529=CARTESIAN_POINT ( 'NONE',  ( -1.842962231260000028, 1515.372048949689997, 213.3835825136090136 ) ) ;
#12532=EDGE_CURVE ( 'NONE', #27116, #21797, #30929, .T. ) ;
#12533=CARTESIAN_POINT ( 'NONE',  ( 2.064218541529331929, 1464.188986783531618, 199.5203533287811126 ) ) ;
#12535=CARTESIAN_POINT ( 'NONE',  ( -6.347844883064759358, 1440.117647072198906, 203.0612122617101818 ) ) ;
#12536=AXIS2_PLACEMENT_3D ( 'NONE', #57396, #109980, #14802 ) ;
#12537=CARTESIAN_POINT ( 'NONE',  ( -3.957900269260000048, 1458.284989000489986, 219.0746905126889885 ) ) ;
#12538=CARTESIAN_POINT ( 'NONE',  ( -4.989533930479999491, 1429.437332217889889, 202.3857892670889953 ) ) ;
#12542=ORIENTED_EDGE ( 'NONE', *, *, #1619, .T. ) ;
#12545=CARTESIAN_POINT ( 'NONE',  ( 7.001391005937890100, 1467.620735506979827, 200.2764061176360144 ) ) ;
#12547=CARTESIAN_POINT ( 'NONE',  ( 17.07372443010000040, 1494.814959774189902, 195.5520917663990019 ) ) ;
#12553=CARTESIAN_POINT ( 'NONE',  ( -9.542479485949998619, 1481.357605531989975, 204.5426345580789871 ) ) ;
#12560=EDGE_LOOP ( 'NONE', ( #98522, #37950, #13338, #27893 ) ) ;
#12561=CARTESIAN_POINT ( 'NONE',  ( -11.32803462625343194, 1502.699820297845008, 207.1273456882843789 ) ) ;
#12571=CARTESIAN_POINT ( 'NONE',  ( 8.075468704329999525, 1426.465554857850066, 211.6438910379590084 ) ) ;
#12577=CARTESIAN_POINT ( 'NONE',  ( 8.978224261840001219, 1452.688325861789963, 212.1105519951989891 ) ) ;
#12578=EDGE_LOOP ( 'NONE', ( #1097, #84747, #108743, #71678 ) ) ;
#12579=ORIENTED_EDGE ( 'NONE', *, *, #76649, .T. ) ;
#12590=CARTESIAN_POINT ( 'NONE',  ( -2.031867801918239902, 1464.998398352370032, 198.3053289726209982 ) ) ;
#12610=CARTESIAN_POINT ( 'NONE',  ( -12.51045652733512625, 1415.677402202029953, 206.7437175916260230 ) ) ;
#12614=VECTOR ( 'NONE', #81199, 1000.000000000000114 ) ;
#12615=CARTESIAN_POINT ( 'NONE',  ( -11.88881437795680007, 1489.631889030339835, 211.9231216160999907 ) ) ;
#12622=CYLINDRICAL_SURFACE ( 'NONE', #81519, 3.750000000000000000 ) ;
#12633=CARTESIAN_POINT ( 'NONE',  ( 7.253078750751489778, 1425.167378741770108, 192.6391490917010287 ) ) ;
#12639=VERTEX_POINT ( 'NONE', #78006 ) ;
#12642=TOROIDAL_SURFACE ( 'NONE', #84164, 7.500000000000000000, 0.2999999999999999889 ) ;
#12645=CARTESIAN_POINT ( 'NONE',  ( 11.66936717579999971, 1421.865521096479824, 204.5896370874590104 ) ) ;
#12646=CARTESIAN_POINT ( 'NONE',  ( 0.6489903397072023239, 1498.624614946328165, 197.8160440545376275 ) ) ;
#12654=CARTESIAN_POINT ( 'NONE',  ( 10.49535538868399875, 1481.102825724099830, 207.9455356762770180 ) ) ;
#12658=CARTESIAN_POINT ( 'NONE',  ( 8.842581916386802021, 1424.898463456729814, 195.7260410483776809 ) ) ;
#12659=CARTESIAN_POINT ( 'NONE',  ( 2.634457758659999538, 1441.548974666690128, 218.6895019696289921 ) ) ;
#12667=CARTESIAN_POINT ( 'NONE',  ( 5.547280765580000050, 1487.873461314389942, 198.4571336758990014 ) ) ;
#12672=CARTESIAN_POINT ( 'NONE',  ( -13.32757262590000025, 1508.445659285190004, 217.0210970315689849 ) ) ;
#12674=CARTESIAN_POINT ( 'NONE',  ( 11.15470940107600128, 1470.295755632079818, 206.9817199298160233 ) ) ;
#12675=CARTESIAN_POINT ( 'NONE',  ( -2.576618889659999745, 1485.526343952190246, 197.4968898064989844 ) ) ;
#12680=CARTESIAN_POINT ( 'NONE',  ( 3.427496190376880136, 1494.480924628220009, 219.9046048467500043 ) ) ;
#12681=CARTESIAN_POINT ( 'NONE',  ( 0.5708535463504419427, 1460.784162354619866, 230.4191111958880072 ) ) ;
#12691=CARTESIAN_POINT ( 'NONE',  ( -20.11385680769999951, 1487.601373209189887, 204.1067431612489997 ) ) ;
#12700=CARTESIAN_POINT ( 'NONE',  ( 4.994880155184180381, 1467.527977092940091, 217.7500441216180036 ) ) ;
#12702=CARTESIAN_POINT ( 'NONE',  ( -0.01406703361950679965, 1515.158574431529814, 213.4488389814559923 ) ) ;
#12704=CARTESIAN_POINT ( 'NONE',  ( -10.67455619629699903, 1480.094165611569906, 214.0407775190860207 ) ) ;
#12708=CARTESIAN_POINT ( 'NONE',  ( 1.396945595908719806, 1473.097535771269804, 219.2356281669150064 ) ) ;
#12710=ORIENTED_EDGE ( 'NONE', *, *, #76076, .F. ) ;
#12712=CARTESIAN_POINT ( 'NONE',  ( -17.98650874570000013, 1489.991360812790163, 195.2845414362990084 ) ) ;
#12714=CARTESIAN_POINT ( 'NONE',  ( 7.782527000790000038, 1421.790398246840141, 195.8641137985989928 ) ) ;
#12719=CARTESIAN_POINT ( 'NONE',  ( 4.327305182180260168, 1515.146653429429989, 209.5728053323190068 ) ) ;
#12733=CARTESIAN_POINT ( 'NONE',  ( -9.138800708037619458, 1447.299821738310129, 212.1281046494140128 ) ) ;
#12738=EDGE_LOOP ( 'NONE', ( #84591, #90261, #101434, #21258 ) ) ;
#12741=CARTESIAN_POINT ( 'NONE',  ( 9.058637367070000224, 1472.814398557089817, 216.2138489941889929 ) ) ;
#12752=CARTESIAN_POINT ( 'NONE',  ( -0.1650793151492190025, 1467.512301221159987, 220.2121120126230096 ) ) ;
#12774=CARTESIAN_POINT ( 'NONE',  ( -13.96688741319999849, 1417.698261240689817, 203.4998333049589974 ) ) ;
#12779=DIRECTION ( 'NONE',  ( -1.156023075842281927E-31, 1.000000000000000000, -1.698192320643030073E-16 ) ) ;
#12785=CARTESIAN_POINT ( 'NONE',  ( -16.65376764594610037, 1508.454796205149933, 213.7212175226700026 ) ) ;
#12795=CARTESIAN_POINT ( 'NONE',  ( 10.21056514295750084, 1500.159686141239945, 203.5544954536850071 ) ) ;
#12798=CARTESIAN_POINT ( 'NONE',  ( -4.360190560360000411, 1441.644575985890015, 201.4346498888789938 ) ) ;
#12800=CARTESIAN_POINT ( 'NONE',  ( -10.99853003760000014, 1492.080317501190166, 210.0618239403530083 ) ) ;
#12803=CARTESIAN_POINT ( 'NONE',  ( -3.117394057747560066, 1508.880977799760103, 204.6292041399409811 ) ) ;
#12812=CARTESIAN_POINT ( 'NONE',  ( -3.326917603050000061, 1476.247319049890166, 199.3214893299089852 ) ) ;
#12815=CARTESIAN_POINT ( 'NONE',  ( -2.515575408287869852, 1448.349567905599997, 188.5842445502629801 ) ) ;
#12816=ORIENTED_EDGE ( 'NONE', *, *, #85138, .T. ) ;
#12818=CARTESIAN_POINT ( 'NONE',  ( 1.720211288050000009, 1484.988610551289867, 201.3271807748389790 ) ) ;
#12820=CARTESIAN_POINT ( 'NONE',  ( 10.97527900237937715, 1503.727326051738601, 212.8216792447624357 ) ) ;
#12822=CARTESIAN_POINT ( 'NONE',  ( -10.12425452533820014, 1472.594269829849964, 207.2375451810740117 ) ) ;
#12838=CARTESIAN_POINT ( 'NONE',  ( -15.84432986099999852, 1419.853212303100008, 210.7451137706489703 ) ) ;
#12854=CARTESIAN_POINT ( 'NONE',  ( -1.603373619530000127, 1416.384743139180046, 204.3300628165089847 ) ) ;
#12857=LINE ( 'NONE', #3942, #60616 ) ;
#12859=CARTESIAN_POINT ( 'NONE',  ( -0.4963980325270009319, 1487.926393457290033, 219.9945907317990077 ) ) ;
#12870=CARTESIAN_POINT ( 'NONE',  ( 10.56408392316350131, 1452.658046758459932, 209.7429679461859848 ) ) ;
#12872=ORIENTED_EDGE ( 'NONE', *, *, #61336, .T. ) ;
#12874=CARTESIAN_POINT ( 'NONE',  ( -15.17703146246870105, 1445.095302021130010, 196.7536351334289861 ) ) ;
#12881=CARTESIAN_POINT ( 'NONE',  ( 2.330134126767420266, 1515.064792882699976, 204.7923971855439902 ) ) ;
#12884=CARTESIAN_POINT ( 'NONE',  ( 5.697020712293880962, 1483.840076960939996, 219.4998280688900252 ) ) ;
#12890=CARTESIAN_POINT ( 'NONE',  ( -3.672693132570179930, 1508.551704069029938, 220.1143460865109773 ) ) ;
#12893=CARTESIAN_POINT ( 'NONE',  ( -9.531705855666331217, 1470.352007687029982, 213.6243478951139991 ) ) ;
#12895=CARTESIAN_POINT ( 'NONE',  ( 9.558212104659999042, 1420.850661932230196, 197.1275686703990004 ) ) ;
#12896=CARTESIAN_POINT ( 'NONE',  ( -1.509201711952470104, 1475.790545536990066, 220.4654702390089938 ) ) ;
#12897=CARTESIAN_POINT ( 'NONE',  ( -7.344663150544599617, 1494.134771815259910, 199.2391034037320026 ) ) ;
#12905=CARTESIAN_POINT ( 'NONE',  ( 19.55988977460000200, 1474.636381753090063, 214.0184790771390055 ) ) ;
#12909=CARTESIAN_POINT ( 'NONE',  ( -15.22934408750000124, 1415.677402202029953, 210.1988070706289875 ) ) ;
#12911=ORIENTED_EDGE ( 'NONE', *, *, #7650, .F. ) ;
#12913=CARTESIAN_POINT ( 'NONE',  ( -8.092117112805246038, 1477.146199184617444, 215.6332617364606392 ) ) ;
#12914=CARTESIAN_POINT ( 'NONE',  ( 9.377597136699939995, 1436.953564941884679, 212.2519927847499162 ) ) ;
#12929=CARTESIAN_POINT ( 'NONE',  ( 12.50106635730310067, 1427.054470077530141, 206.4470538787940086 ) ) ;
#12934=CARTESIAN_POINT ( 'NONE',  ( -4.201139955930000447, 1515.456931311890003, 208.0107056655590156 ) ) ;
#12939=ORIENTED_EDGE ( 'NONE', *, *, #46392, .T. ) ;
#12942=CARTESIAN_POINT ( 'NONE',  ( -11.79257188989999960, 1490.424927487490095, 209.6468054275469797 ) ) ;
#12943=CARTESIAN_POINT ( 'NONE',  ( -2.705738833059999848, 1468.840749178389842, 189.3603025906990069 ) ) ;
#12944=CARTESIAN_POINT ( 'NONE',  ( 10.02421119480000122, 1480.534221758890226, 205.8829018067289951 ) ) ;
#12952=CARTESIAN_POINT ( 'NONE',  ( -4.821236195118149936, 1508.551704408389924, 205.7350742881380086 ) ) ;
#12955=CARTESIAN_POINT ( 'NONE',  ( -2.098112454099999802, 1502.392812899289993, 230.4314219549989957 ) ) ;
#12957=CARTESIAN_POINT ( 'NONE',  ( -9.592658376373048412, 1460.893772936906089, 207.6096792123005343 ) ) ;
#12959=CARTESIAN_POINT ( 'NONE',  ( -5.079869688909999681, 1496.157899184890084, 219.1414376983989882 ) ) ;
#12964=CARTESIAN_POINT ( 'NONE',  ( -9.701071637315321183, 1463.456538005379798, 228.1046814505860141 ) ) ;
#12976=CARTESIAN_POINT ( 'NONE',  ( 11.85236273005710039, 1501.984533761569764, 213.9659136087529987 ) ) ;
#12983=CARTESIAN_POINT ( 'NONE',  ( 3.128860413254639816, 1484.852474905719873, 220.5520654540769954 ) ) ;
#12984=CARTESIAN_POINT ( 'NONE',  ( 10.93419921699999975, 1501.146262457190005, 205.7756198371390042 ) ) ;
#12991=CARTESIAN_POINT ( 'NONE',  ( 9.239580200065189430, 1483.101234906810078, 214.6484747421150132 ) ) ;
#12995=CARTESIAN_POINT ( 'NONE',  ( -17.65533327544169850, 1419.497269525679940, 207.2321674072659903 ) ) ;
#12998=ORIENTED_EDGE ( 'NONE', *, *, #57592, .T. ) ;
#13006=CARTESIAN_POINT ( 'NONE',  ( -1.935234340010000054, 1464.825742489889763, 198.7112508957989974 ) ) ;
#13012=ORIENTED_EDGE ( 'NONE', *, *, #36587, .F. ) ;
#13017=CARTESIAN_POINT ( 'NONE',  ( -8.588755447433969792, 1437.818850531529961, 207.9413692731380081 ) ) ;
#13018=CARTESIAN_POINT ( 'NONE',  ( -17.52838533095563989, 1508.456237627404562, 212.5777381106094879 ) ) ;
#13020=CARTESIAN_POINT ( 'NONE',  ( -8.546921754562520235, 1436.723958230239987, 213.9303451536549971 ) ) ;
#13029=CARTESIAN_POINT ( 'NONE',  ( -10.46978020201859039, 1480.344165297236941, 208.0133452714284772 ) ) ;
#13030=CARTESIAN_POINT ( 'NONE',  ( 3.235048515759559873, 1466.472015849239824, 219.6884157167970102 ) ) ;
#13034=CARTESIAN_POINT ( 'NONE',  ( -6.785810196629999957, 1424.002256156930116, 192.0785610996990158 ) ) ;
#13039=CARTESIAN_POINT ( 'NONE',  ( -15.22114443889999968, 1415.799205417750045, 206.7037562793690029 ) ) ;
#13041=CARTESIAN_POINT ( 'NONE',  ( 7.398264911990000137, 1422.106259636749883, 195.6015909957990289 ) ) ;
#13042=CARTESIAN_POINT ( 'NONE',  ( -5.080191068885199890, 1480.093223193510084, 228.8813504292600101 ) ) ;
#13054=CARTESIAN_POINT ( 'NONE',  ( -0.4102078045352910429, 1463.514555870267714, 199.3390046908783404 ) ) ;
#13057=CARTESIAN_POINT ( 'NONE',  ( -9.828024340748898524, 1446.801136768030119, 212.2328356403849909 ) ) ;
#13070=CARTESIAN_POINT ( 'NONE',  ( -18.17365796220000007, 1441.208305948289762, 213.5442559039389891 ) ) ;
#13071=CARTESIAN_POINT ( 'NONE',  ( 7.196800634449999734, 1423.618640619720054, 213.1214840613790216 ) ) ;
#13074=B_SPLINE_CURVE_WITH_KNOTS ( 'NONE', 5,
 ( #40500, #99286, #22013, #74678, #22562, #15280 ),
 .UNSPECIFIED., .F., .F.,
 ( 6, 6 ),
 ( 496.9399198659999684, 502.1482307969999965 ),
 .UNSPECIFIED. ) ;
#13075=CARTESIAN_POINT ( 'NONE',  ( 12.17122754174319788, 1491.569219868120172, 207.3549893034999911 ) ) ;
#13087=DIRECTION ( 'NONE',  ( 1.000000000000000000, -3.196303315166338322E-31, 4.657260248767550292E-10 ) ) ;
#13092=CARTESIAN_POINT ( 'NONE',  ( -5.192525392799999473, 1454.457094112089862, 201.2666327733590208 ) ) ;
#13094=CARTESIAN_POINT ( 'NONE',  ( 7.156887453669999566, 1427.109879847909951, 213.1306117699590175 ) ) ;
#13097=CARTESIAN_POINT ( 'NONE',  ( -22.99236997363790280, 1417.360559190849926, 209.8837839782780179 ) ) ;
#13101=CARTESIAN_POINT ( 'NONE',  ( 8.171450972760000653, 1453.343394502490128, 214.0171812195989673 ) ) ;
#13111=CARTESIAN_POINT ( 'NONE',  ( -21.50400446119279962, 1505.467562055609960, 209.6175409707290100 ) ) ;
#13122=ORIENTED_EDGE ( 'NONE', *, *, #90559, .F. ) ;
#13123=ORIENTED_EDGE ( 'NONE', *, *, #42629, .F. ) ;
#13131=CARTESIAN_POINT ( 'NONE',  ( -18.87812302109619722, 1508.542151561040100, 209.8906029150280119 ) ) ;
#13145=CARTESIAN_POINT ( 'NONE',  ( -14.12816946494867132, 1415.677402202033818, 214.2877445135121661 ) ) ;
#13165=CARTESIAN_POINT ( 'NONE',  ( 10.54588268310000032, 1424.218227896809822, 206.2742958475490127 ) ) ;
#13171=CARTESIAN_POINT ( 'NONE',  ( 10.77874527468759958, 1470.254009331350062, 207.3979366881200121 ) ) ;
#13175=ORIENTED_EDGE ( 'NONE', *, *, #261, .T. ) ;
#13176=CARTESIAN_POINT ( 'NONE',  ( 9.538745118365339337, 1491.433376268790198, 189.9872206277390205 ) ) ;
#13180=CARTESIAN_POINT ( 'NONE',  ( 10.95536116137719951, 1461.143322918870126, 209.2158675909050203 ) ) ;
#13181=CARTESIAN_POINT ( 'NONE',  ( 9.302468707345267873, 1425.246985399160394, 195.5946313398209213 ) ) ;
#13182=CARTESIAN_POINT ( 'NONE',  ( 2.545036209910000125, 1441.771739723390056, 218.3207620803289899 ) ) ;
#13194=CONICAL_SURFACE ( 'NONE', #27528, 6.911399307709998219, 0.04363323129990067523 ) ;
#13196=CARTESIAN_POINT ( 'NONE',  ( -8.839654036029999773, 1508.551704422490047, 218.8221981809089982 ) ) ;
#13197=DIRECTION ( 'NONE',  ( -1.000000000000000000, 0.000000000000000000, 0.000000000000000000 ) ) ;
#13199=CARTESIAN_POINT ( 'NONE',  ( 11.36218398372849947, 1470.732519598219824, 208.3241800981469964 ) ) ;
#13208=CARTESIAN_POINT ( 'NONE',  ( 9.992011831555620560, 1491.422447192649770, 188.4943338504039900 ) ) ;
#13209=CARTESIAN_POINT ( 'NONE',  ( -14.65515196210479942, 1415.677402204470127, 206.0377850102939874 ) ) ;
#13210=CARTESIAN_POINT ( 'NONE',  ( -9.652435728993630448, 1460.634894123000095, 208.5891384216040194 ) ) ;
#13211=CARTESIAN_POINT ( 'NONE',  ( 4.760952894889999065, 1429.902475422190037, 216.8416751273590251 ) ) ;
#13212=CARTESIAN_POINT ( 'NONE',  ( 5.909797370239999736, 1492.458403186890109, 214.9549538718289909 ) ) ;
#13233=CARTESIAN_POINT ( 'NONE',  ( -9.486023288045011270, 1479.268917112100098, 215.9504765402980127 ) ) ;
#13238=EDGE_LOOP ( 'NONE', ( #70890, #32784, #29631, #97582 ) ) ;
#13240=CARTESIAN_POINT ( 'NONE',  ( -11.72566050890000078, 1483.562230513489794, 228.3064628327989851 ) ) ;
#13246=CARTESIAN_POINT ( 'NONE',  ( 4.642066325181019693, 1484.267353360819925, 220.0190218960080131 ) ) ;
#13248=CARTESIAN_POINT ( 'NONE',  ( -3.957094129160000140, 1456.622155725689936, 217.7529547663189931 ) ) ;
#13251=ORIENTED_EDGE ( 'NONE', *, *, #110557, .F. ) ;
#13254=VERTEX_POINT ( 'NONE', #10534 ) ;
#13257=CARTESIAN_POINT ( 'NONE',  ( -8.949286084602180225, 1447.532838897989905, 212.1309938496879965 ) ) ;
#13263=B_SPLINE_SURFACE_WITH_KNOTS ( 'NONE', 5, 1, ( 
 ( #91994, #49462 ),
 ( #108246, #84141 ),
 ( #108801, #93092 ),
 ( #15271, #16363 ),
 ( #110453, #50562 ),
 ( #82505, #42153 ) ),
 .UNSPECIFIED., .F., .F., .F.,
 ( 6, 6 ),
 ( 2, 2 ),
 ( 0.000000000000000000, 3.454439543779999955 ),
 ( 0.000000000000000000, 14.00000000000000000 ),
 .UNSPECIFIED. ) ;
#13266=B_SPLINE_CURVE_WITH_KNOTS ( 'NONE', 5,
 ( #105299, #20175, #95792, #77895, #52706, #86841 ),
 .UNSPECIFIED., .F., .F.,
 ( 6, 6 ),
 ( 0.000000000000000000, 1.000000000000000000 ),
 .UNSPECIFIED. ) ;
#13268=CARTESIAN_POINT ( 'NONE',  ( 10.51055417280000093, 1471.685891545489994, 212.2894659362390257 ) ) ;
#13277=CARTESIAN_POINT ( 'NONE',  ( -2.080140501524690322, 1467.944488986910301, 220.0539240431270116 ) ) ;
#13284=CARTESIAN_POINT ( 'NONE',  ( 5.178005602700659793, 1441.912561073429970, 216.3756019184010029 ) ) ;
#13298=CARTESIAN_POINT ( 'NONE',  ( 10.56851139279999963, 1489.654861728290143, 206.0672006338689926 ) ) ;
#13299=CARTESIAN_POINT ( 'NONE',  ( -3.494989020446679806, 1476.662911819639930, 199.3633622754599912 ) ) ;
#13306=CARTESIAN_POINT ( 'NONE',  ( -3.263114576272079827E-31, 1414.677402202029953, 209.1218459616989946 ) ) ;
#13307=CARTESIAN_POINT ( 'NONE',  ( -16.10161876792589908, 1508.453223452970178, 214.3744947141610169 ) ) ;
#13309=CARTESIAN_POINT ( 'NONE',  ( 19.37040130519999792, 1457.792564341990101, 211.0127811088189844 ) ) ;
#13316=CARTESIAN_POINT ( 'NONE',  ( -10.32197686275740089, 1470.787254133000033, 211.3220767278949950 ) ) ;
#13317=CARTESIAN_POINT ( 'NONE',  ( 10.99775799211320049, 1499.987872926449882, 204.6284785093779988 ) ) ;
#13319=EDGE_CURVE ( 'NONE', #110093, #53118, #24297, .T. ) ;
#13321=VECTOR ( 'NONE', #20707, 1000.000000000000114 ) ;
#13325=CARTESIAN_POINT ( 'NONE',  ( -4.227553501430000082, 1441.218335795189887, 201.3833937247689789 ) ) ;
#13327=VECTOR ( 'NONE', #96941, 1000.000000000000000 ) ;
#13330=CARTESIAN_POINT ( 'NONE',  ( -11.00005007279999880, 1492.085135258889977, 210.0463809226660032 ) ) ;
#13331=CARTESIAN_POINT ( 'NONE',  ( -1.657661096414910107, 1508.551704408389924, 220.0807554094629666 ) ) ;
#13335=CARTESIAN_POINT ( 'NONE',  ( -11.81627054680200040, 1502.033420305900108, 208.8645209164289724 ) ) ;
#13337=CARTESIAN_POINT ( 'NONE',  ( -0.8521672233359980364, 1489.820358975390036, 188.1651792795989877 ) ) ;
#13338=ORIENTED_EDGE ( 'NONE', *, *, #12532, .T. ) ;
#13341=CARTESIAN_POINT ( 'NONE',  ( 4.391179462425729874, 1508.551704408389924, 205.0152113334139869 ) ) ;
#13344=CARTESIAN_POINT ( 'NONE',  ( -16.53114207763760035, 1465.611540855740031, 220.7423250375829866 ) ) ;
#13349=DIRECTION ( 'NONE',  ( -1.000000000000000000, 0.000000000000000000, 0.000000000000000000 ) ) ;
#13350=CARTESIAN_POINT ( 'NONE',  ( 8.847239431406803689, 1505.230286297941348, 216.6946609004857862 ) ) ;
#13351=CARTESIAN_POINT ( 'NONE',  ( 3.829620113920000346, 1515.551704408389924, 211.4519800804890224 ) ) ;
#13354=B_SPLINE_CURVE_WITH_KNOTS ( 'NONE', 5,
 ( #47127, #90200, #57196, #107016, #29756, #90763, #22991, #5673, #37616 ),
 .UNSPECIFIED., .F., .F.,
 ( 6, 3, 6 ),
 ( -3.000000000000000000, -1.500000000000000222, -5.116429209195416661E-07 ),
 .UNSPECIFIED. ) ;
#13356=CARTESIAN_POINT ( 'NONE',  ( 13.25104486714040775, 1460.521307829560101, 224.0262041468786265 ) ) ;
#13361=ORIENTED_EDGE ( 'NONE', *, *, #976, .F. ) ;
#13364=ADVANCED_FACE ( 'NONE', ( #29212 ), #68720, .T. ) ;
#13366=CARTESIAN_POINT ( 'NONE',  ( -18.71884693102710173, 1442.006986966149952, 209.9877030880639950 ) ) ;
#13368=CARTESIAN_POINT ( 'NONE',  ( 12.89505231660000106, 1420.989630775359956, 203.4267439564690108 ) ) ;
#13378=CARTESIAN_POINT ( 'NONE',  ( -8.822183969887010591, 1447.794223493370055, 211.9042362736150267 ) ) ;
#13384=CARTESIAN_POINT ( 'NONE',  ( 7.289056222716610023, 1425.011265941609963, 212.6780767636349765 ) ) ;
#13385=ORIENTED_EDGE ( 'NONE', *, *, #67252, .T. ) ;
#13388=CARTESIAN_POINT ( 'NONE',  ( -11.88865138995519999, 1491.218756537510217, 206.7026720337979953 ) ) ;
#13401=ORIENTED_EDGE ( 'NONE', *, *, #102475, .T. ) ;
#13402=CARTESIAN_POINT ( 'NONE',  ( 9.181081645171898842, 1450.963532761650185, 210.1934668057190265 ) ) ;
#13403=CARTESIAN_POINT ( 'NONE',  ( 6.345494395550000277, 1423.250787925290069, 195.0535775187989884 ) ) ;
#13409=CARTESIAN_POINT ( 'NONE',  ( 2.487921303217719871, 1508.551704408389924, 214.1089244078229967 ) ) ;
#13410=ORIENTED_EDGE ( 'NONE', *, *, #11224, .T. ) ;
#13416=CARTESIAN_POINT ( 'NONE',  ( 11.55221588404359956, 1480.217597516799970, 211.4789165460060190 ) ) ;
#13418=ORIENTED_EDGE ( 'NONE', *, *, #42680, .F. ) ;
#13421=CARTESIAN_POINT ( 'NONE',  ( -3.139802346294130242, 1508.551704408389924, 219.9904071531209979 ) ) ;
#13422=CARTESIAN_POINT ( 'NONE',  ( 5.726337297911710422, 1499.318321574760148, 199.1886870359400064 ) ) ;
#13425=CARTESIAN_POINT ( 'NONE',  ( 11.78997475979999976, 1420.248503611800061, 199.1713245500889968 ) ) ;
#13426=CARTESIAN_POINT ( 'NONE',  ( 0.7985270487440959686, 1475.099758008560002, 220.5147217360619720 ) ) ;
#13432=CARTESIAN_POINT ( 'NONE',  ( 10.90038547020369997, 1425.457621502399888, 206.5065321829229958 ) ) ;
#13441=CARTESIAN_POINT ( 'NONE',  ( 9.509695062716730263, 1426.375487959860038, 209.7904012934289995 ) ) ;
#13442=CARTESIAN_POINT ( 'NONE',  ( -6.404454395499999286, 1464.203453065390022, 200.1263287045289871 ) ) ;
#13444=CARTESIAN_POINT ( 'NONE',  ( 4.675254175260000089, 1430.199328422790131, 217.3863063698589997 ) ) ;
#13446=CARTESIAN_POINT ( 'NONE',  ( -16.61413016530000064, 1416.994763352589871, 207.8498519981289974 ) ) ;
#13452=CARTESIAN_POINT ( 'NONE',  ( 8.978117882695519469, 1435.738603067889699, 208.3990004362530044 ) ) ;
#13456=CARTESIAN_POINT ( 'NONE',  ( 3.745926128375240083, 1474.358832711759987, 219.9123296517309996 ) ) ;
#13463=CARTESIAN_POINT ( 'NONE',  ( 0.7576697579430009544, 1515.544658147190148, 204.9993528003190022 ) ) ;
#13472=CARTESIAN_POINT ( 'NONE',  ( -1.210798686530613288, 1483.997144534682093, 198.5025898468677212 ) ) ;
#13478=CARTESIAN_POINT ( 'NONE',  ( 8.001917699090000724, 1477.391948627790043, 200.4742795864889899 ) ) ;
#13480=CARTESIAN_POINT ( 'NONE',  ( -11.12609304959999967, 1491.160356708789777, 209.7795734009459920 ) ) ;
#13488=CARTESIAN_POINT ( 'NONE',  ( -12.22594903035199998, 1490.655895506289880, 208.2081491493320016 ) ) ;
#13489=CARTESIAN_POINT ( 'NONE',  ( -4.903489893049830961, 1508.551704408389924, 205.9871227246740091 ) ) ;
#13493=CARTESIAN_POINT ( 'NONE',  ( -4.141727467620000880, 1502.720785751690073, 230.1321099188990047 ) ) ;
#13496=CONICAL_SURFACE ( 'NONE', #83223, 0.9999999999999962252, 1.047197551199999799 ) ;
#13497=CARTESIAN_POINT ( 'NONE',  ( 9.798888871456099992, 1470.345923341260004, 211.5472087270539987 ) ) ;
#13499=CARTESIAN_POINT ( 'NONE',  ( -11.21575968800000034, 1500.080311486090068, 211.0958765857290018 ) ) ;
#13504=B_SPLINE_SURFACE_WITH_KNOTS ( 'NONE', 5, 1, ( 
 ( #58705, #95472 ),
 ( #26597, #92837 ),
 ( #84445, #18738 ),
 ( #41349, #44525 ),
 ( #7731, #78671 ),
 ( #60794, #52390 ),
 ( #52933, #94920 ),
 ( #1989, #19288 ),
 ( #75517, #92287 ) ),
 .UNSPECIFIED., .F., .F., .F.,
 ( 6, 3, 6 ),
 ( 2, 2 ),
 ( 0.000000000000000000, 3.644587434069999965, 7.267547310080000322 ),
 ( 0.000000000000000000, 14.00000000000000000 ),
 .UNSPECIFIED. ) ;
#13506=CARTESIAN_POINT ( 'NONE',  ( -9.563909551760000127, 1464.644246208489903, 228.2425506381989919 ) ) ;
#13517=ORIENTED_EDGE ( 'NONE', *, *, #30305, .T. ) ;
#13518=CARTESIAN_POINT ( 'NONE',  ( -7304.654438325449519, 5182.767774292097783, -10649.19336541359553 ) ) ;
#13522=ORIENTED_EDGE ( 'NONE', *, *, #85721, .T. ) ;
#13523=CARTESIAN_POINT ( 'NONE',  ( 4.326079331027290031, 1515.193466796180928, 207.2788825876957048 ) ) ;
#13525=CARTESIAN_POINT ( 'NONE',  ( 0.7917928493246050303, 1485.631538064390043, 220.9725313029949803 ) ) ;
#13531=B_SPLINE_CURVE_WITH_KNOTS ( 'NONE', 3,
 ( #6191, #49315, #40343, #15662, #7300, #31942, #66137, #83441, #6736, #109224 ),
 .UNSPECIFIED., .F., .F.,
 ( 4, 2, 2, 2, 4 ),
 ( 0.000000000000000000, 0.2500000000000000555, 0.5000000000000001110, 0.7500000000000000000, 1.000000000000000000 ),
 .UNSPECIFIED. ) ;
#13535=CARTESIAN_POINT ( 'NONE',  ( 10.24469654192340151, 1481.487780100139844, 213.2148028526819985 ) ) ;
#13541=CARTESIAN_POINT ( 'NONE',  ( -9.104803454449999833, 1421.479062531979935, 192.1853131694989827 ) ) ;
#13542=CARTESIAN_POINT ( 'NONE',  ( 10.46269364489999987, 1491.122602117189899, 212.5073291737689942 ) ) ;
#13547=CARTESIAN_POINT ( 'NONE',  ( 12.55779355105019945, 1500.097530588729796, 207.3428969177340093 ) ) ;
#13548=CARTESIAN_POINT ( 'NONE',  ( -2.330134120368332784, 1515.551704408390151, 213.0801841075446248 ) ) ;
#13551=CARTESIAN_POINT ( 'NONE',  ( 1.951019270089999980, 1465.893727891289927, 198.2556634289990143 ) ) ;
#13558=VERTEX_POINT ( 'NONE', #59945 ) ;
#13566=CARTESIAN_POINT ( 'NONE',  ( -9.614403431034910241, 1461.326383761360148, 207.8336058208969916 ) ) ;
#13567=CARTESIAN_POINT ( 'NONE',  ( -9.473155674714520913, 1437.814104512410040, 211.9418041017489713 ) ) ;
#13576=CARTESIAN_POINT ( 'NONE',  ( -10.32752872691269985, 1480.656876279547532, 207.0167722732371942 ) ) ;
#13581=CARTESIAN_POINT ( 'NONE',  ( 3.272123973761280169, 1515.551704204689941, 212.7661975563979979 ) ) ;
#13583=CARTESIAN_POINT ( 'NONE',  ( -10.61669498371649922, 1508.551704408389924, 207.6874897006059939 ) ) ;
#13588=CARTESIAN_POINT ( 'NONE',  ( -7.527539147472119829, 1439.311770005190056, 204.6539930853050180 ) ) ;
#13595=ORIENTED_EDGE ( 'NONE', *, *, #37154, .F. ) ;
#13598=CARTESIAN_POINT ( 'NONE',  ( 0.7147294630619990263, 1515.255091259190067, 213.4463119403589815 ) ) ;
#13599=CARTESIAN_POINT ( 'NONE',  ( 10.92694110706779931, 1489.979356094880131, 208.4358879340020110 ) ) ;
#13601=EDGE_CURVE ( 'NONE', #93500, #19377, #44586, .T. ) ;
#13610=CARTESIAN_POINT ( 'NONE',  ( -11.25901873340000137, 1500.172003384790059, 210.8567363195689950 ) ) ;
#13617=CARTESIAN_POINT ( 'NONE',  ( -12.17813008270000097, 1438.571549855089870, 224.0393728361989929 ) ) ;
#13621=CARTESIAN_POINT ( 'NONE',  ( 4.487249773072029768, 1509.038615930399828, 211.6097810847319920 ) ) ;
#13623=CARTESIAN_POINT ( 'NONE',  ( 12.11998591773940070, 1491.481808809230188, 207.0704772481079772 ) ) ;
#13627=CARTESIAN_POINT ( 'NONE',  ( 12.62071130547100140, 1421.509729680500186, 206.8448693545120136 ) ) ;
#13638=CARTESIAN_POINT ( 'NONE',  ( 7.455956092950000169, 1426.129841999370001, 212.4361423238889870 ) ) ;
#13639=CARTESIAN_POINT ( 'NONE',  ( 24.11200011979999758, 1496.633574749990203, 206.8275458132090137 ) ) ;
#13641=CARTESIAN_POINT ( 'NONE',  ( -23.08547268613130043, 1417.322834144340050, 209.8740766914669962 ) ) ;
#13665=CARTESIAN_POINT ( 'NONE',  ( 2.664535259099999805E-15, 1420.121162737279974, 209.1218459616989946 ) ) ;
#13667=ORIENTED_EDGE ( 'NONE', *, *, #108159, .T. ) ;
#13676=CARTESIAN_POINT ( 'NONE',  ( -12.99430343120000053, 1503.123593417290067, 208.6821788852620045 ) ) ;
#13691=EDGE_LOOP ( 'NONE', ( #98945, #53018, #85144, #100202, #109761, #76620 ) ) ;
#13695=CARTESIAN_POINT ( 'NONE',  ( 20.41258333560000082, 1494.156730172889866, 204.1224707391089908 ) ) ;
#13701=CARTESIAN_POINT ( 'NONE',  ( -0.6587146994840009651, 1442.893519126590036, 219.0943606518089837 ) ) ;
#13706=DIRECTION ( 'NONE',  ( 0.000000000000000000, -1.000000000000000000, 1.836970198721029688E-16 ) ) ;
#13714=ADVANCED_FACE ( 'NONE', ( #68350 ), #34719, .T. ) ;
#13718=CARTESIAN_POINT ( 'NONE',  ( 11.44494620870000112, 1422.175562347540108, 206.4125902192689921 ) ) ;
#13721=CARTESIAN_POINT ( 'NONE',  ( -16.32516330111020153, 1416.706030269645225, 208.2451548885862564 ) ) ;
#13724=ORIENTED_EDGE ( 'NONE', *, *, #93831, .T. ) ;
#13732=CARTESIAN_POINT ( 'NONE',  ( 8.961967794501056517, 1424.998307906903619, 195.6926762925650110 ) ) ;
#13734=CARTESIAN_POINT ( 'NONE',  ( 2.353483798069999633, 1441.866266782089951, 218.3762686079190019 ) ) ;
#13746=CARTESIAN_POINT ( 'NONE',  ( -16.39029410570000067, 1508.551704408389924, 213.5052586272289830 ) ) ;
#13748=FACE_OUTER_BOUND ( 'NONE', #69950, .T. ) ;
#13752=VECTOR ( 'NONE', #101987, 1000.000000000000000 ) ;
#13758=CARTESIAN_POINT ( 'NONE',  ( -15.27276080761430066, 1415.677402202069970, 208.6833046621170240 ) ) ;
#13760=CARTESIAN_POINT ( 'NONE',  ( 6.634516952019999358, 1427.014769761329944, 214.0188387700289923 ) ) ;
#13767=CARTESIAN_POINT ( 'NONE',  ( -12.30179092849999911, 1502.247259483089920, 210.0097377508620013 ) ) ;
#13773=EDGE_CURVE ( 'NONE', #42556, #71088, #26302, .T. ) ;
#13780=CARTESIAN_POINT ( 'NONE',  ( 0.1141777316373559920, 1515.158022524200078, 213.4488534336589964 ) ) ;
#13782=CARTESIAN_POINT ( 'NONE',  ( -6.593308786588120363, 1477.792378428569918, 218.6399986688279853 ) ) ;
#13789=CARTESIAN_POINT ( 'NONE',  ( 19.28284482985129955, 1498.021048960190001, 221.9090220746840316 ) ) ;
#13795=CARTESIAN_POINT ( 'NONE',  ( 4.327096512618459734, 1515.154622198469951, 209.3777992006019701 ) ) ;
#13798=CARTESIAN_POINT ( 'NONE',  ( -3.776193667280000277, 1457.838857791890177, 218.3090359982990094 ) ) ;
#13820=CARTESIAN_POINT ( 'NONE',  ( 1.332267629549999902E-15, 1391.913060387289988, 209.1218459616989946 ) ) ;
#13831=AXIS2_PLACEMENT_3D ( 'NONE', #42530, #91825, #43094 ) ;
#13834=EDGE_CURVE ( 'NONE', #84259, #16269, #86685, .T. ) ;
#13837=CARTESIAN_POINT ( 'NONE',  ( 8.311313017077319287, 1438.191820040039829, 214.6582622035640213 ) ) ;
#13838=DIRECTION ( 'NONE',  ( -9.120877578445558697E-47, 1.000000000000000000, -1.836970198721029688E-16 ) ) ;
#13841=EDGE_LOOP ( 'NONE', ( #107525, #1979, #32965, #84928 ) ) ;
#13849=LINE ( 'NONE', #48033, #61073 ) ;
#13862=EDGE_CURVE ( 'NONE', #53297, #36343, #46901, .T. ) ;
#13865=CARTESIAN_POINT ( 'NONE',  ( 0.9117115396459989363, 1473.693686166890075, 219.3348546764989919 ) ) ;
#13870=CARTESIAN_POINT ( 'NONE',  ( -4.329448781177520189, 1515.064792686469900, 210.9648092169189795 ) ) ;
#13872=CARTESIAN_POINT ( 'NONE',  ( -10.26524962935310015, 1471.547416617549970, 209.8736591177010098 ) ) ;
#13881=CARTESIAN_POINT ( 'NONE',  ( 11.36218962193319904, 1502.758839311570000, 211.1250559367580024 ) ) ;
#13891=CARTESIAN_POINT ( 'NONE',  ( -12.18420476197879943, 1502.395317283280065, 208.9521721262090068 ) ) ;
#13893=CARTESIAN_POINT ( 'NONE',  ( -4.848919996459999382, 1489.192135936889827, 188.8958457811990002 ) ) ;
#13897=CARTESIAN_POINT ( 'NONE',  ( -4.124924170559999936, 1474.647204749290040, 198.4545245537989899 ) ) ;
#13900=CARTESIAN_POINT ( 'NONE',  ( 7.755350745836239845, 1459.738700650969804, 228.9106056711640065 ) ) ;
#13908=CARTESIAN_POINT ( 'NONE',  ( 9.549000552458089430, 1470.075890067440014, 212.3436661921319910 ) ) ;
#13909=CARTESIAN_POINT ( 'NONE',  ( 7.731549308429999989, 1490.593532645290225, 209.4666211040999997 ) ) ;
#13913=CARTESIAN_POINT ( 'NONE',  ( -2.170627987649289992, 1485.611815795640041, 197.4219879416550327 ) ) ;
#13923=EDGE_CURVE ( 'NONE', #103948, #70633, #97645, .T. ) ;
#13930=CARTESIAN_POINT ( 'NONE',  ( 19.35628570429999940, 1496.398810548190113, 218.7515486585290034 ) ) ;
#13931=EDGE_CURVE ( 'NONE', #109119, #21788, #76219, .T. ) ;
#13934=CIRCLE ( 'NONE', #4996, 12.73448142120000171 ) ;
#13938=CARTESIAN_POINT ( 'NONE',  ( -3.262203552877475765, 1455.259740959270175, 200.2677761270983297 ) ) ;
#13940=CARTESIAN_POINT ( 'NONE',  ( 7.231911623789289756, 1424.971209983940071, 212.7891681502780159 ) ) ;
#13952=ORIENTED_EDGE ( 'NONE', *, *, #2554, .T. ) ;
#13956=CARTESIAN_POINT ( 'NONE',  ( 10.94703604719999923, 1501.632067650890122, 205.7462135331290085 ) ) ;
#13962=EDGE_CURVE ( 'NONE', #31336, #714, #104390, .T. ) ;
#13965=CARTESIAN_POINT ( 'NONE',  ( 7.557982130680000132, 1491.185578662290027, 210.9716881467189751 ) ) ;
#13980=ORIENTED_EDGE ( 'NONE', *, *, #100225, .F. ) ;
#13987=CARTESIAN_POINT ( 'NONE',  ( 19.33082836830000062, 1455.567049562989951, 210.0625852571630219 ) ) ;
#13989=CARTESIAN_POINT ( 'NONE',  ( -9.783936618240000271, 1438.409968277489952, 210.7790527803989846 ) ) ;
#13993=CARTESIAN_POINT ( 'NONE',  ( 12.11307097544860056, 1426.902643091930031, 206.5905068478429882 ) ) ;
#13995=CARTESIAN_POINT ( 'NONE',  ( -9.810612324704180764, 1440.011860597360055, 207.1182720801899961 ) ) ;
#13999=CARTESIAN_POINT ( 'NONE',  ( 8.968032268709999144, 1477.614756788489785, 227.8520689727990032 ) ) ;
#14003=CARTESIAN_POINT ( 'NONE',  ( 9.362196585121042247, 1423.087187200049812, 210.9628769778060189 ) ) ;
#14004=CARTESIAN_POINT ( 'NONE',  ( 11.21861042134139907, 1425.044613964269956, 203.0203497653440081 ) ) ;
#14006=CARTESIAN_POINT ( 'NONE',  ( 3.789103669029999732, 1428.956962167089841, 216.4960976464589919 ) ) ;
#14010=CARTESIAN_POINT ( 'NONE',  ( 9.327651199099038948, 1434.415569083649871, 206.2244204008570136 ) ) ;
#14012=CARTESIAN_POINT ( 'NONE',  ( 5.291552456182019526, 1457.527819738830203, 199.7187647539589932 ) ) ;
#14018=CARTESIAN_POINT ( 'NONE',  ( -3.703568358935259930, 1497.311626042180023, 220.9591690318370070 ) ) ;
#14022=CARTESIAN_POINT ( 'NONE',  ( 0.7322251555290010261, 1515.253704548189944, 204.7973436813889805 ) ) ;
#14032=CARTESIAN_POINT ( 'NONE',  ( -0.7433232216159980643, 1450.780014651390047, 189.8792753856990032 ) ) ;
#14035=B_SPLINE_CURVE_WITH_KNOTS ( 'NONE', 5,
 ( #36096, #80301, #70836, #104946, #88709, #44498 ),
 .UNSPECIFIED., .F., .F.,
 ( 6, 6 ),
 ( 0.000000000000000000, 1.000000000000000000 ),
 .UNSPECIFIED. ) ;
#14036=CARTESIAN_POINT ( 'NONE',  ( 5.085252852200000007, 1478.772695843590100, 199.8786784519290052 ) ) ;
#14038=CARTESIAN_POINT ( 'NONE',  ( -11.81643738809999888, 1490.595564134589722, 209.0680961509349913 ) ) ;
#14048=CARTESIAN_POINT ( 'NONE',  ( -4.849688736979540060, 1508.551704408389924, 205.8172135933860147 ) ) ;
#14052=CARTESIAN_POINT ( 'NONE',  ( 3.048018904480000124, 1501.579531795289995, 230.2806870085990170 ) ) ;
#14056=CARTESIAN_POINT ( 'NONE',  ( 10.91646513216940129, 1471.120537862260107, 210.1608033267570192 ) ) ;
#14064=CARTESIAN_POINT ( 'NONE',  ( -9.541049972259999734, 1464.842190924689930, 228.2655280639989996 ) ) ;
#14085=CARTESIAN_POINT ( 'NONE',  ( 11.85459489379999987, 1500.917690086590255, 208.6046474440059910 ) ) ;
#14089=EDGE_CURVE ( 'NONE', #89963, #1678, #57604, .T. ) ;
#14092=CARTESIAN_POINT ( 'NONE',  ( 7.192202089616840155, 1484.368469734710061, 217.2056949635710055 ) ) ;
#14097=CARTESIAN_POINT ( 'NONE',  ( -22.15968245387939817, 1485.573395578509917, 217.2083751193320040 ) ) ;
#14098=CARTESIAN_POINT ( 'NONE',  ( -1.150312585214009919, 1431.780365134439990, 200.7950712129770068 ) ) ;
#14099=ORIENTED_EDGE ( 'NONE', *, *, #44566, .F. ) ;
#14106=VECTOR ( 'NONE', #52320, 1000.000000000000000 ) ;
#14109=CARTESIAN_POINT ( 'NONE',  ( 12.63295115314390848, 1420.317390383416978, 200.3640917624317410 ) ) ;
#14111=FACE_OUTER_BOUND ( 'NONE', #42625, .T. ) ;
#14114=ORIENTED_EDGE ( 'NONE', *, *, #76651, .F. ) ;
#14126=CARTESIAN_POINT ( 'NONE',  ( -10.52899351214830048, 1462.479394878560015, 207.9464375330440191 ) ) ;
#14145=CARTESIAN_POINT ( 'NONE',  ( 3.982959079218740595, 1515.551843419029865, 211.9714081247090292 ) ) ;
#14154=CARTESIAN_POINT ( 'NONE',  ( -2.586254842240000240, 1431.686802674690171, 214.1917715254589893 ) ) ;
#14155=CARTESIAN_POINT ( 'NONE',  ( -6.058566992285000730, 1440.303333100529926, 202.7033299732119929 ) ) ;
#14160=CARTESIAN_POINT ( 'NONE',  ( -11.57364750537059805, 1482.638710595820157, 206.3005749242109914 ) ) ;
#14169=CARTESIAN_POINT ( 'NONE',  ( 2.983564572711930651, 1464.490552568307066, 199.7433000633449467 ) ) ;
#14171=CARTESIAN_POINT ( 'NONE',  ( -10.15733737953619986, 1447.239609962909981, 211.0279899296229758 ) ) ;
#14176=CARTESIAN_POINT ( 'NONE',  ( -11.02815901449999991, 1500.365335154690001, 213.0134302711989847 ) ) ;
#14188=B_SPLINE_SURFACE_WITH_KNOTS ( 'NONE', 5, 5, ( 
 ( #105786, #38550, #38017, #106317, #78932, #21173 ),
 ( #11710, #104663, #89512, #71100, #12803, #37464 ),
 ( #46983, #105224, #62142, #96268, #45882, #20100 ),
 ( #81107, #72728, #106853, #30144, #27959, #11177 ),
 ( #19545, #53753, #3340, #87886, #79477, #80019 ),
 ( #74395, #82207, #66552, #109090, #90609, #5512 ) ),
 .UNSPECIFIED., .F., .F., .F.,
 ( 6, 6 ),
 ( 6, 6 ),
 ( 7.548574938123289613, 12.57628284734769863 ),
 ( 0.000000000000000000, 0.5000183579477079920 ),
 .UNSPECIFIED. ) ;
#14193=CARTESIAN_POINT ( 'NONE',  ( 12.84018448277500113, 1421.301739308270044, 205.5319240985589886 ) ) ;
#14195=VERTEX_POINT ( 'NONE', #60726 ) ;
#14196=B_SPLINE_SURFACE_WITH_KNOTS ( 'NONE', 5, 5, ( 
 ( #10618, #17317, #10052, #11181, #51512, #9500 ),
 ( #44786, #87323, #26860, #85644, #62146, #17877 ),
 ( #52074, #78936, #36358, #2789, #95718, #86207 ),
 ( #52626, #95170, #71104, #18983, #8944, #61047 ),
 ( #43665, #77817, #61585, #18426, #45343, #79482 ),
 ( #53180, #86763, #43117, #44226, #77277, #70549 ) ),
 .UNSPECIFIED., .F., .F., .F.,
 ( 6, 6 ),
 ( 6, 6 ),
 ( 0.000000000000000000, 2.079987011550000098 ),
 ( 0.000000000000000000, 2.000000000000000000 ),
 .UNSPECIFIED. ) ;
#14199=CARTESIAN_POINT ( 'NONE',  ( 2.740685684163910008, 1426.136188963130053, 188.7843764270949976 ) ) ;
#14203=CARTESIAN_POINT ( 'NONE',  ( -8.881784197000000993E-16, 1392.213060387289943, 209.1218459616989946 ) ) ;
#14208=CARTESIAN_POINT ( 'NONE',  ( 7.666825005110000646, 1426.360134655189995, 212.0592671631690109 ) ) ;
#14223=CARTESIAN_POINT ( 'NONE',  ( -15.92986207429999901, 1416.139014782290133, 209.7537124246929920 ) ) ;
#14224=CARTESIAN_POINT ( 'NONE',  ( 2.618187928979999857, 1445.209012209990078, 200.3785934838089986 ) ) ;
#14228=CARTESIAN_POINT ( 'NONE',  ( 2.132506400839999650, 1418.942295325089844, 204.3612836522989937 ) ) ;
#14236=VERTEX_POINT ( 'NONE', #41686 ) ;
#14246=CARTESIAN_POINT ( 'NONE',  ( -11.40405654770000154, 1501.068632103089840, 208.2804062866189838 ) ) ;
#14255=EDGE_CURVE ( 'NONE', #1934, #58146, #68018, .T. ) ;
#14259=ORIENTED_EDGE ( 'NONE', *, *, #100225, .T. ) ;
#14263=CARTESIAN_POINT ( 'NONE',  ( -14.00462132320000030, 1415.677402202029953, 214.2425697179989754 ) ) ;
#14268=CARTESIAN_POINT ( 'NONE',  ( 0.02750565378459880056, 1442.646891867090062, 219.1054768861489777 ) ) ;
#14278=LINE ( 'NONE', #84248, #52163 ) ;
#14279=PRODUCT ( 'Feed Screw', 'Feed Screw', '', ( #81854 ) ) ;
#14283=CARTESIAN_POINT ( 'NONE',  ( 11.19329478399999900, 1422.593227753940027, 205.2156856529389870 ) ) ;
#14292=ORIENTED_EDGE ( 'NONE', *, *, #90099, .T. ) ;
#14296=CARTESIAN_POINT ( 'NONE',  ( 10.87641374706830177, 1461.647512902760127, 210.5511653657890179 ) ) ;
#14297=CARTESIAN_POINT ( 'NONE',  ( 8.406304952171057110, 1424.431735268568445, 195.8247349441674032 ) ) ;
#14298=CARTESIAN_POINT ( 'NONE',  ( 2.594761893819999887, 1441.567844146989955, 218.7008844616090073 ) ) ;
#14302=CARTESIAN_POINT ( 'NONE',  ( 7.432030730716068234, 1487.100624600356241, 201.2524259029208054 ) ) ;
#14307=ORIENTED_EDGE ( 'NONE', *, *, #60175, .T. ) ;
#14309=CARTESIAN_POINT ( 'NONE',  ( 11.19358401111760060, 1470.358879059469928, 207.1653923726030087 ) ) ;
#14310=DIRECTION ( 'NONE',  ( -1.000000000000000000, 0.000000000000000000, 0.000000000000000000 ) ) ;
#14318=CARTESIAN_POINT ( 'NONE',  ( -14.01525996361490023, 1415.677402202029953, 204.0303134510289738 ) ) ;
#14319=ADVANCED_FACE ( 'NONE', ( #66910 ), #86444, .T. ) ;
#14321=CARTESIAN_POINT ( 'NONE',  ( -8.551515107930001136, 1437.707591943389843, 226.0657740139990040 ) ) ;
#14326=ORIENTED_EDGE ( 'NONE', *, *, #57405, .T. ) ;
#14335=FACE_OUTER_BOUND ( 'NONE', #104524, .T. ) ;
#14336=CARTESIAN_POINT ( 'NONE',  ( 9.708970498318210574, 1463.715168242549908, 210.4580945914069900 ) ) ;
#14347=CARTESIAN_POINT ( 'NONE',  ( -13.56738355449999922, 1505.237168496690174, 227.8242396965990224 ) ) ;
#14349=CARTESIAN_POINT ( 'NONE',  ( -1.924402692774775270, 1474.171439542113376, 219.1969456462446431 ) ) ;
#14353=CARTESIAN_POINT ( 'NONE',  ( 4.327986479516090057, 1515.120635733899917, 209.9709076042840081 ) ) ;
#14355=CARTESIAN_POINT ( 'NONE',  ( 10.03380816088620087, 1469.200710370999786, 209.4646523673320075 ) ) ;
#14356=CARTESIAN_POINT ( 'NONE',  ( -3.738989945110000157, 1456.530141059690095, 217.8454007011089857 ) ) ;
#14360=ORIENTED_EDGE ( 'NONE', *, *, #32911, .T. ) ;
#14366=CARTESIAN_POINT ( 'NONE',  ( -17.64250891069632843, 1419.640929922183432, 207.0584130580827207 ) ) ;
#14389=CARTESIAN_POINT ( 'NONE',  ( 6.083541831545586476, 1460.052579242508727, 201.6434494505425334 ) ) ;
#14391=CARTESIAN_POINT ( 'NONE',  ( 5.878018521898390247, 1440.945822282649942, 215.8104943704309733 ) ) ;
#14397=CARTESIAN_POINT ( 'NONE',  ( -10.93621683099999942, 1471.189486259790101, 208.1842957432819787 ) ) ;
#14404=CARTESIAN_POINT ( 'NONE',  ( -11.40252061979999887, 1416.855034940659834, 204.2434678627789992 ) ) ;
#14407=CARTESIAN_POINT ( 'NONE',  ( 3.773762947180000271, 1486.021325443789920, 199.0256766443990273 ) ) ;
#14410=EDGE_CURVE ( 'NONE', #23318, #22363, #46680, .T. ) ;
#14412=CARTESIAN_POINT ( 'NONE',  ( 18.14949073579999705, 1432.344282874789997, 211.8258969992290019 ) ) ;
#14418=CARTESIAN_POINT ( 'NONE',  ( -15.62742587511660020, 1508.451903174239987, 214.8815429522870204 ) ) ;
#14419=CARTESIAN_POINT ( 'NONE',  ( 1.617204962490000009, 1473.963834395889990, 219.3699064269989947 ) ) ;
#14423=CARTESIAN_POINT ( 'NONE',  ( -2.933467300942110167, 1454.462654904609963, 199.0544936251469892 ) ) ;
#14425=B_SPLINE_SURFACE_WITH_KNOTS ( 'NONE', 5, 5, ( 
 ( #320, #69172, #50695, #67519, #34445, #86496 ),
 ( #8127, #68621, #102723, #26017, #60214, #24908 ),
 ( #9790, #17610, #94332, #42293, #85952, #94907 ),
 ( #9253, #18181, #77561, #866, #103278, #43957 ),
 ( #19839, #28809, #27701, #96567, #87052, #54044 ),
 ( #12553, #1976, #54586, #88722, #71954, #71405 ),
 ( #35542, #79776, #87621, #36111, #89258, #3083 ),
 ( #11462, #55138, #106065, #36654, #46731, #80865 ),
 ( #103855, #69737, #18722, #45082, #37210, #44512 ) ),
 .UNSPECIFIED., .F., .F., .F.,
 ( 6, 3, 6 ),
 ( 6, 6 ),
 ( 12.02292824550000105, 22.14719212230000167, 26.06149361980000023 ),
 ( 0.000000000000000000, 2.000000000000000000 ),
 .UNSPECIFIED. ) ;
#14427=CARTESIAN_POINT ( 'NONE',  ( -9.915141243902969137, 1471.119519607170105, 211.8083852528800151 ) ) ;
#14428=CARTESIAN_POINT ( 'NONE',  ( 10.00306449797230002, 1469.399223428769801, 210.0757042779839878 ) ) ;
#14434=CARTESIAN_POINT ( 'NONE',  ( -3.578533967270000282, 1442.500416740689843, 200.8327418449289894 ) ) ;
#14435=CARTESIAN_POINT ( 'NONE',  ( 11.35344352881629959, 1502.969967087519990, 211.0626227285410152 ) ) ;
#14437=VECTOR ( 'NONE', #76896, 1000.000000000000000 ) ;
#14438=CARTESIAN_POINT ( 'NONE',  ( 10.80761588395260020, 1422.264295156030130, 211.0685490254289789 ) ) ;
#14440=CARTESIAN_POINT ( 'NONE',  ( 1.108124621956710021, 1508.551704408389924, 219.8565429179099908 ) ) ;
#14445=ADVANCED_FACE ( 'NONE', ( #37703 ), #17704, .T. ) ;
#14447=CARTESIAN_POINT ( 'NONE',  ( -12.30475894872500042, 1502.479826408779900, 208.9714260491429911 ) ) ;
#14452=ORIENTED_EDGE ( 'NONE', *, *, #91698, .T. ) ;
#14456=CARTESIAN_POINT ( 'NONE',  ( 4.072632511270110278, 1508.551704408389924, 204.7001764067349825 ) ) ;
#14461=CARTESIAN_POINT ( 'NONE',  ( -4.324121571198319636, 1515.222544082249897, 206.1650193910969904 ) ) ;
#14463=CARTESIAN_POINT ( 'NONE',  ( -5.142705184740000490, 1462.990135410090033, 200.8040030810390135 ) ) ;
#14466=CARTESIAN_POINT ( 'NONE',  ( 4.326079330760677522, 1515.193466806362267, 211.4519800883807079 ) ) ;
#14472=CARTESIAN_POINT ( 'NONE',  ( 7.647588771564749699, 1433.658576088640075, 203.7587819791999948 ) ) ;
#14483=CARTESIAN_POINT ( 'NONE',  ( -15.24773871110000023, 1420.384425983460005, 211.9003051376789983 ) ) ;
#14494=CARTESIAN_POINT ( 'NONE',  ( 2.958237723154419463, 1515.068899831249155, 204.7925047457962648 ) ) ;
#14495=CARTESIAN_POINT ( 'NONE',  ( 7.439392163950960146, 1425.194634625760045, 212.3718729812599975 ) ) ;
#14509=CARTESIAN_POINT ( 'NONE',  ( -3.030912759255987243, 1457.699420191448780, 218.6115341449503262 ) ) ;
#14512=CARTESIAN_POINT ( 'NONE',  ( 10.41028103169999852, 1461.975860366590041, 210.7993106899690190 ) ) ;
#14513=ORIENTED_EDGE ( 'NONE', *, *, #88115, .T. ) ;
#14523=CARTESIAN_POINT ( 'NONE',  ( 4.058335268219130931, 1508.551704408389924, 213.8008226954089821 ) ) ;
#14527=CARTESIAN_POINT ( 'NONE',  ( -6.465298943309999657, 1427.283379109839871, 203.6615921516590220 ) ) ;
#14532=CARTESIAN_POINT ( 'NONE',  ( 6.822769659250000451, 1469.182992717989691, 208.8962877339269824 ) ) ;
#14534=ORIENTED_EDGE ( 'NONE', *, *, #106284, .T. ) ;
#14536=CARTESIAN_POINT ( 'NONE',  ( -10.37614225292699999, 1479.403275255469907, 210.6296033183759846 ) ) ;
#14537=CARTESIAN_POINT ( 'NONE',  ( -2.688576586735480056, 1508.385808335360025, 220.6470044136009960 ) ) ;
#14539=CARTESIAN_POINT ( 'NONE',  ( 10.24150551940120124, 1502.975079637399858, 216.6982935228119800 ) ) ;
#14540=CARTESIAN_POINT ( 'NONE',  ( 10.45480669290000009, 1420.576652099880221, 197.8458654235990082 ) ) ;
#14541=CARTESIAN_POINT ( 'NONE',  ( 1.690297610143600027, 1474.866452951810061, 220.4152850073089667 ) ) ;
#14543=CARTESIAN_POINT ( 'NONE',  ( -5.038226297060000469, 1495.449696765989984, 198.6986880815990162 ) ) ;
#14547=CARTESIAN_POINT ( 'NONE',  ( 11.95048161449970081, 1426.790502429370008, 206.5664867952030193 ) ) ;
#14558=CARTESIAN_POINT ( 'NONE',  ( 11.14534346802929932, 1422.715803301600090, 203.3389832068340013 ) ) ;
#14560=CARTESIAN_POINT ( 'NONE',  ( 1.839725546759999775, 1430.652037411689889, 217.6678242507890104 ) ) ;
#14562=EDGE_CURVE ( 'NONE', #106368, #78107, #41520, .T. ) ;
#14565=CARTESIAN_POINT ( 'NONE',  ( 3.967440335210983271, 1431.784492063039352, 200.3531908705770093 ) ) ;
#14568=ADVANCED_FACE ( 'NONE', ( #19647 ), #42823, .T. ) ;
#14575=VECTOR ( 'NONE', #51913, 1000.000000000000000 ) ;
#14578=DIRECTION ( 'NONE',  ( -0.9391860388032872153, -1.840964726716158065E-08, 0.3434087717531252304 ) ) ;
#14580=CARTESIAN_POINT ( 'NONE',  ( 12.67629937430701936, 1426.478869958664063, 202.7079000866955028 ) ) ;
#14582=CARTESIAN_POINT ( 'NONE',  ( 20.33508568879010170, 1432.834458530000120, 214.7556887718170060 ) ) ;
#14591=CARTESIAN_POINT ( 'NONE',  ( -11.18562212430000002, 1414.421228241719973, 212.6817167181389721 ) ) ;
#14592=CARTESIAN_POINT ( 'NONE',  ( 2.175409717514719593E-31, 1397.551704408390151, 209.1218459616989946 ) ) ;
#14597=CARTESIAN_POINT ( 'NONE',  ( -11.01499743910000007, 1491.713862414889718, 209.6260353422130152 ) ) ;
#14607=CARTESIAN_POINT ( 'NONE',  ( -12.24955825400350129, 1490.502947928989897, 208.7174997126320193 ) ) ;
#14608=CARTESIAN_POINT ( 'NONE',  ( -4.751625979119149967, 1508.551704408389924, 205.5757039018049852 ) ) ;
#14614=CARTESIAN_POINT ( 'NONE',  ( -1.254332924399999882, 1509.200097453389844, 218.0171178735590161 ) ) ;
#14617=CARTESIAN_POINT ( 'NONE',  ( 10.18337656697590177, 1470.443896296289950, 210.2471389431320006 ) ) ;
#14620=CARTESIAN_POINT ( 'NONE',  ( -11.00301372470000061, 1492.094802143589959, 210.0154403701209844 ) ) ;
#14644=CARTESIAN_POINT ( 'NONE',  ( -2.298816259811510054, 1486.462377102800019, 220.8289805423670202 ) ) ;
#14645=CARTESIAN_POINT ( 'NONE',  ( 11.29999465100000045, 1500.851204880689920, 206.6218521946089766 ) ) ;
#14653=CARTESIAN_POINT ( 'NONE',  ( 12.69768439988109954, 1500.465451651789863, 208.8630517188479985 ) ) ;
#14657=CARTESIAN_POINT ( 'NONE',  ( -18.80013861839099931, 1505.319286544219949, 222.5373194665829999 ) ) ;
#14662=CARTESIAN_POINT ( 'NONE',  ( 10.56204787542680101, 1452.677117374779982, 209.7945773243330052 ) ) ;
#14663=CARTESIAN_POINT ( 'NONE',  ( 11.55221588404359956, 1480.217597516799970, 211.4789165460060190 ) ) ;
#14664=CARTESIAN_POINT ( 'NONE',  ( -21.12755052628529739, 1507.992901756090077, 209.5250462511280034 ) ) ;
#14666=VECTOR ( 'NONE', #38001, 1000.000000000000000 ) ;
#14670=CARTESIAN_POINT ( 'NONE',  ( -18.29243834081962206, 1484.963126390134676, 219.4937029363345573 ) ) ;
#14684=CARTESIAN_POINT ( 'NONE',  ( -18.22821675530000007, 1443.229620277490085, 204.5519556382290034 ) ) ;
#14685=FACE_OUTER_BOUND ( 'NONE', #26789, .T. ) ;
#14693=CARTESIAN_POINT ( 'NONE',  ( 20.08195036849999937, 1474.154268156089984, 211.0972226708090034 ) ) ;
#14695=VERTEX_POINT ( 'NONE', #108616 ) ;
#14700=CARTESIAN_POINT ( 'NONE',  ( 2.958097658348910031, 1515.068899390480283, 213.4512612428040086 ) ) ;
#14702=CARTESIAN_POINT ( 'NONE',  ( -3.829620113550000315, 1515.551704408389924, 211.4519800877889963 ) ) ;
#14703=ORIENTED_EDGE ( 'NONE', *, *, #9048, .T. ) ;
#14709=CARTESIAN_POINT ( 'NONE',  ( -5.209734426898009474, 1441.765094112799943, 201.7747637104849900 ) ) ;
#14712=CARTESIAN_POINT ( 'NONE',  ( -8.630935213989998189, 1438.255193345089992, 208.1083423884190040 ) ) ;
#14725=CARTESIAN_POINT ( 'NONE',  ( -9.954727031183750796, 1446.941805363540198, 211.8349694523599851 ) ) ;
#14727=B_SPLINE_CURVE_WITH_KNOTS ( 'NONE', 3,
 ( #47906, #98298, #21574, #3726, #72567, #97196, #13721, #37856, #63635, #106159, #97749, #21020, #55224, #89354 ),
 .UNSPECIFIED., .F., .F.,
 ( 4, 2, 2, 2, 2, 2, 4 ),
 ( 0.000000000000000000, 0.2499999999999116262, 0.4999999999998232525, 0.6249999999997172262, 0.6874999999997223332, 0.7499999999997273292, 1.000000000000000000 ),
 .UNSPECIFIED. ) ;
#14729=EDGE_CURVE ( 'NONE', #43735, #37608, #43630, .T. ) ;
#14739=CARTESIAN_POINT ( 'NONE',  ( 9.699838620905369524, 1453.359120950689885, 212.1672243862410028 ) ) ;
#14750=CARTESIAN_POINT ( 'NONE',  ( 12.91792090909249779, 1421.070795045020077, 203.9889279772430086 ) ) ;
#14752=ORIENTED_EDGE ( 'NONE', *, *, #40626, .T. ) ;
#14754=CARTESIAN_POINT ( 'NONE',  ( -13.59241398700699932, 1508.144654051440057, 209.5353803071969878 ) ) ;
#14762=CARTESIAN_POINT ( 'NONE',  ( 8.034189947220001571, 1427.422895264749968, 212.2991858979890196 ) ) ;
#14764=B_SPLINE_CURVE_WITH_KNOTS ( 'NONE', 3,
 ( #89643, #72322, #47654, #107548, #46022, #81782, #12929, #37598, #5084, #22406, #90743, #11849, #71800, #63388, #75621, #92946, #67768, #50421, #25172, #85089, #7295, #91298, #33576, #6733, #100254, #99678, #66132, #14580 ),
 .UNSPECIFIED., .F., .F.,
 ( 4, 3, 3, 3, 3, 3, 3, 3, 3, 4 ),
 ( -25.30278714349060110, -25.16708866733689831, -24.99913445276009938, -24.69548176202949819, -24.08817638056840238, -23.17766623311220187, -22.54008017006870190, -21.79135080256759949, -20.68911956487800197, -19.77745725219000050 ),
 .UNSPECIFIED. ) ;
#14766=CARTESIAN_POINT ( 'NONE',  ( -16.43468781389340094, 1420.643514338609975, 203.2794736519120136 ) ) ;
#14772=EDGE_LOOP ( 'NONE', ( #82970, #26827, #50053, #49143 ) ) ;
#14785=CARTESIAN_POINT ( 'NONE',  ( 2.548339227810000107, 1419.358184697269962, 204.5809049373789890 ) ) ;
#14794=EDGE_LOOP ( 'NONE', ( #23752, #91040, #51857, #109550 ) ) ;
#14795=CARTESIAN_POINT ( 'NONE',  ( -12.99775963039999915, 1420.302662752830201, 196.1023006302990268 ) ) ;
#14801=CARTESIAN_POINT ( 'NONE',  ( -13.19474177440000062, 1503.345007237690197, 208.6791437603130248 ) ) ;
#14802=DIRECTION ( 'NONE',  ( -0.8907681516580507886, 0.000000000000000000, 0.4544580288560209347 ) ) ;
#14808=CARTESIAN_POINT ( 'NONE',  ( -7.587902012781059469, 1453.124660370870060, 203.6743039436619824 ) ) ;
#14821=CARTESIAN_POINT ( 'NONE',  ( 2.792478474500000196, 1441.472946933690082, 218.6424847214589988 ) ) ;
#14834=CARTESIAN_POINT ( 'NONE',  ( 11.55388455309999962, 1425.897125911080138, 204.0276920965590080 ) ) ;
#14841=ORIENTED_EDGE ( 'NONE', *, *, #2290, .T. ) ;
#14847=CARTESIAN_POINT ( 'NONE',  ( 8.377797352699728251, 1424.395980914158827, 195.8294568783052512 ) ) ;
#14848=CARTESIAN_POINT ( 'NONE',  ( -0.5525556504920010603, 1444.336369769489920, 218.0684148105289921 ) ) ;
#14859=DIRECTION ( 'NONE',  ( -0.9404331407594663794, 0.3018495643663520744, -0.1564364032222970435 ) ) ;
#14865=CARTESIAN_POINT ( 'NONE',  ( -8.640340473127709586, 1437.525024229920064, 208.5374257294450047 ) ) ;
#14866=CARTESIAN_POINT ( 'NONE',  ( -4.325403553351909736, 1515.219291385429869, 211.4517448057640081 ) ) ;
#14868=CARTESIAN_POINT ( 'NONE',  ( -14.73949824312500034, 1415.677402202700023, 206.3522687176919987 ) ) ;
#14878=ORIENTED_EDGE ( 'NONE', *, *, #107689, .F. ) ;
#14879=CARTESIAN_POINT ( 'NONE',  ( -12.33110954549999860, 1502.406660704589740, 209.5022816524030134 ) ) ;
#14881=CARTESIAN_POINT ( 'NONE',  ( 4.669122900610000571, 1455.239293656489963, 217.7735903674689837 ) ) ;
#14883=CARTESIAN_POINT ( 'NONE',  ( -8.532458278280000030, 1445.788163739789979, 215.0754535007789912 ) ) ;
#14885=CARTESIAN_POINT ( 'NONE',  ( -4.487249775048080203, 1509.038615934839981, 211.6097811040130239 ) ) ;
#14897=CARTESIAN_POINT ( 'NONE',  ( -18.92739547204800132, 1503.346040100430173, 222.1981696246060096 ) ) ;
#14899=CARTESIAN_POINT ( 'NONE',  ( -3.282353412611801691, 1474.704843300428365, 218.8718926834540639 ) ) ;
#14906=CARTESIAN_POINT ( 'NONE',  ( -4.708696172490000720, 1457.421299317690000, 217.4082516364489948 ) ) ;
#14911=VERTEX_POINT ( 'NONE', #48035 ) ;
#14912=EDGE_LOOP ( 'NONE', ( #51320, #25244, #92057, #41977 ) ) ;
#14917=CARTESIAN_POINT ( 'NONE',  ( -17.62549087743260046, 1419.742512564495883, 206.8807750381302242 ) ) ;
#14926=CARTESIAN_POINT ( 'NONE',  ( -1.800870875340000010, 1483.727879433689850, 201.4520989251889773 ) ) ;
#14934=CARTESIAN_POINT ( 'NONE',  ( 10.84031051884389818, 1460.610437092660050, 207.7000986127219733 ) ) ;
#14940=CARTESIAN_POINT ( 'NONE',  ( 5.025113536143859250, 1441.506992453729936, 216.4625214299290121 ) ) ;
#14945=CARTESIAN_POINT ( 'NONE',  ( -9.966716235978671179, 1439.480426183019972, 208.4307555467810005 ) ) ;
#14949=B_SPLINE_CURVE_WITH_KNOTS ( 'NONE', 3,
 ( #33916, #26619, #103886, #36143, #50728, #51845, #85982, #42888, #1432, #26050, #18210, #60244, #95489, #27187, #35576, #94362, #86531, #52406, #16537, #59154, #17643, #68111, #9281, #102224, #52953, #103311, #77592, #87088, #898, #93274, #2008, #84860, #35023, #8710, #9825, #93806, #10372 ),
 .UNSPECIFIED., .F., .F.,
 ( 4, 3, 3, 3, 3, 3, 3, 3, 3, 3, 3, 3, 4 ),
 ( -12.95412176402940041, -12.81270172653739969, -12.11377028864190031, -11.37640253426160086, -10.60196073214190093, -9.777136418881470448, -8.810301696189478449, -7.829449850869419691, -7.084615941809260242, -6.173206107712330137, -5.351908026777899785, -4.634020098607701144, -3.959746331690000787 ),
 .UNSPECIFIED. ) ;
#14950=B_SPLINE_SURFACE_WITH_KNOTS ( 'NONE', 5, 5, ( 
 ( #38157, #72338, #29752, #47124, #82370, #4566 ),
 ( #47671, #26303, #33054, #68351, #42569, #101898 ),
 ( #8398, #50439, #7855, #34165, #75087, #51524 ),
 ( #93505, #109237, #25191, #15675, #43131, #42024 ),
 ( #85659, #8959, #67788, #34714, #75638, #76721 ),
 ( #24628, #49879, #60494, #59394, #40907, #16777 ),
 ( #110320, #7313, #33, #50981, #94614, #49328 ),
 ( #77289, #68905, #102457, #85110, #67243, #25744 ),
 ( #100800, #92962, #16235, #76171, #587, #103006 ) ),
 .UNSPECIFIED., .F., .F., .F.,
 ( 6, 3, 6 ),
 ( 6, 6 ),
 ( 13.33598741418959932, 23.39129113199999921, 32.68035051645690459 ),
 ( -0.0006151925569443899948, 2.000000000000000000 ),
 .UNSPECIFIED. ) ;
#14952=CARTESIAN_POINT ( 'NONE',  ( -4.001284449659999964, 1413.820567198780054, 207.0461413201589949 ) ) ;
#14955=CARTESIAN_POINT ( 'NONE',  ( 5.393840585100000418, 1486.194748859389847, 199.7804271763089901 ) ) ;
#14964=B_SPLINE_SURFACE_WITH_KNOTS ( 'NONE', 3, 3, ( 
 ( #18278, #43512, #60312, #59220 ),
 ( #35094, #87159, #25018, #27251 ),
 ( #51343, #52471, #44062, #94431 ),
 ( #85477, #8776, #9892, #35645 ) ),
 .UNSPECIFIED., .F., .F., .F.,
 ( 4, 4 ),
 ( 4, 4 ),
 ( 0.000000000000000000, 13.62591263460000057 ),
 ( 7.105427357600000794E-15, 6.790838053299999899 ),
 .UNSPECIFIED. ) ;
#14966=CARTESIAN_POINT ( 'NONE',  ( -16.34938676670969926, 1508.551704408389924, 213.4150739050749905 ) ) ;
#14967=CARTESIAN_POINT ( 'NONE',  ( -14.87836745164769958, 1508.449846342590035, 215.6161849205319925 ) ) ;
#14968=CARTESIAN_POINT ( 'NONE',  ( -2.562742973329999785, 1475.717683561390004, 219.5239615403990001 ) ) ;
#14969=CARTESIAN_POINT ( 'NONE',  ( -21.08979015450000105, 1504.838394598090190, 213.3139657128890008 ) ) ;
#14974=CARTESIAN_POINT ( 'NONE',  ( -3.829619994797929916, 1515.551704292389786, 210.9648097401420159 ) ) ;
#14976=CARTESIAN_POINT ( 'NONE',  ( -10.21402431085859952, 1471.431448933499951, 210.3618840756950021 ) ) ;
#14977=CARTESIAN_POINT ( 'NONE',  ( 4.327741874859650117, 1515.129976808880201, 208.3983552552599861 ) ) ;
#14982=CARTESIAN_POINT ( 'NONE',  ( 10.55618159092670005, 1481.139606696229976, 209.6439938450050136 ) ) ;
#14985=CARTESIAN_POINT ( 'NONE',  ( 11.67995417459249907, 1501.899375693250022, 211.4228182329390222 ) ) ;
#14987=CARTESIAN_POINT ( 'NONE',  ( 9.467588392827540389, 1422.608842469059937, 212.7560699654940208 ) ) ;
#14988=CARTESIAN_POINT ( 'NONE',  ( -1.850909961131140147, 1508.551704408389924, 220.0758087861170225 ) ) ;
#14992=CARTESIAN_POINT ( 'NONE',  ( -11.65438896117129808, 1501.787989776810036, 208.8020054899499769 ) ) ;
#14993=CARTESIAN_POINT ( 'NONE',  ( 11.74550440620560110, 1492.414915879079899, 211.0460056930020016 ) ) ;
#14994=CARTESIAN_POINT ( 'NONE',  ( -0.9377529295590010250, 1456.788838343890120, 218.9786281422690024 ) ) ;
#14998=CARTESIAN_POINT ( 'NONE',  ( 8.174873262491109571, 1436.356241397249960, 206.4284659498850090 ) ) ;
#15003=CARTESIAN_POINT ( 'NONE',  ( -11.87328627558470018, 1482.014094172719979, 208.6022272904490080 ) ) ;
#15006=CARTESIAN_POINT ( 'NONE',  ( -8.107801870790000365, 1463.844143246390104, 201.5100198155989801 ) ) ;
#15013=CARTESIAN_POINT ( 'NONE',  ( 2.180749907540250110, 1433.190219894490156, 200.8861995550460051 ) ) ;
#15017=VERTEX_POINT ( 'NONE', #22794 ) ;
#15022=CARTESIAN_POINT ( 'NONE',  ( 12.40160258794860049, 1420.584110727309962, 200.5244627772079866 ) ) ;
#15023=CARTESIAN_POINT ( 'NONE',  ( 6.824596843277944913, 1424.786834349993342, 213.4892281956427098 ) ) ;
#15024=CARTESIAN_POINT ( 'NONE',  ( -14.65275159090000123, 1420.238444720549978, 213.8660283808390261 ) ) ;
#15036=CARTESIAN_POINT ( 'NONE',  ( 7.408918475326540687, 1425.143336949030072, 212.4352455266580080 ) ) ;
#15044=CARTESIAN_POINT ( 'NONE',  ( -1.534154776998204239, 1488.212794018828845, 219.8849755564752115 ) ) ;
#15049=VERTEX_POINT ( 'NONE', #1364 ) ;
#15053=CARTESIAN_POINT ( 'NONE',  ( 9.744365386780000193, 1462.929680191989974, 209.8474545865749974 ) ) ;
#15058=ORIENTED_EDGE ( 'NONE', *, *, #88299, .T. ) ;
#15062=CARTESIAN_POINT ( 'NONE',  ( 4.987082593000310204, 1508.551704408389924, 212.3948883545009778 ) ) ;
#15070=CARTESIAN_POINT ( 'NONE',  ( 6.683036765369180010, 1483.419246594629840, 218.8825796861059985 ) ) ;
#15071=EDGE_CURVE ( 'NONE', #59860, #60953, #31434, .T. ) ;
#15073=CARTESIAN_POINT ( 'NONE',  ( 6.154344797466830386, 1434.513861532099781, 226.5897845999569995 ) ) ;
#15075=CARTESIAN_POINT ( 'NONE',  ( -11.22704429269360027, 1481.056718734030028, 211.0225828912199972 ) ) ;
#15077=CARTESIAN_POINT ( 'NONE',  ( 5.681834224037626058, 1434.688408934563313, 202.7553282809922166 ) ) ;
#15081=CARTESIAN_POINT ( 'NONE',  ( 8.247379814629999473, 1421.181889050119935, 196.1087402428989890 ) ) ;
#15083=CARTESIAN_POINT ( 'NONE',  ( -11.90229160620850024, 1491.340589200470049, 206.1196870462119932 ) ) ;
#15084=FACE_OUTER_BOUND ( 'NONE', #74086, .T. ) ;
#15097=B_SPLINE_SURFACE_WITH_KNOTS ( 'NONE', 5, 5, ( 
 ( #16087, #63393, #29204, #32369, #97508, #92266 ),
 ( #107000, #15536, #98597, #29741, #80711, #75494 ),
 ( #89648, #4557, #41324, #12934, #63929, #98043 ),
 ( #64482, #109628, #50294, #32899, #101197, #24493 ),
 ( #41866, #76018, #20777, #54978, #89103, #86076 ),
 ( #10475, #59789, #44646, #8799, #110723, #9916 ) ),
 .UNSPECIFIED., .F., .F., .F.,
 ( 6, 6 ),
 ( 6, 6 ),
 ( 2.324858856890000158, 4.991117563610000474 ),
 ( 0.000000000000000000, 0.5000000000000000000 ),
 .UNSPECIFIED. ) ;
#15099=CARTESIAN_POINT ( 'NONE',  ( -15.91912926760000246, 1415.990061217859875, 209.7496671253580018 ) ) ;
#15100=EDGE_CURVE ( 'NONE', #62781, #39872, #96895, .T. ) ;
#15101=CARTESIAN_POINT ( 'NONE',  ( 11.66448423075249963, 1421.851407392159899, 203.4123043171020129 ) ) ;
#15107=B_SPLINE_SURFACE_WITH_KNOTS ( 'NONE', 5, 5, ( 
 ( #16824, #86268, #43181, #94669, #42619, #35880 ),
 ( #76771, #87, #103625, #102502, #77333, #68951 ),
 ( #52136, #26351, #43724, #61112, #77877, #104176 ),
 ( #1185, #18491, #95227, #69503, #52686, #10114 ),
 ( #70064, #106917, #47042, #88482, #98520, #21786 ),
 ( #44848, #30206, #70606, #96885, #20695, #2303 ) ),
 .UNSPECIFIED., .F., .F., .F.,
 ( 6, 6 ),
 ( 6, 6 ),
 ( 3.171299407250000257, 3.535033821230000317 ),
 ( 0.000000000000000000, 0.2999999999999999889 ),
 .UNSPECIFIED. ) ;
#15108=PLANE ( 'NONE',  #38367 ) ;
#15118=CARTESIAN_POINT ( 'NONE',  ( -3.156438986539999991, 1479.750519982490005, 229.2993030149989977 ) ) ;
#15120=CARTESIAN_POINT ( 'NONE',  ( 1.117126662530000036, 1515.456827602489966, 204.9211030669989952 ) ) ;
#15127=EDGE_LOOP ( 'NONE', ( #74852, #214, #55923, #40549 ) ) ;
#15134=CARTESIAN_POINT ( 'NONE',  ( 11.26937487549999872, 1478.652699893289991, 205.8601903476990174 ) ) ;
#15137=CARTESIAN_POINT ( 'NONE',  ( -1.743457682199999859, 1468.969847108790191, 189.2470145170989895 ) ) ;
#15140=CARTESIAN_POINT ( 'NONE',  ( -15.07756690969999980, 1414.162796065500061, 212.4126893105689931 ) ) ;
#15142=CARTESIAN_POINT ( 'NONE',  ( 4.138543392800865917, 1515.492058412107781, 210.9648081769078374 ) ) ;
#15145=CARTESIAN_POINT ( 'NONE',  ( 10.65988927221830096, 1426.698688119150120, 208.4127383140620111 ) ) ;
#15149=CARTESIAN_POINT ( 'NONE',  ( 3.401541474470889614, 1468.225229937070026, 218.5224292273400124 ) ) ;
#15152=CARTESIAN_POINT ( 'NONE',  ( 11.37306528310140052, 1471.269141200139984, 210.1781679118379884 ) ) ;
#15160=CARTESIAN_POINT ( 'NONE',  ( 10.10679549600000193, 1451.115179940190046, 206.1347980303889926 ) ) ;
#15163=VECTOR ( 'NONE', #21243, 1000.000000000000114 ) ;
#15165=EDGE_CURVE ( 'NONE', #44275, #35203, #4672, .T. ) ;
#15171=DIRECTION ( 'NONE',  ( -7.436362843295819681E-17, 1.000000000000000000, -1.457576885956999882E-16 ) ) ;
#15176=ORIENTED_EDGE ( 'NONE', *, *, #60710, .F. ) ;
#15177=CARTESIAN_POINT ( 'NONE',  ( 1.673908112249919977, 1485.355439722810161, 220.8689413507970016 ) ) ;
#15178=CARTESIAN_POINT ( 'NONE',  ( 11.27569180979999963, 1501.931370426789954, 206.9838411614990150 ) ) ;
#15187=CARTESIAN_POINT ( 'NONE',  ( 12.66766512233539821, 1500.805898962940091, 210.1506732187789908 ) ) ;
#15193=ORIENTED_EDGE ( 'NONE', *, *, #24163, .T. ) ;
#15215=ORIENTED_EDGE ( 'NONE', *, *, #78076, .T. ) ;
#15222=CARTESIAN_POINT ( 'NONE',  ( -16.76078030769999927, 1420.494757909599912, 203.1294657649889928 ) ) ;
#15227=CARTESIAN_POINT ( 'NONE',  ( 7.778981777592010260, 1467.988552340439810, 201.0890001560949827 ) ) ;
#15231=ORIENTED_EDGE ( 'NONE', *, *, #106125, .F. ) ;
#15234=CARTESIAN_POINT ( 'NONE',  ( -4.863842518140000237, 1453.445020719190097, 199.8398594391789800 ) ) ;
#15238=CARTESIAN_POINT ( 'NONE',  ( 2.801044513573409667, 1515.551704203360032, 212.9510687777460021 ) ) ;
#15248=CARTESIAN_POINT ( 'NONE',  ( -4.453607449379680006, 1428.081049923210003, 200.8976384725820026 ) ) ;
#15249=ADVANCED_FACE ( 'NONE', ( #44909 ), #106115, .T. ) ;
#15250=CARTESIAN_POINT ( 'NONE',  ( -15.22591321480220117, 1441.486322144610085, 221.1269846435299939 ) ) ;
#15252=CARTESIAN_POINT ( 'NONE',  ( -10.56985333086790035, 1482.340625775369972, 205.9074429510509958 ) ) ;
#15253=CARTESIAN_POINT ( 'NONE',  ( -4.794426340529999386, 1463.608615258990085, 228.2108236244990280 ) ) ;
#15265=CARTESIAN_POINT ( 'NONE',  ( -15.31513450300000123, 1417.997849063050126, 203.5151318327289971 ) ) ;
#15268=B_SPLINE_SURFACE_WITH_KNOTS ( 'NONE', 5, 5, ( 
 ( #63671, #45767, #96704, #89395, #13211, #73149 ),
 ( #105096, #54718, #30021, #72603, #107292, #37898 ),
 ( #97783, #54169, #72080, #90485, #106732, #39543 ),
 ( #64214, #106194, #28386, #98336, #55817, #47401 ),
 ( #13760, #3215, #38970, #64775, #98885, #47944 ),
 ( #62587, #19975, #37343, #71540, #105662, #28946 ) ),
 .UNSPECIFIED., .F., .F., .F.,
 ( 6, 6 ),
 ( 6, 6 ),
 ( 0.000000000000000000, 9.314731292829998566 ),
 ( 0.000000000000000000, 2.000000000000000000 ),
 .UNSPECIFIED. ) ;
#15269=CARTESIAN_POINT ( 'NONE',  ( -8.619624426343268198, 1437.672210802470090, 208.2420778849330247 ) ) ;
#15271=CARTESIAN_POINT ( 'NONE',  ( -5.498087649510000396, 1437.444228038389838, 208.8531670801410201 ) ) ;
#15280=CARTESIAN_POINT ( 'NONE',  ( -21.59687142900000012, 1507.523380033690046, 209.4572543540780032 ) ) ;
#15288=B_SPLINE_CURVE_WITH_KNOTS ( 'NONE', 5,
 ( #103927, #42363, #36182, #42931, #19353, #78170 ),
 .UNSPECIFIED., .F., .F.,
 ( 6, 6 ),
 ( 0.000000000000000000, 1.000000000000000000 ),
 .UNSPECIFIED. ) ;
#15292=CARTESIAN_POINT ( 'NONE',  ( -8.268898679290179743, 1439.252518696380093, 228.5874792367960140 ) ) ;
#15293=CARTESIAN_POINT ( 'NONE',  ( 11.45577226660000036, 1502.286415424589904, 208.3140783707030153 ) ) ;
#15295=CARTESIAN_POINT ( 'NONE',  ( -3.071486888918079750, 1470.850328545360071, 187.3986291775349855 ) ) ;
#15300=CARTESIAN_POINT ( 'NONE',  ( -5.582992786199999280, 1454.196299517489933, 201.5533260997290199 ) ) ;
#15303=CARTESIAN_POINT ( 'NONE',  ( -20.02799630220000182, 1485.574563381989947, 204.1280247810589970 ) ) ;
#15306=CARTESIAN_POINT ( 'NONE',  ( -17.47119686262369953, 1420.005972689359851, 204.6300621421460164 ) ) ;
#15319=CARTESIAN_POINT ( 'NONE',  ( -0.02721485961659890138, 1443.931464463489874, 200.0408948413389965 ) ) ;
#15321=EDGE_CURVE ( 'NONE', #79507, #20921, #84277, .T. ) ;
#15323=CARTESIAN_POINT ( 'NONE',  ( -3.127352221352849959, 1464.808845836910223, 198.5552573355170125 ) ) ;
#15324=CARTESIAN_POINT ( 'NONE',  ( 3.018932976099999443, 1424.181238483419975, 191.3872096091990045 ) ) ;
#15331=EDGE_CURVE ( 'NONE', #26097, #93900, #108779, .T. ) ;
#15332=ORIENTED_EDGE ( 'NONE', *, *, #21681, .F. ) ;
#15333=ORIENTED_EDGE ( 'NONE', *, *, #105493, .T. ) ;
#15338=CARTESIAN_POINT ( 'NONE',  ( -19.78960455480000036, 1467.443448038389988, 207.1734148488289975 ) ) ;
#15340=CARTESIAN_POINT ( 'NONE',  ( -11.61154441450000085, 1502.159899280790114, 208.3750068673870146 ) ) ;
#15348=CARTESIAN_POINT ( 'NONE',  ( -8.419044950492288848, 1452.206747589980068, 205.1691836855419808 ) ) ;
#15366=CARTESIAN_POINT ( 'NONE',  ( 16.84849232383349715, 1428.239404528469777, 202.3949443903100018 ) ) ;
#15371=CARTESIAN_POINT ( 'NONE',  ( -19.73295319860160291, 1503.904974312793911, 218.6992394349398126 ) ) ;
#15381=CARTESIAN_POINT ( 'NONE',  ( 5.170487778963170022, 1484.055109584380034, 219.7711518219039988 ) ) ;
#15395=CARTESIAN_POINT ( 'NONE',  ( -6.483871891156958611, 1462.197955881078769, 201.8355004268651953 ) ) ;
#15401=CARTESIAN_POINT ( 'NONE',  ( 10.79528402730720060, 1489.628194868570063, 207.4012257063180016 ) ) ;
#15404=CARTESIAN_POINT ( 'NONE',  ( 5.349014141963440494, 1506.777988995989972, 219.5093220728170138 ) ) ;
#15410=CARTESIAN_POINT ( 'NONE',  ( -5.219497435470000113, 1484.378742230190255, 199.3181751762190004 ) ) ;
#15413=CARTESIAN_POINT ( 'NONE',  ( -9.783890651532770377, 1438.409856597829958, 210.7792734677780118 ) ) ;
#15414=CARTESIAN_POINT ( 'NONE',  ( -3.778540308872590181, 1515.551842517600107, 212.4904177570749937 ) ) ;
#15424=ORIENTED_EDGE ( 'NONE', *, *, #25335, .T. ) ;
#15430=CARTESIAN_POINT ( 'NONE',  ( -4.716923275420001005, 1446.360134133290103, 217.0074177048290096 ) ) ;
#15434=CARTESIAN_POINT ( 'NONE',  ( 6.916306201240000284, 1423.889214271699984, 213.5479170703790146 ) ) ;
#15445=CARTESIAN_POINT ( 'NONE',  ( 24.10516660284129742, 1496.435767336129857, 206.8622324630100309 ) ) ;
#15476=CARTESIAN_POINT ( 'NONE',  ( -2.620823360909999789, 1483.467906750489874, 201.7239643817090098 ) ) ;
#15480=CARTESIAN_POINT ( 'NONE',  ( 5.745386292849999244, 1451.922981708390125, 211.2075068023790152 ) ) ;
#15487=EDGE_CURVE ( 'NONE', #12262, #58610, #102237, .T. ) ;
#15496=CARTESIAN_POINT ( 'NONE',  ( 19.87935007599999793, 1476.501528767390027, 213.0784012132189957 ) ) ;
#15501=CARTESIAN_POINT ( 'NONE',  ( 10.57339846829999885, 1490.054618766489966, 202.8450963736189863 ) ) ;
#15506=CARTESIAN_POINT ( 'NONE',  ( 18.30025784240000064, 1431.961054190390087, 210.0255047360110154 ) ) ;
#15508=VERTEX_POINT ( 'NONE', #79999 ) ;
#15511=CARTESIAN_POINT ( 'NONE',  ( -16.57637045210000082, 1420.575130030530090, 203.2586717730690111 ) ) ;
#15517=CARTESIAN_POINT ( 'NONE',  ( -11.32617949625089970, 1471.108170639839955, 207.7151593947669994 ) ) ;
#15524=CARTESIAN_POINT ( 'NONE',  ( -11.36188915788260090, 1470.553325319990108, 210.0693210479820152 ) ) ;
#15525=CARTESIAN_POINT ( 'NONE',  ( 4.328142686769970382, 1515.114670419599861, 208.1949246329089931 ) ) ;
#15532=CARTESIAN_POINT ( 'NONE',  ( 11.35657976162540095, 1502.829282324059932, 211.1038090253330211 ) ) ;
#15533=CARTESIAN_POINT ( 'NONE',  ( 1847.405368200919384, -8387.357407334282470, 1585.835250321477815 ) ) ;
#15536=CARTESIAN_POINT ( 'NONE',  ( -4.325805487360000257, 1515.203924463989779, 207.6586276196590006 ) ) ;
#15539=CARTESIAN_POINT ( 'NONE',  ( 4.550353367526756898, 1466.224087956547919, 218.4072860836689927 ) ) ;
#15540=FACE_OUTER_BOUND ( 'NONE', #70237, .T. ) ;
#15541=CARTESIAN_POINT ( 'NONE',  ( -2.137491047500000185, 1455.891788169089978, 218.3487140958189912 ) ) ;
#15548=CARTESIAN_POINT ( 'NONE',  ( -8.210973799569998732, 1501.032796100090081, 209.1036754092109788 ) ) ;
#15552=CARTESIAN_POINT ( 'NONE',  ( -8.494781050700002112, 1461.600995454589793, 204.2538046751789977 ) ) ;
#15556=CARTESIAN_POINT ( 'NONE',  ( -8.229900059930191247, 1508.551704408389924, 218.8850718935309771 ) ) ;
#15560=CARTESIAN_POINT ( 'NONE',  ( 4.082546718995279988, 1433.473438342260124, 201.5982916962979914 ) ) ;
#15564=EDGE_LOOP ( 'NONE', ( #44976, #64853, #58273, #63332 ) ) ;
#15568=CARTESIAN_POINT ( 'NONE',  ( 1.842963721827329815, 1515.551704300040001, 212.9514659606769840 ) ) ;
#15569=CARTESIAN_POINT ( 'NONE',  ( -2.657845259230000146, 1476.012816621789852, 198.9905392320989961 ) ) ;
#15574=CARTESIAN_POINT ( 'NONE',  ( 1.197195770085190070, 1429.524192212559910, 217.3433698247590087 ) ) ;
#15575=CARTESIAN_POINT ( 'NONE',  ( -8.255467494119999472, 1424.664513863459888, 207.0640964688590202 ) ) ;
#15580=CARTESIAN_POINT ( 'NONE',  ( 7.445112198176509821, 1425.205606764170170, 212.3599477002399851 ) ) ;
#15590=CARTESIAN_POINT ( 'NONE',  ( 5.615127104817687176, 1507.508085020990166, 219.4002671829225619 ) ) ;
#15597=ORIENTED_EDGE ( 'NONE', *, *, #44069, .F. ) ;
#15615=CARTESIAN_POINT ( 'NONE',  ( 2.898715468759999858, 1428.109906398889962, 213.6762267714089774 ) ) ;
#15617=CARTESIAN_POINT ( 'NONE',  ( -10.41425093117460143, 1479.497781561380179, 210.3960398642789755 ) ) ;
#15621=CARTESIAN_POINT ( 'NONE',  ( 11.18883130367080092, 1502.419542440489977, 215.1996028960269882 ) ) ;
#15622=CARTESIAN_POINT ( 'NONE',  ( 7.634170062339999063, 1421.957731401030060, 195.7691812542990135 ) ) ;
#15623=CARTESIAN_POINT ( 'NONE',  ( -2.295483817934420134, 1432.805523517590018, 218.3736922701850176 ) ) ;
#15624=CARTESIAN_POINT ( 'NONE',  ( 10.93777210243689879, 1478.839323300969909, 205.9316688570750102 ) ) ;
#15637=CARTESIAN_POINT ( 'NONE',  ( 9.217393380133168890, 1426.476016588670063, 210.2456940754379957 ) ) ;
#15638=CARTESIAN_POINT ( 'NONE',  ( 12.34756956475129996, 1421.260964715650061, 203.4353636828009826 ) ) ;
#15639=CARTESIAN_POINT ( 'NONE',  ( -10.93951897979770038, 1462.702982771529832, 207.5546680835130076 ) ) ;
#15647=CARTESIAN_POINT ( 'NONE',  ( 5.253642672657390378, 1466.463266540510176, 217.7249926852120154 ) ) ;
#15649=CARTESIAN_POINT ( 'NONE',  ( 4.606382372549210125, 1474.138419553830090, 219.5757164701410034 ) ) ;
#15653=CARTESIAN_POINT ( 'NONE',  ( 1.433806162063078204, 1478.005084112435952, 198.7945331361510171 ) ) ;
#15654=DIRECTION ( 'NONE',  ( -1.761221539070279927E-08, 1.000000000000000000, 5.441036071155500311E-09 ) ) ;
#15658=FACE_OUTER_BOUND ( 'NONE', #107184, .T. ) ;
#15660=CARTESIAN_POINT ( 'NONE',  ( -15.18482336544590083, 1421.253453350580003, 203.4821423529160143 ) ) ;
#15662=CARTESIAN_POINT ( 'NONE',  ( 6.486349823423054772, 1465.915338427141933, 201.5941921811669886 ) ) ;
#15668=CARTESIAN_POINT ( 'NONE',  ( -20.11385680769999951, 1487.601373209189887, 204.1067431612489997 ) ) ;
#15675=CARTESIAN_POINT ( 'NONE',  ( -8.055949302434040504, 1436.374732820499958, 213.3353392178869967 ) ) ;
#15679=CARTESIAN_POINT ( 'NONE',  ( 4.261736552472805251, 1515.372048948338943, 210.9648081765028849 ) ) ;
#15682=CARTESIAN_POINT ( 'NONE',  ( 10.23375359582179911, 1424.446042691910179, 207.3832406123669898 ) ) ;
#15688=CARTESIAN_POINT ( 'NONE',  ( 5.013709187000000789, 1473.458530729089944, 218.4934638050989975 ) ) ;
#15698=CARTESIAN_POINT ( 'NONE',  ( 6.500020221522261110, 1497.924676537463711, 198.3229680000449662 ) ) ;
#15699=CARTESIAN_POINT ( 'NONE',  ( 8.286340681629999594, 1448.851909210790154, 205.0448464285690306 ) ) ;
#15703=CARTESIAN_POINT ( 'NONE',  ( -9.173749095941850840, 1450.559996438570124, 208.1432995907519796 ) ) ;
#15705=VECTOR ( 'NONE', #14859, 1000.000000000000114 ) ;
#15707=VERTEX_POINT ( 'NONE', #79878 ) ;
#15708=CARTESIAN_POINT ( 'NONE',  ( 3.152929577590128929, 1465.382732736859225, 199.7633066961682857 ) ) ;
#15712=CARTESIAN_POINT ( 'NONE',  ( -17.50517576071650083, 1417.698423450930022, 206.6604295572749947 ) ) ;
#15716=CARTESIAN_POINT ( 'NONE',  ( 11.45577226660000036, 1502.286415424589904, 208.3140783707030153 ) ) ;
#15727=CARTESIAN_POINT ( 'NONE',  ( -13.05162051250000133, 1467.538720777590015, 191.8992815354989716 ) ) ;
#15730=ORIENTED_EDGE ( 'NONE', *, *, #76199, .T. ) ;
#15731=CARTESIAN_POINT ( 'NONE',  ( -2.218918655950000041, 1431.115532604589816, 203.8893403826889994 ) ) ;
#15732=CARTESIAN_POINT ( 'NONE',  ( 10.54758761917650034, 1452.770155221380037, 210.0494888551049826 ) ) ;
#15733=CARTESIAN_POINT ( 'NONE',  ( -5.106228707209799822, 1507.795005401549815, 220.9628779089179886 ) ) ;
#15735=CARTESIAN_POINT ( 'NONE',  ( -10.86173877940340127, 1417.961625830270577, 198.2022571467911405 ) ) ;
#15736=CARTESIAN_POINT ( 'NONE',  ( 2.626093229311771804, 1468.533706331386838, 218.7919682226666112 ) ) ;
#15740=PLANE ( 'NONE',  #37359 ) ;
#15753=CARTESIAN_POINT ( 'NONE',  ( -18.70861292059999670, 1442.610498708490013, 207.2775239616889849 ) ) ;
#15754=CARTESIAN_POINT ( 'NONE',  ( -10.04998969390729968, 1462.307699121839960, 207.4528283373930151 ) ) ;
#15756=CARTESIAN_POINT ( 'NONE',  ( 9.935891866850850462, 1468.906047781809775, 207.5492993768060046 ) ) ;
#15757=CARTESIAN_POINT ( 'NONE',  ( -9.915987190420000985, 1473.542783144990153, 206.4139885101390064 ) ) ;
#15758=CARTESIAN_POINT ( 'NONE',  ( 7.378495474280000188, 1492.475726123489949, 217.4190488244389883 ) ) ;
#15770=CARTESIAN_POINT ( 'NONE',  ( 3.582801916543969512, 1515.224507089990084, 213.1990874413949939 ) ) ;
#15777=CARTESIAN_POINT ( 'NONE',  ( -0.2109842154640010070, 1429.925335880790271, 214.7594818389389957 ) ) ;
#15778=CARTESIAN_POINT ( 'NONE',  ( -5.303217579353759703, 1442.879282873410148, 200.5942580338080177 ) ) ;
#15784=CARTESIAN_POINT ( 'NONE',  ( -10.77555132091760015, 1482.134168720230036, 206.6918653029249811 ) ) ;
#15788=AXIS2_PLACEMENT_3D ( 'NONE', #42323, #33912, #59150 ) ;
#15797=CARTESIAN_POINT ( 'NONE',  ( -15.48826635719999878, 1416.228753145889868, 207.4514652343489729 ) ) ;
#15800=CARTESIAN_POINT ( 'NONE',  ( -16.45418660414503975, 1419.665052300104435, 209.4254846085501072 ) ) ;
#15801=CARTESIAN_POINT ( 'NONE',  ( -3.685267454909999962, 1496.073671761789910, 219.7127564024990249 ) ) ;
#15804=CARTESIAN_POINT ( 'NONE',  ( 10.57423073640600109, 1481.617106639790109, 209.5624278184519937 ) ) ;
#15807=CARTESIAN_POINT ( 'NONE',  ( -5.489226980809999823, 1448.625211962289995, 211.5470588626189965 ) ) ;
#15810=EDGE_CURVE ( 'NONE', #328, #21613, #53029, .T. ) ;
#15816=CARTESIAN_POINT ( 'NONE',  ( 4.138993644310000164, 1515.551749209589843, 208.7474387692110156 ) ) ;
#15823=CARTESIAN_POINT ( 'NONE',  ( 10.17199984938910085, 1480.651875719519921, 206.3463171831010072 ) ) ;
#15824=EDGE_CURVE ( 'NONE', #63638, #45257, #63403, .T. ) ;
#15828=CARTESIAN_POINT ( 'NONE',  ( 4.770050319527739724, 1435.280277859259968, 228.7600612000269678 ) ) ;
#15830=CARTESIAN_POINT ( 'NONE',  ( 5.140110055453729565, 1436.845560459350054, 228.7442478949189990 ) ) ;
#15835=DIRECTION ( 'NONE',  ( 0.9996573249755517088, 0.02617694830808744988, 0.000000000000000000 ) ) ;
#15848=B_SPLINE_CURVE_WITH_KNOTS ( 'NONE', 3,
 ( #66518, #74904, #23905, #13299, #82735, #82175, #73804, #83283, #23368, #65959 ),
 .UNSPECIFIED., .F., .F.,
 ( 4, 3, 3, 4 ),
 ( -24.01273564469999755, -23.57996764826259906, -22.12139829086160248, -20.66572445029999727 ),
 .UNSPECIFIED. ) ;
#15856=CARTESIAN_POINT ( 'NONE',  ( -0.2549939780409989920, 1442.897942418790080, 200.2186398693189915 ) ) ;
#15863=FILL_AREA_STYLE ('',( #26493 ) ) ;
#15874=ORIENTED_EDGE ( 'NONE', *, *, #78050, .F. ) ;
#15879=CARTESIAN_POINT ( 'NONE',  ( -6.945821722360000727, 1473.074358042890026, 208.3699044046250037 ) ) ;
#15884=CARTESIAN_POINT ( 'NONE',  ( -11.93513138720000022, 1502.470134631589872, 208.6121448500909992 ) ) ;
#15891=VERTEX_POINT ( 'NONE', #83720 ) ;
#15908=CARTESIAN_POINT ( 'NONE',  ( 2.901791247649999850, 1441.419505434789926, 218.6084270491589905 ) ) ;
#15914=DIRECTION ( 'NONE',  ( -1.000000000000000000, 0.000000000000000000, 0.000000000000000000 ) ) ;
#15920=CARTESIAN_POINT ( 'NONE',  ( -2.443421232577144497, 1495.151577762832858, 220.0241338615849145 ) ) ;
#15921=CARTESIAN_POINT ( 'NONE',  ( 6.260663917511189780, 1483.739111220829955, 218.7790172297789866 ) ) ;
#15922=CARTESIAN_POINT ( 'NONE',  ( 11.82607906839999856, 1426.795487707440088, 206.5339109993589943 ) ) ;
#15923=CARTESIAN_POINT ( 'NONE',  ( -0.3488295727624319831, 1444.725433255539201, 218.0942056312121622 ) ) ;
#15927=CARTESIAN_POINT ( 'NONE',  ( -9.560134974813159658, 1448.417707445359838, 209.4104641123290094 ) ) ;
#15935=CARTESIAN_POINT ( 'NONE',  ( -8.959719548958744895, 1461.371917847066470, 205.3598266504384355 ) ) ;
#15936=CARTESIAN_POINT ( 'NONE',  ( 4.513979691470000333, 1467.746749492790059, 218.0203306744990357 ) ) ;
#15940=CIRCLE ( 'NONE', #107162, 0.4999999999999449329 ) ;
#15947=CARTESIAN_POINT ( 'NONE',  ( 4.792731738917410667, 1506.992693111409835, 219.7839786367459851 ) ) ;
#15949=ORIENTED_EDGE ( 'NONE', *, *, #56328, .F. ) ;
#15958=CARTESIAN_POINT ( 'NONE',  ( -4.261662193653090291, 1515.372228416479857, 211.4517523182709908 ) ) ;
#15981=CARTESIAN_POINT ( 'NONE',  ( 7.486774210370000127, 1423.123604678139827, 213.9129862981389749 ) ) ;
#15989=VERTEX_POINT ( 'NONE', #20365 ) ;
#15992=CARTESIAN_POINT ( 'NONE',  ( -21.56347740270249957, 1506.734670034049941, 209.3230842351990191 ) ) ;
#16002=CARTESIAN_POINT ( 'NONE',  ( -9.559179497712129603, 1447.160234701620084, 211.6757039224950177 ) ) ;
#16007=ADVANCED_FACE ( 'NONE', ( #90740 ), #77419, .T. ) ;
#16012=ADVANCED_FACE ( 'NONE', ( #57173 ), #20251, .T. ) ;
#16014=( NAMED_UNIT ( * ) PLANE_ANGLE_UNIT ( ) SI_UNIT ( $, .RADIAN. ) );
#16016=B_SPLINE_SURFACE_WITH_KNOTS ( 'NONE', 5, 5, ( 
 ( #69425, #41993, #101306, #110831, #103538, #16204 ),
 ( #76688, #43098, #60462, #77801, #102429, #50951 ),
 ( #58249, #51493, #17298, #92372, #76142, #75610 ),
 ( #109740, #49850, #85624, #77259, #83982, #558 ),
 ( #7281, #41445, #92933, #101868, #25160, #93474 ),
 ( #2225, #62693, #78919, #46426, #88944, #53163 ),
 ( #54819, #79461, #28498, #87305, #37451, #88403 ),
 ( #27388, #97346, #71651, #104097, #95151, #36339 ),
 ( #105770, #20617, #18968, #2772, #3874, #11162 ) ),
 .UNSPECIFIED., .F., .F., .F.,
 ( 6, 3, 6 ),
 ( 6, 6 ),
 ( 2.990692062960830011, 5.133895727739999693, 7.277090745855540277 ),
 ( -0.0004094007421257130183, 2.000000000000000000 ),
 .UNSPECIFIED. ) ;
#16019=( BOUNDED_CURVE ( )  B_SPLINE_CURVE ( 3, ( #103112, #95833, #77932, #94727 ),
 .UNSPECIFIED., .F., .F. ) 
 B_SPLINE_CURVE_WITH_KNOTS ( ( 4, 4 ),
 ( 1.800053338152554971, 2.115542295163019837 ),
 .UNSPECIFIED. ) 
 CURVE ( )  GEOMETRIC_REPRESENTATION_ITEM ( )  RATIONAL_B_SPLINE_CURVE ( ( 1.000000000000000000, 0.9917227450084913354, 0.9917227450084913354, 1.000000000000000000 ) ) 
 REPRESENTATION_ITEM ( '' )  );
#16021=AXIS2_PLACEMENT_3D ( 'NONE', #29353, #73029, #13087 ) ;
#16026=CARTESIAN_POINT ( 'NONE',  ( 11.13973214860000027, 1470.272411968090182, 206.9146623037889867 ) ) ;
#16027=AXIS2_PLACEMENT_3D ( 'NONE', #24105, #6766, #5120 ) ;
#16043=ORIENTED_EDGE ( 'NONE', *, *, #78924, .T. ) ;
#16045=CARTESIAN_POINT ( 'NONE',  ( -10.07108938579999879, 1472.689539964090045, 207.5339997831590040 ) ) ;
#16051=CARTESIAN_POINT ( 'NONE',  ( -17.60447252379999838, 1417.354189540510106, 207.6029927142990061 ) ) ;
#16053=CARTESIAN_POINT ( 'NONE',  ( 4.414384251610000476, 1487.467097172089780, 197.9737507085990273 ) ) ;
#16054=CARTESIAN_POINT ( 'NONE',  ( 1.729065141746580103, 1431.231418718420173, 218.4534901915430112 ) ) ;
#16063=CARTESIAN_POINT ( 'NONE',  ( -16.98381430819999949, 1420.348059816200021, 203.5840860547189948 ) ) ;
#16065=CARTESIAN_POINT ( 'NONE',  ( -2.155783482819999985, 1476.003253452089893, 220.3848946179990094 ) ) ;
#16068=CARTESIAN_POINT ( 'NONE',  ( -11.37853563926020151, 1470.969474876900222, 208.2620529163870060 ) ) ;
#16069=CARTESIAN_POINT ( 'NONE',  ( -4.336924793510721798, 1508.178691706793870, 220.5928148824004040 ) ) ;
#16075=CARTESIAN_POINT ( 'NONE',  ( -2.022195510094900506, 1421.024483011140092, 193.8502759697570070 ) ) ;
#16076=CARTESIAN_POINT ( 'NONE',  ( 4.328570061217780207, 1515.098349647940040, 207.9863157841529926 ) ) ;
#16083=CARTESIAN_POINT ( 'NONE',  ( 7.835586116740000051, 1423.724600923389971, 195.8439878601990074 ) ) ;
#16085=CARTESIAN_POINT ( 'NONE',  ( 9.863053695384421005, 1422.516288235769935, 212.3150749887220172 ) ) ;
#16086=CARTESIAN_POINT ( 'NONE',  ( -2.642143157096769723, 1488.503634608570110, 219.7172765930159812 ) ) ;
#16087=CARTESIAN_POINT ( 'NONE',  ( -4.329448776040000446, 1515.064792882589927, 207.2788837304390199 ) ) ;
#16090=CARTESIAN_POINT ( 'NONE',  ( 10.52942987710000011, 1470.684214315490181, 209.6684282404120268 ) ) ;
#16091=CARTESIAN_POINT ( 'NONE',  ( 10.71868385741180063, 1491.403514958749838, 211.6561026201489994 ) ) ;
#16092=CARTESIAN_POINT ( 'NONE',  ( -2.406810632960000085, 1456.459620267289893, 218.3084222088889987 ) ) ;
#16095=EDGE_CURVE ( 'NONE', #26746, #98016, #66178, .T. ) ;
#16101=ORIENTED_EDGE ( 'NONE', *, *, #50292, .T. ) ;
#16103=CARTESIAN_POINT ( 'NONE',  ( -2.031883754679999932, 1464.998375783689880, 198.3053765207990011 ) ) ;
#16107=B_SPLINE_CURVE_WITH_KNOTS ( 'NONE', 3,
 ( #6442, #110002, #40587, #110549, #84782, #67469, #33279, #41137, #65809, #49560, #23221, #50651, #74759, #102135, #24325, #57421, #84238, #16456, #92638 ),
 .UNSPECIFIED., .F., .F.,
 ( 4, 3, 3, 3, 3, 3, 4 ),
 ( -6.749361099460109870, -6.540428904467110449, -5.576190169441640698, -4.758631760330019667, -4.110056285970450141, -3.404977062924410269, -2.767901846390000031 ),
 .UNSPECIFIED. ) ;
#16108=CARTESIAN_POINT ( 'NONE',  ( 11.74864212650039796, 1479.742741897189944, 210.0210730748829917 ) ) ;
#16110=LINE ( 'NONE', #67113, #5256 ) ;
#16122=CARTESIAN_POINT ( 'NONE',  ( -19.72225066010199868, 1467.596931137250067, 204.3544451804700088 ) ) ;
#16126=CARTESIAN_POINT ( 'NONE',  ( 2.330134126718832910, 1515.372048949687041, 213.3835825136068536 ) ) ;
#16128=CARTESIAN_POINT ( 'NONE',  ( -1.969513130946940027, 1420.780713718789912, 193.8325181973079907 ) ) ;
#16129=CARTESIAN_POINT ( 'NONE',  ( 1.616750372209999842, 1476.357240329989963, 198.1368238248990110 ) ) ;
#16135=CARTESIAN_POINT ( 'NONE',  ( -8.112557822769998594, 1425.521057321509943, 208.4541235294330193 ) ) ;
#16139=B_SPLINE_CURVE_WITH_KNOTS ( 'NONE', 3,
 ( #40210, #58679, #16625, #50821, #14987, #41322, #23401, #92814, #16085, #33441, #67640, #84952, #42412, #82765, #76566, #57036, #91163, #14438, #48635, #6057, #31806, #100115 ),
 .UNSPECIFIED., .F., .F.,
 ( 4, 3, 3, 3, 3, 3, 3, 4 ),
 ( -8.540286635490000222, -8.454071259740000954, -7.782260918187459353, -6.926036427371090376, -6.070163583882830061, -5.213710336174729676, -4.355629079344280008, -3.495541850680000451 ),
 .UNSPECIFIED. ) ;
#16140=B_SPLINE_SURFACE_WITH_KNOTS ( 'NONE', 5, 5, ( 
 ( #5734, #14664, #23051, #99762, #6810, #65095 ),
 ( #39325, #75148, #32021, #66210, #65645, #32580 ),
 ( #91386, #82977, #73498, #98675, #6270, #21937 ),
 ( #81314, #66756, #100858, #24149, #74044, #108173 ),
 ( #47187, #58339, #30916, #4629, #38765, #47733 ),
 ( #31465, #58887, #17953, #93020, #42632, #16293 ),
 ( #49935, #101397, #85723, #69518, #1197, #35329 ),
 ( #59452, #93563, #25804, #51591, #109836, #7372 ),
 ( #26366, #41535, #67304, #84619, #67851, #75693 ) ),
 .UNSPECIFIED., .F., .F., .F.,
 ( 6, 3, 6 ),
 ( 6, 6 ),
 ( 106.4131865259999898, 113.5701753800000091, 117.7436754830000041 ),
 ( 0.000000000000000000, 1.000000014787439939 ),
 .UNSPECIFIED. ) ;
#16142=CARTESIAN_POINT ( 'NONE',  ( -8.147283189284854288, 1471.380150889464176, 215.1678129514797320 ) ) ;
#16143=CARTESIAN_POINT ( 'NONE',  ( 7.295790646376310029, 1426.429901798619994, 212.8040195462420172 ) ) ;
#16152=CARTESIAN_POINT ( 'NONE',  ( 13.45406242349999992, 1426.801272845689937, 196.6926870375990006 ) ) ;
#16154=CARTESIAN_POINT ( 'NONE',  ( 4.952364187259999717, 1425.023410992210302, 209.4642470625779822 ) ) ;
#16158=CARTESIAN_POINT ( 'NONE',  ( 9.881164057279999469, 1462.277409695889901, 209.5389570254230023 ) ) ;
#16159=ORIENTED_EDGE ( 'NONE', *, *, #32082, .F. ) ;
#16166=CARTESIAN_POINT ( 'NONE',  ( 3.224559923908230097, 1508.551704408090018, 213.9552828354289886 ) ) ;
#16174=TOROIDAL_SURFACE ( 'NONE', #5418, 14.90133124319999780, 0.5000000000000000000 ) ;
#16176=ORIENTED_EDGE ( 'NONE', *, *, #70801, .F. ) ;
#16177=CARTESIAN_POINT ( 'NONE',  ( -10.98190293991350153, 1481.156708494670283, 209.8541006977949905 ) ) ;
#16180=CARTESIAN_POINT ( 'NONE',  ( -2.487935123020000194, 1508.551704408389924, 214.1089243778970115 ) ) ;
#16181=CARTESIAN_POINT ( 'NONE',  ( 11.04300719229690131, 1502.511714738169985, 215.4559327082369862 ) ) ;
#16182=CARTESIAN_POINT ( 'NONE',  ( 7.729057984899998957, 1421.712257409790027, 195.7954043856990154 ) ) ;
#16184=CARTESIAN_POINT ( 'NONE',  ( -5.445057622820000276, 1494.866989841090117, 198.0707108858990182 ) ) ;
#16195=CARTESIAN_POINT ( 'NONE',  ( -11.15230584153099969, 1482.963738427830094, 204.9460026512250010 ) ) ;
#16197=CARTESIAN_POINT ( 'NONE',  ( 10.09736402354529794, 1428.020344045030015, 211.7362985889099889 ) ) ;
#16198=CARTESIAN_POINT ( 'NONE',  ( 11.80143010066550069, 1421.702045332599937, 203.4210871111559982 ) ) ;
#16203=CARTESIAN_POINT ( 'NONE',  ( 8.009058649040055045, 1433.461145011983263, 203.5451010711497872 ) ) ;
#16204=CARTESIAN_POINT ( 'NONE',  ( -11.03351704759920082, 1462.446871292220067, 208.7211331332790110 ) ) ;
#16207=CARTESIAN_POINT ( 'NONE',  ( 10.73757766294639993, 1423.674038311519780, 203.2439027591769900 ) ) ;
#16208=CARTESIAN_POINT ( 'NONE',  ( 6.068309900360460141, 1465.453006015229903, 217.9033581894499889 ) ) ;
#16219=CARTESIAN_POINT ( 'NONE',  ( 2.475018581880529922, 1497.111080376900190, 196.9667223532030107 ) ) ;
#16220=CARTESIAN_POINT ( 'NONE',  ( -15.33279031426130068, 1420.632256028889969, 207.8836982448250126 ) ) ;
#16231=CARTESIAN_POINT ( 'NONE',  ( -10.16240513719999861, 1472.558925768189965, 209.8189303923120121 ) ) ;
#16235=CARTESIAN_POINT ( 'NONE',  ( -3.163504309968519834, 1432.488551548530268, 217.0769143716860015 ) ) ;
#16242=CARTESIAN_POINT ( 'NONE',  ( 11.04921975785680033, 1422.238644613519909, 209.3273474340340101 ) ) ;
#16247=CARTESIAN_POINT ( 'NONE',  ( 0.7056569705168199702, 1437.738171567159952, 227.6607474309619761 ) ) ;
#16248=ORIENTED_EDGE ( 'NONE', *, *, #40030, .F. ) ;
#16249=CARTESIAN_POINT ( 'NONE',  ( 2.873384031200000077, 1474.047582638690074, 219.3741047921989775 ) ) ;
#16252=CARTESIAN_POINT ( 'NONE',  ( -10.78591527280000051, 1493.388845731089987, 206.2900157096790110 ) ) ;
#16258=FACE_OUTER_BOUND ( 'NONE', #8995, .T. ) ;
#16260=FACE_OUTER_BOUND ( 'NONE', #63398, .T. ) ;
#16261=CARTESIAN_POINT ( 'NONE',  ( -3.187121981100000223, 1456.171761825189833, 200.1942474277390147 ) ) ;
#16264=ORIENTED_EDGE ( 'NONE', *, *, #80365, .T. ) ;
#16267=CARTESIAN_POINT ( 'NONE',  ( -3.403507246419999799, 1496.471359390990074, 198.2852391338990117 ) ) ;
#16269=VERTEX_POINT ( 'NONE', #11174 ) ;
#16278=DIRECTION ( 'NONE',  ( 7.303600220002790452E-17, 1.000000000000000000, -3.615388577796539518E-17 ) ) ;
#16280=CARTESIAN_POINT ( 'NONE',  ( 8.001917699090000724, 1477.391948627790043, 200.4742795864889899 ) ) ;
#16281=CARTESIAN_POINT ( 'NONE',  ( 12.67493581254619883, 1500.776964490709815, 210.0452443345189977 ) ) ;
#16282=CARTESIAN_POINT ( 'NONE',  ( 4.877535505899020407, 1508.551704408389924, 212.3411737844989773 ) ) ;
#16288=ORIENTED_EDGE ( 'NONE', *, *, #30765, .T. ) ;
#16289=CARTESIAN_POINT ( 'NONE',  ( 0.4279777614790010176, 1433.008008888489940, 203.3794752007089812 ) ) ;
#16293=CARTESIAN_POINT ( 'NONE',  ( -15.30294433438259993, 1508.551704408389924, 210.3674297289989852 ) ) ;
#16295=CARTESIAN_POINT ( 'NONE',  ( -5.720967295801010266, 1454.603207479829962, 201.6563704129750079 ) ) ;
#16298=CARTESIAN_POINT ( 'NONE',  ( 9.181048108447960487, 1450.963731741589982, 210.1938350974689911 ) ) ;
#16306=B_SPLINE_CURVE_WITH_KNOTS ( 'NONE', 5,
 ( #13893, #64896, #106322, #105228, #62716, #13337, #20104, #48079, #88425 ),
 .UNSPECIFIED., .F., .F.,
 ( 6, 3, 6 ),
 ( 395.8612471010000036, 395.8828220460000011, 406.1136973210000178 ),
 .UNSPECIFIED. ) ;
#16307=AXIS2_PLACEMENT_3D ( 'NONE', #5475, #48601, #98427 ) ;
#16312=CARTESIAN_POINT ( 'NONE',  ( -17.53631869671869836, 1419.865669823370126, 206.1936457225280321 ) ) ;
#16314=CARTESIAN_POINT ( 'NONE',  ( -9.843061056976221579, 1461.614501156679808, 208.6143076776489806 ) ) ;
#16316=CARTESIAN_POINT ( 'NONE',  ( 10.23972724447879834, 1469.612255671459934, 207.2726204608819955 ) ) ;
#16317=CARTESIAN_POINT ( 'NONE',  ( -10.17586086920000099, 1472.204187410889972, 204.7702763186189827 ) ) ;
#16318=CARTESIAN_POINT ( 'NONE',  ( -10.90539778630000001, 1489.991646564889834, 212.3805117938089779 ) ) ;
#16325=ORIENTED_EDGE ( 'NONE', *, *, #39548, .T. ) ;
#16333=CARTESIAN_POINT ( 'NONE',  ( -11.41430924156969873, 1500.917495223069864, 211.1256234948569954 ) ) ;
#16336=CARTESIAN_POINT ( 'NONE',  ( -0.3395211818530010084, 1508.109360918889934, 220.9281624441990175 ) ) ;
#16338=CARTESIAN_POINT ( 'NONE',  ( 1.749019635934000005, 1431.032422837999775, 199.8154693994979993 ) ) ;
#16340=CARTESIAN_POINT ( 'NONE',  ( -11.36959371680000075, 1503.847165134090119, 207.0750569533189775 ) ) ;
#16345=CARTESIAN_POINT ( 'NONE',  ( -11.84683861278779915, 1482.181305081889832, 208.0213636573200233 ) ) ;
#16357=CARTESIAN_POINT ( 'NONE',  ( -15.51485357750000205, 1417.141638888899934, 205.6853114639490059 ) ) ;
#16360=CARTESIAN_POINT ( 'NONE',  ( -16.22004022801489143, 1419.733241725250082, 209.9150677488009933 ) ) ;
#16361=CARTESIAN_POINT ( 'NONE',  ( -3.703568344589999839, 1497.311626104689822, 220.9591690177990131 ) ) ;
#16362=CARTESIAN_POINT ( 'NONE',  ( -2.483162238130000254, 1476.934831443589928, 201.9767984309089854 ) ) ;
#16363=CARTESIAN_POINT ( 'NONE',  ( -18.56011888160000112, 1441.602307344989867, 211.8044997558990303 ) ) ;
#16364=CARTESIAN_POINT ( 'NONE',  ( 10.55629857124240090, 1481.744597751460105, 209.9319926063880075 ) ) ;
#16380=CARTESIAN_POINT ( 'NONE',  ( 4.650698360960000777, 1484.263765184789918, 220.0138998524990086 ) ) ;
#16383=CARTESIAN_POINT ( 'NONE',  ( -8.069527880069999881, 1440.230228425089763, 228.7261013027990089 ) ) ;
#16386=CARTESIAN_POINT ( 'NONE',  ( -16.94686494584989944, 1417.489848084730056, 207.8186904396790169 ) ) ;
#16407=CARTESIAN_POINT ( 'NONE',  ( -15.96075179420000367, 1466.903945902690111, 196.1521398069990312 ) ) ;
#16415=CARTESIAN_POINT ( 'NONE',  ( 2.158120808530000101, 1468.703739625189883, 218.9192338835489977 ) ) ;
#16416=FACE_OUTER_BOUND ( 'NONE', #76385, .T. ) ;
#16417=SURFACE_STYLE_FILL_AREA ( #15863 ) ;
#16418=CARTESIAN_POINT ( 'NONE',  ( 4.660514127639999060, 1441.207016471189945, 213.1086252044090088 ) ) ;
#16424=ORIENTED_EDGE ( 'NONE', *, *, #38611, .F. ) ;
#16425=ORIENTED_EDGE ( 'NONE', *, *, #75423, .F. ) ;
#16429=CARTESIAN_POINT ( 'NONE',  ( -7.313058470103319664, 1475.195669987933570, 201.8552237540184535 ) ) ;
#16432=CARTESIAN_POINT ( 'NONE',  ( 11.58978176042640129, 1422.008781663779928, 209.7162554888329851 ) ) ;
#16445=CARTESIAN_POINT ( 'NONE',  ( 3.960829545962760267, 1442.649591851693231, 217.0772145634146284 ) ) ;
#16446=CARTESIAN_POINT ( 'NONE',  ( 5.407632277616277072, 1505.250895293119584, 219.8892970404575919 ) ) ;
#16447=CARTESIAN_POINT ( 'NONE',  ( 7.122515158009999681, 1452.871264857790266, 215.2372064891289654 ) ) ;
#16450=CARTESIAN_POINT ( 'NONE',  ( -3.188751157463979968, 1428.815501146380029, 200.3155279938000035 ) ) ;
#16453=EDGE_CURVE ( 'NONE', #13558, #27509, #71352, .T. ) ;
#16456=CARTESIAN_POINT ( 'NONE',  ( 9.367166360012699755, 1434.455447298550098, 206.3420816845940067 ) ) ;
#16457=CARTESIAN_POINT ( 'NONE',  ( -11.75537608917499810, 1482.386081586160117, 207.2708069926649728 ) ) ;
#16459=EDGE_CURVE ( 'NONE', #95667, #74706, #46744, .T. ) ;
#16467=EDGE_CURVE ( 'NONE', #105726, #714, #81104, .T. ) ;
#16471=CARTESIAN_POINT ( 'NONE',  ( -9.642223397419670050, 1460.679120766980077, 208.4218084076549928 ) ) ;
#16473=DIRECTION ( 'NONE',  ( -8.832268201338159945E-47, 1.000000000000000000, -1.836970198721029688E-16 ) ) ;
#16481=CARTESIAN_POINT ( 'NONE',  ( -7.615310476975459153, 1461.877859386345108, 203.0812156602634957 ) ) ;
#16482=ADVANCED_FACE ( 'NONE', ( #72725 ), #98577, .F. ) ;
#16493=ORIENTED_EDGE ( 'NONE', *, *, #69502, .F. ) ;
#16494=CARTESIAN_POINT ( 'NONE',  ( -7.834251258605340773, 1439.563479556370112, 205.1891270341679956 ) ) ;
#16496=EDGE_CURVE ( 'NONE', #4497, #39082, #25851, .T. ) ;
#16497=CARTESIAN_POINT ( 'NONE',  ( 11.40506975472390039, 1471.056480956299993, 209.4187964280920085 ) ) ;
#16500=CARTESIAN_POINT ( 'NONE',  ( 12.23427440210000050, 1501.005680718390067, 210.1402780287790222 ) ) ;
#16502=CARTESIAN_POINT ( 'NONE',  ( 8.071448428540000108, 1423.066654972070182, 213.1913406456689870 ) ) ;
#16503=CARTESIAN_POINT ( 'NONE',  ( -4.082778200585359230, 1515.071394777460000, 212.7081675216069812 ) ) ;
#16513=ORIENTED_EDGE ( 'NONE', *, *, #85173, .F. ) ;
#16518=CARTESIAN_POINT ( 'NONE',  ( -8.747337044410000928, 1447.713205128089839, 212.1116229988289774 ) ) ;
#16530=ORIENTED_EDGE ( 'NONE', *, *, #57775, .F. ) ;
#16534=CARTESIAN_POINT ( 'NONE',  ( 10.64883854889802706, 1501.422591975932619, 204.8277787321165135 ) ) ;
#16537=CARTESIAN_POINT ( 'NONE',  ( -0.2312796901443630038, 1475.734222155040015, 197.6677150511999912 ) ) ;
#16544=CARTESIAN_POINT ( 'NONE',  ( -4.326992699990039881, 1515.158586642889986, 209.1858684987689969 ) ) ;
#16546=ORIENTED_EDGE ( 'NONE', *, *, #100359, .F. ) ;
#16550=CARTESIAN_POINT ( 'NONE',  ( 8.314894252674610797, 1425.054012563349943, 194.6595790585679993 ) ) ;
#16565=CARTESIAN_POINT ( 'NONE',  ( 19.28191951490000022, 1455.753434004590190, 211.0002536610790003 ) ) ;
#16568=CARTESIAN_POINT ( 'NONE',  ( 10.63748064366419932, 1460.271151926629955, 206.6808178792470017 ) ) ;
#16572=CARTESIAN_POINT ( 'NONE',  ( -5.909698491649999497, 1449.521837735690042, 210.1656816284789784 ) ) ;
#16582=CARTESIAN_POINT ( 'NONE',  ( 7.357707608180000136, 1481.868694410790113, 209.7897133371670009 ) ) ;
#16586=CARTESIAN_POINT ( 'NONE',  ( -6.895941952979999456, 1414.058355658300115, 207.6209997343590032 ) ) ;
#16588=CARTESIAN_POINT ( 'NONE',  ( 3.702952669180000100, 1486.443463639589936, 198.8438389633990084 ) ) ;
#16600=CARTESIAN_POINT ( 'NONE',  ( -16.47162245365960231, 1508.551704408389924, 213.2650820600849784 ) ) ;
#16606=CARTESIAN_POINT ( 'NONE',  ( -11.37017053985569959, 1470.996082497490079, 208.1552749488289749 ) ) ;
#16607=CARTESIAN_POINT ( 'NONE',  ( -4.317515543852133320, 1508.177212360263866, 220.5973697276004657 ) ) ;
#16610=CARTESIAN_POINT ( 'NONE',  ( 9.170460176685850229, 1461.406028138000238, 205.9602226471569963 ) ) ;
#16613=CARTESIAN_POINT ( 'NONE',  ( -4.882940650389359760, 1421.798898707020044, 193.0164659316789937 ) ) ;
#16614=CARTESIAN_POINT ( 'NONE',  ( 10.78159850099999950, 1461.896569178690015, 211.1674767183390031 ) ) ;
#16617=ORIENTED_EDGE ( 'NONE', *, *, #21997, .F. ) ;
#16625=CARTESIAN_POINT ( 'NONE',  ( 9.368311761950069538, 1422.630913921370166, 212.8603802799670177 ) ) ;
#16626=CARTESIAN_POINT ( 'NONE',  ( 2.724649121582150002, 1508.551704408389924, 219.4861637980260127 ) ) ;
#16627=CARTESIAN_POINT ( 'NONE',  ( 2.740701793870000014, 1426.136123009330049, 188.7843822941989913 ) ) ;
#16630=B_SPLINE_CURVE_WITH_KNOTS ( 'NONE', 3,
 ( #102469, #83465, #24640, #43142, #75100, #58838, #6760, #109248, #100812, #16247, #101910, #16788, #9521, #95191, #19005, #77841, #53778, #87346, #11202, #61076, #10076, #62169, #19575, #1150, #60505 ),
 .UNSPECIFIED., .F., .F.,
 ( 4, 3, 3, 3, 3, 3, 3, 3, 4 ),
 ( 0.000000000000000000, 0.9296916835059300110, 1.856438681794639889, 2.777847123387560124, 3.503639760140000003, 4.428889518077550491, 5.349465545739890082, 6.262071350648260371, 6.986073851990000527 ),
 .UNSPECIFIED. ) ;
#16631=CARTESIAN_POINT ( 'NONE',  ( 4.789673499540000101, 1465.867933640490037, 219.0700355186390027 ) ) ;
#16633=CARTESIAN_POINT ( 'NONE',  ( -0.07060758185340119952, 1456.122775716790102, 218.7382961870089844 ) ) ;
#16638=CARTESIAN_POINT ( 'NONE',  ( 4.963083874980020127, 1508.551704408389924, 206.2781155379609856 ) ) ;
#16645=CARTESIAN_POINT ( 'NONE',  ( -0.7896334281179979708, 1469.097698168490069, 189.0743330492990140 ) ) ;
#16647=CARTESIAN_POINT ( 'NONE',  ( 11.59475102981150130, 1480.142125814169958, 211.2619558011750200 ) ) ;
#16654=CARTESIAN_POINT ( 'NONE',  ( 2.454239291473280016, 1432.341654353290096, 200.8702472344759826 ) ) ;
#16659=CARTESIAN_POINT ( 'NONE',  ( 11.10812020650000065, 1480.085810737090014, 229.8010407196990172 ) ) ;
#16664=CARTESIAN_POINT ( 'NONE',  ( -6.402980167960000024, 1474.343588456390080, 205.7752103392290337 ) ) ;
#16667=CARTESIAN_POINT ( 'NONE',  ( -2.168811436099340018, 1421.535665163839894, 193.6021455940999942 ) ) ;
#16669=CARTESIAN_POINT ( 'NONE',  ( -0.7261436049189990971, 1476.159678178889862, 198.3924679319989934 ) ) ;
#16674=CARTESIAN_POINT ( 'NONE',  ( 1.635180021967760133, 1429.354063412989944, 217.2616352817560141 ) ) ;
#16675=CARTESIAN_POINT ( 'NONE',  ( -8.133195396499999674, 1425.296577659349850, 209.0165728948540220 ) ) ;
#16676=AXIS2_PLACEMENT_3D ( 'NONE', #93761, #26575, #43401 ) ;
#16681=CARTESIAN_POINT ( 'NONE',  ( -6.915664125854886990, 1471.020592902175622, 216.5103502196423051 ) ) ;
#16682=CARTESIAN_POINT ( 'NONE',  ( 7.539441653064500315, 1425.666433134689896, 212.1875851909779840 ) ) ;
#16686=CARTESIAN_POINT ( 'NONE',  ( -11.03241518813069888, 1492.218220261629995, 207.1401972973099816 ) ) ;
#16690=CARTESIAN_POINT ( 'NONE',  ( 7.998636686930000295, 1425.977676336709919, 211.5360327896089814 ) ) ;
#16697=CARTESIAN_POINT ( 'NONE',  ( 8.602846452805209765, 1434.993060077820019, 206.5683719099479845 ) ) ;
#16699=ORIENTED_EDGE ( 'NONE', *, *, #72771, .T. ) ;
#16708=CARTESIAN_POINT ( 'NONE',  ( -6.054480185420000993, 1427.105311845340111, 201.8413580458289971 ) ) ;
#16712=CARTESIAN_POINT ( 'NONE',  ( -1.379923010975170117, 1444.345884097049975, 199.1632244479729934 ) ) ;
#16716=ADVANCED_FACE ( 'NONE', ( #96344 ), #22516, .F. ) ;
#16718=CARTESIAN_POINT ( 'NONE',  ( -4.865329319845380418, 1508.551704408389924, 212.3847752591109668 ) ) ;
#16721=CARTESIAN_POINT ( 'NONE',  ( 7.706547837850000526, 1421.685151551939953, 195.7783216092990131 ) ) ;
#16722=CARTESIAN_POINT ( 'NONE',  ( -2.162991289744210288, 1432.744035697870004, 218.4013281355300080 ) ) ;
#16723=DIRECTION ( 'NONE',  ( 0.9235695684098328417, -0.3795957984897049275, 0.05409512063244299035 ) ) ;
#16725=CARTESIAN_POINT ( 'NONE',  ( 3.892685920875734951, 1515.551704408391060, 210.6723607687643494 ) ) ;
#16733=CARTESIAN_POINT ( 'NONE',  ( -11.41675697748640061, 1482.775670443970057, 205.7339590229720159 ) ) ;
#16737=CARTESIAN_POINT ( 'NONE',  ( 0.6988675025901418536, 1421.239614905253347, 193.7316982519299131 ) ) ;
#16738=CARTESIAN_POINT ( 'NONE',  ( -10.96494705889580068, 1462.661034221799810, 207.7545830336519828 ) ) ;
#16744=B_SPLINE_CURVE_WITH_KNOTS ( 'NONE', 3,
 ( #50683, #67506, #101610, #84815 ),
 .UNSPECIFIED., .F., .F.,
 ( 4, 4 ),
 ( 0.000000000000000000, 1.000000000000000000 ),
 .UNSPECIFIED. ) ;
#16746=CARTESIAN_POINT ( 'NONE',  ( 11.17229582740980121, 1425.728672638270154, 197.4068991129149993 ) ) ;
#16748=CARTESIAN_POINT ( 'NONE',  ( 7.590528390105199641, 1465.207167611649993, 215.7443336111830092 ) ) ;
#16749=CARTESIAN_POINT ( 'NONE',  ( -10.06499177390000099, 1481.481388711089949, 205.8730018957789980 ) ) ;
#16753=CARTESIAN_POINT ( 'NONE',  ( -7.749759000068385362, 1426.484231355699649, 206.4869615271631460 ) ) ;
#16754=AXIS2_PLACEMENT_3D ( 'NONE', #109716, #58769, #41963 ) ;
#16755=CARTESIAN_POINT ( 'NONE',  ( 1.770954783930000165, 1478.892269184689894, 229.4302748609989919 ) ) ;
#16758=CARTESIAN_POINT ( 'NONE',  ( -4.994371530956574823, 1391.698117826116459, 203.8075142969990168 ) ) ;
#16759=CARTESIAN_POINT ( 'NONE',  ( -18.65941878286419708, 1468.219764057670091, 201.0822022773610058 ) ) ;
#16762=CARTESIAN_POINT ( 'NONE',  ( -16.30825986473579903, 1420.539997913489970, 204.8045917016430053 ) ) ;
#16772=B_SPLINE_SURFACE_WITH_KNOTS ( 'NONE', 5, 1, ( 
 ( #92225, #108482 ),
 ( #7123, #75453 ),
 ( #84911, #84379 ),
 ( #109045, #110130 ),
 ( #16582, #15496 ),
 ( #49694, #67050 ) ),
 .UNSPECIFIED., .F., .F., .F.,
 ( 6, 6 ),
 ( 2, 2 ),
 ( 0.000000000000000000, 3.826360078679999610 ),
 ( 0.000000000000000000, 14.00000000000000000 ),
 .UNSPECIFIED. ) ;
#16777=CARTESIAN_POINT ( 'NONE',  ( -5.888139897268749756, 1434.739753164839840, 216.8789263783159811 ) ) ;
#16779=CARTESIAN_POINT ( 'NONE',  ( -16.24206877649999825, 1420.056535900020208, 209.7634690437569986 ) ) ;
#16783=MECHANICAL_DESIGN_GEOMETRIC_PRESENTATION_REPRESENTATION('',(#102645),#93697);
#16785=CARTESIAN_POINT ( 'NONE',  ( 10.26114059010819979, 1426.067723122690040, 208.3384717249140010 ) ) ;
#16788=CARTESIAN_POINT ( 'NONE',  ( 0.08317272321623850329, 1437.870240068480143, 227.6823673113509869 ) ) ;
#16790=CARTESIAN_POINT ( 'NONE',  ( 1.617203238019999878, 1473.963834990890064, 219.3699067192990242 ) ) ;
#16793=CARTESIAN_POINT ( 'NONE',  ( -8.009280784559999589, 1493.871781897389837, 199.6961107241290279 ) ) ;
#16797=CARTESIAN_POINT ( 'NONE',  ( 1778.930368298719941, -2340.220200558880151, -8899.082583863100808 ) ) ;
#16798=CARTESIAN_POINT ( 'NONE',  ( 8.992866426550000014, 1449.909640413290163, 206.9381849123989809 ) ) ;
#16800=B_SPLINE_CURVE_WITH_KNOTS ( 'NONE', 3,
 ( #100111, #61326, #74931, #40204, #74386, #31799, #23392, #103259, #57582, #83308 ),
 .UNSPECIFIED., .F., .F.,
 ( 4, 2, 2, 2, 4 ),
 ( 0.000000000000000000, 0.2500000000000000000, 0.5000000000000000000, 0.7500000000000000000, 1.000000000000000000 ),
 .UNSPECIFIED. ) ;
#16805=B_SPLINE_SURFACE_WITH_KNOTS ( 'NONE', 5, 5, ( 
 ( #49278, #31351, #75589, #65535, #109720, #16184 ),
 ( #83407, #66643, #22932, #14543, #82314, #6702 ),
 ( #40305, #100744, #24029, #110261, #82858, #58228 ),
 ( #39765, #74488, #101846, #108615, #6148, #7802 ),
 ( #41968, #33537, #31904, #67737, #59343, #93452 ),
 ( #69401, #36316, #1637, #94012, #35775, #50925 ),
 ( #2202, #42508, #538, #62107, #69957, #78325 ),
 ( #8344, #18947, #85599, #27366, #102409, #8900 ),
 ( #110818, #10015, #70513, #43077, #17276, #34110 ) ),
 .UNSPECIFIED., .F., .F., .F.,
 ( 6, 3, 6 ),
 ( 6, 6 ),
 ( 21.89878892990000026, 23.58501803260000074, 25.27124713539999945 ),
 ( 0.000000000000000000, 2.000000000000000000 ),
 .UNSPECIFIED. ) ;
#16807=CARTESIAN_POINT ( 'NONE',  ( -2.228719191530000199, 1497.815835837290024, 198.0391072666990055 ) ) ;
#16824=CARTESIAN_POINT ( 'NONE',  ( -4.993299342540000296, 1391.657172602489936, 214.7214461112690174 ) ) ;
#16828=CARTESIAN_POINT ( 'NONE',  ( 9.742380785638999896, 1461.526748617359999, 207.6421447878750257 ) ) ;
#16830=ORIENTED_EDGE ( 'NONE', *, *, #40626, .F. ) ;
#16834=CARTESIAN_POINT ( 'NONE',  ( 10.13545575494789830, 1453.511789163979984, 212.2748783515349942 ) ) ;
#16835=B_SPLINE_CURVE_WITH_KNOTS ( 'NONE', 3,
 ( #43111, #94044, #110299, #26853, #35251, #50961, #101880, #34694, #61041, #94592 ),
 .UNSPECIFIED., .F., .F.,
 ( 4, 2, 2, 2, 4 ),
 ( 0.000000000000000000, 0.2500000000000000000, 0.5000000000000000000, 0.7500000000000000000, 1.000000000000000000 ),
 .UNSPECIFIED. ) ;
#16837=CARTESIAN_POINT ( 'NONE',  ( -12.16875361000624345, 1417.446348406323750, 199.6775038949584768 ) ) ;
#16838=CARTESIAN_POINT ( 'NONE',  ( 4.138993644619999301, 1515.551749209489799, 209.1218459616910081 ) ) ;
#16840=CARTESIAN_POINT ( 'NONE',  ( -6.679608332860329512, 1453.902887168129837, 202.5437545341480075 ) ) ;
#16843=CARTESIAN_POINT ( 'NONE',  ( 9.703365291897300793, 1451.752702013299995, 208.6594554766439842 ) ) ;
#16852=ORIENTED_EDGE ( 'NONE', *, *, #46636, .F. ) ;
#16857=CARTESIAN_POINT ( 'NONE',  ( -7.121746155459253380, 1489.817813860794558, 217.4260952101665225 ) ) ;
#16859=CARTESIAN_POINT ( 'NONE',  ( 9.951576027860420837, 1468.973797990169942, 207.5249271240780047 ) ) ;
#16860=CARTESIAN_POINT ( 'NONE',  ( -10.75661188380004418, 1470.034926440792788, 212.8112178691188490 ) ) ;
#16861=B_SPLINE_CURVE_WITH_KNOTS ( 'NONE', 5,
 ( #25878, #94194, #51665, #7443, #41607, #101477, #24764, #50564, #84690 ),
 .UNSPECIFIED., .F., .F.,
 ( 6, 3, 6 ),
 ( 0.000000000000000000, 0.3017171891571077680, 1.000000000000000000 ),
 .UNSPECIFIED. ) ;
#16862=CARTESIAN_POINT ( 'NONE',  ( 5.551014600700000301, 1493.954207117990109, 218.9115156736490064 ) ) ;
#16866=CARTESIAN_POINT ( 'NONE',  ( 8.171970832046620004, 1468.167223887809996, 201.4642853819800052 ) ) ;
#16871=EDGE_CURVE ( 'NONE', #79128, #76640, #40892, .T. ) ;
#16874=CARTESIAN_POINT ( 'NONE',  ( -14.77492446850000007, 1416.181292664740113, 213.5220302499890010 ) ) ;
#16877=ORIENTED_EDGE ( 'NONE', *, *, #74029, .F. ) ;
#16879=CARTESIAN_POINT ( 'NONE',  ( -0.3666539600740010285, 1508.474565598290155, 220.5579631546989958 ) ) ;
#16888=CARTESIAN_POINT ( 'NONE',  ( -11.60387529539999996, 1481.105535806189891, 211.4044418315190228 ) ) ;
#16896=CARTESIAN_POINT ( 'NONE',  ( 3.409608495353340096, 1454.219151911930112, 217.8661643445310006 ) ) ;
#16900=CARTESIAN_POINT ( 'NONE',  ( -16.42372150539999964, 1417.596044428880077, 205.5727566756989972 ) ) ;
#16904=CARTESIAN_POINT ( 'NONE',  ( -7.485183872730000409, 1498.430015208389932, 218.3832652741589868 ) ) ;
#16909=CARTESIAN_POINT ( 'NONE',  ( 10.52884532342740087, 1481.875038510340119, 210.3006225101370035 ) ) ;
#16923=DIRECTION ( 'NONE',  ( 0.9531756543815217420, 0.2975207091418809457, -0.05419962662297508199 ) ) ;
#16926=CARTESIAN_POINT ( 'NONE',  ( 4.146834721160000292, 1484.913268816489790, 219.4317166241989980 ) ) ;
#16927=CARTESIAN_POINT ( 'NONE',  ( 11.60982339427470045, 1478.971968693290137, 207.2338189534640094 ) ) ;
#16930=CARTESIAN_POINT ( 'NONE',  ( 20.44998473589999932, 1433.812659856489972, 214.5407056977390141 ) ) ;
#16932=CARTESIAN_POINT ( 'NONE',  ( 22.14279730894140030, 1473.984189750450014, 210.1089390468149816 ) ) ;
#16933=CARTESIAN_POINT ( 'NONE',  ( -17.00797328670000397, 1417.537217351680056, 207.7155449971589860 ) ) ;
#16936=CARTESIAN_POINT ( 'NONE',  ( 9.814145740701999188, 1435.717597957500175, 209.6091522368750191 ) ) ;
#16938=CARTESIAN_POINT ( 'NONE',  ( 4.382345708037679977, 1446.936631694319885, 199.9395551071150123 ) ) ;
#16943=CARTESIAN_POINT ( 'NONE',  ( 11.65102058319489764, 1433.170051679079961, 223.4015529330449965 ) ) ;
#16951=CARTESIAN_POINT ( 'NONE',  ( -4.675540975309999681, 1462.620895424390028, 200.5633310686890241 ) ) ;
#16952=AXIS2_PLACEMENT_3D ( 'NONE', #20308, #65093, #29818 ) ;
#16959=CARTESIAN_POINT ( 'NONE',  ( 0.9486209649339989447, 1468.174413863890095, 219.2298037005990068 ) ) ;
#16962=CARTESIAN_POINT ( 'NONE',  ( 5.296889735339999739, 1440.180353386090019, 211.9351589163190113 ) ) ;
#16973=CARTESIAN_POINT ( 'NONE',  ( -7.719721968511599641, 1475.003672383036246, 202.3105564095348825 ) ) ;
#16990=CARTESIAN_POINT ( 'NONE',  ( -17.13479123734510168, 1508.551704408389924, 210.3956667297300100 ) ) ;
#16995=CARTESIAN_POINT ( 'NONE',  ( -2.963941339955419974, 1428.941128588449828, 200.2350009049089863 ) ) ;
#17001=CARTESIAN_POINT ( 'NONE',  ( -11.87061842454789939, 1482.038080002969991, 208.5196970344390195 ) ) ;
#17008=CARTESIAN_POINT ( 'NONE',  ( 10.92413054773749970, 1490.487280210450081, 210.1135723924519993 ) ) ;
#17013=CARTESIAN_POINT ( 'NONE',  ( 13.84742034927229959, 1420.584111001059910, 203.1248729974179810 ) ) ;
#17015=CARTESIAN_POINT ( 'NONE',  ( -9.294437129912410001, 1449.358304634600017, 208.4206774063060266 ) ) ;
#17019=CARTESIAN_POINT ( 'NONE',  ( -12.43204788642049863, 1508.443254155279874, 217.5037917836490067 ) ) ;
#17024=CARTESIAN_POINT ( 'NONE',  ( 3.970758181649999496, 1467.502840618489927, 218.2663495880690050 ) ) ;
#17029=CARTESIAN_POINT ( 'NONE',  ( -2.480175263330000046, 1429.207669914089820, 200.0830570310090195 ) ) ;
#17031=CARTESIAN_POINT ( 'NONE',  ( 6.263489101080928378, 1465.252787188384445, 218.2607468416194365 ) ) ;
#17041=CARTESIAN_POINT ( 'NONE',  ( 12.44780703220000184, 1501.268281258290017, 211.7240718627089962 ) ) ;
#17042=CARTESIAN_POINT ( 'NONE',  ( -18.09135377717698034, 1468.316747749531032, 200.5084487035089751 ) ) ;
#17044=B_SPLINE_SURFACE_WITH_KNOTS ( 'NONE', 5, 1, ( 
 ( #96012, #96575 ),
 ( #64089, #19282 ),
 ( #10348, #1984 ),
 ( #99296, #22571 ),
 ( #99851, #107721 ),
 ( #55691, #48940 ) ),
 .UNSPECIFIED., .F., .F., .F.,
 ( 6, 6 ),
 ( 2, 2 ),
 ( 0.000000000000000000, 3.632392088579999623 ),
 ( 0.000000000000000000, 14.00000000000000000 ),
 .UNSPECIFIED. ) ;
#17045=CARTESIAN_POINT ( 'NONE',  ( 7.788301635029999836, 1423.125804053390084, 213.4136639638890074 ) ) ;
#17046=FACE_OUTER_BOUND ( 'NONE', #17723, .T. ) ;
#17057=DIRECTION ( 'NONE',  ( 0.9980318515193541407, 1.681712440757244397E-31, 0.06270903725022322628 ) ) ;
#17061=CARTESIAN_POINT ( 'NONE',  ( -9.033607467220001297, 1447.303979291489895, 212.0883436982290107 ) ) ;
#17066=CARTESIAN_POINT ( 'NONE',  ( -13.32684181309999971, 1469.522592936189994, 191.9925905970989959 ) ) ;
#17071=CARTESIAN_POINT ( 'NONE',  ( -21.53565904410000087, 1506.077647802389947, 209.2113159668039941 ) ) ;
#17074=CARTESIAN_POINT ( 'NONE',  ( 11.19147557906589974, 1422.145537183640045, 210.4506353095700035 ) ) ;
#17083=ADVANCED_FACE ( 'NONE', ( #23880 ), #97161, .T. ) ;
#17089=CARTESIAN_POINT ( 'NONE',  ( -8.773114743372520508, 1448.864173605930091, 211.7399132152989978 ) ) ;
#17092=EDGE_LOOP ( 'NONE', ( #110231, #109888, #54375, #91617 ) ) ;
#17095=ORIENTED_EDGE ( 'NONE', *, *, #50748, .T. ) ;
#17104=EDGE_CURVE ( 'NONE', #14695, #87290, #108720, .T. ) ;
#17119=CARTESIAN_POINT ( 'NONE',  ( 6.832578770827522519, 1420.119835273649869, 222.9246289101963896 ) ) ;
#17132=CARTESIAN_POINT ( 'NONE',  ( -9.647687026466609694, 1493.068473758189839, 201.4942496940060153 ) ) ;
#17149=ADVANCED_BREP_SHAPE_REPRESENTATION ( '', ( #9778, #21632 ), #28938 ) ;
#17156=CARTESIAN_POINT ( 'NONE',  ( -7.220970672452868833, 1508.392792329803569, 219.6893434555957185 ) ) ;
#17158=CARTESIAN_POINT ( 'NONE',  ( 10.93233376569999926, 1490.536113732890044, 207.1036721549689901 ) ) ;
#17161=CARTESIAN_POINT ( 'NONE',  ( -8.629751412190879378, 1419.780543030299896, 195.8880434429399884 ) ) ;
#17162=CARTESIAN_POINT ( 'NONE',  ( 4.327051608332269872, 1515.156337024050117, 208.9297172523390032 ) ) ;
#17166=EDGE_CURVE ( 'NONE', #102315, #106368, #76642, .T. ) ;
#17171=CARTESIAN_POINT ( 'NONE',  ( -10.40181139226799978, 1479.469451619749861, 210.4662640014259978 ) ) ;
#17174=AXIS2_PLACEMENT_3D ( 'NONE', #44761, #44200, #76682 ) ;
#17175=CARTESIAN_POINT ( 'NONE',  ( -14.38096556510000035, 1422.143733531690032, 196.2925564653990023 ) ) ;
#17192=CARTESIAN_POINT ( 'NONE',  ( -4.602356253840000022, 1468.583955076089978, 189.7619545879989857 ) ) ;
#17193=CARTESIAN_POINT ( 'NONE',  ( -6.264689016930000243, 1463.667333189490137, 201.0440036769589938 ) ) ;
#17207=CARTESIAN_POINT ( 'NONE',  ( 10.59812014278140069, 1477.523980704680071, 229.9254261715079792 ) ) ;
#17211=ADVANCED_FACE ( 'NONE', ( #45701 ), #12622, .T. ) ;
#17215=CARTESIAN_POINT ( 'NONE',  ( -12.80491917260000001, 1502.810374455390047, 208.8309748505670029 ) ) ;
#17216=CARTESIAN_POINT ( 'NONE',  ( -2.003732309335499728, 1420.923232009330150, 193.8159282254100049 ) ) ;
#17218=CARTESIAN_POINT ( 'NONE',  ( 0.6561095716360010321, 1477.838425433890052, 198.7002117315989835 ) ) ;
#17225=EDGE_CURVE ( 'NONE', #10311, #106390, #105029, .T. ) ;
#17230=CARTESIAN_POINT ( 'NONE',  ( 7.182548959824419654, 1426.565124233989764, 213.0328279948139993 ) ) ;
#17233=B_SPLINE_CURVE_WITH_KNOTS ( 'NONE', 3,
 ( #60050, #85215, #23663, #15248, #24739, #94168, #49440, #25294, #75195, #149, #34270, #83562, #33163, #68452, #6855, #58936, #67352, #102555, #109346, #74641, #25848, #32627, #100904, #48900, #84119, #83027, #24201, #58387 ),
 .UNSPECIFIED., .F., .F.,
 ( 4, 3, 3, 3, 3, 3, 3, 3, 3, 4 ),
 ( -41.05058650750000027, -39.67091674781929811, -38.29124698813869543, -36.91872546091649809, -35.54143844538869956, -34.17184909951799909, -32.80586366775889928, -31.44473546961619803, -30.07247103563280177, -28.72930409989999845 ),
 .UNSPECIFIED. ) ;
#17239=CARTESIAN_POINT ( 'NONE',  ( 4.718773895884976532, 1428.060710547474855, 215.9373307104791309 ) ) ;
#17242=FACE_OUTER_BOUND ( 'NONE', #5544, .T. ) ;
#17245=ORIENTED_EDGE ( 'NONE', *, *, #83127, .T. ) ;
#17262=CARTESIAN_POINT ( 'NONE',  ( -3.994937571899999984, 1430.106198350590148, 201.8091617873290033 ) ) ;
#17266=CARTESIAN_POINT ( 'NONE',  ( -1.329273608271069884, 1444.363671018100149, 199.1564131946590237 ) ) ;
#17269=CARTESIAN_POINT ( 'NONE',  ( 3.961806501186879270, 1508.551704407889929, 204.5769769800630229 ) ) ;
#17272=CARTESIAN_POINT ( 'NONE',  ( 2.487935123032368967, 1508.551704413348716, 204.2634855739857187 ) ) ;
#17273=CARTESIAN_POINT ( 'NONE',  ( 12.19144863275480084, 1501.599284162290132, 212.7637707930009867 ) ) ;
#17274=CARTESIAN_POINT ( 'NONE',  ( 7.503571368420000276, 1422.857534295030064, 195.6852864414989881 ) ) ;
#17276=CARTESIAN_POINT ( 'NONE',  ( -3.394304855489999717, 1495.766742607790093, 197.6817024317990104 ) ) ;
#17289=CARTESIAN_POINT ( 'NONE',  ( 8.168301522416200555, 1425.263768431070048, 211.0005860271879783 ) ) ;
#17298=CARTESIAN_POINT ( 'NONE',  ( -9.854800274776160052, 1461.491539507700054, 209.0809694339070006 ) ) ;
#17299=CARTESIAN_POINT ( 'NONE',  ( -14.06005930971490159, 1420.585608153310204, 196.0549662394890049 ) ) ;
#17300=CARTESIAN_POINT ( 'NONE',  ( 8.091109713897852274, 1420.444008331189934, 195.3478219760000059 ) ) ;
#17301=CARTESIAN_POINT ( 'NONE',  ( 4.575282349084649702, 1466.769470911500093, 218.0850143904499987 ) ) ;
#17310=CARTESIAN_POINT ( 'NONE',  ( -1.842963219479999859, 1515.064792519189950, 204.7923971761390192 ) ) ;
#17312=CARTESIAN_POINT ( 'NONE',  ( 24.11200014938239988, 1496.633575606299928, 206.8275456630500173 ) ) ;
#17314=CARTESIAN_POINT ( 'NONE',  ( -15.08395737488610067, 1420.916320493289959, 206.4749953940769842 ) ) ;
#17317=CARTESIAN_POINT ( 'NONE',  ( 4.093882882269999968, 1442.069604321789939, 216.9756720149090086 ) ) ;
#17324=CARTESIAN_POINT ( 'NONE',  ( -7.381443632628819529, 1508.551704407720081, 219.0920119588899979 ) ) ;
#17326=CARTESIAN_POINT ( 'NONE',  ( -10.57842363610000014, 1471.306182025889939, 209.0456894757570296 ) ) ;
#17329=CARTESIAN_POINT ( 'NONE',  ( 6.245177529333449939, 1505.788460192030016, 215.5597741259620079 ) ) ;
#17331=CARTESIAN_POINT ( 'NONE',  ( -1.839380708780000040, 1507.096886517889970, 221.8368464039990045 ) ) ;
#17332=CARTESIAN_POINT ( 'NONE',  ( -3.430374836980000008, 1431.708658569990121, 216.7924588047190184 ) ) ;
#17333=CARTESIAN_POINT ( 'NONE',  ( -10.62349018368750109, 1471.736129748900112, 206.9324528759129862 ) ) ;
#17339=CARTESIAN_POINT ( 'NONE',  ( 11.67851423121779852, 1427.517936626490155, 209.0836788490910010 ) ) ;
#17344=CARTESIAN_POINT ( 'NONE',  ( 2.500011071270000329, 1474.146030601790017, 219.4741456703989968 ) ) ;
#17347=CARTESIAN_POINT ( 'NONE',  ( -6.022896404259999947, 1495.447110633389912, 199.4947492194089875 ) ) ;
#17348=EDGE_CURVE ( 'NONE', #45555, #7001, #61913, .T. ) ;
#17353=CARTESIAN_POINT ( 'NONE',  ( 5.094924673369999546, 1446.258997694789969, 201.5711013011589898 ) ) ;
#17354=CARTESIAN_POINT ( 'NONE',  ( -8.530891852070000780, 1512.492641972989759, 210.8763812180689854 ) ) ;
#17356=CARTESIAN_POINT ( 'NONE',  ( -2.416533552610000246, 1456.578277723489919, 199.9325152207989902 ) ) ;
#17361=DIRECTION ( 'NONE',  ( -1.876463901673629690E-05, 8.203947739369057955E-07, 0.9999999998236077658 ) ) ;
#17363=B_SPLINE_CURVE_WITH_KNOTS ( 'NONE', 5,
 ( #46399, #107918, #63744, #5463, #30101, #97857 ),
 .UNSPECIFIED., .F., .F.,
 ( 6, 6 ),
 ( 0.000000000000000000, 1.000000000000000000 ),
 .UNSPECIFIED. ) ;
#17364=CARTESIAN_POINT ( 'NONE',  ( 2.020666342550000216, 1495.217427720489923, 220.5028442773989923 ) ) ;
#17365=ORIENTED_EDGE ( 'NONE', *, *, #68866, .T. ) ;
#17367=LINE ( 'NONE', #618, #92116 ) ;
#17380=CARTESIAN_POINT ( 'NONE',  ( 3.179309441343999953, 1508.551704408389924, 214.0112856217869819 ) ) ;
#17384=CARTESIAN_POINT ( 'NONE',  ( 10.49671714463670114, 1460.103773102299783, 206.1611881418880046 ) ) ;
#17387=ORIENTED_EDGE ( 'NONE', *, *, #96111, .T. ) ;
#17392=CARTESIAN_POINT ( 'NONE',  ( -6.218080811995890578, 1508.050148686579860, 220.4488469885409927 ) ) ;
#17399=CARTESIAN_POINT ( 'NONE',  ( 9.315848094708581328, 1450.961990831169942, 207.9471377613749894 ) ) ;
#17408=EDGE_LOOP ( 'NONE', ( #61118, #70744, #95378, #98258 ) ) ;
#17412=CARTESIAN_POINT ( 'NONE',  ( -7.217719862338501713, 1489.850359190520294, 217.3448569486999133 ) ) ;
#17422=TOROIDAL_SURFACE ( 'NONE', #101432, 7.500000000000000000, 0.2999999999999999889 ) ;
#17428=CARTESIAN_POINT ( 'NONE',  ( -14.35630723490000094, 1415.677402202029953, 213.7176790535390012 ) ) ;
#17429=CARTESIAN_POINT ( 'NONE',  ( -11.25861335519799944, 1500.241393668199862, 210.8792608383079994 ) ) ;
#17430=ORIENTED_EDGE ( 'NONE', *, *, #18739, .T. ) ;
#17431=B_SPLINE_CURVE_WITH_KNOTS ( 'NONE', 5,
 ( #85032, #42487, #76643, #8873, #34642, #26792 ),
 .UNSPECIFIED., .F., .F.,
 ( 6, 6 ),
 ( -2.000000000000000000, 0.000000000000000000 ),
 .UNSPECIFIED. ) ;
#17442=CARTESIAN_POINT ( 'NONE',  ( -10.87893655264359971, 1481.987309145149766, 207.2182299508939991 ) ) ;
#17453=DIRECTION ( 'NONE',  ( -0.9057425179572490270, -0.3859240281742280509, 0.1751945651047430164 ) ) ;
#17454=CARTESIAN_POINT ( 'NONE',  ( -16.24601214319999798, 1417.782919326170031, 204.8291993099989838 ) ) ;
#17457=CARTESIAN_POINT ( 'NONE',  ( -15.84432591830269743, 1419.853212859319910, 210.7451195136700051 ) ) ;
#17459=EDGE_LOOP ( 'NONE', ( #40128, #8393, #29023, #107649 ) ) ;
#17463=CARTESIAN_POINT ( 'NONE',  ( -12.36537603459249901, 1507.934286694269986, 209.0016465257290008 ) ) ;
#17467=CARTESIAN_POINT ( 'NONE',  ( -5.696033815719999893, 1448.953839979589929, 210.9996425703789953 ) ) ;
#17476=CARTESIAN_POINT ( 'NONE',  ( 9.200258835159148774, 1470.370198451841816, 213.4174792157946854 ) ) ;
#17482=CARTESIAN_POINT ( 'NONE',  ( 3.813345290629999607, 1485.053057143089973, 219.5629744241990124 ) ) ;
#17483=CARTESIAN_POINT ( 'NONE',  ( 3.909229062960000167, 1422.563626564619881, 194.1920524380990116 ) ) ;
#17485=CARTESIAN_POINT ( 'NONE',  ( -12.14468697209110104, 1448.084251977639951, 193.6129773812070027 ) ) ;
#17486=CARTESIAN_POINT ( 'NONE',  ( 5.232600787119999985, 1437.236778738189969, 228.7402956028990104 ) ) ;
#17488=CARTESIAN_POINT ( 'NONE',  ( 19.38665597314309963, 1498.811989926609840, 221.8202338665909963 ) ) ;
#17492=CARTESIAN_POINT ( 'NONE',  ( 9.820595928116450324, 1435.622055171000056, 209.3846138168819948 ) ) ;
#17493=CARTESIAN_POINT ( 'NONE',  ( -10.94672739099999959, 1491.935509946189995, 210.5292650763190068 ) ) ;
#17494=CARTESIAN_POINT ( 'NONE',  ( 8.887962835699010355, 1449.864045084309964, 203.7541360747050021 ) ) ;
#17502=CARTESIAN_POINT ( 'NONE',  ( 9.603890370815909350, 1503.574939094829915, 216.4415450440779978 ) ) ;
#17503=CARTESIAN_POINT ( 'NONE',  ( -9.918481311761176755, 1422.650748571832310, 210.6689247654111909 ) ) ;
#17506=EDGE_CURVE ( 'NONE', #55998, #94471, #52665, .T. ) ;
#17507=ORIENTED_EDGE ( 'NONE', *, *, #54487, .F. ) ;
#17514=CARTESIAN_POINT ( 'NONE',  ( -0.7790504975549988886, 1442.687250042790083, 200.2740176171789983 ) ) ;
#17518=FACE_OUTER_BOUND ( 'NONE', #1057, .T. ) ;
#17527=EDGE_LOOP ( 'NONE', ( #98526, #106148, #61048, #24416 ) ) ;
#17528=EDGE_LOOP ( 'NONE', ( #48906, #25476, #62641, #75701 ) ) ;
#17532=CARTESIAN_POINT ( 'NONE',  ( -9.655138005699368975, 1473.799620413477442, 205.6226705925480474 ) ) ;
#17534=B_SPLINE_CURVE_WITH_KNOTS ( 'NONE', 3,
 ( #72577, #47917, #40064, #22677, #30559, #56323, #56877, #74243, #31107, #23248, #13181, #64748, #98860, #31655, #90454, #72052, #98308, #106705, #13732, #48486, #82052, #39517, #108373, #12658, #91007, #81495, #4270, #82625, #65835, #73692, #14297, #57446, #29445, #91573, #14847, #49038, #83174, #6464, #106168, #63644, #97759, #21030, #55234, #21585, #89366, #64186, #46837, #80966, #55792, #38401, #29995 ),
 .UNSPECIFIED., .F., .F.,
 ( 4, 2, 2, 2, 1, 2, 2, 2, 1, 1, 1, 1, 2, 2, 2, 2, 2, 1, 1, 1, 1, 2, 2, 2, 2, 2, 1, 1, 2, 2, 4 ),
 ( 0.000000000000000000, 0.03124999999711828430, 0.06249999999423656860, 0.09374999999135485984, 0.1093749999899146230, 0.1171874999892398156, 0.1249999999885650082, 0.1874999999835806064, 0.2187499999810354201, 0.2343749999797607175, 0.2421874999790658567, 0.2460937499787189953, 0.2480468749786066129, 0.2499999999784942584, 0.3749999999675763807, 0.4374999999621191349, 0.4687499999594437194, 0.4843749999581046795, 0.4921874999573854215, 0.4960937499569785802, 0.4980468749568228715, 0.4990234374567449338, 0.4999999999566671072, 0.6249999999676451035, 0.6874999999731339351, 0.7187499999758150127, 0.7343749999771556070, 0.7421874999778810267, 0.7460937499782968052, 0.7499999999787125837, 1.000000000000000000 ),
 .UNSPECIFIED. ) ;
#17537=CARTESIAN_POINT ( 'NONE',  ( 12.00800514267580077, 1421.841763435350003, 208.7871892364869950 ) ) ;
#17541=EDGE_LOOP ( 'NONE', ( #64106, #73809, #77456, #15949 ) ) ;
#17545=CYLINDRICAL_SURFACE ( 'NONE', #49813, 1.999999999999997335 ) ;
#17549=CARTESIAN_POINT ( 'NONE',  ( 2.280398975811160245, 1423.485262736610139, 192.6506460990210314 ) ) ;
#17559=CARTESIAN_POINT ( 'NONE',  ( -3.549339293766919923, 1428.611355690149821, 200.4582084220010074 ) ) ;
#17564=CARTESIAN_POINT ( 'NONE',  ( -11.84250961054740081, 1482.176269567949930, 208.0354447653020031 ) ) ;
#17574=CARTESIAN_POINT ( 'NONE',  ( 10.86655197540000017, 1422.901418124660040, 206.8976527062889943 ) ) ;
#17577=CARTESIAN_POINT ( 'NONE',  ( -9.938748489107151585, 1448.437396663140134, 208.6016734837719753 ) ) ;
#17582=CARTESIAN_POINT ( 'NONE',  ( -10.10644227791819993, 1508.436924462359912, 218.7282801708559816 ) ) ;
#17587=CARTESIAN_POINT ( 'NONE',  ( -4.326992699989999913, 1515.158586642790169, 209.1218459619010162 ) ) ;
#17588=CARTESIAN_POINT ( 'NONE',  ( 3.550946725939999826, 1467.682858653789935, 218.4445632802489854 ) ) ;
#17594=CARTESIAN_POINT ( 'NONE',  ( 11.65588960887020065, 1480.025413490480105, 210.9188710873860089 ) ) ;
#17603=CARTESIAN_POINT ( 'NONE',  ( 12.67303841979999923, 1500.818571512490053, 210.2049276646989995 ) ) ;
#17606=CARTESIAN_POINT ( 'NONE',  ( 7.747154353170000007, 1424.045375182409998, 212.1192621507390186 ) ) ;
#17610=CARTESIAN_POINT ( 'NONE',  ( -7.113505352310000696, 1482.903954351189896, 201.0855788274590168 ) ) ;
#17613=EDGE_LOOP ( 'NONE', ( #62249, #89302, #78579, #71892 ) ) ;
#17614=CARTESIAN_POINT ( 'NONE',  ( 5.151097723079999469, 1490.744826430290004, 188.9005472705989916 ) ) ;
#17618=CARTESIAN_POINT ( 'NONE',  ( 1.870139295948670011, 1435.444322134060030, 227.4790408562990081 ) ) ;
#17621=CARTESIAN_POINT ( 'NONE',  ( -0.2993477608136759782, 1457.076524069930201, 219.7486934169020003 ) ) ;
#17624=VECTOR ( 'NONE', #102622, 1000.000000000000114 ) ;
#17625=CARTESIAN_POINT ( 'NONE',  ( 7.342390941769999735, 1424.750470890219958, 212.5422998803489918 ) ) ;
#17626=CARTESIAN_POINT ( 'NONE',  ( -9.299436816969999242, 1446.922293007090275, 190.6945112479990030 ) ) ;
#17629=AXIS2_PLACEMENT_3D ( 'NONE', #85383, #8678, #108400 ) ;
#17639=CARTESIAN_POINT ( 'NONE',  ( 8.547640172370703837, 1500.581726597095212, 201.5589322185294634 ) ) ;
#17643=CARTESIAN_POINT ( 'NONE',  ( -0.6340257723134260504, 1475.639747297089798, 197.6856915023410011 ) ) ;
#17644=EDGE_CURVE ( 'NONE', #5861, #20921, #30389, .T. ) ;
#17656=ORIENTED_EDGE ( 'NONE', *, *, #44754, .F. ) ;
#17658=DIRECTION ( 'NONE',  ( 0.9999994573234139983, 0.000000000000000000, -0.001041802705659123675 ) ) ;
#17675=CARTESIAN_POINT ( 'NONE',  ( 4.253777714910000007, 1442.471859903390168, 216.9083338397390150 ) ) ;
#17684=LINE ( 'NONE', #86579, #19831 ) ;
#17689=CARTESIAN_POINT ( 'NONE',  ( -3.512136796220000523, 1429.445925473590023, 201.4575808623890225 ) ) ;
#17695=CARTESIAN_POINT ( 'NONE',  ( 5.009886284249999377, 1430.069699660889910, 217.1776678749689893 ) ) ;
#17704=B_SPLINE_SURFACE_WITH_KNOTS ( 'NONE', 5, 5, ( 
 ( #70246, #86994, #62957, #70796, #62383, #97068 ),
 ( #27104, #1922, #52867, #104909, #19789, #11413 ),
 ( #71905, #78604, #79723, #53990, #97612, #28197 ),
 ( #96509, #54538, #95954, #88672, #88124, #63492 ),
 ( #19214, #20882, #45581, #53417, #3030, #105463 ),
 ( #11950, #106021, #36059, #46131, #29296, #87568 ) ),
 .UNSPECIFIED., .F., .F., .F.,
 ( 6, 6 ),
 ( 6, 6 ),
 ( 14.17748175450000048, 22.88732747950000146 ),
 ( 0.9649189546150001018, 2.000000000000000000 ),
 .UNSPECIFIED. ) ;
#17712=FACE_OUTER_BOUND ( 'NONE', #17904, .T. ) ;
#17714=CARTESIAN_POINT ( 'NONE',  ( -3.609215388063503394, 1508.124843871699341, 220.7461715565221994 ) ) ;
#17718=CARTESIAN_POINT ( 'NONE',  ( 9265.100134287571564, 5182.654794667087117, -1184.579948005114375 ) ) ;
#17720=CARTESIAN_POINT ( 'NONE',  ( -11.47238377808170107, 1419.373738041100069, 197.8436817076510010 ) ) ;
#17721=CARTESIAN_POINT ( 'NONE',  ( 4.329448791022380227, 1515.064792310580060, 207.3461553972610147 ) ) ;
#17723=EDGE_LOOP ( 'NONE', ( #22195, #15193, #47535, #62741 ) ) ;
#17728=CARTESIAN_POINT ( 'NONE',  ( -10.49919538747700010, 1479.838970662580095, 209.4913417018410087 ) ) ;
#17729=B_SPLINE_SURFACE_WITH_KNOTS ( 'NONE', 5, 5, ( 
 ( #80071, #20153, #36412, #12305, #28013, #80629 ),
 ( #96328, #96884, #3392, #19606, #53808, #10678 ),
 ( #11235, #2839, #88481, #45935, #38610, #45397 ),
 ( #71155, #37521, #29120, #106916, #63305, #30205 ),
 ( #97425, #3944, #38071, #106375, #29663, #64396 ),
 ( #63848, #97960, #21230, #55440, #89569, #98517 ),
 ( #12859, #72789, #81165, #4480, #21785, #87383 ),
 ( #44845, #78998, #40268, #48695, #83925, #67151 ),
 ( #100713, #39158, #49244, #41386, #48138, #56537 ) ),
 .UNSPECIFIED., .F., .F., .F.,
 ( 6, 3, 6 ),
 ( 6, 6 ),
 ( 3.197141790549999918, 7.200146509529999683, 12.49638257910000050 ),
 ( 0.000000000000000000, 2.000000000000000000 ),
 .UNSPECIFIED. ) ;
#17732=CARTESIAN_POINT ( 'NONE',  ( -4.633397098031169392, 1377.913060387289988, 204.2654103466966831 ) ) ;
#17739=ORIENTED_EDGE ( 'NONE', *, *, #106847, .F. ) ;
#17751=CARTESIAN_POINT ( 'NONE',  ( 8.638387969371279951, 1437.275665663040172, 209.5904139818730130 ) ) ;
#17756=CARTESIAN_POINT ( 'NONE',  ( 0.4136971850115839788, 1486.226569062650242, 197.2199659705369754 ) ) ;
#17759=CARTESIAN_POINT ( 'NONE',  ( -10.08143941300950175, 1423.969704056519731, 204.5062346435900054 ) ) ;
#17763=CARTESIAN_POINT ( 'NONE',  ( -3.116127822624859878, 1509.034536885679927, 213.6092057278939933 ) ) ;
#17764=CARTESIAN_POINT ( 'NONE',  ( -4.389948488746259869, 1481.757683799150072, 231.0981567811180071 ) ) ;
#17768=CARTESIAN_POINT ( 'NONE',  ( -8.773919776719999675, 1470.032071067190145, 190.9916890139989789 ) ) ;
#17770=CARTESIAN_POINT ( 'NONE',  ( 2.330134126739547451, 1515.219201591195088, 213.4472514034076767 ) ) ;
#17783=CARTESIAN_POINT ( 'NONE',  ( -8.474551757659998685, 1423.809698281529791, 209.1924171156409784 ) ) ;
#17788=CARTESIAN_POINT ( 'NONE',  ( 7.494055247967449596, 1426.002717090129863, 212.3343695544420200 ) ) ;
#17797=CARTESIAN_POINT ( 'NONE',  ( -1.571492423569999852, 1455.857433419590052, 215.6548381990889709 ) ) ;
#17798=CARTESIAN_POINT ( 'NONE',  ( 4.865303301610000908, 1425.588844564269948, 210.1313439721089935 ) ) ;
#17806=VERTEX_POINT ( 'NONE', #90843 ) ;
#17826=CARTESIAN_POINT ( 'NONE',  ( -4.963083875006099710, 1508.551704408389924, 211.9655763852440202 ) ) ;
#17828=CARTESIAN_POINT ( 'NONE',  ( 7.435908444379999871, 1422.989459805909974, 195.6132688577989711 ) ) ;
#17830=B_SPLINE_SURFACE_WITH_KNOTS ( 'NONE', 5, 5, ( 
 ( #8094, #34411, #60748, #109474, #41707, #94871 ),
 ( #83705, #24342, #68583, #66934, #34956, #6999 ),
 ( #42262, #7553, #41158, #15927, #102688, #76410 ),
 ( #50128, #25983, #84257, #75867, #110017, #69140 ),
 ( #43378, #33293, #67486, #101589, #17577, #85916 ),
 ( #110564, #68041, #17015, #8641, #42817, #9220 ),
 ( #77527, #20355, #54015, #62407, #88145, #106041 ),
 ( #70266, #86464, #29318, #37179, #19809, #103825 ),
 ( #3053, #1943, #95429, #36623, #54560, #11433 ) ),
 .UNSPECIFIED., .F., .F., .F.,
 ( 6, 3, 6 ),
 ( 6, 6 ),
 ( 3.058261753925569870, 5.256832519259999614, 7.455370546767019491 ),
 ( -0.0004137009344281229587, 2.000000000000000000 ),
 .UNSPECIFIED. ) ;
#17831=B_SPLINE_CURVE_WITH_KNOTS ( 'NONE', 3,
 ( #10632, #97380, #71118, #87336, #72214, #5533, #57618, #82234, #107428, #30724, #6079, #38034, #23424 ),
 .UNSPECIFIED., .F., .F.,
 ( 4, 2, 1, 1, 1, 2, 2, 4 ),
 ( 0.000000000000000000, 0.2500000000001524336, 0.3750000000002216560, 0.4375000000002614020, 0.4687500000002742806, 0.4843750000002768341, 0.5000000000002794431, 1.000000000000000000 ),
 .UNSPECIFIED. ) ;
#17837=CARTESIAN_POINT ( 'NONE',  ( -15.87405076837314333, 1420.081557989787143, 210.7260919225635405 ) ) ;
#17842=CARTESIAN_POINT ( 'NONE',  ( 4.926620861452232880, 1485.064373513001783, 218.6596911836547861 ) ) ;
#17847=CARTESIAN_POINT ( 'NONE',  ( -0.4768852844176069694, 1420.937210074157747, 193.7246766131215452 ) ) ;
#17858=EDGE_CURVE ( 'NONE', #100027, #65578, #32417, .T. ) ;
#17859=CARTESIAN_POINT ( 'NONE',  ( 20.15123768920399883, 1431.269255322170011, 215.0996795108299864 ) ) ;
#17861=CARTESIAN_POINT ( 'NONE',  ( 10.48742109869949957, 1419.983217468429984, 196.1364727454310071 ) ) ;
#17868=CARTESIAN_POINT ( 'NONE',  ( -7.982037141949999359, 1424.874072662569915, 210.5243721551090061 ) ) ;
#17869=CARTESIAN_POINT ( 'NONE',  ( -3.269259737218870310, 1476.740802116999930, 199.2818558394819775 ) ) ;
#17872=CARTESIAN_POINT ( 'NONE',  ( -5.586163095751780716, 1491.245996555280044, 185.8699225654929990 ) ) ;
#17875=CARTESIAN_POINT ( 'NONE',  ( -20.80698145192160098, 1418.268157419850013, 208.6562635851959726 ) ) ;
#17877=CARTESIAN_POINT ( 'NONE',  ( 3.919202604670000145, 1440.900018029090006, 218.2279973031590146 ) ) ;
#17880=DIRECTION ( 'NONE',  ( 0.4794255386042031719, 0.000000000000000000, 0.8775825618903726477 ) ) ;
#17883=CARTESIAN_POINT ( 'NONE',  ( 5.140114172436319961, 1436.845577873409866, 228.7442477189930230 ) ) ;
#17904=EDGE_LOOP ( 'NONE', ( #68917, #109040, #30086, #72378 ) ) ;
#17905=CARTESIAN_POINT ( 'NONE',  ( 7.323840960111850151, 1466.289181860749977, 215.8067017296629899 ) ) ;
#17906=ORIENTED_EDGE ( 'NONE', *, *, #104887, .T. ) ;
#17907=CARTESIAN_POINT ( 'NONE',  ( 6.020918722830000291, 1451.049614457190046, 209.7855091624759893 ) ) ;
#17909=CARTESIAN_POINT ( 'NONE',  ( -6.173337796650000264, 1494.737438040389861, 198.8902207915990061 ) ) ;
#17925=EDGE_CURVE ( 'NONE', #106043, #87765, #48500, .T. ) ;
#17940=CARTESIAN_POINT ( 'NONE',  ( 4.672324531150159999, 1508.551704408389924, 212.8263036817449745 ) ) ;
#17944=CARTESIAN_POINT ( 'NONE',  ( 10.44641616108000015, 1460.893522529900110, 207.9938650532610041 ) ) ;
#17953=CARTESIAN_POINT ( 'NONE',  ( -15.31509580213619870, 1508.249370024519976, 209.5650669845969958 ) ) ;
#17958=CARTESIAN_POINT ( 'NONE',  ( 10.56406725279730097, 1452.658225117510028, 209.7434485084090170 ) ) ;
#17974=CARTESIAN_POINT ( 'NONE',  ( -7.987427797640509475, 1490.123333955630414, 216.6223879589213936 ) ) ;
#17976=EDGE_CURVE ( 'NONE', #58087, #10311, #80410, .T. ) ;
#17978=CARTESIAN_POINT ( 'NONE',  ( 9.211627749346281036, 1450.348376029699921, 208.8206138348359957 ) ) ;
#17979=CARTESIAN_POINT ( 'NONE',  ( -12.58738889680580186, 1502.045147876100145, 211.1486701620410145 ) ) ;
#17980=CARTESIAN_POINT ( 'NONE',  ( 6.983043359149999851, 1493.573093954689966, 217.9908564108290250 ) ) ;
#17983=CARTESIAN_POINT ( 'NONE',  ( -3.672024168570000136, 1497.313529941189927, 198.4698546893989715 ) ) ;
#17986=AXIS2_PLACEMENT_3D ( 'NONE', #84239, #13706, #7538 ) ;
#17989=ORIENTED_EDGE ( 'NONE', *, *, #103560, .T. ) ;
#17996=CARTESIAN_POINT ( 'NONE',  ( -11.26215388574009957, 1500.310609260709953, 210.9023932557140029 ) ) ;
#18001=EDGE_CURVE ( 'NONE', #54902, #24288, #85754, .T. ) ;
#18003=CARTESIAN_POINT ( 'NONE',  ( 20.08180131570000171, 1474.154670883989866, 211.0997262866790152 ) ) ;
#18004=CARTESIAN_POINT ( 'NONE',  ( -10.83132596424780125, 1461.840861733669954, 211.0446618225340103 ) ) ;
#18005=CARTESIAN_POINT ( 'NONE',  ( -18.22821675530000007, 1443.229620277490085, 204.5519556382290034 ) ) ;
#18011=CARTESIAN_POINT ( 'NONE',  ( -10.51573792566800059, 1480.737017572810146, 208.3487723898410025 ) ) ;
#18026=CARTESIAN_POINT ( 'NONE',  ( -3.578645720892979831, 1485.309967107140210, 197.7694655723200015 ) ) ;
#18027=B_SPLINE_SURFACE_WITH_KNOTS ( 'NONE', 5, 5, ( 
 ( #50410, #7823, #104099, #86192, #1661, #79463, #10039, #43649, #96256 ),
 ( #69982, #94581, #78920, #18969, #104651, #43100, #44770, #44209, #86748 ),
 ( #52059, #17299, #27948, #68874, #78352, #103539, #10598, #52610, #87306 ),
 ( #94035, #69426, #2226, #36342, #102430, #9484, #34684, #35800, #26274 ),
 ( #27389, #70533, #62129, #19531, #53737, #51494, #26843, #61568, #77802 ),
 ( #53164, #2774, #45325, #87874, #95153, #61031, #11164, #68322, #95703 ),
 ( #102976, #25713, #59914, #35239, #85626, #8926, #77260, #1111, #559 ),
 ( #60463, #17859, #18412, #34868, #75239, #42174, #85258, #76325, #16930 ),
 ( #43288, #94211, #102596, #9121, #77436, #34319, #24783, #41623, #92558 ),
 ( #33207, #15828, #25897, #51684, #41062, #17486, #67397, #26458, #69056 ),
 ( #50031, #7461, #93647, #84160, #15292, #110475, #8008, #16383, #60095 ),
 ( #76886, #103157, #75777, #735, #102059, #195, #109930, #101495, #24249 ),
 ( #58985, #51131, #92022, #42727, #59535, #85823, #93112, #109389, #58430 ),
 ( #33753, #25341, #32666, #66844, #50580, #84708, #8555, #67950, #68497 ),
 ( #49485, #83608, #6905, #100954, #37079, #28689, #35988, #1853, #2962 ),
 ( #71283, #52797, #19723, #86928, #27033, #87499, #11344, #88605, #94777 ),
 ( #62893, #70176, #104287, #105396, #69612, #97003, #10219, #53924, #44397 ),
 ( #10789, #45516, #11887, #18054, #96444, #103734, #80192, #52249, #36531 ),
 ( #20266, #61222, #35425, #43832, #54467, #27576, #78539, #61761, #79658 ),
 ( #46059, #44959, #3510, #95887, #37634, #71839, #19147, #105957, #9661 ),
 ( #53354, #79107, #60653, #77978, #2414, #70728, #104840, #28128, #86375 ),
 ( #62319, #95336, #1286, #18597, #88059, #55557, #108132, #29235, #38179 ),
 ( #89682, #57216, #31425, #12964, #65052, #13506, #14064, #65607, #22447 ),
 ( #47147, #99165, #107587, #99719, #38722, #46614, #21896, #89138, #81272 ),
 ( #30873, #41902, #80744, #39281, #30324, #76057, #56647, #73456, #82396 ),
 ( #5693, #4589, #48253, #7739, #72897, #91342, #90781, #39837, #107037 ),
 ( #72359, #64513, #21350, #74000, #16122, #23012, #50327, #84453, #63964 ),
 ( #106491, #20813, #81822, #63424, #12424, #4053, #98628, #56094, #97542 ),
 ( #55011, #47694, #29776, #98079, #90221, #5125, #86656, #69335, #25629 ),
 ( #26182, #60937, #27305, #33474, #35151, #8281, #18882, #101783, #86109 ),
 ( #1571, #42445, #84986, #93394, #44123, #51403, #59821, #85535, #18333 ),
 ( #44680, #95066, #10508, #87218, #52524, #60371, #68785, #9951, #35704 ),
 ( #8830, #76603, #69893, #43565, #77172, #25073, #51968, #78258, #43015 ),
 ( #475, #110755, #104008, #61486, #67676, #93941, #95615, #110200, #34046 ),
 ( #17207, #53080, #59276, #34599, #103443, #94492, #16659, #50857, #26748 ),
 ( #102885, #68236, #77716, #102346, #17764, #9403, #1027, #27863, #105127 ),
 ( #80478, #89966, #19445, #88874, #79928, #13240, #72109, #12159, #21089 ),
 ( #55292, #62616, #63700, #55844, #28418, #106762, #46349, #97810, #96733 ),
 ( #11069, #20004, #71006, #3796, #30053, #29507, #37927, #89422, #2692 ),
 ( #45238, #70448, #20540, #106223, #62043, #96169, #3244, #54198, #12712 ),
 ( #37370, #53643, #79376, #87787, #45795, #36816, #21639, #46896, #81020 ),
 ( #36259, #88323, #104568, #105692, #4329, #38459, #11618, #72633, #54744 ),
 ( #78825, #71571, #28975, #64244, #63163, #98366, #97264, #2136, #31708 ),
 ( #101102, #73177, #48538, #23845, #15445, #22732, #99454, #100564, #56382 ),
 ( #39571, #6514, #73744, #13789, #74295, #108984, #75394, #81553, #83224 ),
 ( #66992, #47973, #65894, #5412, #82113, #100011, #92174, #58036, #7067 ),
 ( #107321, #5967, #57496, #56934, #92716, #32269, #58586, #24402, #49636 ),
 ( #40112, #83773, #41223, #23301, #91063, #107868, #109533, #91621, #14347 ),
 ( #14897, #32807, #82676, #47430, #108426, #31156, #4855, #39000, #30616 ),
 ( #64803, #98912, #90514, #40667, #65346, #22184, #49088, #74840, #66451 ),
 ( #894, #94933, #9276, #15992, #76474, #51839, #94357, #18205, #25498 ) ),
 .UNSPECIFIED., .F., .F., .F.,
 ( 6, 3, 3, 3, 3, 3, 3, 3, 3, 3, 3, 3, 3, 3, 3, 3, 6 ),
 ( 6, 3, 6 ),
 ( 0.000000000000000000, 28.69702819429999963, 61.04778752440000034, 93.62768910810000023, 123.7336603250000024, 156.1762685979999787, 187.3272846180000215, 220.4669312460000015, 237.3878297990000021, 254.2938300590000154, 289.2398204710000300, 325.3030936050000150, 360.8626869010000178, 395.8828220460000011, 432.6128460950000090, 468.8934854820000169, 502.1482307969999965 ),
 ( -0.0001008871253083600000, 2.001700839520000219, 3.002551259279999663 ),
 .UNSPECIFIED. ) ;
#18029=CARTESIAN_POINT ( 'NONE',  ( -4.771756610380000652, 1496.505580869889855, 219.3152549879989692 ) ) ;
#18033=CARTESIAN_POINT ( 'NONE',  ( -11.65744291596249838, 1508.186430388969939, 208.3002178115879985 ) ) ;
#18050=B_SPLINE_CURVE_WITH_KNOTS ( 'NONE', 3,
 ( #49037, #66395, #56876, #83172, #98859, #22123, #7008, #41166, #108923, #31654, #32215, #73691, #91006, #90453, #14296, #82051, #5916, #6463, #100515, #40612, #23793, #99952, #5357, #92118, #65834, #23247, #49583, #107817, #74783, #66941, #48485, #24349, #58533, #13180, #47368, #81494, #68049, #33858, #86887, #102158 ),
 .UNSPECIFIED., .F., .F.,
 ( 4, 3, 3, 3, 3, 3, 3, 3, 3, 3, 3, 3, 3, 4 ),
 ( -7.530765448250459571, -7.506223803491129942, -7.257045730312249532, -6.983326012374050151, -6.698284398290460295, -6.381132500363879245, -5.928019582097629581, -5.598363948206119822, -5.308105043320740180, -5.156242663369150492, -4.738290659457769394, -4.262467497528719562, -3.657517831626029725, -3.085444082959999612 ),
 .UNSPECIFIED. ) ;
#18051=FACE_OUTER_BOUND ( 'NONE', #21061, .T. ) ;
#18052=CARTESIAN_POINT ( 'NONE',  ( 10.43532605497630072, 1480.514957649700136, 207.6513091103709883 ) ) ;
#18054=CARTESIAN_POINT ( 'NONE',  ( 18.98377022170240025, 1454.978415555989841, 200.5246066841559696 ) ) ;
#18056=CARTESIAN_POINT ( 'NONE',  ( -21.46486174371069922, 1504.440211353449740, 215.6677629390230209 ) ) ;
#18060=CARTESIAN_POINT ( 'NONE',  ( -4.992349863779999453, 1391.620913471789891, 203.7504116504090064 ) ) ;
#18062=CARTESIAN_POINT ( 'NONE',  ( -10.81618613060000023, 1491.239992459889891, 211.1797723353990079 ) ) ;
#18063=CARTESIAN_POINT ( 'NONE',  ( 7.173571134148669870, 1448.589511863430062, 201.7444442637240059 ) ) ;
#18071=CARTESIAN_POINT ( 'NONE',  ( 5.430409578133730264, 1505.407880561079992, 219.8354462761509751 ) ) ;
#18080=CARTESIAN_POINT ( 'NONE',  ( -10.36221610374189872, 1448.183279349199893, 208.6963155564749854 ) ) ;
#18081=CARTESIAN_POINT ( 'NONE',  ( -4.491293115488388388, 1508.884207226183435, 211.6097811125350177 ) ) ;
#18087=CARTESIAN_POINT ( 'NONE',  ( 1.939364658240000150, 1467.845018752989972, 219.0547953187090116 ) ) ;
#18091=CARTESIAN_POINT ( 'NONE',  ( -9.996465492614740711, 1423.286309259070094, 207.3024158817219984 ) ) ;
#18096=CARTESIAN_POINT ( 'NONE',  ( -0.8603290292595530131, 1431.922339058240141, 200.7526126593139963 ) ) ;
#18097=ORIENTED_EDGE ( 'NONE', *, *, #95424, .T. ) ;
#18103=CARTESIAN_POINT ( 'NONE',  ( 10.52285531690000120, 1461.267078505790096, 209.0122360621460018 ) ) ;
#18105=CARTESIAN_POINT ( 'NONE',  ( 12.45034049356619832, 1421.619540909540092, 207.5029415923690124 ) ) ;
#18108=CARTESIAN_POINT ( 'NONE',  ( 8.637056729921679832, 1437.983744640310078, 209.9529184353999938 ) ) ;
#18124=CARTESIAN_POINT ( 'NONE',  ( -5.292247061280000331, 1391.913060387289988, 209.1218459616989946 ) ) ;
#18128=CARTESIAN_POINT ( 'NONE',  ( -2.681276382835120042, 1429.097449907909777, 200.1427365742090103 ) ) ;
#18132=CARTESIAN_POINT ( 'NONE',  ( -11.82493131255569985, 1482.231903543040062, 207.8362869629800116 ) ) ;
#18138=EDGE_CURVE ( 'NONE', #21803, #104898, #41730, .T. ) ;
#18139=CARTESIAN_POINT ( 'NONE',  ( 10.62827625601449988, 1490.977054330010105, 211.9199658921150160 ) ) ;
#18148=CARTESIAN_POINT ( 'NONE',  ( -8.840129632021261230, 1448.960675403350024, 211.5120822850410036 ) ) ;
#18158=CARTESIAN_POINT ( 'NONE',  ( -1.636741614903409969, 1469.777368438049962, 219.0527109355280118 ) ) ;
#18164=CARTESIAN_POINT ( 'NONE',  ( 11.13173720219280050, 1480.405744213160006, 211.3599368507180145 ) ) ;
#18165=CARTESIAN_POINT ( 'NONE',  ( -0.5193063452810020575, 1507.010169186189842, 221.5509792533989923 ) ) ;
#18167=ORIENTED_EDGE ( 'NONE', *, *, #481, .T. ) ;
#18173=CARTESIAN_POINT ( 'NONE',  ( 12.60564844770000015, 1500.992646453189991, 210.8169608434889994 ) ) ;
#18175=EDGE_CURVE ( 'NONE', #3936, #74194, #37778, .T. ) ;
#18176=CARTESIAN_POINT ( 'NONE',  ( 7.956617570819999763, 1426.823372744059952, 211.7778627466090029 ) ) ;
#18181=CARTESIAN_POINT ( 'NONE',  ( -7.932780634030001110, 1482.621353729790144, 201.9116440055690020 ) ) ;
#18185=ORIENTED_EDGE ( 'NONE', *, *, #96543, .F. ) ;
#18187=CARTESIAN_POINT ( 'NONE',  ( -16.71982381703620035, 1484.422990366600288, 222.3758235082320027 ) ) ;
#18188=ORIENTED_EDGE ( 'NONE', *, *, #110319, .F. ) ;
#18190=CARTESIAN_POINT ( 'NONE',  ( -2.602924848259999813, 1495.483236843290115, 217.1248042506690297 ) ) ;
#18193=CARTESIAN_POINT ( 'NONE',  ( -9.968644151297580080, 1439.097532313579904, 209.3205140116839971 ) ) ;
#18196=CARTESIAN_POINT ( 'NONE',  ( 7.505459564510000625, 1425.357945906760051, 212.2350828798089992 ) ) ;
#18197=CARTESIAN_POINT ( 'NONE',  ( 5.076283890730000081, 1469.790178736790040, 187.8425608535989966 ) ) ;
#18205=CARTESIAN_POINT ( 'NONE',  ( -21.63026377219999929, 1508.312050283890130, 209.5914177110290098 ) ) ;
#18207=CARTESIAN_POINT ( 'NONE',  ( 7.544486580690446864, 1500.279846028723568, 200.5799775095794075 ) ) ;
#18210=CARTESIAN_POINT ( 'NONE',  ( 1.195572441903639982, 1476.044226966599808, 197.7073300112460004 ) ) ;
#18240=ORIENTED_EDGE ( 'NONE', *, *, #3551, .F. ) ;
#18243=CARTESIAN_POINT ( 'NONE',  ( -8.228435909236443635, 1441.487949711303372, 203.2737885189420410 ) ) ;
#18272=ORIENTED_EDGE ( 'NONE', *, *, #14255, .T. ) ;
#18278=CARTESIAN_POINT ( 'NONE',  ( -21.59687142900000012, 1507.523380033690046, 209.4572543540780032 ) ) ;
#18280=CARTESIAN_POINT ( 'NONE',  ( 2.991069600740460466, 1424.175520158889867, 191.4083219421100353 ) ) ;
#18282=CARTESIAN_POINT ( 'NONE',  ( -3.035119290295845929, 1377.913060387289988, 210.7799391869605188 ) ) ;
#18285=CARTESIAN_POINT ( 'NONE',  ( -7.344230725084723410, 1458.212826010420713, 215.2418586630906532 ) ) ;
#18289=CARTESIAN_POINT ( 'NONE',  ( -10.92886345369909940, 1418.002833451510014, 197.9448744300869976 ) ) ;
#18292=ORIENTED_EDGE ( 'NONE', *, *, #89334, .T. ) ;
#18305=CARTESIAN_POINT ( 'NONE',  ( -5.149250441021638203, 1391.888183122331156, 214.5740113081126310 ) ) ;
#18312=CARTESIAN_POINT ( 'NONE',  ( -14.87799178844600156, 1417.019184689190070, 213.1221934129589783 ) ) ;
#18314=ORIENTED_EDGE ( 'NONE', *, *, #15321, .F. ) ;
#18320=CARTESIAN_POINT ( 'NONE',  ( 9.825411767019899045, 1435.537689025190048, 209.1855920904920083 ) ) ;
#18327=CARTESIAN_POINT ( 'NONE',  ( -9.190602985553210758, 1449.883023889459992, 209.4828535419830189 ) ) ;
#18328=CARTESIAN_POINT ( 'NONE',  ( -12.46654139771550085, 1422.643769205189983, 203.9843212440389948 ) ) ;
#18333=CARTESIAN_POINT ( 'NONE',  ( 4.667614565920000125, 1472.762121965489769, 187.6119789488990079 ) ) ;
#18340=CARTESIAN_POINT ( 'NONE',  ( -1.936437027941079858, 1420.638707705209754, 193.8409875628919963 ) ) ;
#18347=CARTESIAN_POINT ( 'NONE',  ( -9.199049879260000395, 1422.949100153850168, 210.5804414222690184 ) ) ;
#18352=CARTESIAN_POINT ( 'NONE',  ( 7.526870069911640648, 1425.474419429210002, 212.1962186843350082 ) ) ;
#18353=CARTESIAN_POINT ( 'NONE',  ( 0.1490614901714290008, 1496.163810114490161, 221.4655199671470029 ) ) ;
#18354=VERTEX_POINT ( 'NONE', #76530 ) ;
#18356=CARTESIAN_POINT ( 'NONE',  ( -10.93631254607359971, 1492.700895685820115, 207.3057419371699837 ) ) ;
#18360=CARTESIAN_POINT ( 'NONE',  ( 3.696672296620000076, 1460.253338437389857, 228.3281616586990026 ) ) ;
#18361=CARTESIAN_POINT ( 'NONE',  ( -8.666962939886769135, 1439.175798852059870, 207.1921834104900029 ) ) ;
#18362=VERTEX_POINT ( 'NONE', #83280 ) ;
#18368=VERTEX_POINT ( 'NONE', #101711 ) ;
#18380=ORIENTED_EDGE ( 'NONE', *, *, #26320, .F. ) ;
#18385=CARTESIAN_POINT ( 'NONE',  ( 2.487923763832299962, 1508.731372606449895, 204.5668970731580032 ) ) ;
#18388=CARTESIAN_POINT ( 'NONE',  ( 12.44780704128189974, 1501.268281525590055, 211.7240718234590133 ) ) ;
#18402=CARTESIAN_POINT ( 'NONE',  ( -1.033263135950000189, 1463.032196151989865, 228.8909791214989866 ) ) ;
#18405=CARTESIAN_POINT ( 'NONE',  ( -0.3700193229654308857, 1420.964624414496029, 193.7214914399045256 ) ) ;
#18406=CARTESIAN_POINT ( 'NONE',  ( -4.329177920710369776, 1515.075136430330076, 207.6418469693050213 ) ) ;
#18412=CARTESIAN_POINT ( 'NONE',  ( 20.19719966420300139, 1431.660555912299969, 215.0136818726180081 ) ) ;
#18413=CARTESIAN_POINT ( 'NONE',  ( 10.88623464157270071, 1425.216911896579859, 199.6949144308769917 ) ) ;
#18414=CARTESIAN_POINT ( 'NONE',  ( 10.62765097360019872, 1462.208136432790070, 211.9187849626219702 ) ) ;
#18419=CARTESIAN_POINT ( 'NONE',  ( -16.87913774836607672, 1420.004850516591659, 207.9502230898332016 ) ) ;
#18421=CARTESIAN_POINT ( 'NONE',  ( -1.842963430059999963, 1515.219201257890063, 204.7964405181290033 ) ) ;
#18422=CARTESIAN_POINT ( 'NONE',  ( 0.5708672412673110319, 1460.784242060219867, 230.4191149082050174 ) ) ;
#18424=CARTESIAN_POINT ( 'NONE',  ( -9.200421138165051360, 1422.937291722789951, 210.7384568321920142 ) ) ;
#18426=CARTESIAN_POINT ( 'NONE',  ( 3.196982321300000152, 1441.723154499190059, 217.7614377107290125 ) ) ;
#18427=ORIENTED_EDGE ( 'NONE', *, *, #55358, .T. ) ;
#18433=CARTESIAN_POINT ( 'NONE',  ( -2.195050156180049949, 1508.551704408389924, 220.0605044532859722 ) ) ;
#18440=CARTESIAN_POINT ( 'NONE',  ( -3.273236734419999738, 1432.101391978590073, 216.8815162293089713 ) ) ;
#18442=CARTESIAN_POINT ( 'NONE',  ( 1.842963333050209318, 1515.193466656063265, 213.4479253432561450 ) ) ;
#18449=CARTESIAN_POINT ( 'NONE',  ( 12.06590886230689996, 1491.397659232809929, 206.8029289098089691 ) ) ;
#18450=CARTESIAN_POINT ( 'NONE',  ( 0.000000000000000000, 1412.913060387329779, 209.1218459616989946 ) ) ;
#18455=CARTESIAN_POINT ( 'NONE',  ( -14.35646903299999799, 1420.584115152450067, 213.7701001417389932 ) ) ;
#18457=CARTESIAN_POINT ( 'NONE',  ( -6.072056330729999729, 1495.887419368989868, 199.6590240909889928 ) ) ;
#18460=CARTESIAN_POINT ( 'NONE',  ( 11.76730872650090021, 1427.477307142819882, 208.8591088289190054 ) ) ;
#18463=CARTESIAN_POINT ( 'NONE',  ( 3.442292827050000170, 1445.232941965290138, 200.8115267138090019 ) ) ;
#18466=CARTESIAN_POINT ( 'NONE',  ( -13.24484260582790185, 1487.711350369650290, 193.0573247253030047 ) ) ;
#18472=CARTESIAN_POINT ( 'NONE',  ( -3.812371247207599900, 1428.459941768050157, 200.5740418269730014 ) ) ;
#18476=ORIENTED_EDGE ( 'NONE', *, *, #34318, .T. ) ;
#18491=CARTESIAN_POINT ( 'NONE',  ( -4.994708980640000462, 1391.711004509789973, 214.5419497225390160 ) ) ;
#18495=CARTESIAN_POINT ( 'NONE',  ( 10.06105783719169899, 1461.204106559300044, 207.9595875702549961 ) ) ;
#18499=CARTESIAN_POINT ( 'NONE',  ( 8.793327190495521251, 1451.709117791070184, 212.0827695763929910 ) ) ;
#18500=CARTESIAN_POINT ( 'NONE',  ( 8.853113012480001487, 1424.852003149989969, 195.9493848808990037 ) ) ;
#18518=CARTESIAN_POINT ( 'NONE',  ( -6.495308355903510744, 1508.529747571519920, 219.5985094923219947 ) ) ;
#18521=CARTESIAN_POINT ( 'NONE',  ( -5.500484314761993510, 1489.299785632448902, 218.6043133970500776 ) ) ;
#18525=CARTESIAN_POINT ( 'NONE',  ( -6.256968529720000838, 1474.711004521489940, 200.7308274939090040 ) ) ;
#18526=EDGE_CURVE ( 'NONE', #21788, #73262, #71069, .T. ) ;
#18527=CARTESIAN_POINT ( 'NONE',  ( -2.280747111621419965, 1421.889025025900082, 193.3469174479820083 ) ) ;
#18529=VECTOR ( 'NONE', #71427, 1000.000000000000000 ) ;
#18530=DIRECTION ( 'NONE',  ( 0.6480245870892075155, -1.644245901462725924E-32, -0.7616194158028418704 ) ) ;
#18531=CARTESIAN_POINT ( 'NONE',  ( -21.23742229959999861, 1505.497921528590041, 209.2995344244330056 ) ) ;
#18532=CARTESIAN_POINT ( 'NONE',  ( 10.86930439285440109, 1469.920656080350000, 205.9146108117720075 ) ) ;
#18535=CARTESIAN_POINT ( 'NONE',  ( -7.238531764446769934, 1498.497943084040116, 213.6891861245020152 ) ) ;
#18536=ORIENTED_EDGE ( 'NONE', *, *, #47348, .F. ) ;
#18542=CARTESIAN_POINT ( 'NONE',  ( 5.597778194180000888, 1506.679269386989972, 219.3685102149989916 ) ) ;
#18543=CARTESIAN_POINT ( 'NONE',  ( -14.00462132320000030, 1415.677402202029953, 214.2425697179989754 ) ) ;
#18544=CARTESIAN_POINT ( 'NONE',  ( -11.25901873334290038, 1500.172003390719965, 210.8567363214919794 ) ) ;
#18546=CARTESIAN_POINT ( 'NONE',  ( -15.84810074378578726, 1415.892833117942246, 209.7228954066766846 ) ) ;
#18548=CARTESIAN_POINT ( 'NONE',  ( -16.31348683090000051, 1416.654170080089898, 208.8366974938609815 ) ) ;
#18556=CARTESIAN_POINT ( 'NONE',  ( -11.18808235593009925, 1482.416383379920035, 206.6602392150250296 ) ) ;
#18567=CARTESIAN_POINT ( 'NONE',  ( -15.42622997279999986, 1414.667236775670062, 209.1420281344999808 ) ) ;
#18571=CARTESIAN_POINT ( 'NONE',  ( 1.914156610164409855, 1431.087920293139859, 199.8421651263110164 ) ) ;
#18579=CARTESIAN_POINT ( 'NONE',  ( -11.60577372236650007, 1481.108615670409790, 211.3960606566309934 ) ) ;
#18589=CARTESIAN_POINT ( 'NONE',  ( 2.175409717514719593E-31, 1397.551704408390151, 209.1218459616989946 ) ) ;
#18593=CARTESIAN_POINT ( 'NONE',  ( 4.644142782429999450, 1485.095378571789979, 218.9446188854689979 ) ) ;
#18595=CARTESIAN_POINT ( 'NONE',  ( 5.161277829439999465, 1424.205378812969911, 193.2953232350990049 ) ) ;
#18597=CARTESIAN_POINT ( 'NONE',  ( 0.7745446704201689458, 1461.969662288189966, 230.4743262828090167 ) ) ;
#18599=CARTESIAN_POINT ( 'NONE',  ( -9.966728093320000426, 1439.480327435690015, 208.4309914835989730 ) ) ;
#18603=CARTESIAN_POINT ( 'NONE',  ( 9.788188108289379130, 1435.901480349360099, 210.0315044652950007 ) ) ;
#18604=CARTESIAN_POINT ( 'NONE',  ( -10.62155590039999886, 1491.490808487190179, 212.0487326096589982 ) ) ;
#18612=CARTESIAN_POINT ( 'NONE',  ( 7.222610535631719841, 1505.072920045980027, 218.4676445938339953 ) ) ;
#18622=CARTESIAN_POINT ( 'NONE',  ( -10.23585214307190050, 1448.784286493050104, 207.3798671416320190 ) ) ;
#18625=CARTESIAN_POINT ( 'NONE',  ( -1.063763185130000011, 1443.513877504690072, 200.1423821450789831 ) ) ;
#18629=B_SPLINE_CURVE_WITH_KNOTS ( 'NONE', 3,
 ( #96366, #70100, #104213, #36450, #44887, #11808, #71194, #61150, #105316, #53848, #95265, #87985, #52723, #18527, #27500, #61688, #11273, #19077, #79579, #16667, #110207, #69342, #43022, #101791, #103451, #26757, #51975, #101229, #17216, #93949, #16128, #68245, #18340, #77722 ),
 .UNSPECIFIED., .F., .F.,
 ( 4, 3, 3, 3, 3, 3, 3, 3, 3, 3, 3, 4 ),
 ( -1.999999989621509933, -1.903346754608929992, -1.716103420023969983, -1.526665084407200057, -1.336006962675679866, -1.143849630969659970, -0.9512259096668089775, -0.7586077023791939489, -0.5664647939433908874, -0.3759670744414520538, -0.1870530681013899965, 0.000000000000000000 ),
 .UNSPECIFIED. ) ;
#18631=CARTESIAN_POINT ( 'NONE',  ( 2.453786550779999853, 1468.127272575889947, 218.8237816726089875 ) ) ;
#18636=CARTESIAN_POINT ( 'NONE',  ( -8.007800200046078842, 1425.247483720839909, 205.0429105383470016 ) ) ;
#18647=CARTESIAN_POINT ( 'NONE',  ( -13.31089767776890120, 1503.456584347970193, 208.6977459380580058 ) ) ;
#18649=CARTESIAN_POINT ( 'NONE',  ( 2.767945032447589604, 1466.138307348149965, 198.4326037334419937 ) ) ;
#18659=CARTESIAN_POINT ( 'NONE',  ( 11.68483446183100050, 1479.114072787690020, 207.7860290712830249 ) ) ;
#18660=ORIENTED_EDGE ( 'NONE', *, *, #24897, .F. ) ;
#18664=CARTESIAN_POINT ( 'NONE',  ( 2.504416157725709802, 1423.539630124239920, 192.6809389493199660 ) ) ;
#18675=CARTESIAN_POINT ( 'NONE',  ( -3.434354545275740023, 1428.676800484289970, 200.4110178052179947 ) ) ;
#18694=VERTEX_POINT ( 'NONE', #5211 ) ;
#18699=AXIS2_PLACEMENT_3D ( 'NONE', #74801, #83189, #14310 ) ;
#18701=FACE_OUTER_BOUND ( 'NONE', #110734, .T. ) ;
#18703=CARTESIAN_POINT ( 'NONE',  ( 15.58948595390000058, 1452.698291846990060, 196.7507890572990163 ) ) ;
#18707=CARTESIAN_POINT ( 'NONE',  ( -0.8833778638539989680, 1431.444913390889951, 200.7505307741990350 ) ) ;
#18708=CARTESIAN_POINT ( 'NONE',  ( 11.22762520574680067, 1480.213122129130170, 210.8215595684870038 ) ) ;
#18709=B_SPLINE_CURVE_WITH_KNOTS ( 'NONE', 5,
 ( #71075, #29044, #44196, #18402, #10026, #37442 ),
 .UNSPECIFIED., .F., .F.,
 ( 6, 6 ),
 ( 203.4370383600000025, 213.0683255119999728 ),
 .UNSPECIFIED. ) ;
#18713=DIRECTION ( 'NONE',  ( 9.056288633775531119E-47, -1.000000000000000000, 1.836970198721029688E-16 ) ) ;
#18715=CARTESIAN_POINT ( 'NONE',  ( 2.104449570759999943, 1486.697367722790204, 197.3627489980989935 ) ) ;
#18716=CARTESIAN_POINT ( 'NONE',  ( 8.801276039060120127, 1468.409988194280004, 201.9109974982270046 ) ) ;
#18718=CARTESIAN_POINT ( 'NONE',  ( 11.87757256900000158, 1501.074157048189818, 209.1815870390489920 ) ) ;
#18720=CARTESIAN_POINT ( 'NONE',  ( 8.334173048470001177, 1428.385525302790029, 213.5056454938490162 ) ) ;
#18722=CARTESIAN_POINT ( 'NONE',  ( -10.25237677790000035, 1481.942191430589901, 205.9184038113290001 ) ) ;
#18732=CARTESIAN_POINT ( 'NONE',  ( -12.05448508659999973, 1501.734409279790043, 211.4994548207789649 ) ) ;
#18733=CARTESIAN_POINT ( 'NONE',  ( -15.08255442401187452, 1416.081365602056167, 205.7412506966217336 ) ) ;
#18738=CARTESIAN_POINT ( 'NONE',  ( -2.584559296679999729, 1450.363170855389853, 190.1601826918989957 ) ) ;
#18739=EDGE_CURVE ( 'NONE', #80101, #65500, #44328, .T. ) ;
#18742=CARTESIAN_POINT ( 'NONE',  ( 7.536781297509999256, 1425.186457032809813, 212.1414899705590074 ) ) ;
#18743=CARTESIAN_POINT ( 'NONE',  ( -13.97985296220000073, 1420.196174967039951, 195.9955836506989897 ) ) ;
#18748=VERTEX_POINT ( 'NONE', #35934 ) ;
#18756=EDGE_CURVE ( 'NONE', #63442, #2433, #45997, .T. ) ;
#18770=EDGE_CURVE ( 'NONE', #84181, #31410, #21463, .T. ) ;
#18772=DIRECTION ( 'NONE',  ( -1.000000000000000000, 0.000000000000000000, 0.000000000000000000 ) ) ;
#18777=VERTEX_POINT ( 'NONE', #54950 ) ;
#18790=EDGE_CURVE ( 'NONE', #103217, #105896, #25176, .T. ) ;
#18794=CARTESIAN_POINT ( 'NONE',  ( 9.549000552458089430, 1470.075890067440014, 212.3436661921319910 ) ) ;
#18800=CARTESIAN_POINT ( 'NONE',  ( 19.64609177186540023, 1476.662525844680204, 214.0395018079669853 ) ) ;
#18804=ADVANCED_FACE ( 'NONE', ( #72842 ), #98062, .F. ) ;
#18809=ORIENTED_EDGE ( 'NONE', *, *, #10421, .T. ) ;
#18811=CARTESIAN_POINT ( 'NONE',  ( -3.478767832449999986, 1430.446984450989930, 201.5308695822689913 ) ) ;
#18817=CARTESIAN_POINT ( 'NONE',  ( 12.03764642179999989, 1426.191797886159975, 202.7989836356990168 ) ) ;
#18825=CARTESIAN_POINT ( 'NONE',  ( -4.602356253840000022, 1468.583955076089978, 189.7619545879989857 ) ) ;
#18826=ORIENTED_EDGE ( 'NONE', *, *, #95281, .T. ) ;
#18830=CARTESIAN_POINT ( 'NONE',  ( 2.961602933630000045, 1442.729505202489918, 217.4993384840889803 ) ) ;
#18836=CARTESIAN_POINT ( 'NONE',  ( -3.882745883101669904, 1464.675334460000158, 198.8121422478580200 ) ) ;
#18841=EDGE_LOOP ( 'NONE', ( #46931, #70823, #89777, #17365 ) ) ;
#18843=CARTESIAN_POINT ( 'NONE',  ( -4.491284101706960463, 1508.884228866460035, 211.6097700714119867 ) ) ;
#18844=CARTESIAN_POINT ( 'NONE',  ( -21.12854634993719927, 1507.715432715349834, 209.4790063854959783 ) ) ;
#18848=CARTESIAN_POINT ( 'NONE',  ( -11.24594776555490050, 1470.381349896640131, 210.9060676379959887 ) ) ;
#18849=CARTESIAN_POINT ( 'NONE',  ( -9.799324650868589615, 1490.915621052960205, 214.1421080411050184 ) ) ;
#18850=CARTESIAN_POINT ( 'NONE',  ( -2.515593459366479934, 1448.349639805989909, 188.5842434069749913 ) ) ;
#18856=CARTESIAN_POINT ( 'NONE',  ( 10.54727210182790031, 1452.235375780489903, 208.6466202666740060 ) ) ;
#18868=CARTESIAN_POINT ( 'NONE',  ( 9.393521813728380465, 1435.928492946419965, 209.6064062774240142 ) ) ;
#18876=CARTESIAN_POINT ( 'NONE',  ( -16.43158050010680071, 1420.644938884899830, 203.2808245233400157 ) ) ;
#18878=CARTESIAN_POINT ( 'NONE',  ( 4.873735476160000246, 1472.089320948289924, 218.0431589096889695 ) ) ;
#18880=CARTESIAN_POINT ( 'NONE',  ( -2.487921644133310295, 1508.551704408389924, 214.1089243590330113 ) ) ;
#18882=CARTESIAN_POINT ( 'NONE',  ( -3.160253207629999839, 1471.445056511090115, 187.3830100966989960 ) ) ;
#18884=LINE ( 'NONE', #53082, #80265 ) ;
#18898=ORIENTED_EDGE ( 'NONE', *, *, #3187, .F. ) ;
#18903=CARTESIAN_POINT ( 'NONE',  ( -17.61781123130856486, 1419.766076753951438, 206.8127147925555960 ) ) ;
#18904=CARTESIAN_POINT ( 'NONE',  ( 7.069913306463050162, 1426.666554464499995, 213.2414280066960259 ) ) ;
#18905=CARTESIAN_POINT ( 'NONE',  ( 1.724603976620079804, 1495.787172650469984, 221.3394264603180090 ) ) ;
#18910=CARTESIAN_POINT ( 'NONE',  ( 2.251015183664099695, 1487.021489544721135, 219.7028229865901494 ) ) ;
#18912=CARTESIAN_POINT ( 'NONE',  ( 5.346297422500000174, 1473.360741859489963, 218.2967445439789742 ) ) ;
#18913=CARTESIAN_POINT ( 'NONE',  ( -8.312969881423960317, 1439.013910285169914, 206.4662266169680152 ) ) ;
#18914=ORIENTED_EDGE ( 'NONE', *, *, #69366, .F. ) ;
#18944=CARTESIAN_POINT ( 'NONE',  ( 12.27050434115719924, 1501.509400875670053, 212.4841319041250074 ) ) ;
#18947=CARTESIAN_POINT ( 'NONE',  ( -3.674412922749999755, 1496.836503961589870, 198.4902213705989880 ) ) ;
#18953=CARTESIAN_POINT ( 'NONE',  ( 8.915638207339146248, 1427.583583160426770, 192.9091311759471523 ) ) ;
#18962=CARTESIAN_POINT ( 'NONE',  ( 0.8472549444895222104, 1421.277937719025203, 193.7387945151137387 ) ) ;
#18963=CARTESIAN_POINT ( 'NONE',  ( -4.329068131567179734, 1515.079329108559932, 207.7116314705500315 ) ) ;
#18968=CARTESIAN_POINT ( 'NONE',  ( -9.659452839195818541, 1460.929932477109787, 210.9155389501709976 ) ) ;
#18969=CARTESIAN_POINT ( 'NONE',  ( -17.00466766660930062, 1420.052239869899950, 201.4977556186619836 ) ) ;
#18971=CARTESIAN_POINT ( 'NONE',  ( 9.580287517196040881, 1463.259152023979823, 211.7413480895340001 ) ) ;
#18976=CARTESIAN_POINT ( 'NONE',  ( -15.75193611358070456, 1420.305119455802014, 210.1813702474818228 ) ) ;
#18979=CARTESIAN_POINT ( 'NONE',  ( 18.46110513727499836, 1471.786120601949960, 195.2229452025129888 ) ) ;
#18981=CARTESIAN_POINT ( 'NONE',  ( -2201.413669186790685, 11221.53578756870047, 1941.356037698088358 ) ) ;
#18982=CARTESIAN_POINT ( 'NONE',  ( 9.132990796547860057, 1451.136122370250177, 210.6042708154840000 ) ) ;
#18983=CARTESIAN_POINT ( 'NONE',  ( 3.391831335510000045, 1441.614882265790129, 217.6841840411589999 ) ) ;
#18990=CARTESIAN_POINT ( 'NONE',  ( -4.098986974010339956, 1508.551704408389924, 219.8451935736590031 ) ) ;
#18991=ORIENTED_EDGE ( 'NONE', *, *, #25313, .F. ) ;
#18996=CARTESIAN_POINT ( 'NONE',  ( -4.993214567250789493, 1391.653935164599716, 214.7089805434449943 ) ) ;
#18997=CARTESIAN_POINT ( 'NONE',  ( -10.67674005382819935, 1471.688487720359944, 206.9114804947679715 ) ) ;
#19003=ORIENTED_EDGE ( 'NONE', *, *, #72271, .F. ) ;
#19004=CARTESIAN_POINT ( 'NONE',  ( 10.83651939265710062, 1490.169899907720037, 207.5021329017099845 ) ) ;
#19005=CARTESIAN_POINT ( 'NONE',  ( -1.023515647982950139, 1438.105133628250087, 227.6662252542259921 ) ) ;
#19006=ORIENTED_EDGE ( 'NONE', *, *, #53892, .F. ) ;
#19007=CARTESIAN_POINT ( 'NONE',  ( 8.729347899703789437, 1465.224243514420095, 213.7259074896789741 ) ) ;
#19016=CARTESIAN_POINT ( 'NONE',  ( 3.601841467080000303, 1444.840595811589992, 200.9001250664390170 ) ) ;
#19026=CARTESIAN_POINT ( 'NONE',  ( -3.237583812329999589, 1495.897743034890027, 219.8603346627990049 ) ) ;
#19031=EDGE_CURVE ( 'NONE', #38120, #61362, #49677, .T. ) ;
#19042=CARTESIAN_POINT ( 'NONE',  ( 3.262929297844129994, 1508.551704408389924, 213.9871752814069907 ) ) ;
#19046=CARTESIAN_POINT ( 'NONE',  ( 9.591489393450858714, 1462.438986607349989, 207.3792329919180020 ) ) ;
#19048=EDGE_LOOP ( 'NONE', ( #25127, #64280, #110526, #103040 ) ) ;
#19050=CARTESIAN_POINT ( 'NONE',  ( 9.699673965497980888, 1453.359162548709946, 212.1674369800300042 ) ) ;
#19051=CARTESIAN_POINT ( 'NONE',  ( 8.472418160909999330, 1423.407106218679928, 196.2202384860989923 ) ) ;
#19058=CARTESIAN_POINT ( 'NONE',  ( 9.723778708192279296, 1452.046992748000093, 209.3441726741959883 ) ) ;
#19059=CARTESIAN_POINT ( 'NONE',  ( 6.483588104269999874, 1462.707724100489941, 208.1814389384059893 ) ) ;
#19072=CARTESIAN_POINT ( 'NONE',  ( -10.13006551440279956, 1470.128316028900144, 213.2258428534270251 ) ) ;
#19076=CARTESIAN_POINT ( 'NONE',  ( -12.52558728303339919, 1501.938162216189994, 211.4646196275029979 ) ) ;
#19077=CARTESIAN_POINT ( 'NONE',  ( -2.206411215550580174, 1421.659913175079964, 193.5263021252320073 ) ) ;
#19079=CARTESIAN_POINT ( 'NONE',  ( 9.475903704820970219, 1425.358992633405023, 195.5313119463182829 ) ) ;
#19084=CARTESIAN_POINT ( 'NONE',  ( -9.946277618806290022, 1439.610876520569946, 208.1166930489989966 ) ) ;
#19093=CARTESIAN_POINT ( 'NONE',  ( 0.01406703362208180062, 1515.158574431529814, 204.7948529419429917 ) ) ;
#19095=CARTESIAN_POINT ( 'NONE',  ( -16.62146796077700017, 1418.479381249660037, 203.0020891297729975 ) ) ;
#19096=CARTESIAN_POINT ( 'NONE',  ( 2.719262146893400038E-32, 1524.051704408389924, 209.1218459616989946 ) ) ;
#19098=CARTESIAN_POINT ( 'NONE',  ( -2.182355088989220260, 1429.366333297759866, 200.0022119995389858 ) ) ;
#19099=CARTESIAN_POINT ( 'NONE',  ( 2.717866887673947129, 1443.364948805944778, 217.6365403981836835 ) ) ;
#19105=CARTESIAN_POINT ( 'NONE',  ( -4.524029051260000323, 1475.733900273690097, 218.4636560311490143 ) ) ;
#19106=CARTESIAN_POINT ( 'NONE',  ( 543.1695162809550084, 1433.553134552160145, 209.1604895367889867 ) ) ;
#19109=CIRCLE ( 'NONE', #106724, 783.3212999198779016 ) ;
#19123=EDGE_CURVE ( 'NONE', #90525, #94930, #6805, .T. ) ;
#19139=CARTESIAN_POINT ( 'NONE',  ( 4.327507230410000183, 1515.138937518789817, 208.4081006986280045 ) ) ;
#19143=CARTESIAN_POINT ( 'NONE',  ( 11.21638122688047190, 1413.913060387330006, 209.8266014933971064 ) ) ;
#19144=CARTESIAN_POINT ( 'NONE',  ( 3.327063897169999507, 1422.406709332250102, 194.0529592594990049 ) ) ;
#19147=CARTESIAN_POINT ( 'NONE',  ( 19.08743583839999758, 1460.091080419490027, 220.2973930160990221 ) ) ;
#19149=LINE ( 'NONE', #46061, #47885 ) ;
#19151=CARTESIAN_POINT ( 'NONE',  ( -5.156154518200000147, 1391.908488942590111, 203.6345722630290140 ) ) ;
#19153=CARTESIAN_POINT ( 'NONE',  ( -11.63492915560000007, 1490.028483917189988, 211.0527168509590012 ) ) ;
#19158=CARTESIAN_POINT ( 'NONE',  ( -15.52565719226596741, 1421.385870312634552, 199.5589395028577542 ) ) ;
#19161=CARTESIAN_POINT ( 'NONE',  ( -14.46094609940118758, 1420.539308687509902, 213.8039270598953863 ) ) ;
#19164=ORIENTED_EDGE ( 'NONE', *, *, #14562, .F. ) ;
#19169=CARTESIAN_POINT ( 'NONE',  ( -2.354624258718260421, 1456.603527532422959, 199.9289168914013715 ) ) ;
#19170=CARTESIAN_POINT ( 'NONE',  ( 10.92766316470000021, 1501.618322990889965, 205.6861136852989773 ) ) ;
#19175=CARTESIAN_POINT ( 'NONE',  ( -0.2202020877210009997, 1467.752737336390055, 219.8452965410990032 ) ) ;
#19183=ORIENTED_EDGE ( 'NONE', *, *, #66731, .T. ) ;
#19185=CARTESIAN_POINT ( 'NONE',  ( 1.110979151289160027, 1432.780184589570126, 200.7448731778110016 ) ) ;
#19187=ORIENTED_EDGE ( 'NONE', *, *, #21439, .T. ) ;
#19193=CARTESIAN_POINT ( 'NONE',  ( -3.744257397248767383, 1509.032015221108395, 204.8809009245644859 ) ) ;
#19194=CARTESIAN_POINT ( 'NONE',  ( 10.96046450149999885, 1461.176790603689824, 209.3104301672979943 ) ) ;
#19195=B_SPLINE_CURVE_WITH_KNOTS ( 'NONE', 3,
 ( #15303, #10091, #41634, #1719, #44265, #18466, #50589, #95205, #74697, #108829 ),
 .UNSPECIFIED., .F., .F.,
 ( 4, 2, 2, 2, 4 ),
 ( -2.293181918888250070, -1.719760621652620003, -1.147337202555609892, -0.5730822307304319629, 0.000000000000000000 ),
 .UNSPECIFIED. ) ;
#19198=CARTESIAN_POINT ( 'NONE',  ( 2.360870863690000210, 1465.193912104189849, 199.3990268566589918 ) ) ;
#19199=CARTESIAN_POINT ( 'NONE',  ( 8.632911994995870586, 1437.313349126720141, 208.5977050715380017 ) ) ;
#19214=CARTESIAN_POINT ( 'NONE',  ( -6.255913365080000510, 1508.980388112989885, 219.5104367483990018 ) ) ;
#19217=CARTESIAN_POINT ( 'NONE',  ( 5.521731335039999244, 1437.871055919089940, 209.1877786888699973 ) ) ;
#19220=CARTESIAN_POINT ( 'NONE',  ( 1.600144450079999947, 1468.978733938389951, 216.2351156805190158 ) ) ;
#19242=CARTESIAN_POINT ( 'NONE',  ( 4.730384172586849623, 1508.603735228350843, 211.6097810847320204 ) ) ;
#19245=EDGE_CURVE ( 'NONE', #37608, #50173, #82973, .T. ) ;
#19253=B_SPLINE_CURVE_WITH_KNOTS ( 'NONE', 3,
 ( #10156, #37008, #78473, #71201, #35924, #79043, #28615, #61694, #19084, #87426, #44893, #36457, #62817, #70656, #96931, #104772, #28056, #20198, #62247, #30805, #72831, #89064, #30248, #38655, #108060, #22377, #13995, #56577, #47081, #90709, #81205, #63352, #6155, #48181, #107516, #80674, #64442, #82320, #89611, #72289 ),
 .UNSPECIFIED., .F., .F.,
 ( 4, 3, 3, 3, 3, 3, 3, 3, 3, 3, 3, 3, 3, 4 ),
 ( -7.339220616559999577, -7.191616119070119773, -6.955040122091289412, -6.699117395807109965, -6.422619652672629798, -6.106550893931229851, -5.718306387288239812, -5.419628814236969738, -5.176305405323340381, -4.933732890374959545, -4.561789723725830470, -4.129459730253979721, -3.452867597008769884, -3.013389252340000546 ),
 .UNSPECIFIED. ) ;
#19255=CARTESIAN_POINT ( 'NONE',  ( 1.914156564180000020, 1431.087920464090075, 199.8421651513589836 ) ) ;
#19259=CARTESIAN_POINT ( 'NONE',  ( 3.123423494469999895, 1507.140718701690048, 220.4075764222990017 ) ) ;
#19265=CARTESIAN_POINT ( 'NONE',  ( 3.152706770380329537, 1465.853101953990063, 199.3412496788349983 ) ) ;
#19267=CARTESIAN_POINT ( 'NONE',  ( 4.822497006680000808, 1500.099429524390189, 201.8516542630590038 ) ) ;
#19268=CIRCLE ( 'NONE', #22856, 8.104319688360000384 ) ;
#19275=( BOUNDED_CURVE ( )  B_SPLINE_CURVE ( 3, ( #3265, #19471, #20026, #36837 ),
 .UNSPECIFIED., .F., .F. ) 
 B_SPLINE_CURVE_WITH_KNOTS ( ( 4, 4 ),
 ( 1.009476837204658084, 2.132115841021330116 ),
 .UNSPECIFIED. ) 
 CURVE ( )  GEOMETRIC_REPRESENTATION_ITEM ( )  RATIONAL_B_SPLINE_CURVE ( ( 1.000000000000000000, 0.8977023149622460618, 0.8977023149622460618, 1.000000000000000000 ) ) 
 REPRESENTATION_ITEM ( '' )  );
#19277=EDGE_CURVE ( 'NONE', #53387, #23318, #58996, .T. ) ;
#19280=CARTESIAN_POINT ( 'NONE',  ( -7.351108641702090551, 1491.337179302150162, 211.7591575584629879 ) ) ;
#19281=EDGE_LOOP ( 'NONE', ( #57028, #68784, #102726, #37551 ) ) ;
#19282=CARTESIAN_POINT ( 'NONE',  ( -19.47231853460000295, 1466.701452153789887, 212.9249870548489980 ) ) ;
#19283=CARTESIAN_POINT ( 'NONE',  ( -13.58798618625510102, 1508.413595127150074, 209.8328882561570197 ) ) ;
#19284=EDGE_CURVE ( 'NONE', #29958, #6066, #58661, .T. ) ;
#19287=CARTESIAN_POINT ( 'NONE',  ( -9.949472290641201866, 1438.963978288880071, 209.6181135091480030 ) ) ;
#19288=CARTESIAN_POINT ( 'NONE',  ( 3.879157139540000188, 1451.813806661290073, 190.3284334383990029 ) ) ;
#19293=CARTESIAN_POINT ( 'NONE',  ( 7.645128971980000188, 1425.330907912760040, 211.9289184192489870 ) ) ;
#19294=CARTESIAN_POINT ( 'NONE',  ( -16.61337445550000069, 1463.629612651790012, 220.4655171657990138 ) ) ;
#19302=ORIENTED_EDGE ( 'NONE', *, *, #22687, .F. ) ;
#19309=CARTESIAN_POINT ( 'NONE',  ( -2.845798587710199890, 1464.349408459529968, 199.2989423254240080 ) ) ;
#19323=CARTESIAN_POINT ( 'NONE',  ( -4.254366227259999356, 1454.573790426789856, 200.5971711767689953 ) ) ;
#19330=CARTESIAN_POINT ( 'NONE',  ( 4.464821409069999802, 1422.103166678080015, 206.5928916359989955 ) ) ;
#19336=CARTESIAN_POINT ( 'NONE',  ( -11.84353516585279920, 1489.590656028399962, 212.0913857160410032 ) ) ;
#19353=CARTESIAN_POINT ( 'NONE',  ( 19.38539822485692810, 1495.497225806873075, 199.6821155845800888 ) ) ;
#19363=CARTESIAN_POINT ( 'NONE',  ( -2.593205515350000212, 1429.616254713290118, 200.8413778689989897 ) ) ;
#19367=CARTESIAN_POINT ( 'NONE',  ( 3.535327660699999708, 1487.160996047289927, 197.6951164054989931 ) ) ;
#19377=VERTEX_POINT ( 'NONE', #95561 ) ;
#19382=CARTESIAN_POINT ( 'NONE',  ( 2.838547795930000284, 1441.919264588690112, 217.8904307960689835 ) ) ;
#19384=CARTESIAN_POINT ( 'NONE',  ( -2178.386296064867111, -8387.357407334289746, 1972.013908154370711 ) ) ;
#19391=CARTESIAN_POINT ( 'NONE',  ( 6.636923444789999849, 1488.278828811890207, 199.0403411110989964 ) ) ;
#19394=VERTEX_POINT ( 'NONE', #36210 ) ;
#19399=CARTESIAN_POINT ( 'NONE',  ( -4.687677274410000372, 1484.078770814390055, 199.3574548446190136 ) ) ;
#19403=CARTESIAN_POINT ( 'NONE',  ( 5.402657594482866976, 1473.518541113343190, 218.3241216679554100 ) ) ;
#19409=CARTESIAN_POINT ( 'NONE',  ( -8.097225737347908847, 1490.150856172170052, 216.5834626028189973 ) ) ;
#19410=CARTESIAN_POINT ( 'NONE',  ( 7.755364537188749630, 1459.738773378459882, 228.9106043144229830 ) ) ;
#19417=VERTEX_POINT ( 'NONE', #41170 ) ;
#19420=CARTESIAN_POINT ( 'NONE',  ( -14.75654852344869816, 1418.698223271940151, 213.5276923267749964 ) ) ;
#19429=CARTESIAN_POINT ( 'NONE',  ( -4.660842796387490772, 1495.148806942539977, 197.7136934498280141 ) ) ;
#19433=AXIS2_PLACEMENT_3D ( 'NONE', #4356, #105718, #63724 ) ;
#19439=CARTESIAN_POINT ( 'NONE',  ( -9.860632074819870141, 1424.099558978640061, 204.5593013001630140 ) ) ;
#19440=CARTESIAN_POINT ( 'NONE',  ( -12.23489732466240021, 1490.237667237379810, 209.6383001084460034 ) ) ;
#19441=CARTESIAN_POINT ( 'NONE',  ( -19.18813880309999931, 1465.797355387890093, 204.3301597990889888 ) ) ;
#19445=CARTESIAN_POINT ( 'NONE',  ( -11.93924564462519911, 1481.986046384150086, 228.0814323177490053 ) ) ;
#19447=CARTESIAN_POINT ( 'NONE',  ( 7.571416212307459759, 1423.019345442000031, 195.7264161909869813 ) ) ;
#19450=CARTESIAN_POINT ( 'NONE',  ( 4.329177920710189476, 1515.075136430340081, 210.6018449539679978 ) ) ;
#19460=B_SPLINE_CURVE_WITH_KNOTS ( 'NONE', 5,
 ( #11847, #35953, #10754, #36494, #54430, #79072 ),
 .UNSPECIFIED., .F., .F.,
 ( 6, 6 ),
 ( 330.1233636409999690, 340.1768165719999502 ),
 .UNSPECIFIED. ) ;
#19463=CARTESIAN_POINT ( 'NONE',  ( -9.655463540387350108, 1446.888654090670116, 212.1942763251040276 ) ) ;
#19467=CARTESIAN_POINT ( 'NONE',  ( -3.566337987641670093, 1497.263210272700235, 220.9985256183890101 ) ) ;
#19469=EDGE_LOOP ( 'NONE', ( #63051, #27777, #13595, #35069, #103415 ) ) ;
#19471=CARTESIAN_POINT ( 'NONE',  ( 3.497662945300243909, 1505.961916725443189, 220.6749222718410692 ) ) ;
#19474=CARTESIAN_POINT ( 'NONE',  ( -18.15878713041950121, 1508.551704422010062, 211.0186658100620036 ) ) ;
#19475=CARTESIAN_POINT ( 'NONE',  ( 4.873735476160000246, 1472.089320948289924, 218.0431589096889695 ) ) ;
#19476=CARTESIAN_POINT ( 'NONE',  ( -9.966728652698208180, 1439.480322961800084, 208.4310021967300202 ) ) ;
#19481=CARTESIAN_POINT ( 'NONE',  ( 8.721922434858829121, 1435.147675358199876, 206.9711085294910049 ) ) ;
#19486=CARTESIAN_POINT ( 'NONE',  ( -1.126170950785350122, 1467.742527459179882, 220.1728790705329857 ) ) ;
#19487=CARTESIAN_POINT ( 'NONE',  ( -20.61921987750000085, 1486.434067572889944, 211.1039075214289937 ) ) ;
#19493=AXIS2_PLACEMENT_3D ( 'NONE', #48186, #82867, #21281 ) ;
#19499=CARTESIAN_POINT ( 'NONE',  ( 4.229167303610000594, 1436.983388288790138, 227.1518914930990150 ) ) ;
#19520=CARTESIAN_POINT ( 'NONE',  ( -7.195479650174489983, 1484.442662870319964, 199.6339812554890045 ) ) ;
#19523=CARTESIAN_POINT ( 'NONE',  ( -4.326999254989129184, 1515.158336317470003, 209.0580706801189876 ) ) ;
#19530=DIRECTION ( 'NONE',  ( 1.224227143275421080E-16, 0.02617694830808806397, -0.9996573249755517088 ) ) ;
#19531=CARTESIAN_POINT ( 'NONE',  ( 2.931378713556060056, 1425.355483872539935, 188.8538262268459960 ) ) ;
#19542=CARTESIAN_POINT ( 'NONE',  ( -15.99924670575417274, 1420.237028991483839, 209.6647657703803702 ) ) ;
#19545=CARTESIAN_POINT ( 'NONE',  ( -4.987082939647749846, 1508.551704408389924, 205.8487953860969810 ) ) ;
#19548=CARTESIAN_POINT ( 'NONE',  ( 9.078035843596250487, 1451.272942437749862, 210.9408701583590187 ) ) ;
#19549=CARTESIAN_POINT ( 'NONE',  ( 5.083972363190000898, 1436.382653089989844, 207.1318876291190350 ) ) ;
#19557=CARTESIAN_POINT ( 'NONE',  ( -6.763867816925220211, 1508.551704407960187, 219.2477951563350018 ) ) ;
#19560=CARTESIAN_POINT ( 'NONE',  ( 2.091623246919999790, 1485.160878225490251, 201.4201072810890025 ) ) ;
#19563=CARTESIAN_POINT ( 'NONE',  ( -2.427501210939999599, 1432.717019920590019, 217.9482129255790142 ) ) ;
#19564=CARTESIAN_POINT ( 'NONE',  ( -15.05548819430000052, 1420.901177493080013, 212.6278861834389886 ) ) ;
#19569=ADVANCED_FACE ( 'NONE', ( #60758 ), #26445, .T. ) ;
#19573=AXIS2_PLACEMENT_3D ( 'NONE', #12097, #72574, #46292 ) ;
#19574=CARTESIAN_POINT ( 'NONE',  ( 11.84326266240529968, 1491.682748273859943, 208.2990869752020160 ) ) ;
#19575=CARTESIAN_POINT ( 'NONE',  ( -4.073851350468440380, 1438.760108550490258, 227.2697485756019944 ) ) ;
#19577=ORIENTED_EDGE ( 'NONE', *, *, #26368, .T. ) ;
#19594=CARTESIAN_POINT ( 'NONE',  ( 2.135980618300000078, 1495.504087388789912, 220.8536851825989800 ) ) ;
#19606=CARTESIAN_POINT ( 'NONE',  ( 2.869680150050000211, 1485.441877061090054, 219.8814458974989918 ) ) ;
#19617=CARTESIAN_POINT ( 'NONE',  ( 9.485899553554340002, 1452.846731054919928, 211.4225977852020151 ) ) ;
#19618=CARTESIAN_POINT ( 'NONE',  ( -2.114480094995805359, 1486.828170616315219, 220.1547108737681526 ) ) ;
#19621=CARTESIAN_POINT ( 'NONE',  ( -6.144022937698749409, 1419.445111502675900, 195.0001984287017081 ) ) ;
#19626=CARTESIAN_POINT ( 'NONE',  ( 6.177640194960000386, 1462.009621597289879, 206.9307941614490289 ) ) ;
#19635=EDGE_LOOP ( 'NONE', ( #50974, #52674, #104503, #2254 ) ) ;
#19636=CARTESIAN_POINT ( 'NONE',  ( -0.9490323356187280179, 1507.925252277985237, 221.0232043774789759 ) ) ;
#19637=CARTESIAN_POINT ( 'NONE',  ( -6.585747151019099022, 1508.339498974060007, 219.9410548752989882 ) ) ;
#19639=CARTESIAN_POINT ( 'NONE',  ( -9.683432862967901400, 1470.976754966750150, 212.5624612103730158 ) ) ;
#19644=CARTESIAN_POINT ( 'NONE',  ( -5.546142131579999912, 1474.984681366790028, 200.2534476738289868 ) ) ;
#19647=FACE_OUTER_BOUND ( 'NONE', #79674, .T. ) ;
#19648=CARTESIAN_POINT ( 'NONE',  ( -15.05712110500000023, 1503.430198388489998, 209.1799330422220180 ) ) ;
#19659=CARTESIAN_POINT ( 'NONE',  ( 3.964328110410000328, 1507.304896082889854, 220.1351224040989791 ) ) ;
#19660=CARTESIAN_POINT ( 'NONE',  ( -15.04150367899999985, 1415.861021494549959, 212.2455458053489963 ) ) ;
#19661=CARTESIAN_POINT ( 'NONE',  ( -0.9669097429813701128, 1515.111355597239935, 204.7936164732989823 ) ) ;
#19663=CARTESIAN_POINT ( 'NONE',  ( -15.86313006842250317, 1415.917248183199717, 209.7285344443807276 ) ) ;
#19666=CARTESIAN_POINT ( 'NONE',  ( 1.529355925611250111, 1430.956820494460089, 199.7836114767660263 ) ) ;
#19673=CARTESIAN_POINT ( 'NONE',  ( 9.875005135842670256, 1469.705720279170237, 211.0604535260579837 ) ) ;
#19712=DIRECTION ( 'NONE',  ( -1.156023075842281927E-31, 1.000000000000000000, -1.698192320643030073E-16 ) ) ;
#19715=EDGE_CURVE ( 'NONE', #49951, #88894, #66931, .T. ) ;
#19723=CARTESIAN_POINT ( 'NONE',  ( -2.711451550492540274, 1449.129774548599926, 188.5718384860999777 ) ) ;
#19724=CARTESIAN_POINT ( 'NONE',  ( -4.523944140811339665, 1455.378620635879997, 200.8408219016489795 ) ) ;
#19728=DIRECTION ( 'NONE',  ( 0.1189347811660100146, -0.4481226533063590312, 0.8860251720028400335 ) ) ;
#19730=FACE_OUTER_BOUND ( 'NONE', #74865, .T. ) ;
#19731=CARTESIAN_POINT ( 'NONE',  ( 20.41258333560000082, 1494.156730172889866, 204.1224707391089908 ) ) ;
#19732=CARTESIAN_POINT ( 'NONE',  ( 9.774666768839999520, 1462.791335443590015, 210.7173514753790187 ) ) ;
#19738=CARTESIAN_POINT ( 'NONE',  ( -12.18049167383413156, 1421.733962334860962, 210.6454646573376692 ) ) ;
#19740=ORIENTED_EDGE ( 'NONE', *, *, #45419, .F. ) ;
#19742=CARTESIAN_POINT ( 'NONE',  ( 4.329448781177520189, 1515.064792686469900, 207.2788827064790098 ) ) ;
#19745=CARTESIAN_POINT ( 'NONE',  ( 11.82750276210000173, 1499.979357237489921, 206.0369006055389889 ) ) ;
#19755=CARTESIAN_POINT ( 'NONE',  ( -4.192418968486159692, 1427.449526014519961, 207.6357443616469993 ) ) ;
#19759=CARTESIAN_POINT ( 'NONE',  ( 1.227353608591539968, 1432.824896673809917, 200.7599812625429934 ) ) ;
#19765=AXIS2_PLACEMENT_3D ( 'NONE', #81094, #45324, #19530 ) ;
#19768=CARTESIAN_POINT ( 'NONE',  ( 9.698064379080001629, 1462.705242066090022, 208.0596161272490292 ) ) ;
#19771=CARTESIAN_POINT ( 'NONE',  ( 2.846372769239999823, 1466.158655091689980, 198.4435757763990011 ) ) ;
#19773=VERTEX_POINT ( 'NONE', #109838 ) ;
#19778=CARTESIAN_POINT ( 'NONE',  ( 11.75386664412339854, 1479.308097208950130, 208.5149014641469876 ) ) ;
#19784=CARTESIAN_POINT ( 'NONE',  ( 19.75641515910000123, 1473.226389329089898, 205.2875698398590316 ) ) ;
#19786=CARTESIAN_POINT ( 'NONE',  ( -2.618314538174938644, 1456.062981335259792, 218.2460851740787575 ) ) ;
#19789=CARTESIAN_POINT ( 'NONE',  ( -3.535195929379999491, 1507.570998153189976, 221.3286709398989842 ) ) ;
#19791=FACE_OUTER_BOUND ( 'NONE', #63326, .T. ) ;
#19793=CARTESIAN_POINT ( 'NONE',  ( -4.794426340529999386, 1463.608615258990085, 228.2108236244990280 ) ) ;
#19804=CARTESIAN_POINT ( 'NONE',  ( -15.22586266600000116, 1415.677402186129939, 207.8856753661189884 ) ) ;
#19809=CARTESIAN_POINT ( 'NONE',  ( -9.850334483518770057, 1448.894916128399927, 207.6442625542179883 ) ) ;
#19814=CARTESIAN_POINT ( 'NONE',  ( -0.7223987349340009745, 1515.137743094390089, 213.4493844692189839 ) ) ;
#19816=B_SPLINE_CURVE_WITH_KNOTS ( 'NONE', 3,
 ( #14644, #21915, #30343, #56111, #99741, #72920, #23032, #99187, #108709, #5147, #57234, #23593, #73475, #31443, #29799, #98648, #107608, #90243, #80765, #63987, #13525, #72381, #22466, #91365, #47713, #15177, #81843, #4608, #48830, #32000, #4073, #64534, #6245, #38198, #12983, #39857, #30891 ),
 .UNSPECIFIED., .F., .F.,
 ( 4, 3, 3, 3, 3, 3, 3, 3, 3, 3, 3, 3, 4 ),
 ( -12.49638257910000050, -12.31284761734790045, -11.59982707651139933, -10.84582623330600093, -10.05221012059380037, -9.203745996424679277, -8.197201293281651147, -7.200146307280610003, -6.413310767835159965, -5.453294015972889319, -4.614923386693979168, -3.884091819314949845, -3.197141790549999030 ),
 .UNSPECIFIED. ) ;
#19818=CARTESIAN_POINT ( 'NONE',  ( -19.58687656140000399, 1466.791876332389847, 212.2343231219589939 ) ) ;
#19823=CARTESIAN_POINT ( 'NONE',  ( 10.71258033046609803, 1462.053283461631736, 211.5459195315542047 ) ) ;
#19825=CARTESIAN_POINT ( 'NONE',  ( -18.70878219499999773, 1442.609711808290058, 207.2810541335790049 ) ) ;
#19829=CARTESIAN_POINT ( 'NONE',  ( 2.589445462300000056, 1486.845472968690046, 197.4512227720990154 ) ) ;
#19830=CARTESIAN_POINT ( 'NONE',  ( 8.068722499177209073, 1467.590995982949835, 202.7938328808809842 ) ) ;
#19831=VECTOR ( 'NONE', #9327, 1000.000000000000227 ) ;
#19839=CARTESIAN_POINT ( 'NONE',  ( -8.826539524659999358, 1481.764331591789869, 203.1249523938089965 ) ) ;
#19847=CARTESIAN_POINT ( 'NONE',  ( -11.32856707963236609, 1502.802494384597594, 207.1046524659502381 ) ) ;
#19856=CARTESIAN_POINT ( 'NONE',  ( 7.681575139199999569, 1426.029983472850063, 211.9426460963890122 ) ) ;
#19862=CARTESIAN_POINT ( 'NONE',  ( 7.407831571229999135, 1453.765711829389829, 215.1756217022590079 ) ) ;
#19868=CARTESIAN_POINT ( 'NONE',  ( 5.229023875898142215, 1499.677744264015701, 199.0195098952981425 ) ) ;
#19877=CARTESIAN_POINT ( 'NONE',  ( 3.829620113550000315, 1515.551704408389924, 207.0352977830190184 ) ) ;
#19881=ORIENTED_EDGE ( 'NONE', *, *, #11225, .T. ) ;
#19883=CARTESIAN_POINT ( 'NONE',  ( -3.423043413499999854, 1454.376749419989892, 199.6187636058789963 ) ) ;
#19889=CARTESIAN_POINT ( 'NONE',  ( 7.910841848800000520, 1423.398885000399787, 212.8692358303489982 ) ) ;
#19893=ADVANCED_FACE ( 'NONE', ( #76235 ), #103330, .T. ) ;
#19897=EDGE_CURVE ( 'NONE', #35904, #59861, #89724, .T. ) ;
#19903=ORIENTED_EDGE ( 'NONE', *, *, #64081, .T. ) ;
#19913=CARTESIAN_POINT ( 'NONE',  ( 10.61608522903719987, 1426.022631771789975, 194.5346624901540054 ) ) ;
#19919=EDGE_CURVE ( 'NONE', #84881, #102658, #58574, .T. ) ;
#19934=CARTESIAN_POINT ( 'NONE',  ( 10.43360265539999965, 1481.587351803889987, 210.8844954032190060 ) ) ;
#19936=CARTESIAN_POINT ( 'NONE',  ( 10.01009039213920104, 1469.368769691539910, 209.9822530231150211 ) ) ;
#19947=CARTESIAN_POINT ( 'NONE',  ( 1.647714509864909749, 1423.871873006899932, 191.2482835822270033 ) ) ;
#19957=CARTESIAN_POINT ( 'NONE',  ( 3.115880651068799967, 1508.551704408389924, 219.3718644903320012 ) ) ;
#19962=CARTESIAN_POINT ( 'NONE',  ( -2.333997945480000169, 1485.067782868789891, 198.2455608594989940 ) ) ;
#19966=( GEOMETRIC_REPRESENTATION_CONTEXT ( 3 ) GLOBAL_UNCERTAINTY_ASSIGNED_CONTEXT ( ( #78202 ) ) GLOBAL_UNIT_ASSIGNED_CONTEXT ( ( #35457, #58464, #85289 ) ) REPRESENTATION_CONTEXT ( 'NONE', 'WORKASPACE' ) );
#19970=CARTESIAN_POINT ( 'NONE',  ( -11.28984392593030073, 1489.194882175770090, 213.7480122154229889 ) ) ;
#19971=CARTESIAN_POINT ( 'NONE',  ( 16.66443376260370002, 1492.498784242470037, 193.3249348817559792 ) ) ;
#19974=CARTESIAN_POINT ( 'NONE',  ( -5.070931069364330135, 1391.839164954021044, 214.6451533971127787 ) ) ;
#19975=CARTESIAN_POINT ( 'NONE',  ( 7.156881364479999341, 1427.109882774780090, 213.1306227488589968 ) ) ;
#19980=ORIENTED_EDGE ( 'NONE', *, *, #107486, .T. ) ;
#19987=CARTESIAN_POINT ( 'NONE',  ( 8.661242571614819141, 1437.508545366829821, 209.0082535151329921 ) ) ;
#20003=CARTESIAN_POINT ( 'NONE',  ( -13.59512409120000065, 1507.703333874389955, 209.3532891412210120 ) ) ;
#20004=CARTESIAN_POINT ( 'NONE',  ( -21.30923694625010256, 1486.313822144630194, 201.8416180601869883 ) ) ;
#20009=AXIS2_PLACEMENT_3D ( 'NONE', #24068, #15654, #14578 ) ;
#20017=CARTESIAN_POINT ( 'NONE',  ( -8.468559922060000744, 1424.013193781740028, 208.6259767417379862 ) ) ;
#20021=CARTESIAN_POINT ( 'NONE',  ( -5.000000000000000000, 1391.913060387289988, 209.1218459616989946 ) ) ;
#20024=CARTESIAN_POINT ( 'NONE',  ( -1.373535289882310106, 1496.574688335899964, 221.4066534229719991 ) ) ;
#20026=CARTESIAN_POINT ( 'NONE',  ( 3.552059671762092474, 1506.620152441753362, 220.2439066918655044 ) ) ;
#20030=CARTESIAN_POINT ( 'NONE',  ( 9.269681807320001354, 1471.390733202289994, 213.6611325259989940 ) ) ;
#20031=CARTESIAN_POINT ( 'NONE',  ( 4.966881213900000702, 1424.596682296960125, 209.0258764887209963 ) ) ;
#20042=CARTESIAN_POINT ( 'NONE',  ( 11.36840161329240040, 1471.274902997630079, 210.2009342684919773 ) ) ;
#20054=CARTESIAN_POINT ( 'NONE',  ( 1.577336110359999877, 1437.553431094789858, 227.6320445992990074 ) ) ;
#20056=VERTEX_POINT ( 'NONE', #31119 ) ;
#20057=CARTESIAN_POINT ( 'NONE',  ( -4.994775864357231754, 1391.713558696120572, 214.4361776424444770 ) ) ;
#20074=CARTESIAN_POINT ( 'NONE',  ( -7.851774706560000539, 1482.164398796690193, 201.8541463733390060 ) ) ;
#20075=CARTESIAN_POINT ( 'NONE',  ( -8.864084639424179457, 1483.950334342079941, 201.1680632549600034 ) ) ;
#20079=CARTESIAN_POINT ( 'NONE',  ( -4.329407853939799544, 1515.066355634550064, 207.4272903080850199 ) ) ;
#20081=B_SPLINE_CURVE_WITH_KNOTS ( 'NONE', 3,
 ( #109076, #93897, #59776, #17162, #42402, #77129, #23928, #65985, #57578, #91704, #92255, #14977, #49172, #83304, #15525, #49721, #7153, #16076, #41309, #109615, #26698, #60895, #105077, #51923, #11571, #45748, #17721, #87741 ),
 .UNSPECIFIED., .F., .F.,
 ( 4, 3, 3, 3, 3, 3, 3, 3, 3, 4 ),
 ( 4.991132198511049722, 5.278154230586550533, 5.575591039858229792, 5.870273493069539938, 6.165162712962199976, 6.464350792949150382, 6.767514390904109334, 7.076365246789670493, 7.382407343268770461, 7.657648704760000591 ),
 .UNSPECIFIED. ) ;
#20082=CARTESIAN_POINT ( 'NONE',  ( -14.16362979129046629, 1415.677402215299935, 203.9764129101965011 ) ) ;
#20088=EDGE_LOOP ( 'NONE', ( #88431, #25951, #91521, #85168 ) ) ;
#20093=CARTESIAN_POINT ( 'NONE',  ( -1.099350364300000216, 1443.030192123389952, 200.2900125702489902 ) ) ;
#20097=CARTESIAN_POINT ( 'NONE',  ( -17.00402905897148287, 1419.970403769237919, 207.7204247156947474 ) ) ;
#20100=CARTESIAN_POINT ( 'NONE',  ( -3.744255892484579906, 1509.032043295170070, 204.8808982972809929 ) ) ;
#20102=CARTESIAN_POINT ( 'NONE',  ( 3.829620088064810801, 1515.551704408389696, 205.9132086401118897 ) ) ;
#20104=CARTESIAN_POINT ( 'NONE',  ( 1.183438229269999864, 1490.130100670090087, 188.1680879737990040 ) ) ;
#20110=VERTEX_POINT ( 'NONE', #63122 ) ;
#20111=CARTESIAN_POINT ( 'NONE',  ( -6.571754112979030893, 1508.551704408419937, 219.2970873651759973 ) ) ;
#20115=CARTESIAN_POINT ( 'NONE',  ( -0.1912754843509990033, 1484.230304989690012, 201.1822192631990163 ) ) ;
#20117=LINE ( 'NONE', #27415, #5354 ) ;
#20119=CARTESIAN_POINT ( 'NONE',  ( 0.8058879247639990639, 1431.535814502990206, 218.5910766056489933 ) ) ;
#20123=CARTESIAN_POINT ( 'NONE',  ( 17.80745809460000117, 1457.129128898490080, 217.9030147174489969 ) ) ;
#20127=CARTESIAN_POINT ( 'NONE',  ( 11.08214705546439838, 1490.840403352589874, 207.9869870122680027 ) ) ;
#20129=ORIENTED_EDGE ( 'NONE', *, *, #9071, .F. ) ;
#20131=CARTESIAN_POINT ( 'NONE',  ( 1.222757213320049940, 1496.848853757149755, 196.7997600384149735 ) ) ;
#20153=CARTESIAN_POINT ( 'NONE',  ( 3.445649996519999814, 1486.078850449689980, 219.3336985103989889 ) ) ;
#20155=DIRECTION ( 'NONE',  ( -0.8832694813677296475, 0.3761007070153973841, 0.2799701438848439250 ) ) ;
#20166=EDGE_CURVE ( 'NONE', #88852, #92278, #28023, .T. ) ;
#20174=ORIENTED_EDGE ( 'NONE', *, *, #40406, .T. ) ;
#20175=CARTESIAN_POINT ( 'NONE',  ( 2.958239116441710781, 1515.068899845850183, 213.4511871929955760 ) ) ;
#20177=ORIENTED_EDGE ( 'NONE', *, *, #27586, .F. ) ;
#20185=CARTESIAN_POINT ( 'NONE',  ( -5.969756560322280414, 1508.393149768369994, 220.0371670919589917 ) ) ;
#20187=CARTESIAN_POINT ( 'NONE',  ( -2.472525557580699918, 1469.963978788679924, 218.9232492272049910 ) ) ;
#20190=CARTESIAN_POINT ( 'NONE',  ( 2.487935123032369855, 1509.038615930399828, 204.6345961886270004 ) ) ;
#20191=CARTESIAN_POINT ( 'NONE',  ( -4.958563834310000473, 1476.141796556890085, 200.0452578302089819 ) ) ;
#20192=CARTESIAN_POINT ( 'NONE',  ( 9.432521049770000943, 1493.684480589789928, 216.5303968640490098 ) ) ;
#20194=CARTESIAN_POINT ( 'NONE',  ( 9.099391957870764713, 1425.123225031011543, 195.6134721344620573 ) ) ;
#20195=CARTESIAN_POINT ( 'NONE',  ( -19.27879749369999729, 1504.883251382790149, 209.1742019046360213 ) ) ;
#20197=CARTESIAN_POINT ( 'NONE',  ( 12.18097209163730099, 1421.739437254449967, 207.4153353150930172 ) ) ;
#20198=CARTESIAN_POINT ( 'NONE',  ( -9.888015356226818042, 1439.825890703900086, 207.5876242145089918 ) ) ;
#20206=CARTESIAN_POINT ( 'NONE',  ( 5.268140179660000477, 1505.035622830590000, 220.7476737412989962 ) ) ;
#20207=EDGE_CURVE ( 'NONE', #29796, #42338, #47859, .T. ) ;
#20209=CARTESIAN_POINT ( 'NONE',  ( 12.51870136171140047, 1421.160529832679913, 203.4347662715690035 ) ) ;
#20214=CARTESIAN_POINT ( 'NONE',  ( -6.428033936520000324, 1460.873501223489939, 208.8163193724650171 ) ) ;
#20218=CARTESIAN_POINT ( 'NONE',  ( 4.619757391858639650, 1458.438437300470241, 200.4827539045400044 ) ) ;
#20221=CARTESIAN_POINT ( 'NONE',  ( -7.980724843425534232, 1424.839191111710079, 210.5241416197258957 ) ) ;
#20232=CARTESIAN_POINT ( 'NONE',  ( 5.510910596163090542E-16, 1508.551704408389924, 204.6218459616989946 ) ) ;
#20234=CARTESIAN_POINT ( 'NONE',  ( -15.56205866169999830, 1415.965904284230191, 208.3761328791269989 ) ) ;
#20237=CARTESIAN_POINT ( 'NONE',  ( 2.031898713162200387, 1456.477761189839839, 219.5474395429129970 ) ) ;
#20238=CARTESIAN_POINT ( 'NONE',  ( 18.20258715539999983, 1429.723789929190161, 209.1218459616989946 ) ) ;
#20241=CARTESIAN_POINT ( 'NONE',  ( 5.145831880350000276, 1478.320212272790059, 199.9344042191389974 ) ) ;
#20244=CARTESIAN_POINT ( 'NONE',  ( 16.70350999062210917, 1433.635998124934986, 217.7474843568018628 ) ) ;
#20247=CARTESIAN_POINT ( 'NONE',  ( -11.77443355029789984, 1481.434860139880129, 210.4630796381239861 ) ) ;
#20251=B_SPLINE_SURFACE_WITH_KNOTS ( 'NONE', 5, 1, ( 
 ( #48766, #82892 ),
 ( #74517, #108648 ),
 ( #100251, #15118 ),
 ( #32502, #49308 ),
 ( #83434, #66672 ),
 ( #100776, #16755 ),
 ( #43658, #8377 ),
 ( #67765, #93485 ),
 ( #33030, #101878 ) ),
 .UNSPECIFIED., .F., .F., .F.,
 ( 6, 3, 6 ),
 ( 2, 2 ),
 ( 0.000000000000000000, 3.823641809439999761, 7.629352094750000646 ),
 ( 0.000000000000000000, 14.00000000000000000 ),
 .UNSPECIFIED. ) ;
#20257=CARTESIAN_POINT ( 'NONE',  ( 4.325405444010000267, 1515.219201233190006, 207.2788824862290085 ) ) ;
#20261=CARTESIAN_POINT ( 'NONE',  ( -3.975645313330000707, 1495.715016291389929, 219.5897528044989997 ) ) ;
#20263=CARTESIAN_POINT ( 'NONE',  ( -0.6279686910709979530, 1422.602376000430013, 192.9011112487989976 ) ) ;
#20266=CARTESIAN_POINT ( 'NONE',  ( 20.75865026453080020, 1455.056300995470110, 207.3304593591959986 ) ) ;
#20273=CARTESIAN_POINT ( 'NONE',  ( 5.151097723079999469, 1490.744826430290004, 188.9005472705989916 ) ) ;
#20274=CARTESIAN_POINT ( 'NONE',  ( 3.984081752359151185, 1515.551704408386513, 206.7917118350702310 ) ) ;
#20281=ORIENTED_EDGE ( 'NONE', *, *, #4245, .F. ) ;
#20285=CARTESIAN_POINT ( 'NONE',  ( 0.9514631971716608350, 1458.039373609033873, 199.6150042018308568 ) ) ;
#20289=CARTESIAN_POINT ( 'NONE',  ( 7.500000000000000000, 1391.913060387289988, 209.1218459616989946 ) ) ;
#20295=CARTESIAN_POINT ( 'NONE',  ( 9.267786286701291232, 1482.653417688600257, 214.8328156518469996 ) ) ;
#20301=CARTESIAN_POINT ( 'NONE',  ( 18.94655811398780187, 1455.761323333709925, 200.3458120453390165 ) ) ;
#20304=ORIENTED_EDGE ( 'NONE', *, *, #110696, .F. ) ;
#20308=CARTESIAN_POINT ( 'NONE',  ( 2.409034624560000282, 1511.999350511789999, 211.5308805862590020 ) ) ;
#20311=CARTESIAN_POINT ( 'NONE',  ( -1.950867193502480168, 1465.012299926070227, 198.2909385611760342 ) ) ;
#20324=EDGE_CURVE ( 'NONE', #33283, #31336, #34705, .T. ) ;
#20330=CARTESIAN_POINT ( 'NONE',  ( -6.245023087312289611, 1434.989591264769842, 216.5186931948820188 ) ) ;
#20334=CARTESIAN_POINT ( 'NONE',  ( -11.39446832680910049, 1470.674085605409800, 209.5209557487560232 ) ) ;
#20338=CARTESIAN_POINT ( 'NONE',  ( 1.835445324509999976, 1462.582348107689995, 228.7079535844989948 ) ) ;
#20344=CARTESIAN_POINT ( 'NONE',  ( 6.694003047440447496, 1452.460255165136687, 191.0903148363805713 ) ) ;
#20349=CARTESIAN_POINT ( 'NONE',  ( 9.658986663755015911, 1483.195444111240022, 213.6764680106677190 ) ) ;
#20350=CARTESIAN_POINT ( 'NONE',  ( -15.33278908930000028, 1416.031853564230005, 206.6762098088290145 ) ) ;
#20352=CARTESIAN_POINT ( 'NONE',  ( 7.406484258469999915, 1423.002001740159812, 195.5970099228989909 ) ) ;
#20355=CARTESIAN_POINT ( 'NONE',  ( -9.173420980859829044, 1449.906862649680079, 208.3877444760569801 ) ) ;
#20357=EDGE_LOOP ( 'NONE', ( #35741, #13667, #69220, #73151 ) ) ;
#20360=FACE_OUTER_BOUND ( 'NONE', #104340, .T. ) ;
#20365=CARTESIAN_POINT ( 'NONE',  ( -2.330134127310790060, 1515.064792882719985, 213.4512947379739956 ) ) ;
#20369=CARTESIAN_POINT ( 'NONE',  ( -0.4460277715470020166, 1507.325196322990223, 221.2183930200990289 ) ) ;
#20370=CARTESIAN_POINT ( 'NONE',  ( -4.327507230410000183, 1515.138937518789817, 209.8355912247540118 ) ) ;
#20374=CARTESIAN_POINT ( 'NONE',  ( 9.862537306333429399, 1469.102982438359959, 206.4340962994679956 ) ) ;
#20378=CARTESIAN_POINT ( 'NONE',  ( 3.601839739459999912, 1444.840594719589944, 200.9001243581789993 ) ) ;
#20382=B_SPLINE_SURFACE_WITH_KNOTS ( 'NONE', 5, 5, ( 
 ( #84134, #94185, #34837, #41599, #49999, #76854 ),
 ( #58952, #60068, #33178, #77403, #15265, #8522 ),
 ( #109899, #51105, #84682, #83579, #7979, #43256 ),
 ( #23677, #85230, #707, #109363, #6877, #41032 ),
 ( #165, #7434, #58404, #42699, #42146, #17454 ),
 ( #102027, #93621, #25311, #16357, #75753, #16900 ),
 ( #51653, #75210, #34287, #57860, #102571, #85792 ),
 ( #76296, #32641, #110447, #100393, #9090, #66818 ),
 ( #100919, #92529, #15797, #67369, #68468, #25865 ),
 ( #101468, #24755, #93084, #50555, #11852, #80153 ),
 ( #1821, #1255, #20234, #35957, #62858, #61190 ),
 ( #95853, #105363, #11313, #88029, #46025, #3474 ),
 ( #79625, #95307, #27000, #103129, #10760, #103700 ),
 ( #28095, #2929, #35395, #87468, #44930, #2382 ),
 ( #18567, #54435, #52762, #53322, #104257, #86898 ) ),
 .UNSPECIFIED., .F., .F., .F.,
 ( 6, 3, 3, 3, 6 ),
 ( 6, 6 ),
 ( 11.25409733830000114, 13.70140831590000019, 16.14871929349999746, 18.76186865460000064, 19.95016257009999805 ),
 ( 0.000000000000000000, 2.000000000000000000 ),
 .UNSPECIFIED. ) ;
#20387=CARTESIAN_POINT ( 'NONE',  ( -3.078888291435469604, 1508.551704408389924, 204.2041707991759836 ) ) ;
#20399=CARTESIAN_POINT ( 'NONE',  ( 7.893069735660001029, 1424.490648431219824, 211.8460496558390105 ) ) ;
#20400=CARTESIAN_POINT ( 'NONE',  ( -13.90059962640000180, 1502.276548577589892, 227.4029734405989984 ) ) ;
#20406=ORIENTED_EDGE ( 'NONE', *, *, #103603, .F. ) ;
#20411=CARTESIAN_POINT ( 'NONE',  ( -0.7790226144181949808, 1442.687261678630193, 200.2740145696140246 ) ) ;
#20432=ORIENTED_EDGE ( 'NONE', *, *, #102671, .T. ) ;
#20448=CARTESIAN_POINT ( 'NONE',  ( -4.227540919128129460, 1441.218328383909920, 201.3833897788859986 ) ) ;
#20463=CARTESIAN_POINT ( 'NONE',  ( -3.071329290860000061, 1430.205168262290044, 201.3670139598289950 ) ) ;
#20481=CARTESIAN_POINT ( 'NONE',  ( 0.2640960436329990446, 1443.540049495290077, 218.1738625233489870 ) ) ;
#20490=CARTESIAN_POINT ( 'NONE',  ( -10.14920533236069922, 1472.521211810800196, 209.9706665395110292 ) ) ;
#20497=CARTESIAN_POINT ( 'NONE',  ( -3.652869222000000082, 1484.340012570490217, 198.9077488943989920 ) ) ;
#20498=CARTESIAN_POINT ( 'NONE',  ( -16.70830179842720042, 1417.149226859160080, 207.3570905742490140 ) ) ;
#20501=B_SPLINE_SURFACE_WITH_KNOTS ( 'NONE', 5, 5, ( 
 ( #4732, #32528, #85667, #43138, #7321, #33601, #100808, #59954, #67796 ),
 ( #41484, #67250, #23559, #109244, #40916, #50988, #57751, #66700, #24096 ),
 ( #75645, #41, #92410, #49335, #6756, #76179, #42577, #101906, #93513 ),
 ( #25198, #34172, #100279, #58285, #15682, #49887, #84020, #8967, #24636 ),
 ( #58833, #77296, #110328, #102464, #91871, #59401, #109784, #594, #33062 ),
 ( #92970, #101345, #15145, #16785, #83461, #85117, #8405, #16242, #50447 ),
 ( #17339, #84571, #7863, #76728, #68358, #25754, #94070, #51533, #75096 ),
 ( #42030, #34722, #9518, #79503, #70569, #44806, #88447, #28537, #70022 ),
 ( #80042, #53775, #26310, #11737, #52096, #78390, #2266, #94624, #95738 ) ),
 .UNSPECIFIED., .F., .F., .F.,
 ( 6, 3, 6 ),
 ( 6, 3, 6 ),
 ( 3.281786719996299784, 5.680069915599999852, 8.078356001358638849 ),
 ( -0.0002330648786371619999, 1.500000000000000000, 3.000000000000000000 ),
 .UNSPECIFIED. ) ;
#20502=FACE_OUTER_BOUND ( 'NONE', #51284, .T. ) ;
#20504=CARTESIAN_POINT ( 'NONE',  ( -7.652581619519890133, 1489.002915072239830, 217.1598258052599988 ) ) ;
#20505=CARTESIAN_POINT ( 'NONE',  ( -13.05160936328820043, 1467.538640410949938, 191.8992777555500311 ) ) ;
#20510=CARTESIAN_POINT ( 'NONE',  ( -18.70251467970079773, 1443.789633783120053, 211.1888656691189965 ) ) ;
#20515=EDGE_LOOP ( 'NONE', ( #91362, #58291, #84378, #59955 ) ) ;
#20531=CARTESIAN_POINT ( 'NONE',  ( -0.5084571940651050337, 1515.143473212400067, 213.4492344207059773 ) ) ;
#20532=CARTESIAN_POINT ( 'NONE',  ( 11.39903530061180170, 1471.112746094619979, 209.6182361319149834 ) ) ;
#20533=CARTESIAN_POINT ( 'NONE',  ( -5.113737714138570034, 1477.155299723150165, 219.4578886346909883 ) ) ;
#20534=AXIS2_PLACEMENT_3D ( 'NONE', #102580, #25322, #84144 ) ;
#20540=CARTESIAN_POINT ( 'NONE',  ( -17.66645871475320106, 1487.819326808810047, 195.0539618811440050 ) ) ;
#20548=FACE_OUTER_BOUND ( 'NONE', #87581, .T. ) ;
#20555=APPLICATION_CONTEXT ( 'automotive_design' ) ;
#20556=CARTESIAN_POINT ( 'NONE',  ( -10.56464281290000073, 1472.012291739390093, 204.5722061169090011 ) ) ;
#20566=CARTESIAN_POINT ( 'NONE',  ( -8.739857391529799457, 1438.983306933739868, 207.6178224853659913 ) ) ;
#20576=CARTESIAN_POINT ( 'NONE',  ( -1.703340611422059947, 1467.868438609650184, 220.1112480085430150 ) ) ;
#20578=CARTESIAN_POINT ( 'NONE',  ( 7.520437383334657611, 1472.270029459488796, 190.3424407131327882 ) ) ;
#20579=LINE ( 'NONE', #106266, #101944 ) ;
#20595=CARTESIAN_POINT ( 'NONE',  ( -8.320994297830779374, 1422.937291762959831, 213.3671062650610111 ) ) ;
#20597=CARTESIAN_POINT ( 'NONE',  ( 9.674066812699999574, 1488.345346575790018, 203.9346639274390043 ) ) ;
#20598=FACE_OUTER_BOUND ( 'NONE', #6511, .T. ) ;
#20599=ADVANCED_FACE ( 'NONE', ( #54843 ), #70344, .T. ) ;
#20601=EDGE_CURVE ( 'NONE', #75158, #88376, #11971, .T. ) ;
#20611=CARTESIAN_POINT ( 'NONE',  ( 19.09907639360000076, 1458.161943520289924, 212.8891023046390103 ) ) ;
#20617=CARTESIAN_POINT ( 'NONE',  ( -9.519205059868689034, 1460.476570792010079, 210.7622160576040073 ) ) ;
#20626=EDGE_CURVE ( 'NONE', #15891, #3640, #94868, .T. ) ;
#20631=EDGE_CURVE ( 'NONE', #103706, #68962, #48063, .T. ) ;
#20634=CARTESIAN_POINT ( 'NONE',  ( 3.208637255279672473, 1515.551704408389696, 205.2922258088532317 ) ) ;
#20641=CARTESIAN_POINT ( 'NONE',  ( -4.958565512799999908, 1476.141795141989860, 200.0452582524689831 ) ) ;
#20643=ORIENTED_EDGE ( 'NONE', *, *, #89094, .T. ) ;
#20644=CARTESIAN_POINT ( 'NONE',  ( -19.04698019608209947, 1444.155722059970003, 199.5979690564769840 ) ) ;
#20650=CARTESIAN_POINT ( 'NONE',  ( -5.523724626499999957, 1462.904961658189904, 201.0501093365290046 ) ) ;
#20652=CARTESIAN_POINT ( 'NONE',  ( -2.944617142229999818, 1431.901135818789953, 217.0105143139790016 ) ) ;
#20660=CARTESIAN_POINT ( 'NONE',  ( 10.92860598996890076, 1490.384399647580040, 208.1271090416140055 ) ) ;
#20666=CARTESIAN_POINT ( 'NONE',  ( 1.559621619610169985, 1496.922908498869901, 196.8322261072790127 ) ) ;
#20676=EDGE_CURVE ( 'NONE', #2790, #97980, #62778, .T. ) ;
#20692=CARTESIAN_POINT ( 'NONE',  ( -3.665756888920000289, 1509.051704408389924, 214.1089243971590008 ) ) ;
#20695=CARTESIAN_POINT ( 'NONE',  ( -5.199570078000000706, 1391.913060387289988, 214.4361776263990009 ) ) ;
#20702=ORIENTED_EDGE ( 'NONE', *, *, #43903, .T. ) ;
#20703=CARTESIAN_POINT ( 'NONE',  ( 10.55407258484730093, 1452.751878998079974, 209.9968945314950020 ) ) ;
#20707=DIRECTION ( 'NONE',  ( -0.02616798426500960631, -0.9993150019883682011, 0.02616798426500980407 ) ) ;
#20708=CARTESIAN_POINT ( 'NONE',  ( 5.893213018790000035, 1451.599863458789969, 210.6385936290390077 ) ) ;
#20711=CARTESIAN_POINT ( 'NONE',  ( 3.252451448209999985, 1444.627347679690047, 200.7572266927390103 ) ) ;
#20724=ORIENTED_EDGE ( 'NONE', *, *, #51714, .F. ) ;
#20726=CARTESIAN_POINT ( 'NONE',  ( -2.710244495734679848, 1508.047929154919984, 220.9036545897700137 ) ) ;
#20727=CARTESIAN_POINT ( 'NONE',  ( 3.862810189448820264, 1497.382634203200041, 197.2226424524940285 ) ) ;
#20729=CARTESIAN_POINT ( 'NONE',  ( -5.795766362228450319, 1469.762611321129953, 217.6224603134940025 ) ) ;
#20731=CARTESIAN_POINT ( 'NONE',  ( 9.225579725230000250, 1420.892510935600058, 196.8152382223989889 ) ) ;
#20732=CARTESIAN_POINT ( 'NONE',  ( 1.106948036398740065, 1475.016812829990158, 220.4877511142580033 ) ) ;
#20736=CARTESIAN_POINT ( 'NONE',  ( -14.24321357380000030, 1503.441202237889911, 208.7621914785800072 ) ) ;
#20746=CARTESIAN_POINT ( 'NONE',  ( 17.78284146230000218, 1432.724246433989947, 213.5810953123289835 ) ) ;
#20750=ORIENTED_EDGE ( 'NONE', *, *, #69410, .F. ) ;
#20755=CARTESIAN_POINT ( 'NONE',  ( -2.480175250669919951, 1429.207669930499833, 200.0830571243679969 ) ) ;
#20759=CARTESIAN_POINT ( 'NONE',  ( 8.884591108237419377, 1458.997830223579967, 202.8087305887910077 ) ) ;
#20762=CARTESIAN_POINT ( 'NONE',  ( -5.573872061590000371, 1477.238916206189970, 218.8617125876789942 ) ) ;
#20772=CARTESIAN_POINT ( 'NONE',  ( -14.33027067026050005, 1416.949084347329972, 203.2389326530310143 ) ) ;
#20776=CARTESIAN_POINT ( 'NONE',  ( 8.900418934672700289, 1428.280648177160174, 213.0365380470040009 ) ) ;
#20777=CARTESIAN_POINT ( 'NONE',  ( -4.290508133339999475, 1515.379316001789903, 208.7552447710999957 ) ) ;
#20778=EDGE_CURVE ( 'NONE', #72498, #43776, #13934, .T. ) ;
#20784=CARTESIAN_POINT ( 'NONE',  ( 3.029075602040000259, 1477.864648017889749, 199.0898650909989840 ) ) ;
#20786=CARTESIAN_POINT ( 'NONE',  ( -17.14873022714438378, 1468.567877217461501, 198.7365958164457993 ) ) ;
#20791=CARTESIAN_POINT ( 'NONE',  ( -11.69922274234029835, 1481.273184454980083, 210.9363146797530248 ) ) ;
#20797=CARTESIAN_POINT ( 'NONE',  ( -3.660886842309849953, 1508.551704408389924, 204.4275887013349973 ) ) ;
#20799=EDGE_CURVE ( 'NONE', #95904, #30629, #90894, .T. ) ;
#20803=VECTOR ( 'NONE', #29618, 1000.000000000000114 ) ;
#20804=CARTESIAN_POINT ( 'NONE',  ( -0.8241248838030009738, 1509.075058821990069, 218.0915817195690067 ) ) ;
#20813=CARTESIAN_POINT ( 'NONE',  ( -18.51202227299100045, 1466.632449115480085, 200.9222626566809993 ) ) ;
#20820=CARTESIAN_POINT ( 'NONE',  ( -234.5897387251999930, 11221.53578756869865, 2175.945776423289772 ) ) ;
#20826=CARTESIAN_POINT ( 'NONE',  ( -16.76078030769999927, 1420.494757909599912, 203.1294657649889928 ) ) ;
#20829=CARTESIAN_POINT ( 'NONE',  ( -9.148257661150001496, 1423.748799908730007, 207.7944249153989915 ) ) ;
#20836=CARTESIAN_POINT ( 'NONE',  ( -0.8838665694872513967, 1457.292915820307371, 199.6410733348866415 ) ) ;
#20842=CARTESIAN_POINT ( 'NONE',  ( -1.431441865960000115, 1468.042762720489918, 219.7628109989989866 ) ) ;
#20844=CARTESIAN_POINT ( 'NONE',  ( 9.329257343867968899, 1483.543149501509788, 214.5330026594239996 ) ) ;
#20849=CARTESIAN_POINT ( 'NONE',  ( -2.515613294380000031, 1448.349718812090032, 188.5842421506989979 ) ) ;
#20850=CARTESIAN_POINT ( 'NONE',  ( -2.542680546169759914, 1431.030268854349970, 201.1441491798630068 ) ) ;
#20853=ORIENTED_EDGE ( 'NONE', *, *, #63909, .T. ) ;
#20858=CARTESIAN_POINT ( 'NONE',  ( 0.000000000000000000, 1420.584111001019892, 209.1218459616989946 ) ) ;
#20859=CARTESIAN_POINT ( 'NONE',  ( 11.45444494140000025, 1502.281967335889931, 208.2980153205920146 ) ) ;
#20863=CARTESIAN_POINT ( 'NONE',  ( -0.6779417998419989821, 1464.763158441590122, 198.8934648891990093 ) ) ;
#20871=CARTESIAN_POINT ( 'NONE',  ( 11.26937486967429969, 1478.652699849539886, 205.8601904136019982 ) ) ;
#20878=CARTESIAN_POINT ( 'NONE',  ( -9.014963715518330645, 1437.210665075589986, 213.0690570958229841 ) ) ;
#20882=CARTESIAN_POINT ( 'NONE',  ( -6.349044579700000135, 1508.776756645290106, 219.5917579706989784 ) ) ;
#20896=CARTESIAN_POINT ( 'NONE',  ( 8.416897302759883459, 1484.129603243253086, 215.7648255120577687 ) ) ;
#20897=CARTESIAN_POINT ( 'NONE',  ( -14.87384579849999966, 1416.121162261860036, 204.9838385039689683 ) ) ;
#20908=CARTESIAN_POINT ( 'NONE',  ( -0.008119676937300529876, 1515.178500008189985, 213.4483172118689822 ) ) ;
#20916=ADVANCED_FACE ( 'NONE', ( #28256 ), #96243, .T. ) ;
#20917=CARTESIAN_POINT ( 'NONE',  ( 10.78159844869479933, 1461.896569297480028, 211.1674770051990038 ) ) ;
#20921=VERTEX_POINT ( 'NONE', #77568 ) ;
#20923=CARTESIAN_POINT ( 'NONE',  ( 6.762278413896400053, 1467.457330156850048, 200.6363351971689895 ) ) ;
#20927=CARTESIAN_POINT ( 'NONE',  ( 7.000633479060000219, 1424.213547369589833, 212.7272991732289995 ) ) ;
#20931=CARTESIAN_POINT ( 'NONE',  ( 12.29186695254770001, 1491.851815450179856, 208.3259444585769984 ) ) ;
#20939=CARTESIAN_POINT ( 'NONE',  ( -4.660393612750000081, 1436.848553822789881, 227.0391165213990234 ) ) ;
#20940=CARTESIAN_POINT ( 'NONE',  ( -15.58456279011612544, 1415.964423084322789, 207.9695922479936030 ) ) ;
#20947=CARTESIAN_POINT ( 'NONE',  ( 7.422111136049999836, 1427.425960435760089, 212.9291018486189841 ) ) ;
#20956=ORIENTED_EDGE ( 'NONE', *, *, #15331, .F. ) ;
#20976=ORIENTED_EDGE ( 'NONE', *, *, #44595, .T. ) ;
#20978=CARTESIAN_POINT ( 'NONE',  ( 10.93679547204000002, 1490.434980368090010, 209.9321327948960061 ) ) ;
#20983=EDGE_LOOP ( 'NONE', ( #72684, #32704, #44253, #74385 ) ) ;
#21005=CARTESIAN_POINT ( 'NONE',  ( 15.42100696471130128, 1427.564330775570170, 199.6300130664099868 ) ) ;
#21017=CARTESIAN_POINT ( 'NONE',  ( 11.46412257490000108, 1426.137423974189915, 205.4576714340990122 ) ) ;
#21020=CARTESIAN_POINT ( 'NONE',  ( -16.54876248606459299, 1416.988855567187784, 207.7154296687141084 ) ) ;
#21024=ORIENTED_EDGE ( 'NONE', *, *, #18526, .T. ) ;
#21030=CARTESIAN_POINT ( 'NONE',  ( 8.033566663349164472, 1423.901403140259163, 195.8561929068294774 ) ) ;
#21031=PRODUCT_DEFINITION_CONTEXT ( 'detailed design', #20555, 'design' ) ;
#21032=CARTESIAN_POINT ( 'NONE',  ( 2.194612407920000230, 1441.754231285490050, 218.8080856977990152 ) ) ;
#21041=CARTESIAN_POINT ( 'NONE',  ( -9.808790059567231268, 1472.102509068790141, 211.8008741836299862 ) ) ;
#21044=CARTESIAN_POINT ( 'NONE',  ( -13.22667534600000216, 1508.519311693090003, 216.8816497979790086 ) ) ;
#21045=B_SPLINE_CURVE_WITH_KNOTS ( 'NONE', 5,
 ( #81992, #31597, #55734, #12050, #73067, #54636 ),
 .UNSPECIFIED., .F., .F.,
 ( 6, 6 ),
 ( 434.2407011939999961, 439.4753079239999920 ),
 .UNSPECIFIED. ) ;
#21047=VECTOR ( 'NONE', #6509, 1000.000000000000000 ) ;
#21054=CARTESIAN_POINT ( 'NONE',  ( 3.210133688000829988, 1493.596834919620051, 219.7945351484260073 ) ) ;
#21055=CARTESIAN_POINT ( 'NONE',  ( -5.221941033162339707, 1489.269461032029767, 185.8916498237339852 ) ) ;
#21056=CARTESIAN_POINT ( 'NONE',  ( -14.55544240679570045, 1415.677402205800036, 205.6845489372280156 ) ) ;
#21061=EDGE_LOOP ( 'NONE', ( #79972, #1587, #40644, #52689 ) ) ;
#21069=CARTESIAN_POINT ( 'NONE',  ( 7.868158389100000427, 1422.937290482379922, 214.1570520181289794 ) ) ;
#21080=CARTESIAN_POINT ( 'NONE',  ( -0.2472019593338070087, 1515.155075545679892, 213.4489306029969953 ) ) ;
#21082=CARTESIAN_POINT ( 'NONE',  ( -10.27310637450800002, 1479.785839561440071, 214.7842258919359892 ) ) ;
#21087=CARTESIAN_POINT ( 'NONE',  ( -12.20494468169999891, 1503.566125598490089, 208.5052328696230006 ) ) ;
#21089=CARTESIAN_POINT ( 'NONE',  ( -11.64556911059999855, 1484.153277220190148, 228.3908460861989909 ) ) ;
#21094=CARTESIAN_POINT ( 'NONE',  ( 4.327218846664220742, 1515.149950449760127, 209.5076553614100021 ) ) ;
#21102=ORIENTED_EDGE ( 'NONE', *, *, #61460, .F. ) ;
#21105=CARTESIAN_POINT ( 'NONE',  ( -9.191661361731490842, 1447.246705968339938, 212.1312239747880142 ) ) ;
#21113=CARTESIAN_POINT ( 'NONE',  ( -5.144873395449999443, 1502.885538352589947, 229.8910404859989853 ) ) ;
#21117=CARTESIAN_POINT ( 'NONE',  ( 8.822677033039550309, 1435.308442571839805, 207.3766048290129902 ) ) ;
#21120=ORIENTED_EDGE ( 'NONE', *, *, #125, .T. ) ;
#21122=CARTESIAN_POINT ( 'NONE',  ( -1.419179629244010199, 1467.807880198409975, 220.1457629506999751 ) ) ;
#21134=EDGE_LOOP ( 'NONE', ( #102173, #18097, #61819, #72302, #33327 ) ) ;
#21135=CARTESIAN_POINT ( 'NONE',  ( -4.367937192439999450, 1447.898255911189835, 190.6350925615990093 ) ) ;
#21136=CARTESIAN_POINT ( 'NONE',  ( -5.102340803919999779, 1483.010473641589897, 199.7820758705289848 ) ) ;
#21163=CARTESIAN_POINT ( 'NONE',  ( 11.23090178780859993, 1499.222069974919805, 203.1659750294479920 ) ) ;
#21165=CARTESIAN_POINT ( 'NONE',  ( 11.76012779522459972, 1479.338680739629808, 208.6262329665489972 ) ) ;
#21173=CARTESIAN_POINT ( 'NONE',  ( -2.487923653944299929, 1509.038644359520049, 204.6345969248399967 ) ) ;
#21180=CARTESIAN_POINT ( 'NONE',  ( -3.453907602370000163, 1475.036073752090033, 198.6389954596989753 ) ) ;
#21184=CARTESIAN_POINT ( 'NONE',  ( -18.65942656951699874, 1468.219847912240084, 201.0822107266409944 ) ) ;
#21187=CARTESIAN_POINT ( 'NONE',  ( 15.41142278176256575, 1416.181292664740113, 209.1057902910335997 ) ) ;
#21191=CARTESIAN_POINT ( 'NONE',  ( -10.14235463135029924, 1472.524663116719921, 207.2163364872419891 ) ) ;
#21202=CARTESIAN_POINT ( 'NONE',  ( -18.74729292449999818, 1442.199705176290081, 209.1218459616989946 ) ) ;
#21203=CARTESIAN_POINT ( 'NONE',  ( 2.196337318485120260, 1497.056153613870038, 196.9180676716810012 ) ) ;
#21204=CARTESIAN_POINT ( 'NONE',  ( 12.55930903091550022, 1420.665439290649829, 201.1166257793219927 ) ) ;
#21212=ADVANCED_FACE ( 'NONE', ( #49481 ), #88219, .T. ) ;
#21218=CARTESIAN_POINT ( 'NONE',  ( 1.101790807069999989, 1496.828157016689829, 196.7632638577989894 ) ) ;
#21230=CARTESIAN_POINT ( 'NONE',  ( -0.09768190207400140324, 1486.875687893489840, 220.0842578668990086 ) ) ;
#21236=CARTESIAN_POINT ( 'NONE',  ( -4.326079330693803016, 1515.193466806617153, 206.7917118350173382 ) ) ;
#21239=CARTESIAN_POINT ( 'NONE',  ( 10.53595400140370053, 1452.843899432660010, 210.2517208858830031 ) ) ;
#21242=CARTESIAN_POINT ( 'NONE',  ( -2.762222941174190094, 1441.249766939880146, 203.6130042841640204 ) ) ;
#21243=DIRECTION ( 'NONE',  ( 0.1362866687051670078, -0.4503100534970719271, 0.8824096552354309120 ) ) ;
#21246=ORIENTED_EDGE ( 'NONE', *, *, #4050, .T. ) ;
#21254=CARTESIAN_POINT ( 'NONE',  ( 8.824912719755909407, 1482.390745019529959, 216.9842546517499784 ) ) ;
#21258=ORIENTED_EDGE ( 'NONE', *, *, #245, .F. ) ;
#21259=CARTESIAN_POINT ( 'NONE',  ( -11.88114669040890092, 1481.846449482240132, 209.1712150661669796 ) ) ;
#21260=ADVANCED_FACE ( 'NONE', ( #85254 ), #71261, .T. ) ;
#21263=B_SPLINE_CURVE_WITH_KNOTS ( 'NONE', 5,
 ( #77803, #76691, #59366, #3, #86193, #26275 ),
 .UNSPECIFIED., .F., .F.,
 ( 6, 6 ),
 ( 0.000000000000000000, 1.000000000000000000 ),
 .UNSPECIFIED. ) ;
#21265=CARTESIAN_POINT ( 'NONE',  ( -3.048199684790729780, 1468.133964442819888, 219.8853629577970139 ) ) ;
#21267=CARTESIAN_POINT ( 'NONE',  ( 8.315094184529998600, 1421.392059295079889, 196.2232414242990046 ) ) ;
#21275=CARTESIAN_POINT ( 'NONE',  ( 11.42187775320380005, 1422.318575770460029, 207.1307412838170023 ) ) ;
#21277=B_SPLINE_CURVE_WITH_KNOTS ( 'NONE', 5,
 ( #38835, #31541, #80860, #91461, #57335, #55131 ),
 .UNSPECIFIED., .F., .F.,
 ( 6, 6 ),
 ( -2.000000000000000000, 0.000000000000000000 ),
 .UNSPECIFIED. ) ;
#21281=DIRECTION ( 'NONE',  ( -1.000000000000000000, 0.000000000000000000, 0.000000000000000000 ) ) ;
#21285=CARTESIAN_POINT ( 'NONE',  ( -15.47916639359999991, 1416.003150712520210, 210.9846457611390065 ) ) ;
#21287=CARTESIAN_POINT ( 'NONE',  ( -15.88906974165360175, 1420.257646009350083, 209.8690693256239967 ) ) ;
#21289=CARTESIAN_POINT ( 'NONE',  ( 3.959152859930000101, 1428.396642669490120, 216.3690266601789745 ) ) ;
#21293=CARTESIAN_POINT ( 'NONE',  ( -1.860819933241510071, 1429.530525759420243, 199.9260310902689923 ) ) ;
#21297=FACE_OUTER_BOUND ( 'NONE', #63726, .T. ) ;
#21310=AXIS2_PLACEMENT_3D ( 'NONE', #89915, #12109, #46302 ) ;
#21318=CARTESIAN_POINT ( 'NONE',  ( -0.07406262508839699110, 1484.296809990774818, 198.4210634843702508 ) ) ;
#21322=VERTEX_POINT ( 'NONE', #12420 ) ;
#21323=CARTESIAN_POINT ( 'NONE',  ( 4.049945658389999537, 1478.539621255289831, 199.3912200899090124 ) ) ;
#21331=CARTESIAN_POINT ( 'NONE',  ( -19.97968237250000101, 1483.906011188890034, 214.0068283976289933 ) ) ;
#21336=CARTESIAN_POINT ( 'NONE',  ( -4.979503507856909650, 1508.551704408389924, 206.4216282949940364 ) ) ;
#21339=CARTESIAN_POINT ( 'NONE',  ( 5.059013353549999259, 1501.257177412389865, 229.8390314845989906 ) ) ;
#21344=CARTESIAN_POINT ( 'NONE',  ( -3.907660151049999975, 1495.688198251490121, 219.6140096315990036 ) ) ;
#21350=CARTESIAN_POINT ( 'NONE',  ( -19.64813173790599876, 1466.604908830560134, 204.2400468754019869 ) ) ;
#21363=CARTESIAN_POINT ( 'NONE',  ( -9553.690947211385719, 5182.767774292097783, 845.7647807759669831 ) ) ;
#21378=CARTESIAN_POINT ( 'NONE',  ( -0.4528338272850009893, 1469.497291256290055, 219.1901816671989991 ) ) ;
#21380=CARTESIAN_POINT ( 'NONE',  ( 9.978765032700469106, 1482.348874302069817, 212.8318254667499900 ) ) ;
#21386=CARTESIAN_POINT ( 'NONE',  ( 18.28863001267049881, 1430.119171029580002, 201.0315453683600140 ) ) ;
#21398=CARTESIAN_POINT ( 'NONE',  ( -1.157238773510000041, 1464.257248818090147, 199.2213037580589798 ) ) ;
#21405=EDGE_LOOP ( 'NONE', ( #83805, #98486, #73894, #88233 ) ) ;
#21407=B_SPLINE_CURVE_WITH_KNOTS ( 'NONE', 3,
 ( #96211, #13277, #12193, #4895, #63199, #20576, #105729, #21122, #81591, #19486, #2729, #97306, #97846, #55327, #79418, #12752, #53689, #55881, #45279, #27902, #71043, #11653, #90002, #46386, #39035, #105165, #89459, #11119, #3279, #36851, #79962, #80518, #47469, #104609, #3835, #96772, #71608 ),
 .UNSPECIFIED., .F., .F.,
 ( 4, 3, 3, 3, 3, 3, 3, 3, 3, 3, 3, 3, 4 ),
 ( -11.90357780880000149, -11.65138654548870001, -10.97030762600710041, -10.24753412388749929, -9.484849656234679571, -8.666253744101309664, -7.699452457123720173, -6.772837301347459871, -5.935629956368320137, -5.021959782221260049, -4.226855386626629851, -3.539500458311259479, -2.894173653930000256 ),
 .UNSPECIFIED. ) ;
#21410=VERTEX_POINT ( 'NONE', #9948 ) ;
#21414=CARTESIAN_POINT ( 'NONE',  ( -9.783936650027678539, 1438.409968310599879, 210.7790528106160082 ) ) ;
#21430=CARTESIAN_POINT ( 'NONE',  ( -15.52294138480000107, 1421.387829696419885, 199.5510885761390227 ) ) ;
#21436=CARTESIAN_POINT ( 'NONE',  ( -15.22768491250000089, 1415.677402202029953, 208.4617985024749771 ) ) ;
#21439=EDGE_CURVE ( 'NONE', #52400, #10255, #63939, .T. ) ;
#21443=CARTESIAN_POINT ( 'NONE',  ( 6.483588104269999874, 1462.707724100489941, 208.1814389384059893 ) ) ;
#21448=CARTESIAN_POINT ( 'NONE',  ( 0.7442430207950000431, 1515.589102391990082, 213.1386578140389929 ) ) ;
#21452=B_SPLINE_CURVE_WITH_KNOTS ( 'NONE', 3,
 ( #56923, #101639, #76466, #32799, #24928, #83762, #58028, #58578, #50715, #74286, #32261, #6504, #110068, #8145, #99445, #49080, #59138, #5959, #91612 ),
 .UNSPECIFIED., .F., .F.,
 ( 4, 3, 3, 3, 3, 3, 4 ),
 ( -24.12443845425489997, -23.98402014143189831, -23.65737981169450066, -23.29041649494190125, -22.85542232492040071, -22.35670583347129892, -21.97924354190000074 ),
 .UNSPECIFIED. ) ;
#21453=CARTESIAN_POINT ( 'NONE',  ( -10.32838887772869896, 1447.694493972999908, 209.8647986237220096 ) ) ;
#21459=CARTESIAN_POINT ( 'NONE',  ( -4.328507561560000383, 1515.100736413590084, 210.1977440287089962 ) ) ;
#21463=B_SPLINE_CURVE_WITH_KNOTS ( 'NONE', 3,
 ( #27520, #71214, #61705, #105336, #70670, #80128, #45456, #95827, #3447, #79598, #19095, #2902, #28627 ),
 .UNSPECIFIED., .F., .F.,
 ( 4, 3, 3, 3, 4 ),
 ( -1.149508497110000027, -0.3382834629707950347, 0.4737402652647237922, 1.287219781555279718, 1.586334299330000031 ),
 .UNSPECIFIED. ) ;
#21479=CARTESIAN_POINT ( 'NONE',  ( -11.33250792936460805, 1503.032974060135075, 207.0697244187343529 ) ) ;
#21480=CARTESIAN_POINT ( 'NONE',  ( -13.58435925944560196, 1508.516896892319892, 210.0765856309430148 ) ) ;
#21485=CARTESIAN_POINT ( 'NONE',  ( -6.991531664970000115, 1452.433546631890067, 202.2220901360489904 ) ) ;
#21486=EDGE_CURVE ( 'NONE', #108761, #31410, #54740, .T. ) ;
#21489=CARTESIAN_POINT ( 'NONE',  ( 7.799720914009999895, 1426.519650413049931, 211.9402747548089678 ) ) ;
#21490=CARTESIAN_POINT ( 'NONE',  ( 10.99043244679999987, 1479.494642110589893, 229.8297439418990109 ) ) ;
#21495=CARTESIAN_POINT ( 'NONE',  ( 8.225616979109998894, 1452.226705206789802, 213.5360760307489727 ) ) ;
#21496=EDGE_LOOP ( 'NONE', ( #9425, #99335, #107600, #49653 ) ) ;
#21510=CARTESIAN_POINT ( 'NONE',  ( -2.205815343605610046, 1463.135290986430164, 199.5903874811000094 ) ) ;
#21520=VERTEX_POINT ( 'NONE', #63159 ) ;
#21527=ORIENTED_EDGE ( 'NONE', *, *, #11724, .T. ) ;
#21528=CARTESIAN_POINT ( 'NONE',  ( -17.39923563954690167, 1508.493391337249932, 212.6342160743549812 ) ) ;
#21533=VERTEX_POINT ( 'NONE', #19441 ) ;
#21542=EDGE_LOOP ( 'NONE', ( #34998, #18167, #48146, #70745 ) ) ;
#21546=CARTESIAN_POINT ( 'NONE',  ( 21.02430346220000246, 1494.771309273490033, 208.1582823273150211 ) ) ;
#21553=EDGE_CURVE ( 'NONE', #72498, #102504, #87260, .T. ) ;
#21569=CARTESIAN_POINT ( 'NONE',  ( 4.900006679340000559, 1499.255191946190052, 229.7873568473989963 ) ) ;
#21570=CARTESIAN_POINT ( 'NONE',  ( 11.23526700939999934, 1422.470850597359913, 204.4982669692790012 ) ) ;
#21572=VECTOR ( 'NONE', #55002, 1000.000000000000227 ) ;
#21574=CARTESIAN_POINT ( 'NONE',  ( -15.98206112875141827, 1416.141927088484408, 209.1311918923094879 ) ) ;
#21576=CARTESIAN_POINT ( 'NONE',  ( 10.10258394918160008, 1469.588079192369833, 207.6910948265980039 ) ) ;
#21579=EDGE_CURVE ( 'NONE', #54902, #10255, #71029, .T. ) ;
#21585=CARTESIAN_POINT ( 'NONE',  ( 7.972851048953825348, 1423.800244593099478, 195.8527174153489057 ) ) ;
#21587=CARTESIAN_POINT ( 'NONE',  ( 2.539157280710000020, 1443.442079612289945, 217.6697438749490061 ) ) ;
#21590=CARTESIAN_POINT ( 'NONE',  ( 18.99535453092520143, 1472.738766242029897, 202.2605984988649936 ) ) ;
#21592=CARTESIAN_POINT ( 'NONE',  ( 6.460996930076231770, 1486.649525340193122, 200.4524504349261633 ) ) ;
#21600=CARTESIAN_POINT ( 'NONE',  ( -14.42661198839999948, 1508.520312169789804, 215.9309591648589901 ) ) ;
#21602=CARTESIAN_POINT ( 'NONE',  ( 11.13973213087689906, 1470.272412021129867, 206.9146623043149873 ) ) ;
#21608=CARTESIAN_POINT ( 'NONE',  ( 3.746245303161040319, 1495.153263702249888, 220.4845792887770131 ) ) ;
#21609=CARTESIAN_POINT ( 'NONE',  ( -5.586162938070000195, 1491.245995699590139, 185.8699225748990216 ) ) ;
#21613=VERTEX_POINT ( 'NONE', #100560 ) ;
#21623=CARTESIAN_POINT ( 'NONE',  ( 9.756688738945658912, 1436.057734518939924, 210.3833036739349893 ) ) ;
#21629=CARTESIAN_POINT ( 'NONE',  ( 1.324264359491340137, 1515.084669001950033, 213.4507742627420157 ) ) ;
#21631=CARTESIAN_POINT ( 'NONE',  ( -10.12731387375120029, 1479.682647925139918, 215.0256783668529863 ) ) ;
#21632=AXIS2_PLACEMENT_3D ( 'NONE', #110085, #42890, #42328 ) ;
#21638=CARTESIAN_POINT ( 'NONE',  ( -11.79691506120000000, 1504.510891942089984, 208.2439356722240120 ) ) ;
#21639=CARTESIAN_POINT ( 'NONE',  ( -5.695425083339999972, 1491.838932079990172, 185.8634046642990256 ) ) ;
#21641=CARTESIAN_POINT ( 'NONE',  ( 7.854071199910000800, 1421.721864916329878, 195.9105866898989916 ) ) ;
#21645=CARTESIAN_POINT ( 'NONE',  ( 4.099884065022929569, 1484.480468068710024, 220.2376187541709953 ) ) ;
#21647=CARTESIAN_POINT ( 'NONE',  ( -5.637866616400000197, 1457.357056849289847, 216.8187349542390052 ) ) ;
#21650=ORIENTED_EDGE ( 'NONE', *, *, #41252, .T. ) ;
#21655=CARTESIAN_POINT ( 'NONE',  ( -8.557209110492459914, 1448.617779613390212, 212.3361752075699940 ) ) ;
#21657=SURFACE_STYLE_USAGE ( .BOTH. , #98386 ) ;
#21667=VECTOR ( 'NONE', #98996, 1000.000000000000114 ) ;
#21672=ORIENTED_EDGE ( 'NONE', *, *, #20626, .F. ) ;
#21675=CARTESIAN_POINT ( 'NONE',  ( -2.311558444226220033, 1425.028861818389942, 191.2692960788320136 ) ) ;
#21681=EDGE_CURVE ( 'NONE', #88376, #32787, #110623, .T. ) ;
#21686=ORIENTED_EDGE ( 'NONE', *, *, #74031, .F. ) ;
#21694=CARTESIAN_POINT ( 'NONE',  ( -16.82269271239999853, 1418.343879150699877, 203.5371288789889945 ) ) ;
#21705=CARTESIAN_POINT ( 'NONE',  ( -4.878146142590000345, 1474.403035727189945, 198.7818668649990173 ) ) ;
#21709=EDGE_CURVE ( 'NONE', #110516, #345, #30600, .T. ) ;
#21716=CARTESIAN_POINT ( 'NONE',  ( -10.19612387162210076, 1470.689520798050125, 211.8176239230739952 ) ) ;
#21720=CARTESIAN_POINT ( 'NONE',  ( 11.77531401088269902, 1479.418202641479866, 208.9148487659819864 ) ) ;
#21725=CARTESIAN_POINT ( 'NONE',  ( -10.77132304329999890, 1491.639218371489960, 211.5210277313490224 ) ) ;
#21726=CARTESIAN_POINT ( 'NONE',  ( -1.899216484965220220, 1508.551704408389924, 220.0743039580760012 ) ) ;
#21728=CARTESIAN_POINT ( 'NONE',  ( -18.92738908012519872, 1503.346139213670085, 222.1981866595989743 ) ) ;
#21735=AXIS2_PLACEMENT_3D ( 'NONE', #102682, #70260, #78061 ) ;
#21737=CARTESIAN_POINT ( 'NONE',  ( 3.930410875824919881, 1508.551704408389924, 204.5918276205729853 ) ) ;
#21740=CARTESIAN_POINT ( 'NONE',  ( 0.5708410311183980124, 1460.784089514889729, 230.4191078033510109 ) ) ;
#21743=CARTESIAN_POINT ( 'NONE',  ( 2.174856522119999802, 1490.282954593489876, 188.3516094669990082 ) ) ;
#21745=CARTESIAN_POINT ( 'NONE',  ( 8.266917622984580660, 1505.524528093398885, 217.3397827525526509 ) ) ;
#21761=CARTESIAN_POINT ( 'NONE',  ( 12.78079900903480137, 1420.829302377369913, 202.2958744884179794 ) ) ;
#21763=CARTESIAN_POINT ( 'NONE',  ( -14.80319198780000001, 1420.559702942450031, 212.4542102459990076 ) ) ;
#21770=CARTESIAN_POINT ( 'NONE',  ( -9.065759682986140433, 1448.140860388920146, 211.0596819856369848 ) ) ;
#21775=CARTESIAN_POINT ( 'NONE',  ( 7.433591009027219698, 1425.184177341129953, 212.3839561552370014 ) ) ;
#21776=CARTESIAN_POINT ( 'NONE',  ( -7.548339362227099336, 1493.934769483920036, 206.2816082653209833 ) ) ;
#21785=CARTESIAN_POINT ( 'NONE',  ( -0.9121791906100019665, 1486.347595431690024, 220.6238279289989919 ) ) ;
#21786=CARTESIAN_POINT ( 'NONE',  ( -5.277973487429999722, 1391.913060387289988, 214.4789392792089870 ) ) ;
#21788=VERTEX_POINT ( 'NONE', #68645 ) ;
#21796=CARTESIAN_POINT ( 'NONE',  ( 5.437914377660000298, 1423.457374358000152, 194.5338318222989926 ) ) ;
#21797=VERTEX_POINT ( 'NONE', #17071 ) ;
#21800=FACE_BOUND ( 'NONE', #101332, .T. ) ;
#21803=VERTEX_POINT ( 'NONE', #51269 ) ;
#21809=CARTESIAN_POINT ( 'NONE',  ( 11.31504837134619912, 1480.564413193109885, 212.4592244812710078 ) ) ;
#21816=CARTESIAN_POINT ( 'NONE',  ( 4.552654400296909820, 1499.043495457450035, 198.6118221592419957 ) ) ;
#21819=CARTESIAN_POINT ( 'NONE',  ( 10.47155213350000125, 1420.411604161809919, 197.7872679537989882 ) ) ;
#21820=CARTESIAN_POINT ( 'NONE',  ( 1.257109029569680070, 1474.977242891490050, 220.4718170348219815 ) ) ;
#21821=CARTESIAN_POINT ( 'NONE',  ( -7.790472862750560168, 1493.948223036720037, 199.5897708613550208 ) ) ;
#21826=CARTESIAN_POINT ( 'NONE',  ( 10.74706036746959903, 1424.980385092369943, 206.5419776234139988 ) ) ;
#21835=CARTESIAN_POINT ( 'NONE',  ( -15.37186486470000091, 1415.677402295069896, 210.2490173072590096 ) ) ;
#21836=CARTESIAN_POINT ( 'NONE',  ( -17.36663402931900180, 1419.536926980039880, 207.6991980856880105 ) ) ;
#21838=CARTESIAN_POINT ( 'NONE',  ( 3.554081219399999991, 1430.009957168990013, 217.0886355354290060 ) ) ;
#21841=CARTESIAN_POINT ( 'NONE',  ( -8.000190175716028307, 1477.087591074789543, 215.7421536445566801 ) ) ;
#21845=CARTESIAN_POINT ( 'NONE',  ( 9.788553136239070085, 1435.243871060430138, 208.4607419252359932 ) ) ;
#21855=CARTESIAN_POINT ( 'NONE',  ( 1.842962231260000028, 1515.551704408389924, 205.2922258481490303 ) ) ;
#21867=CARTESIAN_POINT ( 'NONE',  ( 2.536775590219999987, 1486.674089103790266, 197.8596855731989876 ) ) ;
#21868=CARTESIAN_POINT ( 'NONE',  ( 7.049774511539999899, 1478.792398035790029, 201.1901003775490153 ) ) ;
#21870=CARTESIAN_POINT ( 'NONE',  ( -11.07948225550000032, 1491.871587465490165, 207.6232410549289966 ) ) ;
#21874=CARTESIAN_POINT ( 'NONE',  ( -9.360741662101576210, 1480.861349342385893, 227.8150666596004328 ) ) ;
#21878=CARTESIAN_POINT ( 'NONE',  ( -12.16337101708979951, 1490.862671263889979, 207.5438459304560013 ) ) ;
#21882=CARTESIAN_POINT ( 'NONE',  ( 0.04730083781539890647, 1508.790176069789823, 218.1427984678689995 ) ) ;
#21889=CARTESIAN_POINT ( 'NONE',  ( -3.839533257769999874, 1495.661383543789952, 219.6378539895989945 ) ) ;
#21896=CARTESIAN_POINT ( 'NONE',  ( -16.50647692859999793, 1466.206009311390062, 220.8253520350990016 ) ) ;
#21908=CARTESIAN_POINT ( 'NONE',  ( 11.14102298704129979, 1502.488688627300007, 213.5626339687910047 ) ) ;
#21909=CARTESIAN_POINT ( 'NONE',  ( -10.55892651390957226, 1422.392461757438696, 210.6415085614188740 ) ) ;
#21913=CARTESIAN_POINT ( 'NONE',  ( 3.958338197117936108, 1515.551704392563124, 207.2788821125622860 ) ) ;
#21915=CARTESIAN_POINT ( 'NONE',  ( -2.260822717048510455, 1486.453532151730087, 220.8355371193659948 ) ) ;
#21916=CARTESIAN_POINT ( 'NONE',  ( 11.49897960310000045, 1501.122200346590034, 207.7066828831089822 ) ) ;
#21924=CARTESIAN_POINT ( 'NONE',  ( 8.091656396857121791, 1483.420753468610201, 216.4477029494279918 ) ) ;
#21930=CARTESIAN_POINT ( 'NONE',  ( -3.812371247207599900, 1428.459941768050157, 200.5740418269730014 ) ) ;
#21933=ADVANCED_FACE ( 'NONE', ( #104431 ), #54266, .T. ) ;
#21937=CARTESIAN_POINT ( 'NONE',  ( -19.37835159994689960, 1508.551704408389924, 210.4314531256320038 ) ) ;
#21940=CARTESIAN_POINT ( 'NONE',  ( -0.7524479025939990740, 1465.050001273689986, 198.5341880975990136 ) ) ;
#21942=CARTESIAN_POINT ( 'NONE',  ( -5.303285988883490454, 1442.879254652209966, 200.5943008362860098 ) ) ;
#21951=ORIENTED_EDGE ( 'NONE', *, *, #69903, .T. ) ;
#21954=CARTESIAN_POINT ( 'NONE',  ( -18.31568283352659066, 1508.457201626663391, 211.3964485825274835 ) ) ;
#21955=CARTESIAN_POINT ( 'NONE',  ( -9.792761917529839266, 1461.792922494570121, 207.9051543940479974 ) ) ;
#21965=B_SPLINE_CURVE_WITH_KNOTS ( 'NONE', 3,
 ( #60905, #17732, #26146, #95031, #76568, #50823, #59242, #8244, #8798, #44086, #51933, #59788, #93907, #42413 ),
 .UNSPECIFIED., .F., .F.,
 ( 4, 2, 2, 1, 1, 2, 2, 4 ),
 ( 0.000000000000000000, 0.2499999999987723154, 0.3749999999981014076, 0.4374999999978853027, 0.4687499999975743292, 0.4843749999974187870, 0.4999999999972633002, 1.000000000000000000 ),
 .UNSPECIFIED. ) ;
#21972=CARTESIAN_POINT ( 'NONE',  ( 16.62866627238343753, 1455.169317704825971, 198.5414531324474865 ) ) ;
#21974=EDGE_LOOP ( 'NONE', ( #34751, #49674, #30665, #18188 ) ) ;
#21978=CARTESIAN_POINT ( 'NONE',  ( -15.11369138130000067, 1415.717925739890006, 206.7297616978289909 ) ) ;
#21979=CARTESIAN_POINT ( 'NONE',  ( -7.855691861358739203, 1441.328234993660089, 203.4967717689210076 ) ) ;
#21991=CARTESIAN_POINT ( 'NONE',  ( -1.491125504899999843, 1515.528285129289998, 213.1665752102589977 ) ) ;
#21992=LINE ( 'NONE', #6328, #85372 ) ;
#21996=CARTESIAN_POINT ( 'NONE',  ( -9.873159097401318363, 1446.847070703570125, 212.1006879182309888 ) ) ;
#21997=EDGE_CURVE ( 'NONE', #87290, #1678, #90366, .T. ) ;
#22013=CARTESIAN_POINT ( 'NONE',  ( -21.34258212929999488, 1507.002782982890039, 212.5338223445889980 ) ) ;
#22014=CARTESIAN_POINT ( 'NONE',  ( 12.03979944771670141, 1491.360865940330086, 206.6897700099570159 ) ) ;
#22019=ADVANCED_FACE ( 'NONE', ( #51010 ), #108243, .T. ) ;
#22020=CARTESIAN_POINT ( 'NONE',  ( -2.572244737866500319, 1508.551704408389924, 204.1347675067580099 ) ) ;
#22022=ORIENTED_EDGE ( 'NONE', *, *, #33518, .F. ) ;
#22023=CARTESIAN_POINT ( 'NONE',  ( 10.56407690400000021, 1452.658140130590027, 209.7432180304350027 ) ) ;
#22025=CARTESIAN_POINT ( 'NONE',  ( -17.66147422868510120, 1440.150478810159939, 218.7822781200609938 ) ) ;
#22027=CARTESIAN_POINT ( 'NONE',  ( -16.30135123648100048, 1416.771455524889916, 208.9839307753329649 ) ) ;
#22033=CARTESIAN_POINT ( 'NONE',  ( 7.563118004889999746, 1426.194615592600030, 212.1958855806589952 ) ) ;
#22034=CARTESIAN_POINT ( 'NONE',  ( -22.19117979949999864, 1483.602007700189915, 216.8115292462290142 ) ) ;
#22036=CARTESIAN_POINT ( 'NONE',  ( -16.25298958656239989, 1420.731237529160126, 203.3078988358529955 ) ) ;
#22040=CARTESIAN_POINT ( 'NONE',  ( 9.699838434020000122, 1453.359120720189821, 212.1672247696689908 ) ) ;
#22041=ORIENTED_EDGE ( 'NONE', *, *, #20799, .T. ) ;
#22042=VERTEX_POINT ( 'NONE', #89006 ) ;
#22050=CARTESIAN_POINT ( 'NONE',  ( -21.51358107078230120, 1505.588370892289959, 209.3658540944720130 ) ) ;
#22071=ADVANCED_FACE ( 'NONE', ( #72240 ), #51108, .T. ) ;
#22073=CARTESIAN_POINT ( 'NONE',  ( -16.80117805631029881, 1508.522152650069984, 213.2817618438170086 ) ) ;
#22095=CARTESIAN_POINT ( 'NONE',  ( 12.43796050777599937, 1426.539880023309934, 196.0224772779999967 ) ) ;
#22106=CARTESIAN_POINT ( 'NONE',  ( 4.487249772970000272, 1509.038615934189920, 211.6097810847190033 ) ) ;
#22108=CARTESIAN_POINT ( 'NONE',  ( 12.10442663210000092, 1426.312261714450187, 203.5844782087590090 ) ) ;
#22109=CARTESIAN_POINT ( 'NONE',  ( -1.351911418288906486, 1498.080636687657943, 197.8999588905911935 ) ) ;
#22113=DIRECTION ( 'NONE',  ( 0.9232892630913372978, -0.3773383177895360263, 0.07178252285910749486 ) ) ;
#22115=CARTESIAN_POINT ( 'NONE',  ( 10.70393068008039883, 1470.122838572239971, 207.0328785961279721 ) ) ;
#22116=ORIENTED_EDGE ( 'NONE', *, *, #47932, .T. ) ;
#22123=CARTESIAN_POINT ( 'NONE',  ( 10.80173838838189937, 1461.850243658630006, 211.0554024487279889 ) ) ;
#22125=CARTESIAN_POINT ( 'NONE',  ( 0.8893565964429990256, 1443.272965271590010, 218.1164608023390201 ) ) ;
#22137=AXIS2_PLACEMENT_3D ( 'NONE', #92880, #67156, #31320 ) ;
#22139=CARTESIAN_POINT ( 'NONE',  ( -11.35634668980000050, 1508.540398121890121, 217.9340572581489823 ) ) ;
#22141=CARTESIAN_POINT ( 'NONE',  ( 11.39624612213719956, 1470.888150039209904, 208.8400483771679887 ) ) ;
#22143=CARTESIAN_POINT ( 'NONE',  ( 3.089458805060000035, 1471.641899322389918, 189.2928579873990032 ) ) ;
#22148=CARTESIAN_POINT ( 'NONE',  ( 2.670462192661819945, 1494.657381268529889, 220.1092738806310081 ) ) ;
#22160=CARTESIAN_POINT ( 'NONE',  ( -11.43660070340000168, 1501.123905251690076, 209.6404345575209902 ) ) ;
#22175=CARTESIAN_POINT ( 'NONE',  ( -7.058092113492199005, 1478.002960266890113, 218.3245252530660139 ) ) ;
#22178=ADVANCED_FACE ( 'NONE', ( #77672 ), #52955, .T. ) ;
#22184=CARTESIAN_POINT ( 'NONE',  ( -21.44268124680000298, 1506.807080485189999, 216.0956879933890207 ) ) ;
#22186=CARTESIAN_POINT ( 'NONE',  ( 0.2984413201195192933, 1473.419535434050658, 219.3416222726238800 ) ) ;
#22191=CARTESIAN_POINT ( 'NONE',  ( 10.03721076337500051, 1469.143571486790051, 209.2919969481099827 ) ) ;
#22192=CARTESIAN_POINT ( 'NONE',  ( -5.931789999490000298, 1459.036866685989935, 218.1324649368089865 ) ) ;
#22195=ORIENTED_EDGE ( 'NONE', *, *, #7641, .T. ) ;
#22202=CARTESIAN_POINT ( 'NONE',  ( -8.701122736030638904, 1447.991463143899864, 212.1854974882720057 ) ) ;
#22205=PRESENTATION_STYLE_ASSIGNMENT (( #21657 ) ) ;
#22211=SHAPE_REPRESENTATION ( 'Feed Screw', ( #21632 ), #28938 ) ;
#22226=CARTESIAN_POINT ( 'NONE',  ( 6.325405113577525107, 1460.162224217434868, 201.8389639430470481 ) ) ;
#22227=CARTESIAN_POINT ( 'NONE',  ( 9.609447197979999800, 1453.954725363390025, 213.7354802858189942 ) ) ;
#22234=LINE ( 'NONE', #106810, #75939 ) ;
#22238=CARTESIAN_POINT ( 'NONE',  ( -5.106893092629549713, 1391.877272788475011, 214.4361776400186557 ) ) ;
#22245=CARTESIAN_POINT ( 'NONE',  ( 3.074703527060000052, 1441.333178254290033, 218.5515148082390056 ) ) ;
#22261=CARTESIAN_POINT ( 'NONE',  ( -10.11770193674129992, 1472.442116771029987, 210.2941300317889954 ) ) ;
#22266=CARTESIAN_POINT ( 'NONE',  ( 10.55879509197319877, 1480.973079402069970, 209.1396683372450127 ) ) ;
#22268=CARTESIAN_POINT ( 'NONE',  ( -2.858448621680000024, 1443.821599769190016, 199.4616741486989895 ) ) ;
#22269=CARTESIAN_POINT ( 'NONE',  ( 7.550320201100000794, 1423.033199310010104, 195.6993168036990198 ) ) ;
#22274=CARTESIAN_POINT ( 'NONE',  ( 2.310682350337450064, 1508.551704408389924, 219.5967718590839866 ) ) ;
#22278=CARTESIAN_POINT ( 'NONE',  ( -11.41800801098339946, 1501.040032621129967, 208.6024801871049874 ) ) ;
#22280=ORIENTED_EDGE ( 'NONE', *, *, #5122, .T. ) ;
#22284=ADVANCED_FACE ( 'NONE', ( #35702 ), #10010, .T. ) ;
#22285=CARTESIAN_POINT ( 'NONE',  ( -3.229911446790000085, 1475.410210782889862, 198.9236622250990081 ) ) ;
#22288=CARTESIAN_POINT ( 'NONE',  ( -20.36852575855199987, 1464.956479398600095, 210.9457983963280014 ) ) ;
#22293=CARTESIAN_POINT ( 'NONE',  ( -4.759967386468179740, 1475.369894740059181, 199.9752752562233979 ) ) ;
#22300=CARTESIAN_POINT ( 'NONE',  ( 4.617353517619999792, 1460.098150474590057, 228.0971968620989969 ) ) ;
#22313=CARTESIAN_POINT ( 'NONE',  ( -14.67572137840000046, 1420.538682257900064, 213.1455671837790078 ) ) ;
#22321=CARTESIAN_POINT ( 'NONE',  ( -9.818885166255999053, 1447.613981975209754, 210.5167627897619980 ) ) ;
#22332=CARTESIAN_POINT ( 'NONE',  ( -11.59563781346980171, 1491.413760601690001, 206.8061924195220058 ) ) ;
#22337=CARTESIAN_POINT ( 'NONE',  ( -4.637174521050656750, 1378.050660721826034, 214.3535596345795966 ) ) ;
#22346=CARTESIAN_POINT ( 'NONE',  ( 9.675872734536000053, 1452.418772690649803, 210.2673697975640152 ) ) ;
#22353=VERTEX_POINT ( 'NONE', #17074 ) ;
#22358=CARTESIAN_POINT ( 'NONE',  ( -7.447340581099999746, 1425.934151271280143, 204.0825129966889904 ) ) ;
#22362=ORIENTED_EDGE ( 'NONE', *, *, #108, .F. ) ;
#22363=VERTEX_POINT ( 'NONE', #8702 ) ;
#22364=CARTESIAN_POINT ( 'NONE',  ( -11.01402028494999996, 1481.503834766900127, 208.8098579862920019 ) ) ;
#22369=CARTESIAN_POINT ( 'NONE',  ( 9.539810668950000405, 1420.903745483679813, 197.1733355697989793 ) ) ;
#22376=CARTESIAN_POINT ( 'NONE',  ( 10.70518913711110010, 1423.800132577800014, 206.7158561157320094 ) ) ;
#22377=CARTESIAN_POINT ( 'NONE',  ( -9.819155800674218781, 1439.994030334630224, 207.1637469923470007 ) ) ;
#22381=CARTESIAN_POINT ( 'NONE',  ( -17.03149518429903608, 1417.396562231937196, 206.8274202490092648 ) ) ;
#22385=CARTESIAN_POINT ( 'NONE',  ( 11.11857203984600062, 1427.722971555709819, 210.2004789491199972 ) ) ;
#22386=CARTESIAN_POINT ( 'NONE',  ( -6.816032832730000379, 1464.119504676089946, 200.4313534491789994 ) ) ;
#22387=ORIENTED_EDGE ( 'NONE', *, *, #82542, .T. ) ;
#22390=CARTESIAN_POINT ( 'NONE',  ( -16.76063698560000148, 1417.345490017750080, 208.1330266677999816 ) ) ;
#22395=CARTESIAN_POINT ( 'NONE',  ( 4.347845440834370301, 1459.306986539150103, 200.4470736973389933 ) ) ;
#22399=CARTESIAN_POINT ( 'NONE',  ( 3.319698225923770174, 1474.465735597630101, 220.0484424645880210 ) ) ;
#22406=CARTESIAN_POINT ( 'NONE',  ( 12.54203963119180010, 1427.020850620109968, 206.2427846923719983 ) ) ;
#22415=DIRECTION ( 'NONE',  ( -1.156023075842281927E-31, 1.000000000000000000, -1.698192320643030073E-16 ) ) ;
#22418=CARTESIAN_POINT ( 'NONE',  ( 3.412268725760000176, 1476.681763699690009, 198.4748995137989880 ) ) ;
#22420=CARTESIAN_POINT ( 'NONE',  ( -11.43222421799999999, 1490.997350406890064, 208.8577229060449838 ) ) ;
#22433=EDGE_CURVE ( 'NONE', #34842, #51303, #78859, .T. ) ;
#22434=CARTESIAN_POINT ( 'NONE',  ( 2.589318363809999912, 1507.773265401989875, 217.6873885498590084 ) ) ;
#22438=CARTESIAN_POINT ( 'NONE',  ( 10.95090191305459904, 1471.837486416480033, 212.3990077965439980 ) ) ;
#22447=CARTESIAN_POINT ( 'NONE',  ( -9.495330813260000724, 1465.238080356989940, 228.3114829157989902 ) ) ;
#22451=CARTESIAN_POINT ( 'NONE',  ( 7.108361874469999897, 1480.745134477889906, 207.3349235958489771 ) ) ;
#22466=CARTESIAN_POINT ( 'NONE',  ( 1.157679221055670116, 1485.519117650379940, 220.9368485806469948 ) ) ;
#22468=CARTESIAN_POINT ( 'NONE',  ( 11.41568233489999962, 1500.982773024489916, 207.1620391477790122 ) ) ;
#22475=CARTESIAN_POINT ( 'NONE',  ( 20.41258333560000082, 1494.156730172889866, 204.1224707391089908 ) ) ;
#22479=CARTESIAN_POINT ( 'NONE',  ( 5.076283890730000081, 1469.790178736790040, 187.8425608535989966 ) ) ;
#22480=CARTESIAN_POINT ( 'NONE',  ( -2.746886073237670089, 1430.908227116830176, 201.2170371325859719 ) ) ;
#22481=EDGE_LOOP ( 'NONE', ( #17989, #2163, #91228, #53290, #85731, #22631, #22280, #89872, #87216, #77620, #52423, #34263 ) ) ;
#22490=CARTESIAN_POINT ( 'NONE',  ( -0.8071984717899990391, 1465.223756610790133, 198.1240437993990042 ) ) ;
#22504=CARTESIAN_POINT ( 'NONE',  ( -9.585289191388769225, 1462.057342544479980, 206.7320176240860121 ) ) ;
#22512=CARTESIAN_POINT ( 'NONE',  ( 6.705798878809999586, 1469.980848758390039, 210.5526231697390074 ) ) ;
#22516=TOROIDAL_SURFACE ( 'NONE', #56529, 10.10241613150000006, 2.000000000000000000 ) ;
#22520=CARTESIAN_POINT ( 'NONE',  ( 2.329898367294779504, 1515.064791340959800, 213.4512947642129745 ) ) ;
#22522=CARTESIAN_POINT ( 'NONE',  ( -11.62069923840673091, 1507.830660535743391, 207.5518435106793618 ) ) ;
#22523=ORIENTED_EDGE ( 'NONE', *, *, #46707, .F. ) ;
#22525=CARTESIAN_POINT ( 'NONE',  ( 1.901370350220000116, 1507.955859758289989, 220.6917275793990143 ) ) ;
#22532=CARTESIAN_POINT ( 'NONE',  ( 10.46140733719999893, 1420.326681975860083, 197.7779852210990157 ) ) ;
#22535=CARTESIAN_POINT ( 'NONE',  ( -10.15848146045460076, 1480.881806938720047, 206.2592734015669862 ) ) ;
#22541=CARTESIAN_POINT ( 'NONE',  ( 10.84315941642620018, 1489.732817849439925, 207.6990053546570039 ) ) ;
#22544=CARTESIAN_POINT ( 'NONE',  ( -1.354610398945402805, 1463.304784733452152, 199.4317993211560065 ) ) ;
#22545=( BOUNDED_SURFACE ( )  B_SPLINE_SURFACE ( 1, 2, ( 
 ( #63970, #62899, #98085, #90787, #2968, #80198, #3516, #98634, #20820 ),
 ( #72366, #71846, #106497, #71289, #88611, #72903, #105402, #54474, #11893 ) ),
 .UNSPECIFIED., .F., .T., .F. ) 
 B_SPLINE_SURFACE_WITH_KNOTS ( ( 2, 2 ),
 ( 3, 2, 2, 2, 3 ),
 ( -10000.00000000000000, 10000.00000000000000 ),
 ( 0.000000000000000000, 1.570796326794899889, 3.141592653589790007, 4.712388980384689674, 6.283185307179590673 ),
 .UNSPECIFIED. ) 
 GEOMETRIC_REPRESENTATION_ITEM ( )  RATIONAL_B_SPLINE_SURFACE ( (
 ( 1.000000000000000000, 0.7071067811865480168, 1.000000000000000000, 0.7071067811865480168, 1.000000000000000000, 0.7071067811865480168, 1.000000000000000000, 0.7071067811865480168, 1.000000000000000000),
 ( 1.000000000000000000, 0.7071067811865480168, 1.000000000000000000, 0.7071067811865480168, 1.000000000000000000, 0.7071067811865480168, 1.000000000000000000, 0.7071067811865480168, 1.000000000000000000) ) ) 
 REPRESENTATION_ITEM ( '' )  SURFACE ( )  );
#22547=CARTESIAN_POINT ( 'NONE',  ( -10.24550950064739929, 1447.425523760389979, 210.5433215532739837 ) ) ;
#22552=CARTESIAN_POINT ( 'NONE',  ( -4.015743051850000356, 1515.588776726489868, 209.8750191343430060 ) ) ;
#22562=CARTESIAN_POINT ( 'NONE',  ( -21.57330136150000044, 1507.349411603790031, 210.4857862235489847 ) ) ;
#22571=CARTESIAN_POINT ( 'NONE',  ( -19.77045317620000020, 1466.948919781690165, 211.0321804172989744 ) ) ;
#22573=CARTESIAN_POINT ( 'NONE',  ( -9.838224505892318561, 1462.268909613540245, 227.9668215274659815 ) ) ;
#22578=CARTESIAN_POINT ( 'NONE',  ( -4.784282693639999806, 1454.717937669690173, 201.0055521229189992 ) ) ;
#22580=CARTESIAN_POINT ( 'NONE',  ( 7.363738131959999933, 1426.807041349819883, 212.7119719394189872 ) ) ;
#22583=CARTESIAN_POINT ( 'NONE',  ( -22.55307526729999879, 1417.538526918689968, 209.9295645762900051 ) ) ;
#22597=CARTESIAN_POINT ( 'NONE',  ( 3.442291544270000170, 1445.232941167789932, 200.8115262291190106 ) ) ;
#22610=ORIENTED_EDGE ( 'NONE', *, *, #63149, .F. ) ;
#22620=CARTESIAN_POINT ( 'NONE',  ( -11.32684497959999881, 1503.073821494790081, 207.0295587123389964 ) ) ;
#22631=ORIENTED_EDGE ( 'NONE', *, *, #28676, .T. ) ;
#22642=CARTESIAN_POINT ( 'NONE',  ( 17.37368555716430052, 1428.575912512719924, 203.8623300055620007 ) ) ;
#22647=DIRECTION ( 'NONE',  ( -0.1151936120068250274, -0.4472295632498141660, -0.8869702077906571613 ) ) ;
#22661=CARTESIAN_POINT ( 'NONE',  ( 10.61261630010000090, 1424.158067204230065, 205.9607122707290046 ) ) ;
#22671=CARTESIAN_POINT ( 'NONE',  ( 10.43886700434340042, 1480.990255025190208, 207.5644369805290239 ) ) ;
#22677=CARTESIAN_POINT ( 'NONE',  ( 9.521227846441806975, 1425.375466301815777, 195.5306922762230215 ) ) ;
#22679=CARTESIAN_POINT ( 'NONE',  ( 0.7868378234909989555, 1442.894628652889878, 218.3517676095690092 ) ) ;
#22683=CARTESIAN_POINT ( 'NONE',  ( 10.52956383476244007, 1489.196172734509446, 206.2018118126233333 ) ) ;
#22686=CARTESIAN_POINT ( 'NONE',  ( 18.20258715539999983, 1429.723789929190161, 209.1218459616989946 ) ) ;
#22687=EDGE_CURVE ( 'NONE', #19377, #47729, #105163, .T. ) ;
#22689=VERTEX_POINT ( 'NONE', #53942 ) ;
#22692=CARTESIAN_POINT ( 'NONE',  ( 11.14479613505110045, 1470.280215154140024, 206.9369914153219838 ) ) ;
#22697=CARTESIAN_POINT ( 'NONE',  ( -8.611480341139710504, 1436.906018617760083, 209.7133912976819943 ) ) ;
#22700=CARTESIAN_POINT ( 'NONE',  ( -21.59687142900000012, 1507.523380033690046, 209.4572543540780032 ) ) ;
#22710=CARTESIAN_POINT ( 'NONE',  ( -11.45038415740000026, 1501.280273630989996, 209.1761187364329828 ) ) ;
#22717=CARTESIAN_POINT ( 'NONE',  ( -5.032977198260000229, 1391.805267112089950, 203.8075142969990168 ) ) ;
#22718=CARTESIAN_POINT ( 'NONE',  ( 9.457965440796609613, 1464.320992644629996, 211.7920758070480076 ) ) ;
#22720=CARTESIAN_POINT ( 'NONE',  ( 1.629715277548020147, 1515.068677689339893, 213.4511930101580219 ) ) ;
#22726=EDGE_CURVE ( 'NONE', #21322, #84181, #49050, .T. ) ;
#22728=ORIENTED_EDGE ( 'NONE', *, *, #19031, .T. ) ;
#22729=ORIENTED_EDGE ( 'NONE', *, *, #56184, .T. ) ;
#22732=CARTESIAN_POINT ( 'NONE',  ( 24.12566577620000174, 1497.029149703290159, 206.7581795058389957 ) ) ;
#22734=CARTESIAN_POINT ( 'NONE',  ( 1.396945595908719806, 1473.097535771269804, 219.2356281669150064 ) ) ;
#22739=CARTESIAN_POINT ( 'NONE',  ( 10.02252456385629920, 1469.313878311580083, 209.8095366709860059 ) ) ;
#22740=CARTESIAN_POINT ( 'NONE',  ( -2.958239116441676586, 1515.068899845848136, 204.7925047304020723 ) ) ;
#22761=CARTESIAN_POINT ( 'NONE',  ( -19.67891453321817963, 1505.885360177188886, 218.9962822164112310 ) ) ;
#22771=CARTESIAN_POINT ( 'NONE',  ( 3.753290028884420426, 1426.393640232169901, 191.4546578126879979 ) ) ;
#22776=CARTESIAN_POINT ( 'NONE',  ( 6.721016565425069089, 1460.347746334779004, 202.1888905636935192 ) ) ;
#22778=CARTESIAN_POINT ( 'NONE',  ( 6.590784414382070189, 1439.968245627540000, 215.2411843296279983 ) ) ;
#22794=CARTESIAN_POINT ( 'NONE',  ( 11.36216713388179933, 1503.110266152410077, 211.0233809544849919 ) ) ;
#22796=CARTESIAN_POINT ( 'NONE',  ( -18.31482527320000031, 1445.278739201789904, 204.5307550449689984 ) ) ;
#22810=CARTESIAN_POINT ( 'NONE',  ( -3.527118517899999972, 1475.290297289889850, 218.8061209762090016 ) ) ;
#22820=CARTESIAN_POINT ( 'NONE',  ( 3.235048521747439842, 1466.472015811129950, 219.6884157710169916 ) ) ;
#22825=AXIS2_PLACEMENT_3D ( 'NONE', #62864, #97513, #1260 ) ;
#22827=CARTESIAN_POINT ( 'NONE',  ( -2.530629316699999798, 1443.373190519289892, 200.1619764056190149 ) ) ;
#22831=CARTESIAN_POINT ( 'NONE',  ( -4.848919996459999382, 1489.192135936889827, 188.8958457811990002 ) ) ;
#22838=CARTESIAN_POINT ( 'NONE',  ( -12.78943302956389871, 1502.708798875820094, 209.0180534851929792 ) ) ;
#22840=CARTESIAN_POINT ( 'NONE',  ( -2.320817964079999740, 1456.878784100789971, 218.4789852815589768 ) ) ;
#22841=ORIENTED_EDGE ( 'NONE', *, *, #22726, .T. ) ;
#22844=CARTESIAN_POINT ( 'NONE',  ( 2.716551985052390261, 1508.551704408389924, 204.1452468848800095 ) ) ;
#22855=CARTESIAN_POINT ( 'NONE',  ( -16.24421748424699885, 1508.551704408389924, 213.5434314520410339 ) ) ;
#22856=AXIS2_PLACEMENT_3D ( 'NONE', #27278, #86628, #36235 ) ;
#22859=CARTESIAN_POINT ( 'NONE',  ( 8.731332846349999954, 1459.404707344790040, 227.0651519182989944 ) ) ;
#22869=CARTESIAN_POINT ( 'NONE',  ( -15.57028380409999890, 1420.200962988549918, 211.3154909670090262 ) ) ;
#22881=CARTESIAN_POINT ( 'NONE',  ( 7.471609634030699887, 1425.264358481019826, 212.3048529994830176 ) ) ;
#22884=CARTESIAN_POINT ( 'NONE',  ( -0.5624325259219991047, 1417.052906817089934, 204.0409946397689964 ) ) ;
#22916=CARTESIAN_POINT ( 'NONE',  ( 10.14952118758730037, 1481.589675501239981, 215.1524303884280300 ) ) ;
#22918=CARTESIAN_POINT ( 'NONE',  ( 6.802837640179999923, 1469.003421131590130, 208.5716255075389824 ) ) ;
#22923=EDGE_CURVE ( 'NONE', #7222, #777, #17367, .T. ) ;
#22927=CARTESIAN_POINT ( 'NONE',  ( 6.195357806510189747, 1504.701517326509929, 220.2771928074470225 ) ) ;
#22929=CARTESIAN_POINT ( 'NONE',  ( 12.65728676320000012, 1420.119835126070029, 200.3472210942090044 ) ) ;
#22931=FACE_OUTER_BOUND ( 'NONE', #45893, .T. ) ;
#22932=CARTESIAN_POINT ( 'NONE',  ( -5.030159814880000191, 1495.846928005290010, 198.9636958132990117 ) ) ;
#22936=CARTESIAN_POINT ( 'NONE',  ( 11.43232951270710096, 1426.317992301700087, 206.5079432659420036 ) ) ;
#22938=AXIS2_PLACEMENT_3D ( 'NONE', #60665, #59548, #8568 ) ;
#22947=CARTESIAN_POINT ( 'NONE',  ( 19.88011795350000099, 1476.500998830189928, 213.0752383808189734 ) ) ;
#22948=CARTESIAN_POINT ( 'NONE',  ( 11.04498765331799959, 1424.577033446239966, 203.0973991204349716 ) ) ;
#22950=CARTESIAN_POINT ( 'NONE',  ( 2.495739975459999815, 1430.974676233789978, 218.2901151006489897 ) ) ;
#22965=CARTESIAN_POINT ( 'NONE',  ( -7.654188446680000091, 1491.752080352689973, 210.6569740451089956 ) ) ;
#22966=CARTESIAN_POINT ( 'NONE',  ( 6.063466852619999514, 1461.859068799589977, 206.6237464781989956 ) ) ;
#22968=CARTESIAN_POINT ( 'NONE',  ( -0.7398872336889990020, 1515.545288638290003, 204.9978666827690006 ) ) ;
#22970=CARTESIAN_POINT ( 'NONE',  ( -17.11733441484010143, 1420.830776991170069, 201.6585818365429645 ) ) ;
#22981=CARTESIAN_POINT ( 'NONE',  ( -3.994937574034520100, 1430.106198372560129, 201.8091617894969829 ) ) ;
#22986=CARTESIAN_POINT ( 'NONE',  ( -11.03225848849999835, 1492.060404916889865, 208.5626278536280154 ) ) ;
#22991=CARTESIAN_POINT ( 'NONE',  ( 8.758613636697381466, 1427.348504481640020, 211.4846159547069817 ) ) ;
#23012=CARTESIAN_POINT ( 'NONE',  ( -19.76672171450000093, 1468.192140521490046, 204.4230837022790297 ) ) ;
#23028=ORIENTED_EDGE ( 'NONE', *, *, #61812, .T. ) ;
#23032=CARTESIAN_POINT ( 'NONE',  ( -1.740723996199489809, 1486.328230267929939, 220.9124301049980090 ) ) ;
#23033=CARTESIAN_POINT ( 'NONE',  ( 11.42348759009999881, 1501.742913944189922, 208.1569337396019819 ) ) ;
#23042=CARTESIAN_POINT ( 'NONE',  ( 4.923775256296569758, 1508.551704408389924, 212.1750878591210210 ) ) ;
#23044=CARTESIAN_POINT ( 'NONE',  ( -5.586172216781320365, 1491.246046052670181, 185.8699220213879926 ) ) ;
#23051=CARTESIAN_POINT ( 'NONE',  ( -21.12444512610820269, 1508.254181376620181, 209.6686171012820239 ) ) ;
#23056=CARTESIAN_POINT ( 'NONE',  ( -12.63439616088674633, 1483.510510869872178, 226.0832403630100771 ) ) ;
#23073=CARTESIAN_POINT ( 'NONE',  ( -9.456798816358269022, 1461.539703310480036, 206.9210100075549974 ) ) ;
#23082=CARTESIAN_POINT ( 'NONE',  ( 6.784288798619999561, 1469.672316088890057, 209.8806407344229967 ) ) ;
#23098=EDGE_CURVE ( 'NONE', #73262, #43039, #86684, .T. ) ;
#23100=CARTESIAN_POINT ( 'NONE',  ( -15.73032604960000036, 1415.742867544160163, 209.5189867902049912 ) ) ;
#23103=CARTESIAN_POINT ( 'NONE',  ( 7.943378312860001067, 1421.399538177179920, 195.9193817166990073 ) ) ;
#23104=CARTESIAN_POINT ( 'NONE',  ( -3.052469087571969997, 1446.532390927849974, 214.7242444357609941 ) ) ;
#23106=CARTESIAN_POINT ( 'NONE',  ( -11.41675301695839906, 1482.775673471900063, 205.7339463974809917 ) ) ;
#23109=ORIENTED_EDGE ( 'NONE', *, *, #35830, .F. ) ;
#23113=CARTESIAN_POINT ( 'NONE',  ( 10.95494146437559912, 1490.325474812490029, 209.5571900555880234 ) ) ;
#23118=CARTESIAN_POINT ( 'NONE',  ( -10.31774485735029856, 1447.649174093579859, 209.9773725357489980 ) ) ;
#23121=LINE ( 'NONE', #57325, #65884 ) ;
#23123=CARTESIAN_POINT ( 'NONE',  ( -11.67169904650000056, 1501.458093402889972, 211.3450001610790139 ) ) ;
#23131=DIRECTION ( 'NONE',  ( 0.06270903725022243524, -1.833354768615425389E-16, -0.9980318515193542517 ) ) ;
#23136=B_SPLINE_SURFACE_WITH_KNOTS ( 'NONE', 5, 5, ( 
 ( #45453, #62826, #11823, #38664, #106972, #96382 ),
 ( #104780, #105893, #80681, #19660, #80125, #70666 ),
 ( #79595, #53864, #29174, #106431, #89618, #72300 ),
 ( #88539, #45993, #98014, #3444, #21285, #55493 ),
 ( #12909, #21835, #37017, #30259, #4530, #56033 ),
 ( #88003, #11286, #31364, #82328, #15099, #7273 ) ),
 .UNSPECIFIED., .F., .F., .F.,
 ( 6, 6 ),
 ( 6, 6 ),
 ( 30.99314794090000191, 41.27704706610000329 ),
 ( 0.000000000000000000, 0.5000000000000000000 ),
 .UNSPECIFIED. ) ;
#23137=CARTESIAN_POINT ( 'NONE',  ( 12.13947661551040014, 1491.513716010349981, 207.1733083333600121 ) ) ;
#23141=CARTESIAN_POINT ( 'NONE',  ( 12.90425579462769790, 1421.183432210740193, 204.7522736897579989 ) ) ;
#23146=DIRECTION ( 'NONE',  ( 0.9528104219824277132, 0.2959442204286599210, -0.06759673184807767077 ) ) ;
#23147=DIRECTION ( 'NONE',  ( 0.000000000000000000, 0.000000000000000000, 1.000000000000000000 ) ) ;
#23148=CARTESIAN_POINT ( 'NONE',  ( 0.9103524645702290030, 1462.760075378919964, 230.5111400575189862 ) ) ;
#23154=CARTESIAN_POINT ( 'NONE',  ( -14.35646903299999799, 1420.584115152450067, 213.7701001417389932 ) ) ;
#23155=CARTESIAN_POINT ( 'NONE',  ( -4.732406976500000084, 1453.644983325290013, 200.2083546425689917 ) ) ;
#23157=CARTESIAN_POINT ( 'NONE',  ( 8.309621275030000476, 1427.613389394789920, 212.3081093229889973 ) ) ;
#23160=CARTESIAN_POINT ( 'NONE',  ( -17.74072797668249990, 1419.883333100649907, 204.5911605323600213 ) ) ;
#23174=CARTESIAN_POINT ( 'NONE',  ( 1.514255875599999968, 1444.175298751890068, 200.2744927717990038 ) ) ;
#23177=CARTESIAN_POINT ( 'NONE',  ( -3.841809705010690301, 1464.683280171979959, 198.7835890369999845 ) ) ;
#23178=CARTESIAN_POINT ( 'NONE',  ( -1.971951421069999988, 1423.054295909000075, 191.2999637764989984 ) ) ;
#23186=DIRECTION ( 'NONE',  ( 1.000000000000000000, 0.000000000000000000, 0.000000000000000000 ) ) ;
#23187=VERTEX_POINT ( 'NONE', #33930 ) ;
#23195=ORIENTED_EDGE ( 'NONE', *, *, #87035, .F. ) ;
#23196=CARTESIAN_POINT ( 'NONE',  ( -11.71166783339999995, 1503.433515124489986, 208.0502066329989930 ) ) ;
#23201=B_SPLINE_CURVE_WITH_KNOTS ( 'NONE', 3,
 ( #4348, #38477, #61505, #18903, #55865, #31178, #14917, #23324, #47449, #56401, #32291, #40134, #74318, #14366, #90533, #100583, #73764, #108448, #31728, #99473, #57517, #107341, #81573 ),
 .UNSPECIFIED., .F., .F.,
 ( 4, 2, 1, 2, 2, 2, 2, 2, 2, 2, 2, 4 ),
 ( 0.000000000000000000, 0.1249999999991294464, 0.1874999999988291033, 0.2187499999987238541, 0.2499999999986186050, 0.3749999999983899546, 0.4374999999980648258, 0.4999999999977396969, 0.6249999999977112752, 0.6874999999976637577, 0.7499999999976162401, 1.000000000000000000 ),
 .UNSPECIFIED. ) ;
#23204=VECTOR ( 'NONE', #86362, 1000.000000000000114 ) ;
#23205=CARTESIAN_POINT ( 'NONE',  ( -7.305485514955160298, 1453.383523734929895, 203.2828978378740032 ) ) ;
#23218=CARTESIAN_POINT ( 'NONE',  ( 2.713660715419999647, 1441.511099666689915, 218.6663635638090000 ) ) ;
#23221=CARTESIAN_POINT ( 'NONE',  ( 9.602386435385879437, 1434.766419721330067, 207.2149381967969930 ) ) ;
#23223=( BOUNDED_CURVE ( )  B_SPLINE_CURVE ( 3, ( #89768, #97085, #37173, #47227 ),
 .UNSPECIFIED., .F., .F. ) 
 B_SPLINE_CURVE_WITH_KNOTS ( ( 4, 4 ),
 ( 4.148492618474420190, 5.276285279552140217 ),
 .UNSPECIFIED. ) 
 CURVE ( )  GEOMETRIC_REPRESENTATION_ITEM ( )  RATIONAL_B_SPLINE_CURVE ( ( 1.000000000000000000, 0.8967860053317929792, 0.8967860053317929792, 1.000000000000000000 ) ) 
 REPRESENTATION_ITEM ( '' )  );
#23228=AXIS2_PLACEMENT_3D ( 'NONE', #105018, #59851, #93975 ) ;
#23235=CARTESIAN_POINT ( 'NONE',  ( 12.08449222550000002, 1421.674727768539924, 206.2100432727989983 ) ) ;
#23240=CARTESIAN_POINT ( 'NONE',  ( 0.6209246841665734262, 1515.589587247402505, 205.1019389779893913 ) ) ;
#23247=CARTESIAN_POINT ( 'NONE',  ( 10.94084016961279993, 1461.364874240460040, 209.8155579094599830 ) ) ;
#23248=CARTESIAN_POINT ( 'NONE',  ( 9.319248534172345444, 1425.257639114323183, 195.5897260868380272 ) ) ;
#23249=CARTESIAN_POINT ( 'NONE',  ( -0.6891144619180010755, 1443.914159960489997, 218.1634325674289698 ) ) ;
#23261=EDGE_CURVE ( 'NONE', #41661, #106368, #45097, .T. ) ;
#23268=CARTESIAN_POINT ( 'NONE',  ( -9.518234561902950475, 1438.815826527629952, 209.5578901295930052 ) ) ;
#23271=CARTESIAN_POINT ( 'NONE',  ( -14.37435889315949922, 1415.677402204050168, 205.0862553119529821 ) ) ;
#23278=DIRECTION ( 'NONE',  ( -1.000000000000000000, 0.000000000000000000, 0.000000000000000000 ) ) ;
#23281=CARTESIAN_POINT ( 'NONE',  ( -11.92170027740000116, 1502.281711308889953, 208.9298100184969940 ) ) ;
#23283=CARTESIAN_POINT ( 'NONE',  ( 2.629563630540000307, 1456.337126530590012, 219.4237753482989888 ) ) ;
#23285=CARTESIAN_POINT ( 'NONE',  ( -2.274880353649999964, 1445.428165552290011, 217.8632208591889992 ) ) ;
#23300=EDGE_CURVE ( 'NONE', #97433, #18368, #100978, .T. ) ;
#23301=CARTESIAN_POINT ( 'NONE',  ( -13.76731767608630008, 1503.460756753999931, 227.5714742811019846 ) ) ;
#23303=CARTESIAN_POINT ( 'NONE',  ( -0.1116522590836569045, 1473.547763220521347, 219.3528841741646147 ) ) ;
#23308=EDGE_CURVE ( 'NONE', #714, #42229, #21045, .T. ) ;
#23309=CARTESIAN_POINT ( 'NONE',  ( -7.291808457750000194, 1480.410216369889895, 208.6747883837709878 ) ) ;
#23312=CARTESIAN_POINT ( 'NONE',  ( -3.776018960370000066, 1457.468576287289807, 218.0147105414490056 ) ) ;
#23317=CARTESIAN_POINT ( 'NONE',  ( -4.327403558811090178, 1515.142896577510101, 209.6457263099750037 ) ) ;
#23318=VERTEX_POINT ( 'NONE', #29940 ) ;
#23324=CARTESIAN_POINT ( 'NONE',  ( -17.62619653710081025, 1419.739949534606012, 206.8872665010755156 ) ) ;
#23336=CARTESIAN_POINT ( 'NONE',  ( -17.54330095577449811, 1486.685527788949912, 197.8065059920220108 ) ) ;
#23344=CARTESIAN_POINT ( 'NONE',  ( -0.007179413344095889743, 1425.548651214390020, 191.0976962420139955 ) ) ;
#23349=CARTESIAN_POINT ( 'NONE',  ( 7.369559949379922870, 1460.670680854289913, 202.8482577992020310 ) ) ;
#23359=VERTEX_POINT ( 'NONE', #103780 ) ;
#23367=CARTESIAN_POINT ( 'NONE',  ( 7.003830488220000206, 1486.892509085090069, 200.8568873985890093 ) ) ;
#23368=CARTESIAN_POINT ( 'NONE',  ( -4.724155950714410857, 1476.228105402329902, 199.9129071112880069 ) ) ;
#23376=CARTESIAN_POINT ( 'NONE',  ( -17.90910890133720201, 1508.551704408389924, 211.2475455717739976 ) ) ;
#23378=CARTESIAN_POINT ( 'NONE',  ( -3.441085532370000255, 1476.342819318190095, 219.6507254485989904 ) ) ;
#23381=CARTESIAN_POINT ( 'NONE',  ( -3.676556857354845942, 1508.129772564241193, 220.7334657978175017 ) ) ;
#23384=CARTESIAN_POINT ( 'NONE',  ( 1.480207909756110052, 1456.259238296559943, 198.6472058902120068 ) ) ;
#23385=DIRECTION ( 'NONE',  ( -1.224646799147350002E-16, 1.836970198721029688E-16, 1.000000000000000000 ) ) ;
#23387=CARTESIAN_POINT ( 'NONE',  ( -10.70956146626689964, 1470.466741431640230, 211.3590706241550095 ) ) ;
#23392=CARTESIAN_POINT ( 'NONE',  ( 7.844692007760903252, 1439.683743732501171, 213.0755470696874454 ) ) ;
#23397=CARTESIAN_POINT ( 'NONE',  ( 8.239807433079999299, 1424.467077651120235, 195.8470003964989985 ) ) ;
#23401=CARTESIAN_POINT ( 'NONE',  ( 9.642184866601970938, 1422.568599004970110, 212.5648991404160029 ) ) ;
#23407=CARTESIAN_POINT ( 'NONE',  ( 11.09105618205479971, 1492.398032610720065, 212.1352801084049986 ) ) ;
#23408=CARTESIAN_POINT ( 'NONE',  ( 0.8903357919429990552, 1455.384224998389982, 218.5322622568489805 ) ) ;
#23411=ADVANCED_FACE ( 'NONE', ( #72937 ), #30914, .T. ) ;
#23413=CARTESIAN_POINT ( 'NONE',  ( -3.603670846500000025, 1475.686176941090025, 199.3076260124989858 ) ) ;
#23414=ORIENTED_EDGE ( 'NONE', *, *, #33709, .F. ) ;
#23417=DIRECTION ( 'NONE',  ( 1.000000000000000000, 1.810374147724000060E-32, 1.224646799147351975E-16 ) ) ;
#23418=CARTESIAN_POINT ( 'NONE',  ( -2.329957330370640456, 1515.551704201149960, 205.2926810898260044 ) ) ;
#23422=CARTESIAN_POINT ( 'NONE',  ( -9.861036302450001401, 1463.031815716689835, 205.0798590038790223 ) ) ;
#23424=CARTESIAN_POINT ( 'NONE',  ( -15.84432591830269743, 1419.853212859319910, 210.7451195136700051 ) ) ;
#23426=CARTESIAN_POINT ( 'NONE',  ( -10.30687864337570048, 1508.551704408389924, 218.1317960845860000 ) ) ;
#23429=CARTESIAN_POINT ( 'NONE',  ( 17.91453291880564080, 1458.959407450137860, 216.8828771306792191 ) ) ;
#23430=CARTESIAN_POINT ( 'NONE',  ( 1.799588937954729850, 1431.296473388759978, 200.2099206183030162 ) ) ;
#23436=EDGE_CURVE ( 'NONE', #88852, #1678, #32199, .T. ) ;
#23452=CARTESIAN_POINT ( 'NONE',  ( 7.502917382035859895, 1425.357894886970143, 212.2409982979840208 ) ) ;
#23465=ORIENTED_EDGE ( 'NONE', *, *, #95662, .T. ) ;
#23481=ORIENTED_EDGE ( 'NONE', *, *, #62860, .F. ) ;
#23488=CARTESIAN_POINT ( 'NONE',  ( 6.445177767125850110, 1483.523613335260052, 219.0471454115900087 ) ) ;
#23490=CARTESIAN_POINT ( 'NONE',  ( 8.236825666079377939, 1479.663677487053747, 202.5474313781959950 ) ) ;
#23492=CARTESIAN_POINT ( 'NONE',  ( -10.84028572272250024, 1480.780801381620222, 210.8784252212099943 ) ) ;
#23496=CARTESIAN_POINT ( 'NONE',  ( 7.431520146699999607, 1422.886000214980186, 195.6153521392990058 ) ) ;
#23498=CARTESIAN_POINT ( 'NONE',  ( -11.38101510873019961, 1491.910250263850230, 204.5016764512789962 ) ) ;
#23499=CARTESIAN_POINT ( 'NONE',  ( 10.76386117010460097, 1478.973846364719975, 205.9615306354030224 ) ) ;
#23507=ORIENTED_EDGE ( 'NONE', *, *, #74271, .F. ) ;
#23512=CARTESIAN_POINT ( 'NONE',  ( 10.03585564278080078, 1426.955176195429885, 209.6792063305699969 ) ) ;
#23513=CARTESIAN_POINT ( 'NONE',  ( 12.16717212215749910, 1426.186041745560033, 202.7890921220440248 ) ) ;
#23517=CARTESIAN_POINT ( 'NONE',  ( -8.053024569705350189, 1477.121180019175654, 215.6798857060248622 ) ) ;
#23521=CARTESIAN_POINT ( 'NONE',  ( -16.80834505000999712, 1420.460051406040066, 203.2687812860760062 ) ) ;
#23523=CARTESIAN_POINT ( 'NONE',  ( 5.945385552781929484, 1466.587269241879994, 217.1256145497779926 ) ) ;
#23525=CARTESIAN_POINT ( 'NONE',  ( -10.01326586723869916, 1481.014341800280135, 205.7823588363200145 ) ) ;
#23526=CARTESIAN_POINT ( 'NONE',  ( 2.644243049506179943, 1474.633123746480123, 220.2308870144509854 ) ) ;
#23527=CARTESIAN_POINT ( 'NONE',  ( 3.313501335607582643, 1397.551704408390151, 215.1871694724064810 ) ) ;
#23529=CARTESIAN_POINT ( 'NONE',  ( -7.351095455360000308, 1491.337165262789995, 211.7591980188690002 ) ) ;
#23535=CARTESIAN_POINT ( 'NONE',  ( -19.04700355086820096, 1444.155872664750177, 199.5980004632280043 ) ) ;
#23550=CARTESIAN_POINT ( 'NONE',  ( -10.90040294519999975, 1492.525757351089851, 207.2558712963190146 ) ) ;
#23551=EDGE_CURVE ( 'NONE', #38761, #13254, #107932, .T. ) ;
#23552=CARTESIAN_POINT ( 'NONE',  ( 2.123005411769999906, 1469.492284959789913, 189.2609491558989987 ) ) ;
#23554=FACE_OUTER_BOUND ( 'NONE', #69817, .T. ) ;
#23559=CARTESIAN_POINT ( 'NONE',  ( 11.20703803478759930, 1426.374986909809877, 206.7608603490599819 ) ) ;
#23564=EDGE_LOOP ( 'NONE', ( #49947, #75689, #100976, #31666 ) ) ;
#23565=CARTESIAN_POINT ( 'NONE',  ( 3.790668365970000231, 1474.135722993289846, 219.4689549067989844 ) ) ;
#23566=CARTESIAN_POINT ( 'NONE',  ( 10.71811212121339807, 1471.486163717210047, 211.4980701100689942 ) ) ;
#23575=CARTESIAN_POINT ( 'NONE',  ( 9.145064070970001069, 1450.428955669789957, 207.9342079490990045 ) ) ;
#23577=EDGE_CURVE ( 'NONE', #35203, #25053, #40243, .T. ) ;
#23593=CARTESIAN_POINT ( 'NONE',  ( -0.9396743887285590180, 1486.122836457870108, 220.9886464860670117 ) ) ;
#23606=CARTESIAN_POINT ( 'NONE',  ( -21.51339057090000040, 1505.551704408389924, 209.1218459616989946 ) ) ;
#23607=ADVANCED_FACE ( 'NONE', ( #86277 ), #100211, .T. ) ;
#23609=ORIENTED_EDGE ( 'NONE', *, *, #16496, .T. ) ;
#23611=DIRECTION ( 'NONE',  ( 1.000000000000000000, 0.000000000000000000, 0.000000000000000000 ) ) ;
#23612=CARTESIAN_POINT ( 'NONE',  ( 10.41388400344690091, 1453.143260227160226, 211.1213780663029809 ) ) ;
#23615=CARTESIAN_POINT ( 'NONE',  ( -2.330134127310790060, 1515.064792882719985, 213.4512947379739956 ) ) ;
#23618=VECTOR ( 'NONE', #50524, 999.9999999999998863 ) ;
#23622=CARTESIAN_POINT ( 'NONE',  ( -19.96011951328586420, 1485.861506872206974, 214.4463820970520374 ) ) ;
#23637=CARTESIAN_POINT ( 'NONE',  ( -17.59976141832330043, 1419.797097700060021, 206.6695233765389901 ) ) ;
#23638=CARTESIAN_POINT ( 'NONE',  ( -9.362058791585690543, 1461.114539333109860, 206.6197382024370199 ) ) ;
#23640=CARTESIAN_POINT ( 'NONE',  ( 9.987216885397780075, 1469.109414354970113, 207.4754563298509993 ) ) ;
#23641=CARTESIAN_POINT ( 'NONE',  ( 7.443246446248299009, 1423.092341332710021, 195.6161848952980051 ) ) ;
#23646=CARTESIAN_POINT ( 'NONE',  ( 19.79329231029999647, 1474.474811148189929, 213.0571447478990024 ) ) ;
#23658=CARTESIAN_POINT ( 'NONE',  ( 2.413234528069999829, 1507.615208039690060, 220.6132374451989904 ) ) ;
#23660=FACE_OUTER_BOUND ( 'NONE', #41576, .T. ) ;
#23661=CARTESIAN_POINT ( 'NONE',  ( -5.618830611241669715, 1441.039434150369743, 202.2715367274489893 ) ) ;
#23663=CARTESIAN_POINT ( 'NONE',  ( -4.244126290243009691, 1428.207434869309964, 200.7816286936110259 ) ) ;
#23664=CARTESIAN_POINT ( 'NONE',  ( -4.999835795559509855, 1447.920857802409955, 212.7698679858029891 ) ) ;
#23667=CARTESIAN_POINT ( 'NONE',  ( -6.121215447810000043, 1471.624333221390089, 212.8646130425990179 ) ) ;
#23672=CARTESIAN_POINT ( 'NONE',  ( 10.90953519108039949, 1489.918727231739922, 208.2510843807270078 ) ) ;
#23675=CARTESIAN_POINT ( 'NONE',  ( -11.41676025498539815, 1482.775671442730072, 205.7339583212410048 ) ) ;
#23677=CARTESIAN_POINT ( 'NONE',  ( -14.58700458240000053, 1416.104883097150150, 204.1284875012190128 ) ) ;
#23681=CARTESIAN_POINT ( 'NONE',  ( -4.282693164180000345, 1515.349926011190064, 210.2223588092890054 ) ) ;
#23698=CARTESIAN_POINT ( 'NONE',  ( 12.53106854449860030, 1421.570172124900182, 207.2100616318859920 ) ) ;
#23699=CARTESIAN_POINT ( 'NONE',  ( 10.10120055931009908, 1480.591734632540010, 206.1129840487050160 ) ) ;
#23701=EDGE_LOOP ( 'NONE', ( #66557, #55785, #81306, #56138 ) ) ;
#23704=CARTESIAN_POINT ( 'NONE',  ( 14.43085696104800064, 1426.807557148669957, 195.4949581798340148 ) ) ;
#23709=CARTESIAN_POINT ( 'NONE',  ( -5.334733590569999073, 1453.182326120890139, 200.0999779489789887 ) ) ;
#23714=CARTESIAN_POINT ( 'NONE',  ( -18.61832818047690097, 1419.362210733380152, 205.9667898552229985 ) ) ;
#23728=CARTESIAN_POINT ( 'NONE',  ( 0.2567668993620010331, 1444.957971160790066, 199.0403769168990209 ) ) ;
#23731=CARTESIAN_POINT ( 'NONE',  ( -4.748715079035791042, 1463.075537724480000, 200.5807050376280074 ) ) ;
#23732=CARTESIAN_POINT ( 'NONE',  ( -17.47648986376090008, 1417.884872443149789, 206.9675092925560023 ) ) ;
#23740=ORIENTED_EDGE ( 'NONE', *, *, #64067, .F. ) ;
#23747=EDGE_LOOP ( 'NONE', ( #11255, #77715, #18240, #106247, #18914, #11264, #100383 ) ) ;
#23748=CARTESIAN_POINT ( 'NONE',  ( -11.74584741039999969, 1503.658473360889957, 208.1214727982489876 ) ) ;
#23752=ORIENTED_EDGE ( 'NONE', *, *, #37154, .T. ) ;
#23773=CARTESIAN_POINT ( 'NONE',  ( -9.789290102761340151, 1501.631178984691360, 228.6396138205003012 ) ) ;
#23779=CARTESIAN_POINT ( 'NONE',  ( 11.76014171143800091, 1479.338753478690023, 208.6264959333659874 ) ) ;
#23781=CARTESIAN_POINT ( 'NONE',  ( 4.957272291311130452, 1484.564628183469949, 219.0507141408710083 ) ) ;
#23782=CARTESIAN_POINT ( 'NONE',  ( -6.119584447340000288, 1461.516739343589961, 206.9548908960190090 ) ) ;
#23793=CARTESIAN_POINT ( 'NONE',  ( 10.92329970540940032, 1461.467203400760127, 210.0859975044730277 ) ) ;
#23794=CARTESIAN_POINT ( 'NONE',  ( 12.51045652733512981, 1414.677402202029953, 211.4999743317719663 ) ) ;
#23809=CARTESIAN_POINT ( 'NONE',  ( -5.443435778090000454, 1484.664955501689974, 199.0097654132990215 ) ) ;
#23813=CARTESIAN_POINT ( 'NONE',  ( -8.638199857644998758, 1437.437583958759888, 209.7090198132510181 ) ) ;
#23828=CARTESIAN_POINT ( 'NONE',  ( 2.319193188279999873, 1454.536622715790145, 218.2400033011389837 ) ) ;
#23830=CARTESIAN_POINT ( 'NONE',  ( -6.605784529800000193, 1446.202031244890122, 215.7107487543390221 ) ) ;
#23833=CARTESIAN_POINT ( 'NONE',  ( -19.23853081770000273, 1466.576780668189940, 213.8528554934590034 ) ) ;
#23842=VERTEX_POINT ( 'NONE', #65933 ) ;
#23845=CARTESIAN_POINT ( 'NONE',  ( 24.08466742948269967, 1495.842384968879969, 206.9662854201800144 ) ) ;
#23847=CARTESIAN_POINT ( 'NONE',  ( -3.657993755839999750, 1474.872004365689918, 218.7367895275489786 ) ) ;
#23859=EDGE_LOOP ( 'NONE', ( #68084, #964, #21672, #6819 ) ) ;
#23880=FACE_OUTER_BOUND ( 'NONE', #66340, .T. ) ;
#23890=CARTESIAN_POINT ( 'NONE',  ( 3.991339022206620069, 1441.662322080260083, 217.1481258823889959 ) ) ;
#23895=CARTESIAN_POINT ( 'NONE',  ( -10.13788858020000028, 1473.082980680690071, 207.8827380507390217 ) ) ;
#23902=CARTESIAN_POINT ( 'NONE',  ( -9.573074595669998743, 1414.882314128850112, 207.6164979793489920 ) ) ;
#23904=CARTESIAN_POINT ( 'NONE',  ( 9.374206578739999074, 1489.420254891390186, 201.2494609442489946 ) ) ;
#23905=CARTESIAN_POINT ( 'NONE',  ( -3.420065937103660136, 1476.688851773250008, 199.3353256554640041 ) ) ;
#23912=B_SPLINE_SURFACE_WITH_KNOTS ( 'NONE', 5, 5, ( 
 ( #92793, #22810, #41298, #74372, #23378, #58111 ),
 ( #30686, #64872, #91692, #98980, #48614, #83295 ),
 ( #32879, #39646, #40740, #14968, #58657, #31784 ),
 ( #65975, #73815, #100098, #49162, #6590, #16065 ),
 ( #74916, #50268, #109066, #23916, #107943, #24469 ),
 ( #56453, #66527, #67069, #82187, #100631, #101175 ),
 ( #84398, #92244, #49711, #41843, #7685, #107389 ),
 ( #90588, #13865, #5487, #31235, #65418, #99525 ),
 ( #57017, #91142, #14419, #101730, #93885, #53023 ) ),
 .UNSPECIFIED., .F., .F., .F.,
 ( 6, 3, 6 ),
 ( 6, 6 ),
 ( 4.070471747090000036, 8.034185059020000352, 13.29188982760000037 ),
 ( 0.000000000000000000, 2.000000000000000000 ),
 .UNSPECIFIED. ) ;
#23913=CARTESIAN_POINT ( 'NONE',  ( -16.61546743539999937, 1420.545275466900193, 203.3817927211090080 ) ) ;
#23916=CARTESIAN_POINT ( 'NONE',  ( -1.100961233750000101, 1475.184615464690069, 219.7712113178990023 ) ) ;
#23917=DIRECTION ( 'NONE',  ( 0.000000000000000000, 1.000000000000000000, -1.836970198721029688E-16 ) ) ;
#23919=CARTESIAN_POINT ( 'NONE',  ( -11.31495002440830078, 1471.132454865509999, 207.6217866740839781 ) ) ;
#23923=CARTESIAN_POINT ( 'NONE',  ( 0.5238578764187010739, 1455.924360441900035, 198.5814542928440289 ) ) ;
#23928=CARTESIAN_POINT ( 'NONE',  ( 4.327230971739109755, 1515.149487411880045, 208.7301753859959774 ) ) ;
#23933=CARTESIAN_POINT ( 'NONE',  ( -4.775348822359999801, 1443.097051919790147, 200.2639737031189782 ) ) ;
#23937=CARTESIAN_POINT ( 'NONE',  ( -0.6435652335515109623, 1508.551704408389924, 220.0605423497629829 ) ) ;
#23943=CARTESIAN_POINT ( 'NONE',  ( 11.08064054948859933, 1491.588519825060075, 210.5260817967020159 ) ) ;
#23944=CARTESIAN_POINT ( 'NONE',  ( 0.08652916374279870371, 1456.779921165790029, 219.3623944633989993 ) ) ;
#23949=ORIENTED_EDGE ( 'NONE', *, *, #73711, .T. ) ;
#23953=CARTESIAN_POINT ( 'NONE',  ( -3.778541329980729557, 1515.551842520359969, 205.7532489892629997 ) ) ;
#23954=CARTESIAN_POINT ( 'NONE',  ( -11.87761131804900039, 1481.971403308739809, 208.7488170094680129 ) ) ;
#23957=CARTESIAN_POINT ( 'NONE',  ( 11.76839603954939939, 1479.635942723670041, 209.6667243029050098 ) ) ;
#23961=CARTESIAN_POINT ( 'NONE',  ( -16.16605818406190309, 1508.551704408389924, 213.6368797843010157 ) ) ;
#23964=CARTESIAN_POINT ( 'NONE',  ( 10.65100542576229437, 1461.074092667963441, 226.0091726112900403 ) ) ;
#23965=CARTESIAN_POINT ( 'NONE',  ( 1.515247566503459931, 1431.991194283580171, 200.7184132697910002 ) ) ;
#23969=VERTEX_POINT ( 'NONE', #6002 ) ;
#23974=CARTESIAN_POINT ( 'NONE',  ( -13.08802352330000041, 1503.233211745590097, 208.6735908916250253 ) ) ;
#23976=CARTESIAN_POINT ( 'NONE',  ( 0.9225549254600009519, 1476.549448786289986, 198.3955259652989866 ) ) ;
#23980=CARTESIAN_POINT ( 'NONE',  ( 17.01540922059999872, 1497.106364323189837, 222.9636020297990058 ) ) ;
#23981=CARTESIAN_POINT ( 'NONE',  ( 2.738034649980079838, 1428.914299196640059, 216.9389116324280167 ) ) ;
#23986=CARTESIAN_POINT ( 'NONE',  ( 7.466935644698990515, 1425.252733620679919, 212.3145299656949874 ) ) ;
#24000=CARTESIAN_POINT ( 'NONE',  ( 9.677596946179999549, 1463.237936564790061, 210.5383604994590030 ) ) ;
#24017=ORIENTED_EDGE ( 'NONE', *, *, #29949, .F. ) ;
#24019=CARTESIAN_POINT ( 'NONE',  ( -0.2511677605985540018, 1444.763459584839893, 199.0663387163230027 ) ) ;
#24022=CARTESIAN_POINT ( 'NONE',  ( 4.987082680427550763, 1508.551704408389924, 205.8487925209399805 ) ) ;
#24023=CARTESIAN_POINT ( 'NONE',  ( 5.428693282926851715, 1434.565645669088553, 202.5455567000074950 ) ) ;
#24025=CARTESIAN_POINT ( 'NONE',  ( 10.06093830045220194, 1503.068099882679917, 216.9326386128159925 ) ) ;
#24026=CARTESIAN_POINT ( 'NONE',  ( 8.268376058639999471, 1421.225653048179993, 196.1217719269989743 ) ) ;
#24029=CARTESIAN_POINT ( 'NONE',  ( -4.855393136690000055, 1495.916459891889872, 198.8750123678989894 ) ) ;
#24034=CARTESIAN_POINT ( 'NONE',  ( 10.94058267569030107, 1425.550681174790043, 206.5022529322419871 ) ) ;
#24047=CARTESIAN_POINT ( 'NONE',  ( 9.996610684277881020, 1422.882004021880221, 210.0220379297240072 ) ) ;
#24048=CARTESIAN_POINT ( 'NONE',  ( 10.95736455730619952, 1423.486173266069954, 203.2510385470160088 ) ) ;
#24050=CARTESIAN_POINT ( 'NONE',  ( -10.94864045059309987, 1462.689136093790239, 207.6212922226960131 ) ) ;
#24068=CARTESIAN_POINT ( 'NONE',  ( 4.806901123144410257E-05, 1416.181292948460168, 209.1218310849390036 ) ) ;
#24069=CARTESIAN_POINT ( 'NONE',  ( 0.7508624519860009894, 1515.469918561890154, 204.9042454670689892 ) ) ;
#24072=CARTESIAN_POINT ( 'NONE',  ( 20.10528725740779876, 1430.878053006679920, 215.1856555508250040 ) ) ;
#24078=ORIENTED_EDGE ( 'NONE', *, *, #87815, .T. ) ;
#24085=CARTESIAN_POINT ( 'NONE',  ( -1.119918677100000037, 1484.477289159689917, 198.4557079161989748 ) ) ;
#24089=EDGE_CURVE ( 'NONE', #41219, #101100, #6128, .T. ) ;
#24090=CARTESIAN_POINT ( 'NONE',  ( 6.768931428559999297, 1468.810414616219987, 208.2491176692980162 ) ) ;
#24096=CARTESIAN_POINT ( 'NONE',  ( 12.35725348643379995, 1421.674275332549996, 207.8249747856479814 ) ) ;
#24097=EDGE_CURVE ( 'NONE', #68962, #37552, #39463, .T. ) ;
#24102=FACE_OUTER_BOUND ( 'NONE', #43455, .T. ) ;
#24103=CARTESIAN_POINT ( 'NONE',  ( 18.20623948849710061, 1429.807643283219932, 209.5135666361939855 ) ) ;
#24105=CARTESIAN_POINT ( 'NONE',  ( -2.664535259099999805E-15, 1424.786834349990158, 209.1218459616989946 ) ) ;
#24110=DIRECTION ( 'NONE',  ( 0.8809280347472114858, -0.3866361631380628161, 0.2729070811655368578 ) ) ;
#24114=CARTESIAN_POINT ( 'NONE',  ( -1.491852088959999989, 1457.030208651289740, 199.7005471962389720 ) ) ;
#24118=AXIS2_PLACEMENT_3D ( 'NONE', #20232, #89644, #54433 ) ;
#24121=B_SPLINE_CURVE_WITH_KNOTS ( 'NONE', 5,
 ( #9578, #58902, #102524, #101976, #85185, #7928 ),
 .UNSPECIFIED., .F., .F.,
 ( 6, 6 ),
 ( 171.9180602750000162, 176.6690472260000035 ),
 .UNSPECIFIED. ) ;
#24127=CARTESIAN_POINT ( 'NONE',  ( 12.68801089449999964, 1500.413651719489962, 208.6561537547790124 ) ) ;
#24135=CARTESIAN_POINT ( 'NONE',  ( -3.829620088063210748, 1515.551704408389696, 212.3304832847908017 ) ) ;
#24138=CARTESIAN_POINT ( 'NONE',  ( 4.983582722859440040, 1508.551704408389924, 211.7624053699070146 ) ) ;
#24141=CARTESIAN_POINT ( 'NONE',  ( 19.12715434829999950, 1496.834837384790035, 222.0421819495990121 ) ) ;
#24148=CARTESIAN_POINT ( 'NONE',  ( -5.943657091278290672, 1507.986285603529950, 220.5847158657419982 ) ) ;
#24149=CARTESIAN_POINT ( 'NONE',  ( -18.42841025093079921, 1508.451658788899977, 209.8501139522570043 ) ) ;
#24150=CARTESIAN_POINT ( 'NONE',  ( 4.261736551909999449, 1515.372048949689997, 210.9648081929590262 ) ) ;
#24163=EDGE_CURVE ( 'NONE', #63442, #15989, #102309, .T. ) ;
#24169=CIRCLE ( 'NONE', #86772, 7.500000000000000000 ) ;
#24170=CARTESIAN_POINT ( 'NONE',  ( -9.957211913627739719, 1462.411460094509948, 206.9659526157329879 ) ) ;
#24174=CARTESIAN_POINT ( 'NONE',  ( -10.03141690779999884, 1472.765117886789994, 207.2972482850190090 ) ) ;
#24175=CARTESIAN_POINT ( 'NONE',  ( 7.459255098270000772, 1492.932273812890116, 217.3740738590289823 ) ) ;
#24180=LINE ( 'NONE', #57288, #23618 ) ;
#24188=EDGE_CURVE ( 'NONE', #88662, #35462, #27566, .T. ) ;
#24189=CARTESIAN_POINT ( 'NONE',  ( 4.020407408656390125, 1515.375307573260216, 212.6641671072679856 ) ) ;
#24192=CARTESIAN_POINT ( 'NONE',  ( -12.39813691047029920, 1501.849957302749999, 211.5949719684760169 ) ) ;
#24193=ORIENTED_EDGE ( 'NONE', *, *, #108, .T. ) ;
#24194=CARTESIAN_POINT ( 'NONE',  ( -15.59626543754127859, 1415.697927852701469, 209.6280133318726371 ) ) ;
#24198=CARTESIAN_POINT ( 'NONE',  ( 3.335053448420000066, 1435.130189762789996, 227.2785100434990113 ) ) ;
#24200=CARTESIAN_POINT ( 'NONE',  ( -18.31482527320000031, 1445.278739201789904, 204.5307550449689984 ) ) ;
#24201=CARTESIAN_POINT ( 'NONE',  ( -8.214410069903289369, 1425.179819099440010, 204.7529498726069903 ) ) ;
#24202=CARTESIAN_POINT ( 'NONE',  ( 4.989246313819999834, 1471.909539260290103, 189.7082128665990126 ) ) ;
#24205=CARTESIAN_POINT ( 'NONE',  ( -11.49997733492739904, 1482.708633644570000, 206.0163858927470244 ) ) ;
#24215=CARTESIAN_POINT ( 'NONE',  ( 3.782892722810800468, 1454.105688421529976, 217.7082469129449862 ) ) ;
#24218=CARTESIAN_POINT ( 'NONE',  ( -10.76610293753739889, 1461.751116445120033, 211.3389343603909936 ) ) ;
#24221=CARTESIAN_POINT ( 'NONE',  ( -8.644357649085678830, 1437.214323335709878, 209.1429500785100117 ) ) ;
#24222=CARTESIAN_POINT ( 'NONE',  ( -5.363702833240000523, 1497.797094973989942, 219.9207493420989863 ) ) ;
#24232=EDGE_CURVE ( 'NONE', #27509, #63858, #96992, .T. ) ;
#24249=CARTESIAN_POINT ( 'NONE',  ( -17.44087122180000193, 1443.080660932889941, 219.4520116906990097 ) ) ;
#24252=CARTESIAN_POINT ( 'NONE',  ( -9.104803454178981070, 1421.479062530849887, 192.1853131694120123 ) ) ;
#24254=CARTESIAN_POINT ( 'NONE',  ( -2.487935098691028912, 1508.731359868551181, 204.5668839584545537 ) ) ;
#24256=DIRECTION ( 'NONE',  ( 2.491197269910784929E-47, 1.000000000000000000, -1.836970198721029688E-16 ) ) ;
#24257=CARTESIAN_POINT ( 'NONE',  ( 10.23405869452090045, 1451.409005433660013, 206.7712507236010140 ) ) ;
#24275=CARTESIAN_POINT ( 'NONE',  ( 4.082778200585179817, 1515.071394777460000, 205.5355244017910081 ) ) ;
#24276=CARTESIAN_POINT ( 'NONE',  ( 0.2645265605250010088, 1443.121736177289904, 200.2023345980989859 ) ) ;
#24282=( LENGTH_UNIT ( ) NAMED_UNIT ( * ) SI_UNIT ( .MILLI., .METRE. ) );
#24288=VERTEX_POINT ( 'NONE', #10709 ) ;
#24297=B_SPLINE_CURVE_WITH_KNOTS ( 'NONE', 5,
 ( #71250, #88037, #17042, #20786, #26010, #60207, #105373, #94326, #33877 ),
 .UNSPECIFIED., .F., .F.,
 ( 6, 3, 6 ),
 ( 0.000000000000000000, 0.4555160169310293328, 1.000000000000000000 ),
 .UNSPECIFIED. ) ;
#24299=CARTESIAN_POINT ( 'NONE',  ( -11.92597359959999892, 1502.382029717889964, 208.7016622767430079 ) ) ;
#24306=ORIENTED_EDGE ( 'NONE', *, *, #94927, .F. ) ;
#24314=CARTESIAN_POINT ( 'NONE',  ( -15.89125153416810043, 1508.551704408389924, 210.3764243748509841 ) ) ;
#24322=CARTESIAN_POINT ( 'NONE',  ( 2.833473913299999758, 1441.452951622389946, 218.6297931320189889 ) ) ;
#24325=CARTESIAN_POINT ( 'NONE',  ( 9.477234549875239722, 1434.583635821490134, 206.7094033099960200 ) ) ;
#24327=DIRECTION ( 'NONE',  ( 0.000000000000000000, -1.000000000000000000, 1.836970198721029688E-16 ) ) ;
#24336=CARTESIAN_POINT ( 'NONE',  ( -1.334110822913096461, 1494.791028558611742, 220.2012359351212183 ) ) ;
#24337=CARTESIAN_POINT ( 'NONE',  ( 6.140260223881050194, 1484.047191686760016, 218.4413122911290088 ) ) ;
#24339=CARTESIAN_POINT ( 'NONE',  ( -1.073559340110749938, 1444.993510080170154, 218.0402162255370229 ) ) ;
#24342=CARTESIAN_POINT ( 'NONE',  ( -9.134223394739478863, 1449.159919330089906, 209.9164564190560043 ) ) ;
#24349=CARTESIAN_POINT ( 'NONE',  ( 10.95484118540970009, 1461.213211890040157, 209.4073241984519882 ) ) ;
#24350=CARTESIAN_POINT ( 'NONE',  ( 4.653713395369999617, 1466.070346627889876, 218.6934685164889913 ) ) ;
#24358=CARTESIAN_POINT ( 'NONE',  ( 4.449447964721140458, 1507.123567759500020, 219.9414455400390125 ) ) ;
#24361=CARTESIAN_POINT ( 'NONE',  ( -9.526144281750038800, 1440.436505751970117, 205.9995517796429851 ) ) ;
#24362=CARTESIAN_POINT ( 'NONE',  ( 5.456719627610000067, 1455.595244131089885, 218.2350948550090095 ) ) ;
#24363=LINE ( 'NONE', #25457, #98558 ) ;
#24368=CARTESIAN_POINT ( 'NONE',  ( -8.674200344734190438, 1437.754171787169980, 209.1145358281810047 ) ) ;
#24369=CARTESIAN_POINT ( 'NONE',  ( -3.982959088878220033, 1515.551843419129909, 211.9714090624810012 ) ) ;
#24379=DIRECTION ( 'NONE',  ( -6.922360974429999144E-17, -1.000000000000000000, 2.302693041820029802E-16 ) ) ;
#24382=CARTESIAN_POINT ( 'NONE',  ( -12.78943350980000027, 1502.708798922290043, 209.0180533589250160 ) ) ;
#24384=CARTESIAN_POINT ( 'NONE',  ( 4.035142546699999500, 1455.426291782089947, 218.0958705512090035 ) ) ;
#24386=B_SPLINE_CURVE_WITH_KNOTS ( 'NONE', 5,
 ( #91909, #84606, #57789, #33102, #16280, #49373, #65633, #99194, #56674 ),
 .UNSPECIFIED., .F., .F.,
 ( 6, 3, 6 ),
 ( 0.000000000000000000, 0.4999999999999998335, 1.000000000000000000 ),
 .UNSPECIFIED. ) ;
#24387=CARTESIAN_POINT ( 'NONE',  ( -7.550047457009999796, 1446.700195908890009, 214.6466464486289851 ) ) ;
#24390=CARTESIAN_POINT ( 'NONE',  ( 9.717824533310780666, 1463.678478211699939, 210.3770741684630252 ) ) ;
#24391=CARTESIAN_POINT ( 'NONE',  ( 7.911464481230000345, 1423.187191425399988, 213.2893462354790017 ) ) ;
#24402=CARTESIAN_POINT ( 'NONE',  ( 0.1080666684629969926, 1502.828674633789888, 233.2928853222989858 ) ) ;
#24407=CARTESIAN_POINT ( 'NONE',  ( 18.00963447456260269, 1431.117864245919918, 206.0875853561470024 ) ) ;
#24410=CARTESIAN_POINT ( 'NONE',  ( -9.077803069467520913, 1448.962985536510132, 210.3449884047199987 ) ) ;
#24415=DIRECTION ( 'NONE',  ( 0.9109019969992648846, -0.3842787907060009056, -0.1502909274583290045 ) ) ;
#24416=ORIENTED_EDGE ( 'NONE', *, *, #881, .F. ) ;
#24419=CARTESIAN_POINT ( 'NONE',  ( 9.297632061492119959, 1425.336027861749926, 195.2545234328350148 ) ) ;
#24424=VERTEX_POINT ( 'NONE', #29153 ) ;
#24432=ORIENTED_EDGE ( 'NONE', *, *, #4394, .T. ) ;
#24436=CARTESIAN_POINT ( 'NONE',  ( 0.8756585369989179357, 1425.746450835400083, 191.1126529878390272 ) ) ;
#24440=CARTESIAN_POINT ( 'NONE',  ( 1.145290945507940084, 1458.110487998910003, 199.6352770989870180 ) ) ;
#24448=CARTESIAN_POINT ( 'NONE',  ( -10.16826309620000224, 1472.406893517490062, 208.4967702181029665 ) ) ;
#24454=CARTESIAN_POINT ( 'NONE',  ( -4.119767774860000564, 1413.537972784140266, 207.3346887680889949 ) ) ;
#24456=CARTESIAN_POINT ( 'NONE',  ( 4.989613516749999533, 1487.671035670790161, 198.1975016566989893 ) ) ;
#24457=CARTESIAN_POINT ( 'NONE',  ( 2.356294384139039799, 1431.021013722109956, 218.3169074369490090 ) ) ;
#24466=CARTESIAN_POINT ( 'NONE',  ( -16.76646998270000211, 1420.451233668469968, 203.6167452475490052 ) ) ;
#24468=ADVANCED_FACE ( 'NONE', ( #105872 ), #168, .T. ) ;
#24469=CARTESIAN_POINT ( 'NONE',  ( -1.062402653849999989, 1475.637717254689960, 220.5408259888989733 ) ) ;
#24472=CARTESIAN_POINT ( 'NONE',  ( 1.133338450661860008, 1423.755929587430046, 191.2144893514050068 ) ) ;
#24473=CARTESIAN_POINT ( 'NONE',  ( -11.39934036035690035, 1470.872822770500079, 208.6597014105470294 ) ) ;
#24474=CARTESIAN_POINT ( 'NONE',  ( -5.382670666700607676, 1508.259648345004507, 220.3115702328250336 ) ) ;
#24481=CARTESIAN_POINT ( 'NONE',  ( -10.54622137524750158, 1471.119434090909863, 209.8143280353739897 ) ) ;
#24492=CARTESIAN_POINT ( 'NONE',  ( -2.074768463076620328, 1486.986234437389840, 220.1251915955149911 ) ) ;
#24493=CARTESIAN_POINT ( 'NONE',  ( -4.015749066599999750, 1515.588778490289997, 208.3687103823360189 ) ) ;
#24497=CARTESIAN_POINT ( 'NONE',  ( 10.95202006776319870, 1490.978190374230053, 210.0828909271359919 ) ) ;
#24498=CARTESIAN_POINT ( 'NONE',  ( -2.788614694270000083, 1456.607942948890013, 218.2023089652089993 ) ) ;
#24508=CARTESIAN_POINT ( 'NONE',  ( 1.161830502209999949, 1469.358622120289965, 189.0813358120989847 ) ) ;
#24509=CARTESIAN_POINT ( 'NONE',  ( -6.973120769980000411, 1462.078774314090197, 202.2276825251889818 ) ) ;
#24514=LINE ( 'NONE', #58703, #44216 ) ;
#24518=CARTESIAN_POINT ( 'NONE',  ( 6.050886996877059332, 1433.308159904890090, 202.4648030222659827 ) ) ;
#24522=VERTEX_POINT ( 'NONE', #38540 ) ;
#24530=FACE_OUTER_BOUND ( 'NONE', #95588, .T. ) ;
#24536=CARTESIAN_POINT ( 'NONE',  ( -8.700499408960000736, 1424.079320566130036, 207.5589903581490034 ) ) ;
#24540=CARTESIAN_POINT ( 'NONE',  ( 7.354254828809129840, 1426.340165684199974, 212.6766371994280007 ) ) ;
#24542=ORIENTED_EDGE ( 'NONE', *, *, #7637, .F. ) ;
#24546=CARTESIAN_POINT ( 'NONE',  ( -0.9691334048877314755, 1488.056577045728773, 219.9420655526842552 ) ) ;
#24549=CARTESIAN_POINT ( 'NONE',  ( 3.401541474470889614, 1468.225229937070026, 218.5224292273400124 ) ) ;
#24550=CARTESIAN_POINT ( 'NONE',  ( 18.19476890929999868, 1429.544292015390056, 208.2833220268470029 ) ) ;
#24551=ORIENTED_EDGE ( 'NONE', *, *, #19277, .T. ) ;
#24554=CARTESIAN_POINT ( 'NONE',  ( 9.808373588480000294, 1462.684821613489930, 210.4841290881089719 ) ) ;
#24558=ORIENTED_EDGE ( 'NONE', *, *, #87183, .F. ) ;
#24566=B_SPLINE_CURVE_WITH_KNOTS ( 'NONE', 3,
 ( #12785, #31783, #57016, #91690, #13307, #91141, #14418, #48611, #82744, #14967, #6037, #74370, #65974, #49161, #72177, #76415, #85920, #34960, #17019, #95433, #9224, #51218, #85349, #290, #51782, #43382, #70270, #68045, #17582, #10313, #59630, #104379, #36085, #33854, #102155, #77531, #25435 ),
 .UNSPECIFIED., .F., .F.,
 ( 4, 3, 3, 3, 3, 3, 3, 3, 3, 3, 3, 3, 4 ),
 ( -77.98062027567270604, -77.28570685305760435, -75.84252669430900085, -74.37770857730430407, -72.90452813415019762, -71.43163176466710240, -69.96926794057800691, -68.52392561414599470, -67.09989659765190595, -66.56132197703499287, -65.17789798084180575, -63.76799573968669677, -62.33963421229999824 ),
 .UNSPECIFIED. ) ;
#24569=ORIENTED_EDGE ( 'NONE', *, *, #56222, .F. ) ;
#24571=CARTESIAN_POINT ( 'NONE',  ( -0.6532060423541629079, 1444.609809648689861, 199.0872701831330005 ) ) ;
#24572=CARTESIAN_POINT ( 'NONE',  ( 4.069411599699999549, 1427.113643276370112, 212.3578269758590125 ) ) ;
#24574=CARTESIAN_POINT ( 'NONE',  ( -11.31803579276679983, 1481.249050730999897, 210.4920860573550101 ) ) ;
#24575=CARTESIAN_POINT ( 'NONE',  ( 5.380056979554551866, 1434.542470706314134, 202.5070600846412106 ) ) ;
#24577=CARTESIAN_POINT ( 'NONE',  ( 11.69850812630680004, 1502.052734125200232, 214.1386926423620025 ) ) ;
#24578=CARTESIAN_POINT ( 'NONE',  ( 7.758184319229999737, 1421.576654411539948, 195.8091089427989857 ) ) ;
#24580=CARTESIAN_POINT ( 'NONE',  ( 10.11567626329839875, 1479.961683375350049, 205.9716079530940078 ) ) ;
#24584=AXIS2_PLACEMENT_3D ( 'NONE', #71246, #3479, #103705 ) ;
#24588=ORIENTED_EDGE ( 'NONE', *, *, #54213, .F. ) ;
#24589=LINE ( 'NONE', #68310, #94541 ) ;
#24590=AXIS2_PLACEMENT_3D ( 'NONE', #27696, #55677, #79219 ) ;
#24593=CARTESIAN_POINT ( 'NONE',  ( 10.39728290242030084, 1427.483012415709936, 210.1624185323059919 ) ) ;
#24594=CARTESIAN_POINT ( 'NONE',  ( 10.94186774115649996, 1423.753146808589918, 203.2164765458729789 ) ) ;
#24602=CARTESIAN_POINT ( 'NONE',  ( 9.031927925652290412, 1421.291943124229874, 197.0056667342660148 ) ) ;
#24612=CARTESIAN_POINT ( 'NONE',  ( -19.86464710103360076, 1441.435714288719964, 212.6459465483729900 ) ) ;
#24613=CARTESIAN_POINT ( 'NONE',  ( -19.30744623537299987, 1418.880101625140014, 208.8299352253080201 ) ) ;
#24624=CARTESIAN_POINT ( 'NONE',  ( 10.84148007940000014, 1478.843050295790135, 205.9629258051089948 ) ) ;
#24628=CARTESIAN_POINT ( 'NONE',  ( -5.666956068895039778, 1433.164882934490151, 215.5009249933730189 ) ) ;
#24636=CARTESIAN_POINT ( 'NONE',  ( 12.14434402762229936, 1421.782244358430034, 208.4503354109049837 ) ) ;
#24640=CARTESIAN_POINT ( 'NONE',  ( 3.454899550169740152, 1437.151257404700118, 227.3279159481639908 ) ) ;
#24642=CARTESIAN_POINT ( 'NONE',  ( 4.134276593080000062, 1473.270938484690078, 218.6199709919989971 ) ) ;
#24645=CARTESIAN_POINT ( 'NONE',  ( -10.81171726419999857, 1492.479041299990058, 205.9913540356689907 ) ) ;
#24649=CARTESIAN_POINT ( 'NONE',  ( 1776.370103581280091, 5181.793945261120825, -8870.008376233501622 ) ) ;
#24650=CARTESIAN_POINT ( 'NONE',  ( 8.343671689369999811, 1449.263932163490153, 204.8140308564489942 ) ) ;
#24651=CARTESIAN_POINT ( 'NONE',  ( -21.48880489289999929, 1507.176470023590127, 211.5094435469989946 ) ) ;
#24652=CARTESIAN_POINT ( 'NONE',  ( -4.987078435459999071, 1509.051704408389924, 209.1218459616989946 ) ) ;
#24664=ORIENTED_EDGE ( 'NONE', *, *, #21486, .T. ) ;
#24674=EDGE_CURVE ( 'NONE', #86208, #50172, #105212, .T. ) ;
#24681=CARTESIAN_POINT ( 'NONE',  ( 4.902792406504040024, 1508.551704408389924, 212.2587853230709811 ) ) ;
#24684=CARTESIAN_POINT ( 'NONE',  ( -18.32377786700000399, 1464.077817829789865, 217.4721512913189940 ) ) ;
#24688=CARTESIAN_POINT ( 'NONE',  ( 1.332267629549999902E-15, 1412.913060387329779, 209.1218459616989946 ) ) ;
#24689=CARTESIAN_POINT ( 'NONE',  ( 10.55962377587460033, 1452.696006162120057, 209.8459794650469803 ) ) ;
#24690=CARTESIAN_POINT ( 'NONE',  ( -6.487810219224459551, 1508.114173656130106, 220.3031569931239915 ) ) ;
#24691=VECTOR ( 'NONE', #35719, 1000.000000000000000 ) ;
#24693=CARTESIAN_POINT ( 'NONE',  ( 4.201139955930000447, 1515.456931311890003, 210.2329862578490065 ) ) ;
#24704=ORIENTED_EDGE ( 'NONE', *, *, #70951, .F. ) ;
#24711=EDGE_CURVE ( 'NONE', #76707, #15508, #49173, .T. ) ;
#24712=CARTESIAN_POINT ( 'NONE',  ( -2.844617774716496239, 1488.558558072584219, 219.6378750350716587 ) ) ;
#24714=CARTESIAN_POINT ( 'NONE',  ( 9.905242068095489572, 1468.560492227489931, 207.6656469818879884 ) ) ;
#24715=FACE_OUTER_BOUND ( 'NONE', #103097, .T. ) ;
#24720=CARTESIAN_POINT ( 'NONE',  ( -21.63156322749999916, 1505.770867997990081, 209.2235208569570091 ) ) ;
#24721=CARTESIAN_POINT ( 'NONE',  ( 7.578766088578010596, 1467.899149354640031, 200.9046483899009843 ) ) ;
#24722=CARTESIAN_POINT ( 'NONE',  ( 6.753961865179999968, 1469.830701748189995, 210.2167338168290200 ) ) ;
#24725=EDGE_CURVE ( 'NONE', #106056, #2195, #74927, .T. ) ;
#24732=ORIENTED_EDGE ( 'NONE', *, *, #86267, .T. ) ;
#24734=CARTESIAN_POINT ( 'NONE',  ( 1.699897556570000079, 1508.551704408389924, 219.7511403508990213 ) ) ;
#24739=CARTESIAN_POINT ( 'NONE',  ( -4.663088608516360978, 1427.954664977100038, 201.0136482515530076 ) ) ;
#24742=CARTESIAN_POINT ( 'NONE',  ( -21.50400446119279962, 1505.467562055609960, 209.6175409707290100 ) ) ;
#24743=CARTESIAN_POINT ( 'NONE',  ( -16.00058974059999883, 1465.442699635990039, 221.9149816820990111 ) ) ;
#24755=CARTESIAN_POINT ( 'NONE',  ( -15.35926873949999916, 1415.632233529220002, 207.7221835180689880 ) ) ;
#24758=CARTESIAN_POINT ( 'NONE',  ( -16.30759486957349580, 1419.707542479528001, 209.7289770706684351 ) ) ;
#24759=CARTESIAN_POINT ( 'NONE',  ( -7.402577614759999314, 1497.624368088290112, 217.8806385702189914 ) ) ;
#24760=CARTESIAN_POINT ( 'NONE',  ( -0.7270621067209990240, 1477.679265261989940, 201.4865919325389996 ) ) ;
#24761=FACE_OUTER_BOUND ( 'NONE', #49649, .T. ) ;
#24764=CARTESIAN_POINT ( 'NONE',  ( -7.233415693649337008, 1421.233009521309668, 193.8023935178989916 ) ) ;
#24774=CARTESIAN_POINT ( 'NONE',  ( 4.873735476160000246, 1472.089320948289924, 218.0431589096889695 ) ) ;
#24779=CARTESIAN_POINT ( 'NONE',  ( 3.675002922379999593, 1484.816058337290087, 219.9704011141990350 ) ) ;
#24780=EDGE_CURVE ( 'NONE', #52522, #84750, #55544, .T. ) ;
#24781=CARTESIAN_POINT ( 'NONE',  ( 11.49453118813409880, 1478.838340461310054, 206.6810620774099903 ) ) ;
#24783=CARTESIAN_POINT ( 'NONE',  ( 11.82788503319999940, 1436.101494931290063, 225.5825002257989809 ) ) ;
#24785=CARTESIAN_POINT ( 'NONE',  ( -13.67844807081490011, 1504.250361896059985, 227.6838271028410077 ) ) ;
#24811=CARTESIAN_POINT ( 'NONE',  ( 3.375977098360000372, 1446.395221917490062, 199.5681764228489783 ) ) ;
#24817=CARTESIAN_POINT ( 'NONE',  ( 2.738491091690000268, 1419.583501618159971, 204.7124688696490011 ) ) ;
#24826=ORIENTED_EDGE ( 'NONE', *, *, #15487, .T. ) ;
#24831=CARTESIAN_POINT ( 'NONE',  ( -9.922940940763762541, 1473.528715622569734, 206.4586403660501901 ) ) ;
#24837=CARTESIAN_POINT ( 'NONE',  ( 11.19147557906589974, 1422.145537183640045, 210.4506353095700035 ) ) ;
#24841=ORIENTED_EDGE ( 'NONE', *, *, #53684, .T. ) ;
#24869=CARTESIAN_POINT ( 'NONE',  ( 8.800000000000002487, 1412.913060387329779, 209.1218459616989946 ) ) ;
#24870=CARTESIAN_POINT ( 'NONE',  ( -3.393167906721693328, 1495.486076169147736, 219.7910603749398604 ) ) ;
#24871=CARTESIAN_POINT ( 'NONE',  ( 12.55935747509999878, 1421.555442417790118, 207.1258153896989995 ) ) ;
#24880=B_SPLINE_SURFACE_WITH_KNOTS ( 'NONE', 5, 1, ( 
 ( #104401, #61882 ),
 ( #3077, #45076 ),
 ( #19267, #37204 ),
 ( #53470, #12547 ),
 ( #95998, #71948 ),
 ( #37756, #46726 ) ),
 .UNSPECIFIED., .F., .F., .F.,
 ( 6, 6 ),
 ( 2, 2 ),
 ( 0.000000000000000000, 17.60720389089999927 ),
 ( 0.000000000000000000, 14.00000000000000000 ),
 .UNSPECIFIED. ) ;
#24884=CARTESIAN_POINT ( 'NONE',  ( 4.244807866439999522, 1467.382213863189918, 218.1353146091890096 ) ) ;
#24897=EDGE_CURVE ( 'NONE', #77481, #31705, #81387, .T. ) ;
#24901=CARTESIAN_POINT ( 'NONE',  ( 11.79936509490000063, 1501.494630616190079, 210.6141959002089834 ) ) ;
#24906=CARTESIAN_POINT ( 'NONE',  ( 3.394586470828380165, 1484.752177860970050, 220.4731790445629827 ) ) ;
#24908=CARTESIAN_POINT ( 'NONE',  ( -7.135977434860000024, 1484.469329130889946, 199.5068056354589885 ) ) ;
#24917=CARTESIAN_POINT ( 'NONE',  ( 0.07780472814651649693, 1435.826791670900093, 227.5930969672339756 ) ) ;
#24918=CARTESIAN_POINT ( 'NONE',  ( -15.37131439997841120, 1416.019838768163936, 206.9134041253344662 ) ) ;
#24919=CARTESIAN_POINT ( 'NONE',  ( 2.254281109099999902, 1456.426090434989874, 219.5085644225989938 ) ) ;
#24921=CARTESIAN_POINT ( 'NONE',  ( -8.920901164470000921, 1446.486419407289986, 213.5435801750889766 ) ) ;
#24926=CARTESIAN_POINT ( 'NONE',  ( 6.917355500260000234, 1424.874072686129921, 213.3478120366190183 ) ) ;
#24928=CARTESIAN_POINT ( 'NONE',  ( -3.402680045398430053, 1454.224139754760017, 199.2091369326260235 ) ) ;
#24932=CARTESIAN_POINT ( 'NONE',  ( 3.902836639019999776, 1495.323243335989901, 220.8767694861990094 ) ) ;
#24952=CARTESIAN_POINT ( 'NONE',  ( -4.328706393743980030, 1515.093143318830244, 210.3280110370420175 ) ) ;
#24958=CARTESIAN_POINT ( 'NONE',  ( 5.441863932033339069, 1424.278296144239903, 193.3859063792879738 ) ) ;
#24962=CARTESIAN_POINT ( 'NONE',  ( -10.93162295028230169, 1470.132889486390013, 212.2376398131100075 ) ) ;
#24978=CARTESIAN_POINT ( 'NONE',  ( 3.973077635731362633, 1441.765784966813499, 217.0264645807230011 ) ) ;
#24988=CARTESIAN_POINT ( 'NONE',  ( -6.016757112579999678, 1449.943096111989917, 209.5823369759550019 ) ) ;
#24995=CARTESIAN_POINT ( 'NONE',  ( -10.17795364999999919, 1472.274701162789825, 208.9856853541390080 ) ) ;
#25002=CARTESIAN_POINT ( 'NONE',  ( -4.218809310280000169, 1413.234397187750119, 207.6255014893789905 ) ) ;
#25005=CARTESIAN_POINT ( 'NONE',  ( 5.387574631020000560, 1487.707168882490123, 198.8464060204989892 ) ) ;
#25008=VECTOR ( 'NONE', #16923, 1000.000000000000114 ) ;
#25015=CARTESIAN_POINT ( 'NONE',  ( -17.13546891859999732, 1420.255476167079905, 203.8193908791089939 ) ) ;
#25016=VERTEX_POINT ( 'NONE', #19957 ) ;
#25018=CARTESIAN_POINT ( 'NONE',  ( -17.13806402160000175, 1505.874291994889973, 209.1215054657809844 ) ) ;
#25021=CARTESIAN_POINT ( 'NONE',  ( -11.20494725878380038, 1471.318229655669938, 206.9400762973899930 ) ) ;
#25022=CARTESIAN_POINT ( 'NONE',  ( -5.036431363644181758, 1508.232884704754269, 220.4119323058353928 ) ) ;
#25029=CARTESIAN_POINT ( 'NONE',  ( -13.42843082903999985, 1417.384064304789945, 201.4800834699910297 ) ) ;
#25032=ORIENTED_EDGE ( 'NONE', *, *, #93122, .F. ) ;
#25035=CARTESIAN_POINT ( 'NONE',  ( -18.44417578049999662, 1443.022497311789948, 205.4505639164189859 ) ) ;
#25045=CARTESIAN_POINT ( 'NONE',  ( 11.13874570262469987, 1491.363259792560029, 209.7171445221170245 ) ) ;
#25046=CARTESIAN_POINT ( 'NONE',  ( 0.5688480841909990815, 1456.339328993690060, 218.9825356867290225 ) ) ;
#25049=B_SPLINE_SURFACE_WITH_KNOTS ( 'NONE', 5, 1, ( 
 ( #100736, #60431 ),
 ( #109712, #15073 ),
 ( #58218, #50915 ),
 ( #49269, #75023 ),
 ( #15615, #7252 ),
 ( #83396, #101836 ),
 ( #24572, #85046 ),
 ( #6694, #109174 ),
 ( #32460, #66635 ) ),
 .UNSPECIFIED., .F., .F., .F.,
 ( 6, 3, 6 ),
 ( 2, 2 ),
 ( 0.000000000000000000, 7.657578151330000082, 15.28728567399999960 ),
 ( 0.000000000000000000, 14.00000771804140065 ),
 .UNSPECIFIED. ) ;
#25051=CARTESIAN_POINT ( 'NONE',  ( -2.418973636230000057, 1431.127469431690088, 217.1544448978289950 ) ) ;
#25053=VERTEX_POINT ( 'NONE', #12112 ) ;
#25060=CARTESIAN_POINT ( 'NONE',  ( -10.17701436070000121, 1462.839837603090018, 206.1633447294989878 ) ) ;
#25063=FACE_OUTER_BOUND ( 'NONE', #43188, .T. ) ;
#25064=CARTESIAN_POINT ( 'NONE',  ( -14.07384742208520123, 1508.551704408389924, 215.7439646766590045 ) ) ;
#25072=VERTEX_POINT ( 'NONE', #3199 ) ;
#25073=CARTESIAN_POINT ( 'NONE',  ( 22.26425649109999938, 1476.353502809590054, 209.6940367010219859 ) ) ;
#25075=FACE_OUTER_BOUND ( 'NONE', #55392, .T. ) ;
#25079=EDGE_CURVE ( 'NONE', #17806, #75555, #54286, .T. ) ;
#25080=CARTESIAN_POINT ( 'NONE',  ( 9.326420915248059273, 1460.944044860930035, 206.0389257843339976 ) ) ;
#25082=CARTESIAN_POINT ( 'NONE',  ( -19.14812029890000034, 1505.318613837190014, 209.0594768593419985 ) ) ;
#25083=CARTESIAN_POINT ( 'NONE',  ( -1.756482616760000059, 1475.875686602589894, 198.5418275763989868 ) ) ;
#25089=CARTESIAN_POINT ( 'NONE',  ( -9.148257661150001496, 1423.748799908730007, 207.7944249153989915 ) ) ;
#25095=CARTESIAN_POINT ( 'NONE',  ( 7.438626391280539707, 1426.170359921889940, 212.4786103371660033 ) ) ;
#25105=CARTESIAN_POINT ( 'NONE',  ( 3.165859372309999920, 1420.089904188009996, 205.0081603533590169 ) ) ;
#25120=CARTESIAN_POINT ( 'NONE',  ( 4.491284065468319930, 1508.884228858900087, 211.6097700378190041 ) ) ;
#25127=ORIENTED_EDGE ( 'NONE', *, *, #68595, .T. ) ;
#25133=CARTESIAN_POINT ( 'NONE',  ( 4.554948924558070544, 1508.731372610989865, 206.6339222123599768 ) ) ;
#25134=CARTESIAN_POINT ( 'NONE',  ( 4.755330316939417656, 1434.245644035614077, 202.0163905304680441 ) ) ;
#25135=CARTESIAN_POINT ( 'NONE',  ( -4.554659022055290052, 1508.551704408389924, 213.0139469008600202 ) ) ;
#25137=CARTESIAN_POINT ( 'NONE',  ( 7.450392350589999602, 1422.132270461650251, 195.6329181414990046 ) ) ;
#25139=CARTESIAN_POINT ( 'NONE',  ( 10.81956120968489898, 1478.925883878960121, 205.9529814458820169 ) ) ;
#25146=ORIENTED_EDGE ( 'NONE', *, *, #80204, .F. ) ;
#25153=CARTESIAN_POINT ( 'NONE',  ( 8.877746755106400656, 1422.885059916349974, 212.4210226277380116 ) ) ;
#25154=CARTESIAN_POINT ( 'NONE',  ( 10.94861482359589999, 1423.583840232799957, 203.2386481640710088 ) ) ;
#25160=CARTESIAN_POINT ( 'NONE',  ( -10.53669503535969909, 1461.974058373740036, 209.9839194512770177 ) ) ;
#25162=CARTESIAN_POINT ( 'NONE',  ( -1.636741614903409969, 1469.777368438049962, 219.0527109355280118 ) ) ;
#25163=CARTESIAN_POINT ( 'NONE',  ( 5.896221088274059774, 1466.153673113790092, 217.3008473279559780 ) ) ;
#25169=CARTESIAN_POINT ( 'NONE',  ( 1.107190807272493860, 1477.934341428328935, 198.7592707807304748 ) ) ;
#25171=CARTESIAN_POINT ( 'NONE',  ( -19.09790268268400126, 1508.458003811930212, 210.0050661408479868 ) ) ;
#25172=CARTESIAN_POINT ( 'NONE',  ( 12.72754940664999879, 1426.782577209239889, 204.7399120111390118 ) ) ;
#25173=CARTESIAN_POINT ( 'NONE',  ( -2.775555772024459689, 1468.867611297260055, 187.4507004145660005 ) ) ;
#25175=CARTESIAN_POINT ( 'NONE',  ( -18.35007156173510268, 1419.478779913980134, 206.0032569124829820 ) ) ;
#25176=( BOUNDED_CURVE ( )  B_SPLINE_CURVE ( 3, ( #47091, #30263, #63902, #29718 ),
 .UNSPECIFIED., .F., .F. ) 
 B_SPLINE_CURVE_WITH_KNOTS ( ( 4, 4 ),
 ( 0.9158457003869029389, 2.225909800249735060 ),
 .UNSPECIFIED. ) 
 CURVE ( )  GEOMETRIC_REPRESENTATION_ITEM ( )  RATIONAL_B_SPLINE_CURVE ( ( 1.000000000000000000, 0.8620189361215893076, 0.8620189361215893076, 1.000000000000000000 ) ) 
 REPRESENTATION_ITEM ( '' )  );
#25187=CARTESIAN_POINT ( 'NONE',  ( -10.16565329039999988, 1472.147622277889923, 209.4747181525780206 ) ) ;
#25191=CARTESIAN_POINT ( 'NONE',  ( -7.873917804663410180, 1436.018178901780175, 213.0668616092210073 ) ) ;
#25193=CARTESIAN_POINT ( 'NONE',  ( -15.66177877319999823, 1418.090152389999957, 210.6205366076489724 ) ) ;
#25198=CARTESIAN_POINT ( 'NONE',  ( 12.22179537434220009, 1427.254335307449992, 207.6012072736810126 ) ) ;
#25199=EDGE_LOOP ( 'NONE', ( #53404, #1526, #83088, #54067 ) ) ;
#25204=CARTESIAN_POINT ( 'NONE',  ( 1.498516750899999916, 1473.533416210889982, 219.2408104862990115 ) ) ;
#25205=CARTESIAN_POINT ( 'NONE',  ( 18.15402009115259929, 1430.058659865889922, 210.6865277441139881 ) ) ;
#25212=CARTESIAN_POINT ( 'NONE',  ( 9.014216207049999596, 1449.483768445589931, 207.1212598930990225 ) ) ;
#25216=CARTESIAN_POINT ( 'NONE',  ( -1.042889439659999917, 1455.537194040490022, 199.0056471502989837 ) ) ;
#25220=CARTESIAN_POINT ( 'NONE',  ( -2.443439238509999889, 1496.401426496290014, 197.7599957902989729 ) ) ;
#25236=CARTESIAN_POINT ( 'NONE',  ( 12.69299105715940001, 1500.682136716359992, 209.6945769240809909 ) ) ;
#25238=CARTESIAN_POINT ( 'NONE',  ( 4.626410093743990259, 1508.551704408389924, 212.9021791863180226 ) ) ;
#25242=CARTESIAN_POINT ( 'NONE',  ( 10.10890582563189888, 1461.386743975740046, 208.4428558525590063 ) ) ;
#25244=ORIENTED_EDGE ( 'NONE', *, *, #51843, .T. ) ;
#25247=CARTESIAN_POINT ( 'NONE',  ( 10.51591518309250084, 1452.897324824680254, 210.4058924105359836 ) ) ;
#25250=CARTESIAN_POINT ( 'NONE',  ( -10.95001104760099331, 1417.929106870156829, 198.2904426808065352 ) ) ;
#25251=CARTESIAN_POINT ( 'NONE',  ( 4.226426730560000067, 1515.477082009289916, 209.1218459616539747 ) ) ;
#25252=CARTESIAN_POINT ( 'NONE',  ( -4.726277182027989632, 1455.252851925170035, 200.9609556798399979 ) ) ;
#25253=CARTESIAN_POINT ( 'NONE',  ( 12.65750243759436877, 1420.218673000053741, 200.3470716195499790 ) ) ;
#25270=CARTESIAN_POINT ( 'NONE',  ( -11.01150942929239918, 1462.569953727359916, 208.1811703706719925 ) ) ;
#25272=CARTESIAN_POINT ( 'NONE',  ( 10.09433608495039891, 1469.369659831060062, 207.3742786837029826 ) ) ;
#25273=CARTESIAN_POINT ( 'NONE',  ( -10.93162295028230169, 1470.132889486390013, 212.2376398131100075 ) ) ;
#25286=CARTESIAN_POINT ( 'NONE',  ( -14.77610201870000139, 1416.023439710309958, 213.5223809413389802 ) ) ;
#25292=CARTESIAN_POINT ( 'NONE',  ( -11.03695077974730054, 1462.414655202809854, 208.8602946956429776 ) ) ;
#25294=CARTESIAN_POINT ( 'NONE',  ( -5.266928095709999980, 1427.575715857079786, 201.4004753664689815 ) ) ;
#25297=CARTESIAN_POINT ( 'NONE',  ( -11.36422223541920040, 1482.111961209009905, 207.7636347213490069 ) ) ;
#25303=B_SPLINE_CURVE_WITH_KNOTS ( 'NONE', 3,
 ( #40119, #7075, #30625, #58592, #100019, #99461, #39580, #101111, #90521, #73752, #64812, #22191, #14355, #48547, #22739, #58044 ),
 .UNSPECIFIED., .F., .F.,
 ( 4, 3, 3, 3, 3, 4 ),
 ( -7.456423346589999390, -6.951387445693330669, -5.975502946654870584, -5.002829108848499295, -4.031542647132239310, -3.062118867579999737 ),
 .UNSPECIFIED. ) ;
#25309=CARTESIAN_POINT ( 'NONE',  ( 4.687651746879999415, 1478.378160227390254, 228.9010599218989910 ) ) ;
#25311=CARTESIAN_POINT ( 'NONE',  ( -15.18421651749999945, 1416.713354283420131, 205.6620439543090129 ) ) ;
#25313=EDGE_CURVE ( 'NONE', #60042, #45216, #74188, .T. ) ;
#25316=CARTESIAN_POINT ( 'NONE',  ( -8.588755447433969792, 1437.818850531529961, 207.9413692731380081 ) ) ;
#25317=CARTESIAN_POINT ( 'NONE',  ( -4.712600100240000423, 1496.928403841490081, 219.5050635169990016 ) ) ;
#25319=CARTESIAN_POINT ( 'NONE',  ( -1.758949987490000089, 1470.986537992489957, 189.1593042989989897 ) ) ;
#25322=DIRECTION ( 'NONE',  ( -1.224646799147353947E-16, 1.836970198721029688E-16, 1.000000000000000000 ) ) ;
#25332=CARTESIAN_POINT ( 'NONE',  ( 7.034613962576056423, 1471.361440081786668, 216.4463950981275673 ) ) ;
#25333=CARTESIAN_POINT ( 'NONE',  ( 11.39903768489999969, 1471.112746669390162, 209.6182361446229834 ) ) ;
#25335=EDGE_CURVE ( 'NONE', #1907, #40693, #59623, .T. ) ;
#25338=CARTESIAN_POINT ( 'NONE',  ( 4.167208771420000346, 1485.303719113790066, 219.1667848572990067 ) ) ;
#25340=CARTESIAN_POINT ( 'NONE',  ( -15.24384917251130034, 1447.147816755560143, 196.6853903820460232 ) ) ;
#25341=CARTESIAN_POINT ( 'NONE',  ( -19.10748961539120216, 1444.545920780599999, 199.6793401393300087 ) ) ;
#25348=CARTESIAN_POINT ( 'NONE',  ( 9.798333899899640542, 1435.847786354059963, 209.9101837937189998 ) ) ;
#25350=EDGE_CURVE ( 'NONE', #106884, #7587, #95446, .T. ) ;
#25351=CARTESIAN_POINT ( 'NONE',  ( 6.385148413900250119, 1448.088845170490004, 201.0945304462800038 ) ) ;
#25361=ORIENTED_EDGE ( 'NONE', *, *, #17925, .T. ) ;
#25368=CARTESIAN_POINT ( 'NONE',  ( 4.329448802513499395, 1515.064791340959800, 206.7919475944040073 ) ) ;
#25374=CARTESIAN_POINT ( 'NONE',  ( 2.356138219550000024, 1466.787411483390088, 219.9406446673989990 ) ) ;
#25383=ORIENTED_EDGE ( 'NONE', *, *, #33530, .T. ) ;
#25410=CARTESIAN_POINT ( 'NONE',  ( -2.897185018188709993, 1428.978219621640164, 200.2122387005069868 ) ) ;
#25418=VERTEX_POINT ( 'NONE', #78646 ) ;
#25430=FACE_OUTER_BOUND ( 'NONE', #21974, .T. ) ;
#25435=CARTESIAN_POINT ( 'NONE',  ( -7.756928808066270165, 1508.430203411700177, 219.4938965895260026 ) ) ;
#25441=CARTESIAN_POINT ( 'NONE',  ( -7.532310163755457033, 1461.903255937187396, 202.9766630830429506 ) ) ;
#25442=CARTESIAN_POINT ( 'NONE',  ( -1.591560612370000127, 1443.444047302290073, 218.6175903739389810 ) ) ;
#25443=CARTESIAN_POINT ( 'NONE',  ( 1.681169524081967515, 1468.860615669657591, 219.0052562536231733 ) ) ;
#25450=CARTESIAN_POINT ( 'NONE',  ( 4.789673499540000101, 1465.867933640490037, 219.0700355186390027 ) ) ;
#25455=CARTESIAN_POINT ( 'NONE',  ( 2.258742332965870236, 1456.424467550069949, 219.5015882959719988 ) ) ;
#25457=CARTESIAN_POINT ( 'NONE',  ( -16.43158760069999857, 1420.644935630790087, 203.2808212549290090 ) ) ;
#25460=CARTESIAN_POINT ( 'NONE',  ( 11.71837906060000023, 1501.675020862189967, 211.1788615571589958 ) ) ;
#25463=CARTESIAN_POINT ( 'NONE',  ( 8.458662811369999091, 1427.983063278090185, 212.5922379039890018 ) ) ;
#25476=ORIENTED_EDGE ( 'NONE', *, *, #35626, .T. ) ;
#25477=CARTESIAN_POINT ( 'NONE',  ( 3.822819546398629864, 1435.023558107709960, 227.1593522666110232 ) ) ;
#25478=CARTESIAN_POINT ( 'NONE',  ( -15.55291268160981666, 1415.973418256078048, 207.8029067794451805 ) ) ;
#25482=CARTESIAN_POINT ( 'NONE',  ( -1.937821456590000047, 1444.357003194489835, 218.0146419597290048 ) ) ;
#25483=EDGE_CURVE ( 'NONE', #87765, #89963, #99647, .T. ) ;
#25487=CARTESIAN_POINT ( 'NONE',  ( 7.153413542260000924, 1423.448481430999891, 213.6996531375289976 ) ) ;
#25491=EDGE_CURVE ( 'NONE', #86033, #61245, #3383, .T. ) ;
#25498=CARTESIAN_POINT ( 'NONE',  ( -21.63861185800000086, 1508.509217846390129, 209.6249585502670243 ) ) ;
#25510=CARTESIAN_POINT ( 'NONE',  ( -4.328426199472169777, 1515.103843506339899, 210.1872473502739922 ) ) ;
#25515=CARTESIAN_POINT ( 'NONE',  ( 5.568562089822329142, 1424.311407511700054, 193.4294382966939736 ) ) ;
#25524=DIRECTION ( 'NONE',  ( 9.341989762165448955E-47, -1.000000000000000000, 1.836970198721029688E-16 ) ) ;
#25542=CARTESIAN_POINT ( 'NONE',  ( -6.049104812149999510, 1450.166793888889970, 209.2893785837540293 ) ) ;
#25545=EDGE_LOOP ( 'NONE', ( #49673, #103234, #13123, #103899 ) ) ;
#25551=ADVANCED_FACE ( 'NONE', ( #15540 ), #9093, .T. ) ;
#25552=CARTESIAN_POINT ( 'NONE',  ( -11.96603475488899981, 1491.247197521090129, 206.3905183836859862 ) ) ;
#25555=CARTESIAN_POINT ( 'NONE',  ( -6.654072516460000308, 1414.646055428690033, 206.6656543076690014 ) ) ;
#25558=CARTESIAN_POINT ( 'NONE',  ( 4.290424513729999667, 1486.223672784390146, 199.2226467242190040 ) ) ;
#25562=DIRECTION ( 'NONE',  ( -1.272749556696019889E-16, 0.000000000000000000, 1.000000000000000000 ) ) ;
#25569=CARTESIAN_POINT ( 'NONE',  ( -17.50570382702689898, 1508.551704408389924, 211.8647386576619738 ) ) ;
#25574=CARTESIAN_POINT ( 'NONE',  ( -11.39518164335769868, 1470.898556086270219, 208.5524656631309881 ) ) ;
#25575=CARTESIAN_POINT ( 'NONE',  ( -6.941072381584187490, 1508.373530314580194, 219.7906263800470583 ) ) ;
#25582=CARTESIAN_POINT ( 'NONE',  ( -6.792894082628190944, 1420.761421989889868, 194.5362997547140083 ) ) ;
#25590=CARTESIAN_POINT ( 'NONE',  ( 2.157536728406360904, 1378.913060387289988, 207.9431782750411912 ) ) ;
#25593=CARTESIAN_POINT ( 'NONE',  ( 4.977085520756839188, 1423.895666356600032, 194.0366106666719759 ) ) ;
#25596=CARTESIAN_POINT ( 'NONE',  ( 2.985527909515199863, 1508.551704408389924, 219.4114903352459862 ) ) ;
#25597=FACE_OUTER_BOUND ( 'NONE', #45406, .T. ) ;
#25602=CARTESIAN_POINT ( 'NONE',  ( 10.56891618719440018, 1452.605324780220144, 209.6008627037060137 ) ) ;
#25610=CARTESIAN_POINT ( 'NONE',  ( -12.74986059157959950, 1462.837634083790135, 224.9935237458099948 ) ) ;
#25615=CARTESIAN_POINT ( 'NONE',  ( 11.73451145560060027, 1479.801820424849893, 210.2140368403210005 ) ) ;
#25621=CARTESIAN_POINT ( 'NONE',  ( -0.7527848377683918901, 1485.932384399170132, 197.2449775714050020 ) ) ;
#25622=CARTESIAN_POINT ( 'NONE',  ( 10.58843039633059924, 1471.621789236399991, 212.0273906003420166 ) ) ;
#25624=CARTESIAN_POINT ( 'NONE',  ( 4.249059288160469627, 1433.039579511759939, 201.5637155983669970 ) ) ;
#25629=CARTESIAN_POINT ( 'NONE',  ( -13.46445246340000068, 1470.514529015489870, 192.0392451277990062 ) ) ;
#25635=CARTESIAN_POINT ( 'NONE',  ( 9.611939569861299049, 1460.529529387680213, 206.0552052590290089 ) ) ;
#25638=CARTESIAN_POINT ( 'NONE',  ( 0.06163407857050130084, 1477.698269665189855, 198.6861886841990099 ) ) ;
#25644=CARTESIAN_POINT ( 'NONE',  ( 3.611741757648789797, 1428.548660076119859, 216.5582848978089885 ) ) ;
#25645=CARTESIAN_POINT ( 'NONE',  ( -7.887122863889999280, 1426.208111655430002, 206.9861596317290093 ) ) ;
#25651=CARTESIAN_POINT ( 'NONE',  ( 7.532152985507379661, 1425.792267630160040, 212.2199176514089913 ) ) ;
#25655=CARTESIAN_POINT ( 'NONE',  ( -11.34466715848219920, 1491.663308851389957, 206.9207944444179930 ) ) ;
#25658=CARTESIAN_POINT ( 'NONE',  ( -3.269259737218870310, 1476.740802116999930, 199.2818558394819775 ) ) ;
#25659=CARTESIAN_POINT ( 'NONE',  ( 2.738491027449999837, 1419.583501809659765, 204.7124689335390144 ) ) ;
#25662=ORIENTED_EDGE ( 'NONE', *, *, #54341, .F. ) ;
#25682=CARTESIAN_POINT ( 'NONE',  ( -1.430539248151910137, 1444.328264662749916, 199.1703804428329931 ) ) ;
#25684=EDGE_LOOP ( 'NONE', ( #34785, #54051, #19187, #74443, #103440, #21951, #47235, #101996, #14452, #91089, #94861, #61313, #103988, #10077 ) ) ;
#25687=CARTESIAN_POINT ( 'NONE',  ( 2.487935123032368967, 1508.783371655767951, 204.5758637342562452 ) ) ;
#25689=CARTESIAN_POINT ( 'NONE',  ( 7.377575598780000021, 1422.796019154259966, 195.5835889348989838 ) ) ;
#25703=CARTESIAN_POINT ( 'NONE',  ( 8.576574437940319484, 1426.670950778500128, 211.0879220285609961 ) ) ;
#25705=CARTESIAN_POINT ( 'NONE',  ( -10.99440994877370059, 1462.600064137660183, 208.0385998618030214 ) ) ;
#25706=ADVANCED_FACE ( 'NONE', ( #56353 ), #15268, .T. ) ;
#25713=CARTESIAN_POINT ( 'NONE',  ( 18.36305868314869727, 1428.555240223059855, 201.4018503782459959 ) ) ;
#25714=CARTESIAN_POINT ( 'NONE',  ( 12.37883759903940017, 1420.474967537750217, 199.7601132055380049 ) ) ;
#25716=CARTESIAN_POINT ( 'NONE',  ( 5.938839624758309732, 1465.760319836029794, 217.5705628005549954 ) ) ;
#25722=ADVANCED_FACE ( 'NONE', ( #41741 ), #33181, .T. ) ;
#25725=CARTESIAN_POINT ( 'NONE',  ( 10.34950188612880062, 1451.639534178259964, 207.2650128704659949 ) ) ;
#25727=CARTESIAN_POINT ( 'NONE',  ( -12.04602614745110145, 1481.198043355260097, 227.9689297718389867 ) ) ;
#25729=CARTESIAN_POINT ( 'NONE',  ( -20.71620237759999839, 1418.282126647740142, 210.1201477243000113 ) ) ;
#25740=CARTESIAN_POINT ( 'NONE',  ( -10.17543907640000000, 1472.210474395689971, 209.2297550078889969 ) ) ;
#25744=CARTESIAN_POINT ( 'NONE',  ( -4.150844423549710172, 1433.756621307029945, 217.8254834218780047 ) ) ;
#25749=B_SPLINE_SURFACE_WITH_KNOTS ( 'NONE', 5, 5, ( 
 ( #104853, #102612, #61238, #18071, #25912, #52266 ),
 ( #9140, #10802, #94227, #9678, #1869, #69627 ),
 ( #76904, #43303, #18612, #36543, #8572, #44972 ),
 ( #43847, #77994, #753, #103750, #61776, #1299 ),
 ( #27052, #95352, #60110, #17502, #52812, #93664 ),
 ( #44411, #78551, #51146, #36002, #70195, #27591 ),
 ( #95900, #85272, #79120, #21908, #56104, #12976 ),
 ( #47159, #54482, #3522, #71295, #46073, #88072 ),
 ( #63979, #81286, #72373, #4601, #55571, #11359 ) ),
 .UNSPECIFIED., .F., .F., .F.,
 ( 6, 3, 6 ),
 ( 6, 6 ),
 ( -3.623787203323129550E-05, 8.942376592629999621, 17.88478942317200193 ),
 ( -3.623787203323129550E-05, 2.000000000000000000 ),
 .UNSPECIFIED. ) ;
#25754=CARTESIAN_POINT ( 'NONE',  ( 10.05758522378950026, 1423.330231444269884, 209.0100830007820321 ) ) ;
#25760=CARTESIAN_POINT ( 'NONE',  ( 1.959285271270000184, 1474.800623574289830, 220.3715841371990223 ) ) ;
#25762=CARTESIAN_POINT ( 'NONE',  ( -18.17365796220000007, 1441.208305948289762, 213.5442559039389891 ) ) ;
#25764=CARTESIAN_POINT ( 'NONE',  ( -7.208571784880000166, 1494.204594205489911, 199.0650244531990154 ) ) ;
#25768=CARTESIAN_POINT ( 'NONE',  ( 9108.204429824800172, -2340.220200558880151, 1988.052214260419987 ) ) ;
#25769=CARTESIAN_POINT ( 'NONE',  ( 7.253065918429999925, 1447.817965204990060, 203.4084464636989935 ) ) ;
#25778=CARTESIAN_POINT ( 'NONE',  ( 1.702416242259999768, 1493.957958499289816, 220.1113518661990156 ) ) ;
#25792=CARTESIAN_POINT ( 'NONE',  ( 3.742606737671509975, 1508.551704408389924, 213.7724622950010200 ) ) ;
#25796=CARTESIAN_POINT ( 'NONE',  ( -19.29973955919999895, 1464.638518991389901, 213.2496029295089954 ) ) ;
#25801=CARTESIAN_POINT ( 'NONE',  ( 5.277460848200000498, 1426.742654866309977, 191.8370381630989812 ) ) ;
#25804=CARTESIAN_POINT ( 'NONE',  ( -14.16755010633700174, 1508.249070031330120, 209.5474642701840082 ) ) ;
#25805=CARTESIAN_POINT ( 'NONE',  ( 4.282704111100000155, 1515.349907855090123, 210.2219876055189900 ) ) ;
#25809=CARTESIAN_POINT ( 'NONE',  ( 10.57600172136130112, 1452.469479793819801, 209.2385615662339831 ) ) ;
#25822=CARTESIAN_POINT ( 'NONE',  ( -3.847490228401430734, 1488.832123754849817, 219.3169755907300384 ) ) ;
#25825=CARTESIAN_POINT ( 'NONE',  ( -9.700924147820000343, 1472.526415508389846, 203.7850276454490199 ) ) ;
#25829=CARTESIAN_POINT ( 'NONE',  ( -21.66822351760000132, 1505.633081141090088, 209.3276579973889966 ) ) ;
#25830=CARTESIAN_POINT ( 'NONE',  ( 3.485764247198380072, 1466.371155763999923, 198.6273673771169967 ) ) ;
#25832=B_SPLINE_CURVE_WITH_KNOTS ( 'NONE', 3,
 ( #5903, #66385, #32203, #108360, #82039, #47904, #12646, #47355, #90441, #4254, #55781, #49024, #99386, #22109, #65273, #98296, #100504, #83160, #6453, #72565, #107805, #81483, #31642 ),
 .UNSPECIFIED., .F., .F.,
 ( 4, 2, 1, 1, 1, 2, 2, 2, 2, 1, 1, 2, 2, 4 ),
 ( 0.000000000000000000, 0.1249999999997535305, 0.1874999999996302402, 0.2187499999995681232, 0.2343749999995374256, 0.2421874999995221045, 0.2499999999995067834, 0.4999999999996687094, 0.6249999999997648548, 0.6874999999998291367, 0.7187499999998765432, 0.7343749999998833156, 0.7499999999998901989, 1.000000000000000000 ),
 .UNSPECIFIED. ) ;
#25840=CARTESIAN_POINT ( 'NONE',  ( -0.5721718501029199322, 1515.139735159960082, 204.7943596184780120 ) ) ;
#25846=CARTESIAN_POINT ( 'NONE',  ( -10.88434851486570132, 1461.922897766000006, 210.7637379796009895 ) ) ;
#25848=CARTESIAN_POINT ( 'NONE',  ( -7.467969047550820250, 1425.935834671629891, 203.5501275869820290 ) ) ;
#25851=B_SPLINE_CURVE_WITH_KNOTS ( 'NONE', 5,
 ( #56474, #57037, #13330, #12800, #30703, #89509, #21725, #6058, #82203, #29596, #46980, #5509 ),
 .UNSPECIFIED., .F., .F.,
 ( 6, 3, 3, 6 ),
 ( -7.661770164330000021, -7.525802029310000307, -3.316542704129999741, -3.139241426659999945 ),
 .UNSPECIFIED. ) ;
#25853=CARTESIAN_POINT ( 'NONE',  ( -10.62969216458879984, 1481.435998155740208, 207.6925002982229955 ) ) ;
#25858=CARTESIAN_POINT ( 'NONE',  ( 1.497499201727195306, 1455.575695172564792, 218.4485741766675346 ) ) ;
#25865=CARTESIAN_POINT ( 'NONE',  ( -16.73160448879999862, 1417.112108414879913, 207.5092061429490116 ) ) ;
#25869=CARTESIAN_POINT ( 'NONE',  ( -17.00277584490474680, 1419.505931447407647, 208.3295775563994710 ) ) ;
#25870=CARTESIAN_POINT ( 'NONE',  ( -5.405424721240001062, 1496.292287258489750, 218.9823198700590012 ) ) ;
#25872=B_SPLINE_CURVE_WITH_KNOTS ( 'NONE', 5,
 ( #76913, #18081, #221, #41648, #86401, #109956 ),
 .UNSPECIFIED., .F., .F.,
 ( 6, 6 ),
 ( 0.000000000000000000, 1.000000000000000000 ),
 .UNSPECIFIED. ) ;
#25875=B_SPLINE_SURFACE_WITH_KNOTS ( 'NONE', 5, 1, ( 
 ( #85219, #15253 ),
 ( #9079, #50544 ),
 ( #58392, #43246 ),
 ( #8511, #24743 ),
 ( #23667, #93610 ),
 ( #49444, #83568 ) ),
 .UNSPECIFIED., .F., .F., .F.,
 ( 6, 6 ),
 ( 2, 2 ),
 ( 0.000000000000000000, 16.34325491069999714 ),
 ( 0.000000000000000000, 14.00000000000000000 ),
 .UNSPECIFIED. ) ;
#25877=CARTESIAN_POINT ( 'NONE',  ( -11.64956323076249944, 1508.434911808069955, 208.7884202097649791 ) ) ;
#25878=CARTESIAN_POINT ( 'NONE',  ( -15.62861149524349891, 1418.244676918490086, 203.0179538217920197 ) ) ;
#25880=CARTESIAN_POINT ( 'NONE',  ( -5.598467674920000192, 1448.782436168089816, 211.2741064300589926 ) ) ;
#25893=CARTESIAN_POINT ( 'NONE',  ( 4.868883885119999810, 1484.326762180689911, 219.4762353022989885 ) ) ;
#25897=CARTESIAN_POINT ( 'NONE',  ( 4.862561345523300105, 1435.671581979260054, 228.7561080407950271 ) ) ;
#25899=CARTESIAN_POINT ( 'NONE',  ( -11.77904575181089974, 1483.168265960099916, 228.2502168366870023 ) ) ;
#25904=CARTESIAN_POINT ( 'NONE',  ( -10.70370633090000112, 1490.481523645589959, 212.1270248953690043 ) ) ;
#25905=CARTESIAN_POINT ( 'NONE',  ( 9.283513090479321050, 1450.226982269150085, 204.4123054901219803 ) ) ;
#25911=CARTESIAN_POINT ( 'NONE',  ( 1.847634001515719993, 1478.089546411300262, 198.8590795898780073 ) ) ;
#25912=CARTESIAN_POINT ( 'NONE',  ( 5.517763559299710074, 1505.096907884720167, 220.1774585940589759 ) ) ;
#25915=VERTEX_POINT ( 'NONE', #74132 ) ;
#25916=VERTEX_POINT ( 'NONE', #100947 ) ;
#25928=CARTESIAN_POINT ( 'NONE',  ( 3.266173989019999890, 1467.802313959489993, 218.5517745389790036 ) ) ;
#25939=ORIENTED_EDGE ( 'NONE', *, *, #95346, .F. ) ;
#25942=CARTESIAN_POINT ( 'NONE',  ( -11.46285746319973953, 1503.757028837903590, 207.6153346572946532 ) ) ;
#25943=DIRECTION ( 'NONE',  ( 1.000000000000000000, -3.196303315166338322E-31, 4.657260248767550292E-10 ) ) ;
#25951=ORIENTED_EDGE ( 'NONE', *, *, #73390, .T. ) ;
#25960=CARTESIAN_POINT ( 'NONE',  ( -15.28723455579760149, 1508.551704408389924, 210.3672327514449876 ) ) ;
#25961=CARTESIAN_POINT ( 'NONE',  ( -5.062212390315069754, 1474.342205398819942, 198.8731691453010058 ) ) ;
#25970=CARTESIAN_POINT ( 'NONE',  ( -11.86894174216629949, 1482.050028868399977, 208.4783409248709916 ) ) ;
#25980=CARTESIAN_POINT ( 'NONE',  ( 12.45033887509999992, 1421.619541826690238, 207.5029467985389999 ) ) ;
#25983=CARTESIAN_POINT ( 'NONE',  ( -9.172189383897210391, 1449.366367657520186, 209.4775503665190115 ) ) ;
#25992=CARTESIAN_POINT ( 'NONE',  ( 3.461590032740000211, 1467.254004089789987, 218.5936129320489840 ) ) ;
#25993=CARTESIAN_POINT ( 'NONE',  ( -1.221263722386547901, 1469.682530730686949, 219.1105054375227894 ) ) ;
#25997=CARTESIAN_POINT ( 'NONE',  ( -1.749097280350000005, 1429.787493520590033, 200.2727799645290077 ) ) ;
#26002=CARTESIAN_POINT ( 'NONE',  ( -9.103468112560660686, 1449.499701819690017, 210.3008494512589834 ) ) ;
#26009=CARTESIAN_POINT ( 'NONE',  ( 12.24365544940000028, 1500.600793972790143, 208.6479367508759992 ) ) ;
#26010=CARTESIAN_POINT ( 'NONE',  ( -14.61611649526098589, 1469.120177286887611, 195.1467201088773606 ) ) ;
#26013=CARTESIAN_POINT ( 'NONE',  ( 8.239069889199999608, 1423.385677187009833, 212.2461209534189948 ) ) ;
#26017=CARTESIAN_POINT ( 'NONE',  ( -6.588204561759999578, 1484.019114425890166, 200.1196401685189983 ) ) ;
#26020=ORIENTED_EDGE ( 'NONE', *, *, #88002, .T. ) ;
#26021=B_SPLINE_CURVE_WITH_KNOTS ( 'NONE', 5,
 ( #90015, #55342, #22238, #107373, #20057, #54251 ),
 .UNSPECIFIED., .F., .F.,
 ( 6, 6 ),
 ( 0.000000000000000000, 1.000000000000000000 ),
 .UNSPECIFIED. ) ;
#26024=VERTEX_POINT ( 'NONE', #32110 ) ;
#26029=CARTESIAN_POINT ( 'NONE',  ( -9.927759914837499977, 1438.851595397029996, 209.8644134391970226 ) ) ;
#26034=CARTESIAN_POINT ( 'NONE',  ( 6.908704138140000062, 1424.414520317140159, 213.3241070330990112 ) ) ;
#26036=CARTESIAN_POINT ( 'NONE',  ( -17.51440555739999994, 1442.103933559090137, 219.2287671671990097 ) ) ;
#26042=ORIENTED_EDGE ( 'NONE', *, *, #48835, .F. ) ;
#26050=CARTESIAN_POINT ( 'NONE',  ( 1.355095489612469839, 1476.075987768590039, 197.7236685275530021 ) ) ;
#26058=ORIENTED_EDGE ( 'NONE', *, *, #53028, .F. ) ;
#26064=CARTESIAN_POINT ( 'NONE',  ( 5.703720466386680066, 1424.346729877480129, 193.4758770404599773 ) ) ;
#26067=VERTEX_POINT ( 'NONE', #96437 ) ;
#26095=CARTESIAN_POINT ( 'NONE',  ( -11.71533056565333553, 1414.421228241719973, 208.3857400952160788 ) ) ;
#26097=VERTEX_POINT ( 'NONE', #70720 ) ;
#26098=FACE_BOUND ( 'NONE', #33963, .T. ) ;
#26100=EDGE_CURVE ( 'NONE', #108726, #31217, #79753, .T. ) ;
#26104=CARTESIAN_POINT ( 'NONE',  ( -9.415828895194328751, 1493.189318859109790, 201.2122058663049700 ) ) ;
#26114=CARTESIAN_POINT ( 'NONE',  ( 6.824596708572589598, 1424.815923006090998, 213.4892281219103154 ) ) ;
#26119=CARTESIAN_POINT ( 'NONE',  ( -17.12870856829999866, 1420.279571949720093, 203.5620527584690080 ) ) ;
#26121=ADVANCED_FACE ( 'NONE', ( #79099 ), #75214, .T. ) ;
#26124=FACE_OUTER_BOUND ( 'NONE', #58480, .T. ) ;
#26126=CARTESIAN_POINT ( 'NONE',  ( 2.901843670269999897, 1442.289985319589960, 217.6299988927789855 ) ) ;
#26128=CARTESIAN_POINT ( 'NONE',  ( -762.4595027414246715, -8387.357407334298841, -1619.876006850564636 ) ) ;
#26130=CARTESIAN_POINT ( 'NONE',  ( 11.21247613359999917, 1490.926120241489798, 206.9376360906590264 ) ) ;
#26134=CARTESIAN_POINT ( 'NONE',  ( -14.06060368556070017, 1417.615943288039944, 202.3868150088759990 ) ) ;
#26135=CARTESIAN_POINT ( 'NONE',  ( -5.034319209093887082, 1391.795857067797897, 203.5666908100943715 ) ) ;
#26139=CARTESIAN_POINT ( 'NONE',  ( -4.678144232538111069, 1508.611354625609920, 211.6097690136730023 ) ) ;
#26142=CARTESIAN_POINT ( 'NONE',  ( -10.41319835519830050, 1479.501835575390032, 210.3840731168270111 ) ) ;
#26146=CARTESIAN_POINT ( 'NONE',  ( -4.634289585198445138, 1377.926009802909448, 204.1816958463118112 ) ) ;
#26149=CARTESIAN_POINT ( 'NONE',  ( 11.69992624430000028, 1435.514532378290141, 225.6365414701989778 ) ) ;
#26155=( BOUNDED_SURFACE ( )  B_SPLINE_SURFACE ( 1, 2, ( 
 ( #87888, #18981, #88960, #71102, #2243, #105226, #28513, #61583, #10616 ),
 ( #79480, #10050, #1674, #27961, #38019, #78934, #11179, #45340, #44223 ) ),
 .UNSPECIFIED., .F., .T., .T. ) 
 B_SPLINE_SURFACE_WITH_KNOTS ( ( 2, 2 ),
 ( 3, 2, 2, 2, 3 ),
 ( -10000.00000000000000, 10000.00000000000000 ),
 ( 0.000000000000000000, 1.570796326794899889, 3.141592653589790007, 4.712388980384689674, 6.283185307179590673 ),
 .UNSPECIFIED. ) 
 GEOMETRIC_REPRESENTATION_ITEM ( )  RATIONAL_B_SPLINE_SURFACE ( (
 ( 1.000000000000000000, 0.7071067811865480168, 1.000000000000000000, 0.7071067811865480168, 1.000000000000000000, 0.7071067811865480168, 1.000000000000000000, 0.7071067811865480168, 1.000000000000000000),
 ( 1.000000000000000000, 0.7071067811865480168, 1.000000000000000000, 0.7071067811865480168, 1.000000000000000000, 0.7071067811865480168, 1.000000000000000000, 0.7071067811865480168, 1.000000000000000000) ) ) 
 REPRESENTATION_ITEM ( '' )  SURFACE ( )  );
#26161=CARTESIAN_POINT ( 'NONE',  ( 8.473460899918398681, 1436.816749859699939, 207.5081568175040161 ) ) ;
#26168=CARTESIAN_POINT ( 'NONE',  ( 4.351134154479999516, 1486.174099317390073, 218.9925762311689823 ) ) ;
#26171=EDGE_CURVE ( 'NONE', #107938, #234, #99523, .T. ) ;
#26175=CARTESIAN_POINT ( 'NONE',  ( 1.980108968457849894, 1486.664140084620158, 197.3565552069889861 ) ) ;
#26177=CARTESIAN_POINT ( 'NONE',  ( 8.601478387608290532, 1434.291646609100098, 205.4210292933150015 ) ) ;
#26178=CARTESIAN_POINT ( 'NONE',  ( -16.38663586692679885, 1420.666626819609974, 203.2878343952710054 ) ) ;
#26182=CARTESIAN_POINT ( 'NONE',  ( -2.775540907220860110, 1468.867511704140043, 187.4507030301369923 ) ) ;
#26185=CARTESIAN_POINT ( 'NONE',  ( -9.526128307108560733, 1440.436522615020067, 205.9995050262249947 ) ) ;
#26186=CARTESIAN_POINT ( 'NONE',  ( -10.69712516999999963, 1469.751244810890057, 192.0684298487989849 ) ) ;
#26187=B_SPLINE_CURVE_WITH_KNOTS ( 'NONE', 3,
 ( #11287, #45454, #79596, #2900, #37018, #20209, #101300, #15638, #83420, #67750, #92926, #66110, #49292, #49844, #16198, #57706, #15101, #110278, #6716, #7274, #91278, #91822, #109734, #31365, #100234, #101860, #14558, #41986, #57153, #48748, #6165, #33554, #108070, #108630, #24048, #25154, #32484, #24594, #5628, #82329, #82872, #58243, #67200, #41438, #40872, #90720, #22948, #39780, #40319, #73939, #75048, #14004, #74501, #48191, #66656, #109200, #84528, #50400, #31917, #65548, #100758, #92365, #7816, #83974, #99657, #75604, #23513, #33014, #76135, #58787, #69973, #34677, #86185 ),
 .UNSPECIFIED., .F., .F.,
 ( 4, 3, 3, 3, 3, 3, 3, 3, 3, 3, 3, 3, 3, 3, 3, 3, 3, 3, 3, 3, 3, 3, 3, 3, 4 ),
 ( -3.000000000000000000, -2.908102647996280155, -2.782376461063030160, -2.655195141559369976, -2.527218228074600059, -2.398166538595950303, -2.268699843587460130, -2.139077724919949741, -2.009568716481330064, -1.880785536864220120, -1.752803873385159861, -1.625825473067359805, -1.500001823732700190, -1.408018940171470001, -1.282042450005529854, -1.154645469624880239, -1.026484574474419986, -0.8973212114648321247, -0.7677990144031130448, -0.6381809425520890144, -0.5087351739316061661, -0.3801018622984368989, -0.2523159959961591703, -0.1255687713132269678, -1.339495774743681977E-06 ),
 .UNSPECIFIED. ) ;
#26193=CARTESIAN_POINT ( 'NONE',  ( -2.703378773469999885, 1475.094742016189912, 198.0005565889990180 ) ) ;
#26201=ORIENTED_EDGE ( 'NONE', *, *, #94114, .F. ) ;
#26204=CARTESIAN_POINT ( 'NONE',  ( -5.064170362302888861, 1470.551699771569702, 217.9081933660337143 ) ) ;
#26205=CARTESIAN_POINT ( 'NONE',  ( 7.523283297491509813, 1425.862182174410009, 212.2493654379539976 ) ) ;
#26213=CARTESIAN_POINT ( 'NONE',  ( 2.197066704608598098, 1487.041132010079082, 219.7150323356243575 ) ) ;
#26215=ADVANCED_FACE ( 'NONE', ( #9810 ), #60071, .F. ) ;
#26218=ORIENTED_EDGE ( 'NONE', *, *, #42400, .T. ) ;
#26243=ORIENTED_EDGE ( 'NONE', *, *, #51535, .T. ) ;
#26244=CARTESIAN_POINT ( 'NONE',  ( 3.945788320329008503, 1515.565606824783117, 207.8723252021519272 ) ) ;
#26247=CARTESIAN_POINT ( 'NONE',  ( -4.771130221740180311, 1508.551704408389924, 212.6291175505820092 ) ) ;
#26263=CARTESIAN_POINT ( 'NONE',  ( -17.43675326300159867, 1417.688629928019964, 206.2161178420579972 ) ) ;
#26266=CARTESIAN_POINT ( 'NONE',  ( -0.1950033126530047733, 1421.009551141655493, 193.7183299770628651 ) ) ;
#26267=CARTESIAN_POINT ( 'NONE',  ( -4.327305182179610021, 1515.146653429449998, 208.6708865915660169 ) ) ;
#26274=CARTESIAN_POINT ( 'NONE',  ( -9.807154110200000829, 1424.402417317040090, 192.4107027041989966 ) ) ;
#26275=CARTESIAN_POINT ( 'NONE',  ( -1.842962231260000028, 1515.064792882589927, 213.4512947377390049 ) ) ;
#26281=CARTESIAN_POINT ( 'NONE',  ( -8.111163737316729794, 1425.152143030509933, 209.4308767762499599 ) ) ;
#26285=CARTESIAN_POINT ( 'NONE',  ( -1.105873109679999855, 1515.456834174690130, 204.9203193849689910 ) ) ;
#26287=CARTESIAN_POINT ( 'NONE',  ( 13.52268454819029841, 1497.923627212899873, 227.8730059201319875 ) ) ;
#26289=CARTESIAN_POINT ( 'NONE',  ( -17.81440792103600046, 1419.712128143199834, 206.0771405611880027 ) ) ;
#26291=CARTESIAN_POINT ( 'NONE',  ( 18.22756002379999529, 1431.409129072690121, 207.4347713430790066 ) ) ;
#26297=CARTESIAN_POINT ( 'NONE',  ( 11.69994445601069977, 1435.514615917619949, 225.6365337787890155 ) ) ;
#26301=CARTESIAN_POINT ( 'NONE',  ( 6.725176165684159102, 1446.961637082904645, 203.0350805069372484 ) ) ;
#26302=LINE ( 'NONE', #94613, #60669 ) ;
#26303=CARTESIAN_POINT ( 'NONE',  ( -8.459774974535099190, 1436.681737689380043, 211.0369107578229944 ) ) ;
#26310=CARTESIAN_POINT ( 'NONE',  ( 10.30462054015580087, 1426.851742110210125, 209.1703782512580005 ) ) ;
#26315=CARTESIAN_POINT ( 'NONE',  ( 6.786745158321280336, 1466.611179241469927, 216.3706489178590004 ) ) ;
#26316=ORIENTED_EDGE ( 'NONE', *, *, #69366, .T. ) ;
#26319=CARTESIAN_POINT ( 'NONE',  ( -10.48582348350000082, 1492.891079834690117, 204.9070088834189960 ) ) ;
#26320=EDGE_CURVE ( 'NONE', #77955, #75598, #101130, .T. ) ;
#26324=DIRECTION ( 'NONE',  ( 0.000000000000000000, 1.000000000000000000, -1.836970198721029688E-16 ) ) ;
#26334=CARTESIAN_POINT ( 'NONE',  ( -3.607508154840000092, 1496.493922223389973, 219.8931764588990063 ) ) ;
#26340=B_SPLINE_CURVE_WITH_KNOTS ( 'NONE', 3,
 ( #94257, #69099, #110520, #93693, #16429, #16973, #67996, #9171, #35469, #34914, #51734, #94825, #8051, #102642, #27083, #50621, #101542, #17532, #24831, #59036 ),
 .UNSPECIFIED., .F., .F.,
 ( 4, 2, 2, 2, 1, 1, 1, 1, 2, 2, 2, 4 ),
 ( 0.000000000000000000, 0.2499999999984017229, 0.3749999999975950904, 0.4374999999971947440, 0.4687499999969976794, 0.4843749999969083619, 0.4921874999968666176, 0.4960937499968487430, 0.4980468749968492426, 0.4999999999968497422, 0.7499999999984249266, 1.000000000000000000 ),
 .UNSPECIFIED. ) ;
#26349=ADVANCED_FACE ( 'NONE', ( #33220 ), #74699, .T. ) ;
#26351=CARTESIAN_POINT ( 'NONE',  ( -4.994803988990000221, 1391.714632731289839, 214.5952593868790075 ) ) ;
#26355=CARTESIAN_POINT ( 'NONE',  ( 9.633682766397971164, 1462.526647204680103, 207.6052849751269775 ) ) ;
#26364=VERTEX_POINT ( 'NONE', #34879 ) ;
#26366=CARTESIAN_POINT ( 'NONE',  ( -13.59512379659999937, 1507.703333832490216, 209.3532891243080201 ) ) ;
#26368=EDGE_CURVE ( 'NONE', #53580, #23969, #36659, .T. ) ;
#26371=CARTESIAN_POINT ( 'NONE',  ( 10.56996490077299811, 1452.372263598349946, 208.9876866165449769 ) ) ;
#26374=VERTEX_POINT ( 'NONE', #69623 ) ;
#26377=ORIENTED_EDGE ( 'NONE', *, *, #73348, .T. ) ;
#26382=CARTESIAN_POINT ( 'NONE',  ( -6.427049037362169592, 1508.551704408389924, 219.3403462825500014 ) ) ;
#26384=CARTESIAN_POINT ( 'NONE',  ( -1.636404844837480166, 1469.777808224259843, 219.0527859593750009 ) ) ;
#26387=CARTESIAN_POINT ( 'NONE',  ( 3.116134665881934662, 1509.034509761476329, 204.6344887231309997 ) ) ;
#26388=CARTESIAN_POINT ( 'NONE',  ( -12.48995958582669985, 1501.883328869510024, 211.6213070116990025 ) ) ;
#26392=CARTESIAN_POINT ( 'NONE',  ( -4.804225480384130442, 1496.882362067949998, 198.9430272844270178 ) ) ;
#26395=B_SPLINE_CURVE_WITH_KNOTS ( 'NONE', 3,
 ( #47221, #96521, #3041, #107114, #72976, #37713, #38253, #47768, #39361, #62396, #28763, #11959, #46145, #80275, #3589, #83553, #75730, #99244, #99799, #40456, #50531, #56723 ),
 .UNSPECIFIED., .F., .F.,
 ( 4, 3, 3, 3, 3, 3, 3, 4 ),
 ( -15.61492507820850051, -14.86289102913099924, -13.52885667192749963, -12.35991797187899977, -11.57914177227580055, -10.59814511392120018, -9.795446212852318979, -9.104900351529998659 ),
 .UNSPECIFIED. ) ;
#26396=CIRCLE ( 'NONE', #46106, 7.146147325060000277 ) ;
#26405=CARTESIAN_POINT ( 'NONE',  ( -14.71755666980000044, 1415.865102022439942, 213.5049452957989899 ) ) ;
#26406=CARTESIAN_POINT ( 'NONE',  ( -0.3081309750529439562, 1515.153045852119931, 204.7947081710710222 ) ) ;
#26408=CARTESIAN_POINT ( 'NONE',  ( -15.46337563405010052, 1415.677402202039957, 209.5778891453549875 ) ) ;
#26414=DIRECTION ( 'NONE',  ( 8.881784197000000007E-16, -1.000000000000000000, 1.836970198721029688E-16 ) ) ;
#26417=CARTESIAN_POINT ( 'NONE',  ( -9.809506047440001097, 1478.918602606890090, 213.0364292658189811 ) ) ;
#26426=CARTESIAN_POINT ( 'NONE',  ( -15.03352721073179943, 1417.917664510099939, 203.1866864770329926 ) ) ;
#26432=CARTESIAN_POINT ( 'NONE',  ( 17.77898125735369916, 1428.911568982719928, 205.3667159481209978 ) ) ;
#26433=CARTESIAN_POINT ( 'NONE',  ( -3.584844276230000126, 1496.864215754190127, 220.1846649233989979 ) ) ;
#26438=CARTESIAN_POINT ( 'NONE',  ( 10.49820941578430045, 1481.974680494319955, 210.5709914680880104 ) ) ;
#26445=B_SPLINE_SURFACE_WITH_KNOTS ( 'NONE', 5, 1, ( 
 ( #52356, #43388 ),
 ( #35523, #104385 ),
 ( #27134, #18703 ),
 ( #841, #34421 ),
 ( #94882, #43933 ),
 ( #8651, #86473 ) ),
 .UNSPECIFIED., .F., .F., .F.,
 ( 6, 6 ),
 ( 2, 2 ),
 ( 0.000000000000000000, 16.10035485789999754 ),
 ( 0.000000000000000000, 14.00000000000000000 ),
 .UNSPECIFIED. ) ;
#26451=CARTESIAN_POINT ( 'NONE',  ( -15.73033044518626333, 1415.742871371153342, 209.5189858198543220 ) ) ;
#26455=CARTESIAN_POINT ( 'NONE',  ( 3.759063234690000144, 1484.612424520689956, 220.3580642450990013 ) ) ;
#26456=CARTESIAN_POINT ( 'NONE',  ( 5.046810547520000689, 1422.880139949140130, 194.5523469769989902 ) ) ;
#26458=CARTESIAN_POINT ( 'NONE',  ( 5.325107150730000072, 1437.628063137190111, 228.7363426427990305 ) ) ;
#26460=CARTESIAN_POINT ( 'NONE',  ( 20.33643750506929848, 1475.138452887649919, 218.0161091833910234 ) ) ;
#26461=CARTESIAN_POINT ( 'NONE',  ( -16.69478953993380088, 1417.256065975089996, 208.2559420391330036 ) ) ;
#26464=DIRECTION ( 'NONE',  ( -0.2778957479319200119, -0.4510399357639849338, 0.8481373294622629455 ) ) ;
#26465=CARTESIAN_POINT ( 'NONE',  ( -11.44853639979999826, 1489.809568400389935, 211.8872501198590044 ) ) ;
#26466=CARTESIAN_POINT ( 'NONE',  ( 3.553091682609760049, 1446.489235633270255, 199.6236789066639972 ) ) ;
#26470=CARTESIAN_POINT ( 'NONE',  ( 4.571596902580940203, 1429.775350729068123, 216.5860468117702169 ) ) ;
#26472=CARTESIAN_POINT ( 'NONE',  ( 17.30273524950730035, 1431.037683288380094, 215.1927343395939829 ) ) ;
#26477=ORIENTED_EDGE ( 'NONE', *, *, #47494, .T. ) ;
#26478=ORIENTED_EDGE ( 'NONE', *, *, #91780, .T. ) ;
#26483=CARTESIAN_POINT ( 'NONE',  ( -10.35394977520730109, 1447.847288705600022, 209.4908303012460067 ) ) ;
#26486=CARTESIAN_POINT ( 'NONE',  ( -1.430539319850000046, 1444.328264637789971, 199.1703804529689990 ) ) ;
#26490=CARTESIAN_POINT ( 'NONE',  ( 2.309279387819999751, 1467.303868143789941, 219.2083978630990089 ) ) ;
#26492=EDGE_CURVE ( 'NONE', #11469, #78070, #82446, .T. ) ;
#26493=FILL_AREA_STYLE_COLOUR ( '', #9015 ) ;
#26496=CARTESIAN_POINT ( 'NONE',  ( -11.39395055920610034, 1422.323217934379954, 208.3944487261120173 ) ) ;
#26500=CARTESIAN_POINT ( 'NONE',  ( -0.5665393661006929982, 1432.061368030950007, 200.7215048253549980 ) ) ;
#26508=CARTESIAN_POINT ( 'NONE',  ( 1.034685474009820139, 1465.654288377450257, 198.1561616953400176 ) ) ;
#26509=CARTESIAN_POINT ( 'NONE',  ( 11.95411458668919913, 1421.865014672959887, 208.9185006178269930 ) ) ;
#26511=CARTESIAN_POINT ( 'NONE',  ( 2.345806028950000233, 1465.851187384389959, 198.7475428451990069 ) ) ;
#26512=EDGE_CURVE ( 'NONE', #63858, #11469, #43825, .T. ) ;
#26514=ORIENTED_EDGE ( 'NONE', *, *, #60175, .F. ) ;
#26516=EDGE_LOOP ( 'NONE', ( #10809, #68060, #4365, #71040 ) ) ;
#26524=CARTESIAN_POINT ( 'NONE',  ( 1.694839287372699843, 1423.343597660659952, 192.5785702911879866 ) ) ;
#26525=VERTEX_POINT ( 'NONE', #6723 ) ;
#26527=CARTESIAN_POINT ( 'NONE',  ( -18.39846574424100112, 1508.551704408389924, 210.4158962701780240 ) ) ;
#26529=CARTESIAN_POINT ( 'NONE',  ( -3.892685920502783059, 1515.551704408390833, 207.5713311529123644 ) ) ;
#26536=CARTESIAN_POINT ( 'NONE',  ( -2.672560874067200221, 1429.102242977169908, 200.1400491528160046 ) ) ;
#26541=CARTESIAN_POINT ( 'NONE',  ( -11.83738977962950045, 1482.193131579070041, 207.9752198576520072 ) ) ;
#26544=AXIS2_PLACEMENT_3D ( 'NONE', #8990, #43161, #34746 ) ;
#26551=LINE ( 'NONE', #1940, #55520 ) ;
#26554=CARTESIAN_POINT ( 'NONE',  ( 12.68801083313210043, 1500.413651417279880, 208.6561539661539939 ) ) ;
#26562=DIRECTION ( 'NONE',  ( 0.4794255386042031719, 0.000000000000000000, 0.8775825618903726477 ) ) ;
#26563=CARTESIAN_POINT ( 'NONE',  ( -19.72258750869999844, 1466.915458833189859, 211.2872857108489768 ) ) ;
#26568=CARTESIAN_POINT ( 'NONE',  ( 11.31762420324339935, 1479.941427780220010, 210.0023256529900095 ) ) ;
#26574=CARTESIAN_POINT ( 'NONE',  ( 3.451256915079999654, 1486.991676997989771, 198.1002658732990085 ) ) ;
#26575=DIRECTION ( 'NONE',  ( 0.000000000000000000, 1.000000000000000000, -1.836970198721029688E-16 ) ) ;
#26577=CARTESIAN_POINT ( 'NONE',  ( 12.70252038000000105, 1500.491347428390100, 208.9664825564809689 ) ) ;
#26580=CARTESIAN_POINT ( 'NONE',  ( 8.405796631650000350, 1426.718801237130037, 211.2874662749189838 ) ) ;
#26588=ORIENTED_EDGE ( 'NONE', *, *, #52749, .T. ) ;
#26593=CARTESIAN_POINT ( 'NONE',  ( 2.654812158838510072, 1435.276104861070053, 227.3789647914429963 ) ) ;
#26596=CARTESIAN_POINT ( 'NONE',  ( -1.042127096165949895, 1457.293139024839775, 219.7093524084000080 ) ) ;
#26597=CARTESIAN_POINT ( 'NONE',  ( -2.494390017649999791, 1456.456026124890059, 202.8045864964890086 ) ) ;
#26601=CARTESIAN_POINT ( 'NONE',  ( 7.465511834920000922, 1425.245174624619949, 212.3173831568290097 ) ) ;
#26602=CARTESIAN_POINT ( 'NONE',  ( -17.66147422859999949, 1440.150478811289986, 218.7822781203190061 ) ) ;
#26607=CARTESIAN_POINT ( 'NONE',  ( 5.215576331900000362, 1455.428525482890109, 217.8852023316690065 ) ) ;
#26614=CARTESIAN_POINT ( 'NONE',  ( 8.356958208356386919, 1500.521215832928192, 201.3523197060887355 ) ) ;
#26616=B_SPLINE_CURVE_WITH_KNOTS ( 'NONE', 3,
 ( #57791, #100846, #24138, #41525, #31453, #101386, #75683, #23042, #24681, #16282, #107621, #44286, #51579, #103052, #635, #61647, #67840, #17940, #25238, #101951, #34212, #78430, #60547, #34764, #35316, #27460, #51025, #9007, #94109, #86823, #95775, #76223, #25792, #1742, #93552, #68397, #42073, #110367, #19042, #17380, #85711, #53244, #85160, #33645, #9554, #7902, #59991, #26923, #8446 ),
 .UNSPECIFIED., .F., .F.,
 ( 4, 3, 3, 3, 3, 3, 3, 3, 3, 3, 3, 3, 3, 3, 3, 3, 4 ),
 ( -12.57638456940000005, -12.28317881101169995, -11.95680856207710008, -11.62570944449999999, -11.51472436910760067, -11.17721019327809984, -10.83638269496280060, -10.49376598039089892, -10.14927727062430129, -9.804494080932538935, -9.458815399652909406, -9.117616601314919578, -8.780289088742080139, -8.445887015311230428, -8.114782774053489689, -7.787209585589999428, -7.548674336869999557 ),
 .UNSPECIFIED. ) ;
#26619=CARTESIAN_POINT ( 'NONE',  ( 2.297639806071400059, 1476.253136155009997, 197.8580381094499785 ) ) ;
#26627=VERTEX_POINT ( 'NONE', #74509 ) ;
#26628=CARTESIAN_POINT ( 'NONE',  ( 4.124127541549999165, 1440.791920158089852, 218.1322488136489994 ) ) ;
#26637=ORIENTED_EDGE ( 'NONE', *, *, #9071, .T. ) ;
#26648=ORIENTED_EDGE ( 'NONE', *, *, #96767, .T. ) ;
#26657=CARTESIAN_POINT ( 'NONE',  ( 13.01048185389249845, 1478.887107457059983, 225.7213801538089797 ) ) ;
#26666=CARTESIAN_POINT ( 'NONE',  ( -9.209823531518070538, 1493.295436042139954, 200.9664195331480130 ) ) ;
#26668=B_SPLINE_SURFACE_WITH_KNOTS ( 'NONE', 5, 1, ( 
 ( #15731, #42627 ),
 ( #101394, #59999 ),
 ( #82974, #50493 ),
 ( #58884, #34220 ),
 ( #33113, #33654 ),
 ( #76779, #97 ),
 ( #108727, #6267 ),
 ( #100326, #93017 ),
 ( #16289, #25801 ) ),
 .UNSPECIFIED., .F., .F., .F.,
 ( 6, 3, 6 ),
 ( 2, 2 ),
 ( 0.000000000000000000, 3.291079314230000108, 6.557401248809999750 ),
 ( 0.000000000000000000, 14.00000000000000000 ),
 .UNSPECIFIED. ) ;
#26672=CARTESIAN_POINT ( 'NONE',  ( 2.175409717514719593E-31, 1397.551704408390151, 209.1218459616989946 ) ) ;
#26689=CARTESIAN_POINT ( 'NONE',  ( 3.114546081289999435, 1442.643943093889902, 217.4397813744189989 ) ) ;
#26693=CARTESIAN_POINT ( 'NONE',  ( -3.159798962964550206, 1454.349606548080146, 199.1257215370219740 ) ) ;
#26694=CARTESIAN_POINT ( 'NONE',  ( 9.611936100793599280, 1460.529534319539835, 206.0552085173229955 ) ) ;
#26697=CARTESIAN_POINT ( 'NONE',  ( -15.17668789299639975, 1418.088918213290071, 203.1695124900660119 ) ) ;
#26698=CARTESIAN_POINT ( 'NONE',  ( 4.328976357965480304, 1515.082833801169954, 207.7712354839940190 ) ) ;
#26700=ORIENTED_EDGE ( 'NONE', *, *, #75300, .F. ) ;
#26701=CARTESIAN_POINT ( 'NONE',  ( -8.282452265539999914, 1508.539485426189913, 219.0858899887390123 ) ) ;
#26702=CARTESIAN_POINT ( 'NONE',  ( -4.832611339330879829, 1508.551704408389924, 211.6097681392950278 ) ) ;
#26709=B_SPLINE_CURVE_WITH_KNOTS ( 'NONE', 5,
 ( #26828, #54265, #95140, #52599, #86735, #27934, #10025, #62117, #63229 ),
 .UNSPECIFIED., .F., .F.,
 ( 6, 3, 6 ),
 ( 0.000000000000000000, 0.3434076321145757560, 1.000000000000000000 ),
 .UNSPECIFIED. ) ;
#26710=CARTESIAN_POINT ( 'NONE',  ( -11.35534575645690047, 1470.545164360740046, 210.1099061434680095 ) ) ;
#26711=CARTESIAN_POINT ( 'NONE',  ( -4.069166842042879928, 1487.126672562190151, 220.0157357502849891 ) ) ;
#26712=CARTESIAN_POINT ( 'NONE',  ( -13.97983671313290088, 1420.196096071459806, 195.9955716203340046 ) ) ;
#26719=ADVANCED_FACE ( 'NONE', ( #101308 ), #18027, .F. ) ;
#26726=CARTESIAN_POINT ( 'NONE',  ( -14.65245215464970130, 1420.119839417710182, 213.8659310620899987 ) ) ;
#26727=ORIENTED_EDGE ( 'NONE', *, *, #66731, .F. ) ;
#26731=CARTESIAN_POINT ( 'NONE',  ( -6.223685729618609663, 1459.529526055099950, 211.3909926741320078 ) ) ;
#26734=CARTESIAN_POINT ( 'NONE',  ( 4.626199203489999690, 1486.054098565890172, 218.8608866932789851 ) ) ;
#26735=CARTESIAN_POINT ( 'NONE',  ( 9.362162057066138132, 1436.138703257420048, 210.0625319500269939 ) ) ;
#26740=CARTESIAN_POINT ( 'NONE',  ( -1.708234279288180169, 1485.711368808090128, 197.3465205308800137 ) ) ;
#26746=VERTEX_POINT ( 'NONE', #85405 ) ;
#26747=CARTESIAN_POINT ( 'NONE',  ( -3.137381254594690194, 1508.729448404669938, 213.6787528672270184 ) ) ;
#26748=CARTESIAN_POINT ( 'NONE',  ( 11.18657871290000116, 1480.479923154690141, 229.7819052381989877 ) ) ;
#26757=CARTESIAN_POINT ( 'NONE',  ( -2.057188004130400039, 1421.133947679400080, 193.7687826666459898 ) ) ;
#26766=CARTESIAN_POINT ( 'NONE',  ( -8.042714958110000367, 1424.476437214510042, 210.0061173360819851 ) ) ;
#26771=CARTESIAN_POINT ( 'NONE',  ( -1.636741614903409969, 1469.777368438049962, 219.0527109355280118 ) ) ;
#26772=CARTESIAN_POINT ( 'NONE',  ( 7.538868782738779473, 1425.612187812159846, 212.1827042067879745 ) ) ;
#26775=VERTEX_POINT ( 'NONE', #102219 ) ;
#26779=CARTESIAN_POINT ( 'NONE',  ( 3.584503077415259753, 1486.500511906220027, 219.3043361390229791 ) ) ;
#26780=CARTESIAN_POINT ( 'NONE',  ( -18.80034332280520104, 1508.551704409080230, 209.8506955288309825 ) ) ;
#26781=CARTESIAN_POINT ( 'NONE',  ( 2.761692215590000110, 1460.406946357790048, 228.5031849494990013 ) ) ;
#26782=CARTESIAN_POINT ( 'NONE',  ( -8.552145378091630334, 1438.550163890339945, 207.4884571577819941 ) ) ;
#26789=EDGE_LOOP ( 'NONE', ( #22728, #60599, #58584, #69532 ) ) ;
#26792=CARTESIAN_POINT ( 'NONE',  ( -10.48474110849999974, 1480.275079708390194, 208.2232256045050178 ) ) ;
#26808=CARTESIAN_POINT ( 'NONE',  ( 4.679791067032149421, 1508.610720099250102, 205.9457795546310024 ) ) ;
#26811=CARTESIAN_POINT ( 'NONE',  ( 2.487935123032369411, 1508.909942010395071, 204.6312267424608820 ) ) ;
#26827=ORIENTED_EDGE ( 'NONE', *, *, #74806, .T. ) ;
#26828=CARTESIAN_POINT ( 'NONE',  ( -4.794426340529999386, 1463.608615258990085, 228.2108236244990280 ) ) ;
#26831=CARTESIAN_POINT ( 'NONE',  ( -20.16530468839962609, 1508.094484761909825, 209.6061611864197687 ) ) ;
#26833=CARTESIAN_POINT ( 'NONE',  ( 1.089943175529721975, 1421.340729913779114, 193.7538244426485790 ) ) ;
#26834=CARTESIAN_POINT ( 'NONE',  ( -10.76760958711749971, 1462.889620211719830, 206.6132149273230141 ) ) ;
#26841=B_SPLINE_SURFACE_WITH_KNOTS ( 'NONE', 5, 5, ( 
 ( #34040, #100682, #23965, #82790, #23430, #32396 ),
 ( #15013, #84980, #16654, #42439, #41895, #83339 ),
 ( #91739, #58708, #50322, #84448, #92290, #6635 ),
 ( #74967, #15560, #25624, #100144, #59270, #49761 ),
 ( #93388, #76598, #83890, #24518, #7734, #68231 ),
 ( #59815, #6084, #76052, #66577, #14472, #48664 ),
 ( #40236, #41353, #75520, #74419, #109654, #108545 ),
 ( #31836, #86649, #78815, #104002, #26177, #86103 ),
 ( #51397, #60930, #9944, #102879, #78251, #1020 ) ),
 .UNSPECIFIED., .F., .F., .F.,
 ( 6, 3, 6 ),
 ( 6, 6 ),
 ( 12.43653261939170029, 21.89999795660000004, 30.61791799421799709 ),
 ( -4.891601802749729813E-05, 2.000000000000000000 ),
 .UNSPECIFIED. ) ;
#26843=CARTESIAN_POINT ( 'NONE',  ( 2.597701311440000271, 1426.721572854839906, 188.7323019695990070 ) ) ;
#26853=CARTESIAN_POINT ( 'NONE',  ( 3.266092768566498439, 1508.418517148852288, 219.8660019118054834 ) ) ;
#26855=CARTESIAN_POINT ( 'NONE',  ( -0.3862241457470880213, 1500.063268800599872, 233.1571801898780052 ) ) ;
#26857=CARTESIAN_POINT ( 'NONE',  ( -21.76329145269999898, 1417.858357255770215, 210.0119042203199911 ) ) ;
#26859=EDGE_CURVE ( 'NONE', #57781, #59685, #47524, .T. ) ;
#26860=CARTESIAN_POINT ( 'NONE',  ( 3.810264595240000052, 1441.769887200890025, 217.2430996589589824 ) ) ;
#26861=ORIENTED_EDGE ( 'NONE', *, *, #7637, .T. ) ;
#26864=CARTESIAN_POINT ( 'NONE',  ( -4.467521880299999637, 1476.320660351190099, 199.7823413832389861 ) ) ;
#26866=EDGE_LOOP ( 'NONE', ( #100130, #4792, #6198, #90490 ) ) ;
#26867=CARTESIAN_POINT ( 'NONE',  ( -4.774552475180789735, 1508.551704408389924, 219.7184675692020051 ) ) ;
#26871=CARTESIAN_POINT ( 'NONE',  ( 4.391835068428125766, 1445.322768932143845, 201.2232284873072103 ) ) ;
#26875=CARTESIAN_POINT ( 'NONE',  ( 0.6272946189549990503, 1431.084551388790032, 217.8556865675190011 ) ) ;
#26877=CARTESIAN_POINT ( 'NONE',  ( -14.82737418450000000, 1417.731569263860138, 213.2974731918289706 ) ) ;
#26888=CARTESIAN_POINT ( 'NONE',  ( 7.808553570872349248, 1465.967952420329993, 215.2103419416679913 ) ) ;
#26890=CARTESIAN_POINT ( 'NONE',  ( 6.044783878490000539, 1450.853430557689990, 209.5026623076140027 ) ) ;
#26892=CARTESIAN_POINT ( 'NONE',  ( -7.596603738389999805, 1494.381468487990105, 200.3558461181089854 ) ) ;
#26902=CARTESIAN_POINT ( 'NONE',  ( 0.5910745650690010233, 1455.956094962490170, 198.5601078200990059 ) ) ;
#26907=CARTESIAN_POINT ( 'NONE',  ( -1.119159361899999983, 1498.157713505790070, 197.8376082938989953 ) ) ;
#26908=CARTESIAN_POINT ( 'NONE',  ( 0.4190295626039989840, 1494.278158734189901, 220.2761818919989878 ) ) ;
#26923=CARTESIAN_POINT ( 'NONE',  ( 2.550017816056660003, 1508.551704408389924, 214.1089244005430317 ) ) ;
#26927=CARTESIAN_POINT ( 'NONE',  ( 9.540313770239269076, 1461.184271939180007, 206.7184343888850151 ) ) ;
#26930=ORIENTED_EDGE ( 'NONE', *, *, #39548, .F. ) ;
#26931=CARTESIAN_POINT ( 'NONE',  ( 8.722999621409400106, 1451.780902529460036, 212.2858504672719846 ) ) ;
#26932=CARTESIAN_POINT ( 'NONE',  ( 9.419895454800000678, 1425.271803998110045, 195.8713000332990077 ) ) ;
#26933=ORIENTED_EDGE ( 'NONE', *, *, #106125, .T. ) ;
#26935=CARTESIAN_POINT ( 'NONE',  ( -12.17364444887732233, 1417.444261838927787, 199.6837928435173524 ) ) ;
#26941=CARTESIAN_POINT ( 'NONE',  ( 10.34945510115269940, 1451.639433892800071, 207.2647969978239928 ) ) ;
#26944=EDGE_LOOP ( 'NONE', ( #45070, #105974, #87137, #43964 ) ) ;
#26958=CARTESIAN_POINT ( 'NONE',  ( 9.224548086651552126, 1450.561207767010046, 209.2764872802650018 ) ) ;
#26960=CARTESIAN_POINT ( 'NONE',  ( 9.739193628800000724, 1492.624356258490025, 214.7590332456690021 ) ) ;
#26962=CARTESIAN_POINT ( 'NONE',  ( 8.930916390941154859, 1424.998531210375177, 195.6484565887391227 ) ) ;
#26963=CARTESIAN_POINT ( 'NONE',  ( -21.25454558919999926, 1505.414223313590128, 209.4451586182409812 ) ) ;
#26964=CARTESIAN_POINT ( 'NONE',  ( 10.01604805806510079, 1469.197346657220123, 203.9457370999409989 ) ) ;
#26966=EDGE_CURVE ( 'NONE', #42556, #105229, #87865, .T. ) ;
#26975=CARTESIAN_POINT ( 'NONE',  ( -14.58313706979999935, 1416.023439710309958, 214.1199149666390156 ) ) ;
#26976=CARTESIAN_POINT ( 'NONE',  ( 0.7087989430401649971, 1515.130721759790049, 204.7941235941219986 ) ) ;
#26978=CARTESIAN_POINT ( 'NONE',  ( -15.88400460199908615, 1415.958461537839639, 209.7364282889150218 ) ) ;
#26980=CARTESIAN_POINT ( 'NONE',  ( 20.21728935790000037, 1475.862786327189951, 209.1218459616989946 ) ) ;
#26981=EDGE_CURVE ( 'NONE', #21533, #49433, #74574, .T. ) ;
#26982=CARTESIAN_POINT ( 'NONE',  ( -16.05592744339999811, 1416.237390274000063, 209.1226952231629923 ) ) ;
#26984=CARTESIAN_POINT ( 'NONE',  ( -10.76610293753739889, 1461.751116445120033, 211.3389343603909936 ) ) ;
#26989=CARTESIAN_POINT ( 'NONE',  ( -8.203088214330000127, 1478.337535159890194, 216.4441348706290285 ) ) ;
#27000=CARTESIAN_POINT ( 'NONE',  ( -15.57711053439999915, 1415.747624789430120, 209.0870974357659975 ) ) ;
#27014=CARTESIAN_POINT ( 'NONE',  ( -5.780263042159999642, 1449.134363676490011, 210.7231825170590014 ) ) ;
#27019=AXIS2_PLACEMENT_3D ( 'NONE', #50202, #84327, #39007 ) ;
#27023=EDGE_CURVE ( 'NONE', #18694, #67656, #40157, .T. ) ;
#27025=CARTESIAN_POINT ( 'NONE',  ( 4.274333237420000486, 1515.341807516890185, 207.6471969281190013 ) ) ;
#27030=CARTESIAN_POINT ( 'NONE',  ( 4.637205103430000364, 1484.703917610690041, 219.2115800062989877 ) ) ;
#27031=CARTESIAN_POINT ( 'NONE',  ( 11.27956504841369956, 1479.374699450910157, 208.0836311270099941 ) ) ;
#27033=CARTESIAN_POINT ( 'NONE',  ( -2.956277750134179705, 1450.104957259319917, 188.5563321079999923 ) ) ;
#27035=CARTESIAN_POINT ( 'NONE',  ( 10.99044570490370099, 1479.494708708640019, 229.8297407083400117 ) ) ;
#27039=CARTESIAN_POINT ( 'NONE',  ( -5.222641464789999688, 1391.931189815790049, 203.5968850314390011 ) ) ;
#27040=CARTESIAN_POINT ( 'NONE',  ( 9.808398454338320249, 1435.362476046070242, 208.7559545901820002 ) ) ;
#27041=CARTESIAN_POINT ( 'NONE',  ( -14.96851909909330125, 1420.519469560630114, 212.0434853293359936 ) ) ;
#27044=CARTESIAN_POINT ( 'NONE',  ( 4.325405441708593202, 1515.219201591195542, 206.7917118349596421 ) ) ;
#27052=CARTESIAN_POINT ( 'NONE',  ( 9.536702226868399634, 1504.881375799320040, 215.9278409599580186 ) ) ;
#27060=CARTESIAN_POINT ( 'NONE',  ( -1.485124824312086922, 1457.022419630208788, 199.7284311504454877 ) ) ;
#27061=CARTESIAN_POINT ( 'NONE',  ( -10.32117538795129974, 1448.479331933469894, 208.0292346068879965 ) ) ;
#27065=EDGE_CURVE ( 'NONE', #26775, #92807, #105298, .T. ) ;
#27066=CARTESIAN_POINT ( 'NONE',  ( 17.88837883210679891, 1459.164429878010196, 217.9459145873090051 ) ) ;
#27073=CARTESIAN_POINT ( 'NONE',  ( -11.94865520339239851, 1422.082048078050093, 208.3249290792549857 ) ) ;
#27083=CARTESIAN_POINT ( 'NONE',  ( -8.356582281726788963, 1474.676444402793095, 203.1368637855367183 ) ) ;
#27085=CARTESIAN_POINT ( 'NONE',  ( -1.910306335979069958, 1465.019396637220098, 198.2840305075910123 ) ) ;
#27087=CARTESIAN_POINT ( 'NONE',  ( 11.46028677100449933, 1422.055054995990076, 209.9672720893090059 ) ) ;
#27101=CARTESIAN_POINT ( 'NONE',  ( 0.5938345015652835013, 1455.008249108801238, 218.5312979207114950 ) ) ;
#27102=CARTESIAN_POINT ( 'NONE',  ( 18.72979941119999836, 1454.437773883689943, 204.5413093961989830 ) ) ;
#27103=CARTESIAN_POINT ( 'NONE',  ( -5.387811863060000483, 1496.648312753189884, 199.2595355468089906 ) ) ;
#27104=CARTESIAN_POINT ( 'NONE',  ( -3.252554812490000113, 1508.258009291689859, 220.7618944614989971 ) ) ;
#27105=CARTESIAN_POINT ( 'NONE',  ( 2.175771579259999644, 1492.304798991390044, 188.2630637080989970 ) ) ;
#27116=VERTEX_POINT ( 'NONE', #81294 ) ;
#27125=CARTESIAN_POINT ( 'NONE',  ( -8.681712390459869866, 1448.751914763990044, 212.0069377265070045 ) ) ;
#27127=ORIENTED_EDGE ( 'NONE', *, *, #100930, .T. ) ;
#27134=CARTESIAN_POINT ( 'NONE',  ( 5.602114820939999795, 1448.090347409289961, 206.1652803823789952 ) ) ;
#27139=CARTESIAN_POINT ( 'NONE',  ( -0.7394123279979990526, 1431.039654945390112, 200.6341525829290049 ) ) ;
#27142=CARTESIAN_POINT ( 'NONE',  ( -0.1522252554610010189, 1508.600545075490118, 220.9033078710990026 ) ) ;
#27143=CARTESIAN_POINT ( 'NONE',  ( -7.847012372209785980, 1448.000573986833842, 213.8304041876558301 ) ) ;
#27145=CARTESIAN_POINT ( 'NONE',  ( 0.000000000000000000, 1378.913060387289988, 209.1218459616989946 ) ) ;
#27146=CARTESIAN_POINT ( 'NONE',  ( 2.526502914729999993, 1486.393260774789951, 198.2275259192990120 ) ) ;
#27147=CARTESIAN_POINT ( 'NONE',  ( 5.518436134040229923, 1466.731182993539960, 200.2557783364140107 ) ) ;
#27149=CARTESIAN_POINT ( 'NONE',  ( 11.66538825820000014, 1501.769421336390224, 211.4581643459090117 ) ) ;
#27151=CARTESIAN_POINT ( 'NONE',  ( 8.000563468399999323, 1425.311447451950016, 211.1882539080190213 ) ) ;
#27154=EDGE_CURVE ( 'NONE', #35203, #34173, #19816, .T. ) ;
#27164=CARTESIAN_POINT ( 'NONE',  ( -11.25901873070000114, 1500.172003391289991, 210.8567363387790010 ) ) ;
#27167=CARTESIAN_POINT ( 'NONE',  ( 0.3787159155534669530, 1456.889667869769937, 219.7399949435159954 ) ) ;
#27171=CARTESIAN_POINT ( 'NONE',  ( 7.428831053269999707, 1425.174870893220032, 212.3938909338090184 ) ) ;
#27172=CARTESIAN_POINT ( 'NONE',  ( 20.33508558929999666, 1432.834457682990205, 214.7556889579689994 ) ) ;
#27187=CARTESIAN_POINT ( 'NONE',  ( 0.7060385530502589768, 1475.942608798000037, 197.6738236987649771 ) ) ;
#27197=ORIENTED_EDGE ( 'NONE', *, *, #83079, .F. ) ;
#27200=CARTESIAN_POINT ( 'NONE',  ( -4.162247305190000191, 1453.824586353890027, 199.5089249234089834 ) ) ;
#27209=B_SPLINE_CURVE_WITH_KNOTS ( 'NONE', 3,
 ( #74755, #58505, #92089, #56848, #65259, #101024, #73660, #48459, #108892, #31626, #43225, #107792, #90980, #109456, #108343, #47888, #34806, #32185, #56294 ),
 .UNSPECIFIED., .F., .F.,
 ( 4, 3, 3, 3, 3, 3, 4 ),
 ( -7.874164591667580204, -7.680830555785009395, -6.505323578896399894, -5.552647998340869862, -4.828139871705260155, -4.001703595992710305, -3.231130238939999622 ),
 .UNSPECIFIED. ) ;
#27220=CARTESIAN_POINT ( 'NONE',  ( 2.326513286163319538, 1476.258183507229887, 197.8633931498989966 ) ) ;
#27225=CARTESIAN_POINT ( 'NONE',  ( 8.631813300402768618, 1438.018477990890005, 210.0180809498099848 ) ) ;
#27235=CARTESIAN_POINT ( 'NONE',  ( -3.703976537560000004, 1430.299880473189887, 201.6469541626590001 ) ) ;
#27248=DIRECTION ( 'NONE',  ( -1.224646799147353947E-16, 1.836970198721029688E-16, 1.000000000000000000 ) ) ;
#27251=CARTESIAN_POINT ( 'NONE',  ( -17.06552703839999907, 1504.165251161390188, 208.8534522804940252 ) ) ;
#27253=CARTESIAN_POINT ( 'NONE',  ( 3.060046444349999728, 1442.201648410489952, 217.5704250855989983 ) ) ;
#27255=CARTESIAN_POINT ( 'NONE',  ( 1966.210325831229966, 11216.44053380570040, 439.9203465415980077 ) ) ;
#27271=CARTESIAN_POINT ( 'NONE',  ( -4.458756895905489515, 1488.529440655459894, 219.1126515454099888 ) ) ;
#27272=CARTESIAN_POINT ( 'NONE',  ( -19.34949465300000071, 1446.106505183189938, 200.0047805777890062 ) ) ;
#27278=CARTESIAN_POINT ( 'NONE',  ( 1.711055448681089940E-31, 1424.874073124720098, 209.1218459616989946 ) ) ;
#27283=EDGE_CURVE ( 'NONE', #94338, #1934, #24169, .T. ) ;
#27287=B_SPLINE_CURVE_WITH_KNOTS ( 'NONE', 3,
 ( #98920, #105134, #72115, #98373, #105699, #21645, #55853, #13246, #47436, #73183 ),
 .UNSPECIFIED., .F., .F.,
 ( 4, 3, 3, 4 ),
 ( -3.121899831669039838, -2.863851907766889582, -1.429084544020210013, 4.440892098500626162E-16 ),
 .UNSPECIFIED. ) ;
#27288=CARTESIAN_POINT ( 'NONE',  ( -19.15307798683139850, 1464.559873833900156, 213.8318764457040118 ) ) ;
#27289=CARTESIAN_POINT ( 'NONE',  ( 6.824596748387858014, 1424.393356309073852, 213.4892280596932892 ) ) ;
#27292=CARTESIAN_POINT ( 'NONE',  ( 9.357192914159959685, 1435.432353859119985, 208.4552369967489938 ) ) ;
#27300=CARTESIAN_POINT ( 'NONE',  ( -16.32813191276419928, 1420.694869237870080, 203.2969751068219750 ) ) ;
#27301=CARTESIAN_POINT ( 'NONE',  ( -11.12609304200080018, 1491.160356735590085, 209.7795734073339986 ) ) ;
#27304=CARTESIAN_POINT ( 'NONE',  ( -12.45097904980000081, 1507.808706184189987, 209.1434958805429858 ) ) ;
#27305=CARTESIAN_POINT ( 'NONE',  ( -2.893915299462510138, 1469.660611638019873, 187.4298741930020071 ) ) ;
#27314=CARTESIAN_POINT ( 'NONE',  ( -10.06805134449999883, 1461.229810737490197, 212.3649339894689945 ) ) ;
#27319=CARTESIAN_POINT ( 'NONE',  ( -8.116268411100000080, 1423.917527323469812, 210.3428539577589902 ) ) ;
#27325=ORIENTED_EDGE ( 'NONE', *, *, #83079, .T. ) ;
#27329=CARTESIAN_POINT ( 'NONE',  ( 1.429289317213857879, 1487.311642763506370, 219.8598652476721611 ) ) ;
#27331=DIRECTION ( 'NONE',  ( -0.7600087925167848812, -0.4999999999970536346, 0.4151946956550925383 ) ) ;
#27332=CARTESIAN_POINT ( 'NONE',  ( -8.565099867639800024, 1437.917637130210096, 207.7375823160310233 ) ) ;
#27344=CARTESIAN_POINT ( 'NONE',  ( 18.58525782085794731, 1474.564397078151160, 201.0252237832114020 ) ) ;
#27345=B_SPLINE_CURVE_WITH_KNOTS ( 'NONE', 5,
 ( #99842, #41048, #92007, #93100, #101483, #47808 ),
 .UNSPECIFIED., .F., .F.,
 ( 6, 6 ),
 ( -2.000000000000000000, -8.403479023755267008E-09 ),
 .UNSPECIFIED. ) ;
#27358=CARTESIAN_POINT ( 'NONE',  ( 3.829619994797929916, 1515.551704292389786, 207.2788821832570250 ) ) ;
#27364=CARTESIAN_POINT ( 'NONE',  ( 7.513730101630000213, 1422.952558782609913, 195.6781497891990114 ) ) ;
#27366=CARTESIAN_POINT ( 'NONE',  ( -3.560962994120000058, 1496.007316878489974, 198.0872883060989977 ) ) ;
#27376=CARTESIAN_POINT ( 'NONE',  ( -17.14979733940000273, 1417.522661905800078, 207.4349891442189744 ) ) ;
#27380=CARTESIAN_POINT ( 'NONE',  ( -20.23414992579679605, 1508.068540423656941, 209.5914070171807850 ) ) ;
#27388=CARTESIAN_POINT ( 'NONE',  ( -9.556981692808550477, 1460.090769935110075, 210.4171492488110005 ) ) ;
#27389=CARTESIAN_POINT ( 'NONE',  ( 3.217394093085149898, 1424.184525167369884, 188.9579921258149966 ) ) ;
#27390=DIRECTION ( 'NONE',  ( -1.000000000000000000, 0.000000000000000000, 0.000000000000000000 ) ) ;
#27391=CARTESIAN_POINT ( 'NONE',  ( 9.957354707566970831, 1462.547202367510181, 211.2474092644970085 ) ) ;
#27398=CARTESIAN_POINT ( 'NONE',  ( -13.67845548232380004, 1504.250296044910101, 227.6838177328889969 ) ) ;
#27400=CARTESIAN_POINT ( 'NONE',  ( -11.71402071852000049, 1489.483213258419937, 212.5376296399540195 ) ) ;
#27406=CARTESIAN_POINT ( 'NONE',  ( -4.016810458580000187, 1476.004922423390099, 199.5922506328190025 ) ) ;
#27407=EDGE_CURVE ( 'NONE', #87891, #84881, #108194, .T. ) ;
#27410=CARTESIAN_POINT ( 'NONE',  ( -7.003352422824639767, 1508.551704404799921, 219.1865514027120128 ) ) ;
#27415=CARTESIAN_POINT ( 'NONE',  ( -1.430539319850000046, 1444.328264637789971, 199.1703804529689990 ) ) ;
#27416=CARTESIAN_POINT ( 'NONE',  ( 0.2166670160139989865, 1431.553687047090079, 218.2358754814289910 ) ) ;
#27424=CARTESIAN_POINT ( 'NONE',  ( 11.13284031615599901, 1491.007009142829929, 208.5102145449120030 ) ) ;
#27427=CARTESIAN_POINT ( 'NONE',  ( 8.937899474855068860, 1465.013579540770252, 213.2848641858089991 ) ) ;
#27431=CARTESIAN_POINT ( 'NONE',  ( -0.7474653422925290336, 1496.370314053810034, 196.7891267297500235 ) ) ;
#27447=CARTESIAN_POINT ( 'NONE',  ( 1.060739532880000002, 1494.110723351890101, 220.2175052815989886 ) ) ;
#27450=ORIENTED_EDGE ( 'NONE', *, *, #86810, .F. ) ;
#27460=CARTESIAN_POINT ( 'NONE',  ( 4.240165130249540226, 1508.551704408389924, 213.3930704938919973 ) ) ;
#27464=CARTESIAN_POINT ( 'NONE',  ( 10.41168706946910127, 1460.024584131529764, 205.9060538633809756 ) ) ;
#27468=CARTESIAN_POINT ( 'NONE',  ( 9.367229934758190879, 1453.004463604660259, 211.8810869144209903 ) ) ;
#27469=CARTESIAN_POINT ( 'NONE',  ( 7.975553363950000474, 1424.201270073840078, 195.7335007005989951 ) ) ;
#27470=VERTEX_POINT ( 'NONE', #80064 ) ;
#27472=CARTESIAN_POINT ( 'NONE',  ( -2.518203147932353225, 1420.414483601807888, 193.9149677586775908 ) ) ;
#27479=DIRECTION ( 'NONE',  ( -0.9099290007293374671, 0.3041652670682291060, 0.2819799708153441498 ) ) ;
#27485=VERTEX_POINT ( 'NONE', #105835 ) ;
#27495=CARTESIAN_POINT ( 'NONE',  ( -3.950491156583319619, 1468.310306949679898, 219.6290600318629913 ) ) ;
#27500=CARTESIAN_POINT ( 'NONE',  ( -2.262341589641910122, 1421.834387796660167, 193.3950565057020015 ) ) ;
#27502=CARTESIAN_POINT ( 'NONE',  ( 9.028476196572741586, 1425.072251678628390, 195.6284098769293678 ) ) ;
#27504=CARTESIAN_POINT ( 'NONE',  ( -17.55491153119999836, 1504.812299793789862, 208.9605407232600101 ) ) ;
#27509=VERTEX_POINT ( 'NONE', #34624 ) ;
#27513=B_SPLINE_SURFACE_WITH_KNOTS ( 'NONE', 5, 5, ( 
 ( #52493, #76017, #68750, #24492, #103407, #78225 ),
 ( #16086, #1536, #34565, #9371, #102853, #991 ),
 ( #35117, #101195, #50293, #69300, #26711, #62582 ),
 ( #36229, #27271, #96131, #95580, #46318, #45760 ),
 ( #79897, #62010, #54164, #12125, #37894, #44645 ),
 ( #79343, #36782, #20504, #71536, #105657, #72076 ),
 ( #19409, #70414, #3210, #70974, #78787, #28380 ),
 ( #53611, #37339, #96699, #63130, #97232, #80447 ),
 ( #18849, #53045, #11035, #106190, #87753, #2655 ),
 ( #87184, #28942, #105090, #88289, #54713, #19970 ),
 ( #69857, #3760, #11584, #45202, #88839, #104534 ),
 ( #103976, #61455, #27830, #10474, #2101, #27400 ) ),
 .UNSPECIFIED., .F., .F., .F.,
 ( 6, 3, 3, 6 ),
 ( 6, 6 ),
 ( 13.45148704079599966, 21.22852775220000154, 29.00530734079999817, 33.91527837888789776 ),
 ( -0.0002611228039829010042, 2.000000000000000000 ),
 .UNSPECIFIED. ) ;
#27515=CARTESIAN_POINT ( 'NONE',  ( 4.025751050180000234, 1506.805340958390161, 220.0912426404989901 ) ) ;
#27518=CARTESIAN_POINT ( 'NONE',  ( -0.2432117950169480070, 1515.155210303460080, 204.7947648491820019 ) ) ;
#27520=CARTESIAN_POINT ( 'NONE',  ( -17.43675326300159867, 1417.688629928019964, 206.2161178420579972 ) ) ;
#27528=AXIS2_PLACEMENT_3D ( 'NONE', #98525, #63313, #36970 ) ;
#27533=CARTESIAN_POINT ( 'NONE',  ( -10.94901061624040040, 1481.831333076229839, 207.7501958990100093 ) ) ;
#27543=B_SPLINE_CURVE_WITH_KNOTS ( 'NONE', 5,
 ( #56002, #47056, #5030, #107483, #11784, #39175, #4496, #20711, #38629 ),
 .UNSPECIFIED., .F., .F.,
 ( 6, 3, 6 ),
 ( -12.84112607031869935, -7.747513759300000302, -3.918736331710000798 ),
 .UNSPECIFIED. ) ;
#27552=ORIENTED_EDGE ( 'NONE', *, *, #79593, .F. ) ;
#27555=CARTESIAN_POINT ( 'NONE',  ( -12.85018798063330081, 1508.236131449000140, 209.4043565344470039 ) ) ;
#27566=B_SPLINE_CURVE_WITH_KNOTS ( 'NONE', 5,
 ( #51059, #6289, #15753, #67322, #66777, #14684 ),
 .UNSPECIFIED., .F., .F.,
 ( 6, 6 ),
 ( 115.1755349879999955, 119.9142073339999968 ),
 .UNSPECIFIED. ) ;
#27574=CARTESIAN_POINT ( 'NONE',  ( 3.926929841440000235, 1423.889174606040115, 192.9370842642990169 ) ) ;
#27575=CARTESIAN_POINT ( 'NONE',  ( -4.390441442984810649, 1449.947851038559975, 190.5482995516449876 ) ) ;
#27576=CARTESIAN_POINT ( 'NONE',  ( 20.82993010370000064, 1457.408288935790097, 206.8069621084789844 ) ) ;
#27582=CARTESIAN_POINT ( 'NONE',  ( -12.19439603320000032, 1490.074496100290162, 210.2238046367189952 ) ) ;
#27585=CARTESIAN_POINT ( 'NONE',  ( 4.329448776040000446, 1515.064792882589927, 206.7917118356089929 ) ) ;
#27586=EDGE_CURVE ( 'NONE', #5707, #69529, #26340, .T. ) ;
#27591=CARTESIAN_POINT ( 'NONE',  ( 11.36583536198319955, 1502.344531051060130, 215.0256689626610012 ) ) ;
#27600=CARTESIAN_POINT ( 'NONE',  ( 0.1035575932523252335, 1457.708278094112984, 199.5842560823692793 ) ) ;
#27605=B_SPLINE_CURVE_WITH_KNOTS ( 'NONE', 3,
 ( #68558, #60152, #70242, #94273, #104349, #85316, #45577, #56149, #97064, #98139, #38238, #5190, #89201, #64026, #106017, #20330, #63488, #12494, #72421, #73520, #55625, #89748, #30939, #39345, #29293, #55074, #72961, #105459, #97608, #65116, #53986, #13020, #99227, #28749, #47206, #20878, #62953, #46676, #80808, #46127, #13567, #79719, #106552, #54534, #90286, #21414 ),
 .UNSPECIFIED., .F., .F.,
 ( 4, 3, 3, 3, 3, 3, 3, 3, 3, 3, 3, 3, 3, 3, 3, 4 ),
 ( -32.67973531808329568, -31.64931769156649821, -30.28925356829410021, -28.92077687594739999, -27.54739078441340183, -26.16616490320429733, -24.78057410064459987, -23.39129159825840176, -22.83865932529860032, -21.47138836030729792, -20.09934210731429971, -18.72767567390599908, -17.36349881665530148, -16.00861653030469967, -14.66567884330130056, -13.33660260599999958 ),
 .UNSPECIFIED. ) ;
#27606=EDGE_CURVE ( 'NONE', #54763, #40367, #78307, .T. ) ;
#27613=CARTESIAN_POINT ( 'NONE',  ( -5.849558551512059168, 1424.853816168500089, 209.2574496775069974 ) ) ;
#27614=CARTESIAN_POINT ( 'NONE',  ( 4.987363906429999716, 1436.241616669089808, 206.8881657794889861 ) ) ;
#27625=CARTESIAN_POINT ( 'NONE',  ( 2.026230520227449983, 1465.919631588679977, 198.2820304006920082 ) ) ;
#27628=CARTESIAN_POINT ( 'NONE',  ( 3.350944662710000355, 1464.628126271390101, 199.8699733667390035 ) ) ;
#27630=CARTESIAN_POINT ( 'NONE',  ( 8.644029068445851394, 1437.385894306310092, 208.7514692825569966 ) ) ;
#27635=CARTESIAN_POINT ( 'NONE',  ( 11.73501141340019949, 1479.231774555940092, 208.2345455324859813 ) ) ;
#27643=CARTESIAN_POINT ( 'NONE',  ( 0.9695034778824223043, 1454.901985832918399, 218.4941352939971466 ) ) ;
#27649=CARTESIAN_POINT ( 'NONE',  ( 4.186152965159999795, 1492.613584369290038, 188.5705375364989891 ) ) ;
#27657=CARTESIAN_POINT ( 'NONE',  ( -11.68864801762120109, 1482.492120394230142, 206.8697282117639986 ) ) ;
#27668=CIRCLE ( 'NONE', #99173, 15.09021984820000029 ) ;
#27677=EDGE_CURVE ( 'NONE', #12462, #86830, #58293, .T. ) ;
#27682=CARTESIAN_POINT ( 'NONE',  ( 3.235048502819999783, 1466.472015869789857, 219.6884156563990018 ) ) ;
#27683=CARTESIAN_POINT ( 'NONE',  ( 1.156001302284453303, 1469.029874416468601, 219.0895512148256046 ) ) ;
#27687=CARTESIAN_POINT ( 'NONE',  ( 1.515282459810000093, 1431.991175246789908, 200.7184021833390091 ) ) ;
#27689=CARTESIAN_POINT ( 'NONE',  ( 2.446683647589999566, 1506.492871364290068, 220.9379107316989916 ) ) ;
#27690=CARTESIAN_POINT ( 'NONE',  ( -4.226426730290000044, 1515.477082009390188, 209.4928634131090348 ) ) ;
#27693=CARTESIAN_POINT ( 'NONE',  ( 2.975001697819999791, 1486.548690899389840, 198.3380112669989899 ) ) ;
#27694=CARTESIAN_POINT ( 'NONE',  ( 10.04185642635390074, 1469.459450719869892, 207.3542015582230249 ) ) ;
#27696=CARTESIAN_POINT ( 'NONE',  ( -8.881784197000000993E-16, 1414.413060387330006, 209.1218459616989946 ) ) ;
#27698=CARTESIAN_POINT ( 'NONE',  ( 8.348235655690000812, 1423.006858839259849, 212.9515974749489828 ) ) ;
#27701=CARTESIAN_POINT ( 'NONE',  ( -9.087499124679998985, 1482.679315955489756, 203.1872625214689947 ) ) ;
#27709=CARTESIAN_POINT ( 'NONE',  ( -13.58739845499320076, 1508.434607234060195, 209.8723785710020309 ) ) ;
#27711=CARTESIAN_POINT ( 'NONE',  ( 2.045814292219999775, 1449.354251884889891, 190.1385047842989877 ) ) ;
#27713=CARTESIAN_POINT ( 'NONE',  ( -2.259335814679200194, 1457.676294062130182, 219.5407953899610050 ) ) ;
#27717=CARTESIAN_POINT ( 'NONE',  ( 7.746190077790000572, 1425.513952521069996, 211.7745271020289977 ) ) ;
#27718=CARTESIAN_POINT ( 'NONE',  ( 18.94656048379999902, 1455.761273475090093, 200.3458234316790083 ) ) ;
#27749=CARTESIAN_POINT ( 'NONE',  ( 7.901745564190000515, 1424.856359000810016, 211.6778634635190031 ) ) ;
#27767=CARTESIAN_POINT ( 'NONE',  ( 4.687651746879999415, 1478.378160227390254, 228.9010599218989910 ) ) ;
#27777=ORIENTED_EDGE ( 'NONE', *, *, #26981, .T. ) ;
#27783=CARTESIAN_POINT ( 'NONE',  ( -2.738226213839999978, 1429.529162839389755, 200.8905597157389877 ) ) ;
#27795=CARTESIAN_POINT ( 'NONE',  ( 10.92462469921369994, 1470.600674883090051, 208.4273988239069979 ) ) ;
#27796=EDGE_LOOP ( 'NONE', ( #44696, #83769, #39083, #38997 ) ) ;
#27798=EDGE_CURVE ( 'NONE', #4789, #86013, #91789, .T. ) ;
#27799=CARTESIAN_POINT ( 'NONE',  ( 8.000452546092619244, 1425.311357000540056, 211.1883339932590218 ) ) ;
#27808=UNCERTAINTY_MEASURE_WITH_UNIT (LENGTH_MEASURE( 1.000000000000000082E-05 ), #24282, 'distance_accuracy_value', 'NONE');
#27809=CARTESIAN_POINT ( 'NONE',  ( 2.792478474500000196, 1441.472946933690082, 218.6424847214589988 ) ) ;
#27819=CARTESIAN_POINT ( 'NONE',  ( -5.074768907954896768, 1391.842035882342770, 203.6019732846310717 ) ) ;
#27825=CARTESIAN_POINT ( 'NONE',  ( -4.347083409420000599, 1484.166081217490046, 199.1975610816789981 ) ) ;
#27830=CARTESIAN_POINT ( 'NONE',  ( -10.62221739863140080, 1490.415717394859939, 212.3810854760239977 ) ) ;
#27831=CARTESIAN_POINT ( 'NONE',  ( -19.73707534100000061, 1467.795347597790169, 204.3773262252089751 ) ) ;
#27849=CARTESIAN_POINT ( 'NONE',  ( -3.686527624546230175, 1495.487496192859908, 197.3578822790109939 ) ) ;
#27857=CARTESIAN_POINT ( 'NONE',  ( -13.35343597923650094, 1422.178733618030037, 203.8110371803210228 ) ) ;
#27861=CARTESIAN_POINT ( 'NONE',  ( -4.058188250217909854, 1508.551704408389924, 213.8008314270979895 ) ) ;
#27863=CARTESIAN_POINT ( 'NONE',  ( -4.214505117019999858, 1482.742666855489915, 231.1823280205989875 ) ) ;
#27865=CARTESIAN_POINT ( 'NONE',  ( 8.315094184529998600, 1421.392059295079889, 196.2232414242990046 ) ) ;
#27873=CARTESIAN_POINT ( 'NONE',  ( -8.059380280939999253, 1459.910125804190102, 215.8672651265090110 ) ) ;
#27877=ORIENTED_EDGE ( 'NONE', *, *, #52826, .T. ) ;
#27878=CARTESIAN_POINT ( 'NONE',  ( -8.835341282630000848, 1423.496088729460098, 209.1285750384680284 ) ) ;
#27879=VERTEX_POINT ( 'NONE', #14663 ) ;
#27884=CARTESIAN_POINT ( 'NONE',  ( -2.497291879483329868, 1496.910934660279963, 221.2460707102099775 ) ) ;
#27889=CARTESIAN_POINT ( 'NONE',  ( -0.3911955968562167429, 1487.889068533830141, 219.9704178722953429 ) ) ;
#27890=CARTESIAN_POINT ( 'NONE',  ( -16.92975820021440114, 1508.551704415790027, 212.8312192336030080 ) ) ;
#27891=CARTESIAN_POINT ( 'NONE',  ( 7.003548532139999949, 1472.375330369690118, 216.7528799998890179 ) ) ;
#27892=CARTESIAN_POINT ( 'NONE',  ( -9.119406448533400322, 1439.059517726039985, 208.3668274699830079 ) ) ;
#27893=ORIENTED_EDGE ( 'NONE', *, *, #45670, .F. ) ;
#27897=CARTESIAN_POINT ( 'NONE',  ( 9.468608843732580382, 1434.567639565649870, 206.6665354939389943 ) ) ;
#27902=CARTESIAN_POINT ( 'NONE',  ( 0.6065152646886989851, 1467.309601164520018, 220.1865271459919882 ) ) ;
#27905=B_SPLINE_CURVE_WITH_KNOTS ( 'NONE', 3,
 ( #82120, #41231, #5422, #24407, #107875, #5974, #49644, #31163, #74304, #6522, #92181, #83780, #32814 ),
 .UNSPECIFIED., .F., .F.,
 ( 4, 3, 3, 3, 4 ),
 ( 0.000000000000000000, 0.9022774465060450222, 1.803253076899530072, 2.701853961413190230, 3.242714680140000194 ),
 .UNSPECIFIED. ) ;
#27934=CARTESIAN_POINT ( 'NONE',  ( -15.75277756397573725, 1465.459959653623173, 221.5528956270499918 ) ) ;
#27935=CARTESIAN_POINT ( 'NONE',  ( -9.878262157267270638, 1481.129258223239958, 205.3616989145060074 ) ) ;
#27941=CARTESIAN_POINT ( 'NONE',  ( -4.327392289582439489, 1515.143326931960019, 208.6051541441859740 ) ) ;
#27948=CARTESIAN_POINT ( 'NONE',  ( -14.14028587358620115, 1420.975139497910050, 196.1143637960159936 ) ) ;
#27949=ORIENTED_EDGE ( 'NONE', *, *, #48082, .T. ) ;
#27956=CARTESIAN_POINT ( 'NONE',  ( -17.01076621896756791, 1419.968529181750682, 207.7081154596805277 ) ) ;
#27959=CARTESIAN_POINT ( 'NONE',  ( -4.246467356640679647, 1508.879014458369966, 205.3739677720240024 ) ) ;
#27961=CARTESIAN_POINT ( 'NONE',  ( 1766.069695707609526, -8382.262153571264207, 2383.103299250912187 ) ) ;
#27963=CARTESIAN_POINT ( 'NONE',  ( 5.311671089129999856, 1436.871628643890062, 207.8685812842290375 ) ) ;
#27966=CARTESIAN_POINT ( 'NONE',  ( -4.818091668840000175, 1474.858187015290014, 199.5909790158089834 ) ) ;
#27969=CARTESIAN_POINT ( 'NONE',  ( -7.198248339227330206, 1508.551704405200098, 219.1372379941830388 ) ) ;
#27970=ORIENTED_EDGE ( 'NONE', *, *, #88751, .F. ) ;
#27975=CARTESIAN_POINT ( 'NONE',  ( -2.479799395000000128, 1432.887831698689979, 218.3414119524190085 ) ) ;
#27976=CARTESIAN_POINT ( 'NONE',  ( -11.02285301547030016, 1471.443673802609965, 206.7922591627839779 ) ) ;
#27986=VERTEX_POINT ( 'NONE', #101962 ) ;
#27987=ORIENTED_EDGE ( 'NONE', *, *, #46007, .T. ) ;
#27990=CARTESIAN_POINT ( 'NONE',  ( -2.425929306259190010, 1495.896635296460090, 197.0250612545490014 ) ) ;
#27992=CARTESIAN_POINT ( 'NONE',  ( 11.52300753767129926, 1427.577114572419759, 209.4088601504140286 ) ) ;
#28002=CARTESIAN_POINT ( 'NONE',  ( 0.8070291312159990627, 1495.806080077989918, 221.0513106237990257 ) ) ;
#28013=CARTESIAN_POINT ( 'NONE',  ( 3.323701945149999393, 1484.956221099589811, 220.0842286830989849 ) ) ;
#28015=CARTESIAN_POINT ( 'NONE',  ( 19.52205342210000083, 1473.076230373790168, 204.3554439105789982 ) ) ;
#28021=ORIENTED_EDGE ( 'NONE', *, *, #95276, .F. ) ;
#28023=B_SPLINE_CURVE_WITH_KNOTS ( 'NONE', 3,
 ( #24362, #7575, #41729, #77001, #105366, #97511, #77549, #37605, #103264, #37048, #9241, #52366, #46579, #96973, #80713, #4022, #85367, #25455, #34434, #20237, #51799, #59649 ),
 .UNSPECIFIED., .F., .F.,
 ( 4, 3, 3, 3, 3, 3, 3, 4 ),
 ( 0.000000000000000000, 1.302509916939140089, 2.511839277136839854, 3.228995734685269792, 4.125930029771439855, 5.291961157905718416, 6.057839889249209797, 6.457992286039999641 ),
 .UNSPECIFIED. ) ;
#28024=CARTESIAN_POINT ( 'NONE',  ( 9.164720064741960215, 1452.458489836430090, 211.4562277055130153 ) ) ;
#28025=CARTESIAN_POINT ( 'NONE',  ( 8.043354450609999873, 1424.603816335180227, 195.4430761869989794 ) ) ;
#28027=CARTESIAN_POINT ( 'NONE',  ( -7.604289863101939773, 1426.735970264149955, 206.0920986175900111 ) ) ;
#28043=CARTESIAN_POINT ( 'NONE',  ( -3.747744696529340391, 1508.283495248520012, 220.6268602264730134 ) ) ;
#28045=CARTESIAN_POINT ( 'NONE',  ( -7.584666794553579727, 1470.726758701579911, 215.8813880928350102 ) ) ;
#28050=CARTESIAN_POINT ( 'NONE',  ( 9.946821680530000265, 1491.974962277590066, 214.0087608140690065 ) ) ;
#28052=CARTESIAN_POINT ( 'NONE',  ( 8.327730581979166047, 1424.424880086262192, 195.7445179161305191 ) ) ;
#28053=CARTESIAN_POINT ( 'NONE',  ( -19.29582496549999959, 1504.771663335689937, 209.4684985698930006 ) ) ;
#28054=CARTESIAN_POINT ( 'NONE',  ( 2.719262146893400038E-32, 1524.051704408389924, 209.1218459616989946 ) ) ;
#28056=CARTESIAN_POINT ( 'NONE',  ( -9.897863003022139949, 1439.796600576999936, 207.6605474465260102 ) ) ;
#28057=B_SPLINE_CURVE_WITH_KNOTS ( 'NONE', 5,
 ( #86895, #10756, #53319, #103125, #103697, #104254 ),
 .UNSPECIFIED., .F., .F.,
 ( 6, 6 ),
 ( -48.30090645053910237, -44.26078367470000074 ),
 .UNSPECIFIED. ) ;
#28065=CARTESIAN_POINT ( 'NONE',  ( 5.247543271890000582, 1505.478499777190109, 219.9306779546989787 ) ) ;
#28067=CARTESIAN_POINT ( 'NONE',  ( 1.345088944733950020, 1515.083299843980058, 204.7928818079469977 ) ) ;
#28069=CARTESIAN_POINT ( 'NONE',  ( -15.77920420956434278, 1415.808500209527892, 209.6969280600988270 ) ) ;
#28073=CARTESIAN_POINT ( 'NONE',  ( -6.403692060479999171, 1460.996305860290249, 208.5086931504900178 ) ) ;
#28081=CARTESIAN_POINT ( 'NONE',  ( -3.439963044070000198, 1475.703222825189869, 218.9903645809689863 ) ) ;
#28092=CARTESIAN_POINT ( 'NONE',  ( -15.09085391114290076, 1417.962848745290103, 203.1738905416179932 ) ) ;
#28093=FACE_OUTER_BOUND ( 'NONE', #89378, .T. ) ;
#28095=CARTESIAN_POINT ( 'NONE',  ( -15.42581583419999980, 1414.720317085819943, 208.9801203947009753 ) ) ;
#28107=CARTESIAN_POINT ( 'NONE',  ( -11.75272968278660102, 1481.381864203570103, 210.6216001990260054 ) ) ;
#28128=CARTESIAN_POINT ( 'NONE',  ( 8.279103254549998070, 1462.500663624690105, 228.8590808785990021 ) ) ;
#28132=CARTESIAN_POINT ( 'NONE',  ( -5.177091008439999698, 1391.906304745790067, 203.7213657723089852 ) ) ;
#28134=CARTESIAN_POINT ( 'NONE',  ( -11.71870426870000159, 1490.183039387389726, 210.4915346308890207 ) ) ;
#28141=CARTESIAN_POINT ( 'NONE',  ( 9105.849827169598939, -2339.246371527900010, 1987.591931316750106 ) ) ;
#28150=CARTESIAN_POINT ( 'NONE',  ( 11.74132753969999854, 1499.920429264490167, 205.7525976432890218 ) ) ;
#28153=CARTESIAN_POINT ( 'NONE',  ( 4.637775890913160559, 1462.124487089030026, 228.1829411063220050 ) ) ;
#28157=CARTESIAN_POINT ( 'NONE',  ( -0.8252990750830009326, 1467.903802984689946, 219.8254095440989886 ) ) ;
#28161=EDGE_CURVE ( 'NONE', #67656, #53131, #59688, .T. ) ;
#28163=CARTESIAN_POINT ( 'NONE',  ( -4.721762350340170222, 1427.756354696789913, 206.2331009145199801 ) ) ;
#28166=CARTESIAN_POINT ( 'NONE',  ( 3.217370068670000194, 1424.184623524309927, 188.9579833761989960 ) ) ;
#28171=ORIENTED_EDGE ( 'NONE', *, *, #51535, .F. ) ;
#28177=CARTESIAN_POINT ( 'NONE',  ( 9.854289541820000053, 1461.890233428590136, 208.5812305969039926 ) ) ;
#28181=CARTESIAN_POINT ( 'NONE',  ( 2.329876351239999810, 1465.568987598989906, 199.1151359320989798 ) ) ;
#28187=VERTEX_POINT ( 'NONE', #28027 ) ;
#28192=CARTESIAN_POINT ( 'NONE',  ( 6.784288798619999561, 1469.672316088890057, 209.8806407344229967 ) ) ;
#28197=CARTESIAN_POINT ( 'NONE',  ( -4.721942846059999255, 1507.702795164189865, 221.1964433947989903 ) ) ;
#28199=CARTESIAN_POINT ( 'NONE',  ( 5.365832140090000202, 1437.051389308390071, 208.1168906416689879 ) ) ;
#28207=CARTESIAN_POINT ( 'NONE',  ( 18.03609881821840233, 1455.831125781012133, 201.4491494968732468 ) ) ;
#28213=CARTESIAN_POINT ( 'NONE',  ( -14.85774914289999948, 1415.975901282089808, 204.9891733264790048 ) ) ;
#28226=CARTESIAN_POINT ( 'NONE',  ( -1.125259334100000119, 1515.531689041389882, 213.2129490267590199 ) ) ;
#28231=CARTESIAN_POINT ( 'NONE',  ( 3.544347521480000207, 1468.165829367189872, 218.4679976267089785 ) ) ;
#28236=CARTESIAN_POINT ( 'NONE',  ( -1.397191924980000000, 1429.761471156189828, 199.8249656450389864 ) ) ;
#28238=CARTESIAN_POINT ( 'NONE',  ( 2.495851582740000296, 1506.888954652989923, 220.6874564687990130 ) ) ;
#28243=CARTESIAN_POINT ( 'NONE',  ( 4.342298062439800432, 1465.915122575709802, 200.0011775771919815 ) ) ;
#28256=FACE_OUTER_BOUND ( 'NONE', #57255, .T. ) ;
#28258=CARTESIAN_POINT ( 'NONE',  ( -11.33647332202903080, 1502.116505749242378, 207.3325129751629845 ) ) ;
#28262=CARTESIAN_POINT ( 'NONE',  ( -9.913260568299229192, 1438.794448387919829, 209.9868099401009829 ) ) ;
#28265=ADVANCED_FACE ( 'NONE', ( #49258 ), #7972, .T. ) ;
#28268=CARTESIAN_POINT ( 'NONE',  ( 7.595196814659999518, 1425.935899813689957, 212.0840209023990042 ) ) ;
#28269=CARTESIAN_POINT ( 'NONE',  ( -3.071476887830000280, 1470.850261538789937, 187.3986309372990036 ) ) ;
#28282=CARTESIAN_POINT ( 'NONE',  ( 1.968601690575629615, 1498.935401749600032, 197.9561509338619771 ) ) ;
#28286=CARTESIAN_POINT ( 'NONE',  ( -2.989231773490640176, 1464.638009085429985, 198.9533349682120047 ) ) ;
#28309=CARTESIAN_POINT ( 'NONE',  ( 8.220300753029999186, 1427.204169894219831, 212.0038158565590152 ) ) ;
#28315=CARTESIAN_POINT ( 'NONE',  ( 11.86100282799569960, 1492.894947744830006, 212.5846961511890072 ) ) ;
#28317=CARTESIAN_POINT ( 'NONE',  ( 9.600314864117150293, 1462.464356163139882, 207.4456482718869950 ) ) ;
#28331=CARTESIAN_POINT ( 'NONE',  ( -13.90061681514290015, 1502.276395855860073, 227.4029517098429949 ) ) ;
#28333=ORIENTED_EDGE ( 'NONE', *, *, #43903, .F. ) ;
#28339=CARTESIAN_POINT ( 'NONE',  ( -2.875332210020000279, 1429.155786104789968, 200.6010274126990112 ) ) ;
#28342=CARTESIAN_POINT ( 'NONE',  ( -5.311724842150000292, 1500.891271500089942, 229.7588813323989996 ) ) ;
#28349=CARTESIAN_POINT ( 'NONE',  ( 10.36759898501759913, 1469.933492258360047, 207.4161449764170015 ) ) ;
#28357=CARTESIAN_POINT ( 'NONE',  ( 3.090732370630000059, 1442.657375189589857, 217.4492349673389811 ) ) ;
#28359=CARTESIAN_POINT ( 'NONE',  ( -1847.405368200898920, -8387.357407334300660, -1167.591558398288043 ) ) ;
#28366=CARTESIAN_POINT ( 'NONE',  ( -5.152852264748282174, 1391.896122684712282, 203.6724224095950149 ) ) ;
#28369=FACE_OUTER_BOUND ( 'NONE', #103505, .T. ) ;
#28380=CARTESIAN_POINT ( 'NONE',  ( -9.202353901899998689, 1488.302798292690113, 217.0664071269289934 ) ) ;
#28381=CARTESIAN_POINT ( 'NONE',  ( -13.67845557849999949, 1504.250295190390034, 227.6838176112990197 ) ) ;
#28386=CARTESIAN_POINT ( 'NONE',  ( 6.406055020080000162, 1428.231850363690000, 214.6517644217489931 ) ) ;
#28387=CARTESIAN_POINT ( 'NONE',  ( -18.83642247210000065, 1444.248298674089938, 209.1218459616989946 ) ) ;
#28404=CARTESIAN_POINT ( 'NONE',  ( -4.137865169369999485, 1481.950712913389907, 229.2071242064990315 ) ) ;
#28409=CARTESIAN_POINT ( 'NONE',  ( -1.548360550261279833, 1515.071586600709907, 213.4511168375470049 ) ) ;
#28411=CARTESIAN_POINT ( 'NONE',  ( -9.197351350889000798, 1424.498960654269922, 204.7249030865850159 ) ) ;
#28418=CARTESIAN_POINT ( 'NONE',  ( -22.16283322808959966, 1485.376191718830114, 217.1686774328890124 ) ) ;
#28425=CARTESIAN_POINT ( 'NONE',  ( -9.941476430729998981, 1461.322233694490023, 211.0754656104689957 ) ) ;
#28429=CARTESIAN_POINT ( 'NONE',  ( -8.101682389679998764, 1423.901782527849946, 210.4428033686490096 ) ) ;
#28430=ORIENTED_EDGE ( 'NONE', *, *, #89948, .T. ) ;
#28434=PLANE ( 'NONE',  #85510 ) ;
#28435=CARTESIAN_POINT ( 'NONE',  ( 7.091651353261220869, 1426.649169667290153, 213.2026143799430145 ) ) ;
#28436=AXIS2_PLACEMENT_3D ( 'NONE', #9734, #59599, #109996 ) ;
#28438=B_SPLINE_SURFACE_WITH_KNOTS ( 'NONE', 5, 5, ( 
 ( #102538, #101429, #25829, #24720, #95269, #60587 ),
 ( #77915, #26963, #18531, #103665, #10153, #1222 ),
 ( #69544, #75719, #33142, #58917, #93048, #50522 ),
 ( #62243, #54931, #36454, #2341, #78470, #96928 ),
 ( #28053, #3432, #20195, #89060, #12345, #35920 ),
 ( #37563, #70652, #29703, #104769, #28612, #79582 ),
 ( #11276, #37005, #53284, #54394, #96369, #27504 ),
 ( #45981, #61691, #97467, #72286, #87423, #98002 ),
 ( #19648, #87988, #2887, #53851, #45439, #70103 ),
 ( #88526, #10719, #71197, #20736, #63349, #71763 ),
 ( #11811, #46536, #80670, #104216, #80113, #105880 ),
 ( #3984, #105319, #62812, #29161, #38108, #106418 ) ),
 .UNSPECIFIED., .F., .F., .F.,
 ( 6, 3, 3, 6 ),
 ( 6, 6 ),
 ( 6.066676742310000314, 9.538385084389998880, 13.68355489660000046, 19.24621227249999933 ),
 ( 0.000000000000000000, 0.5000000000000000000 ),
 .UNSPECIFIED. ) ;
#28443=AXIS2_PLACEMENT_3D ( 'NONE', #63963, #90780, #57215 ) ;
#28445=CARTESIAN_POINT ( 'NONE',  ( 9.079459637170000263, 1470.934168148190111, 213.6782594943889819 ) ) ;
#28446=CARTESIAN_POINT ( 'NONE',  ( -8.178798132767068907, 1438.657504337420050, 206.1307692081600180 ) ) ;
#28451=CARTESIAN_POINT ( 'NONE',  ( 8.537244690487868937, 1435.714930654649834, 207.3103916605290067 ) ) ;
#28454=ORIENTED_EDGE ( 'NONE', *, *, #15810, .F. ) ;
#28456=CARTESIAN_POINT ( 'NONE',  ( 11.39540147253980074, 1471.141865352140258, 209.7217653457960012 ) ) ;
#28458=CARTESIAN_POINT ( 'NONE',  ( 15.45719918680149974, 1473.646226760320360, 195.7768488996430847 ) ) ;
#28461=CARTESIAN_POINT ( 'NONE',  ( 9.247631459069999948, 1454.170661380389902, 214.4254682548290134 ) ) ;
#28468=ORIENTED_EDGE ( 'NONE', *, *, #41104, .F. ) ;
#28480=CARTESIAN_POINT ( 'NONE',  ( 10.92857262880000135, 1460.888923995989899, 208.5047758091729690 ) ) ;
#28484=CARTESIAN_POINT ( 'NONE',  ( 16.86071788331999954, 1430.053758721836402, 201.2513078365784622 ) ) ;
#28488=CARTESIAN_POINT ( 'NONE',  ( -16.81730356679999971, 1417.162085555489966, 207.4277572267089909 ) ) ;
#28493=CARTESIAN_POINT ( 'NONE',  ( -10.61999372029469946, 1462.990852176999852, 206.0510140530389833 ) ) ;
#28498=CARTESIAN_POINT ( 'NONE',  ( -9.743700617285488974, 1461.082141979609787, 210.4654820370750201 ) ) ;
#28500=CARTESIAN_POINT ( 'NONE',  ( 9.559657396529310347, 1499.907619752240180, 202.5223157849819984 ) ) ;
#28505=CARTESIAN_POINT ( 'NONE',  ( -1.208143323520000090, 1443.877572099090230, 199.8977861043090059 ) ) ;
#28506=CARTESIAN_POINT ( 'NONE',  ( -16.83458865165958329, 1489.059916236708887, 195.6887827414307424 ) ) ;
#28509=CARTESIAN_POINT ( 'NONE',  ( 7.360599658199999062, 1427.547306193929899, 213.0878178632989943 ) ) ;
#28513=CARTESIAN_POINT ( 'NONE',  ( 1966.823930461590180, 11221.53578756869865, 443.7115846868979929 ) ) ;
#28516=ORIENTED_EDGE ( 'NONE', *, *, #8529, .T. ) ;
#28521=CARTESIAN_POINT ( 'NONE',  ( -4.462434020839999960, 1475.381478586690037, 199.6802092454289834 ) ) ;
#28524=CARTESIAN_POINT ( 'NONE',  ( 2.740681441353109982, 1426.136206333369955, 188.7843748818769996 ) ) ;
#28525=ORIENTED_EDGE ( 'NONE', *, *, #100665, .F. ) ;
#28527=CARTESIAN_POINT ( 'NONE',  ( 2.453554202689999908, 1485.341762335490102, 201.5382166200789698 ) ) ;
#28531=CARTESIAN_POINT ( 'NONE',  ( -2.762666289370000250, 1431.313464822989999, 217.0512884656089909 ) ) ;
#28537=CARTESIAN_POINT ( 'NONE',  ( 10.77406844824080068, 1422.341328632539899, 209.8534941415630044 ) ) ;
#28540=CARTESIAN_POINT ( 'NONE',  ( 11.37862535051929846, 1491.234308450049866, 207.8509436897950025 ) ) ;
#28548=CARTESIAN_POINT ( 'NONE',  ( 12.04784982253540093, 1427.346391823369913, 208.1256229127970130 ) ) ;
#28551=CARTESIAN_POINT ( 'NONE',  ( 12.45034049356619832, 1421.619540909540092, 207.5029415923690124 ) ) ;
#28566=B_SPLINE_CURVE_WITH_KNOTS ( 'NONE', 3,
 ( #21602, #22692, #38416, #12674, #49052, #64201, #83188, #14309, #48501, #31670, #56892, #91023, #106183, #82640, #47389, #106720, #29465, #74257, #30574, #63658, #97773, #55807, #89924, #13199, #81510, #98875, #22141, #84817, #85368, #16497, #94322 ),
 .UNSPECIFIED., .F., .F.,
 ( 4, 3, 3, 3, 3, 3, 3, 3, 3, 3, 4 ),
 ( -7.456423346589999390, -7.344770142544849278, -7.144274285211090536, -6.832125223832170136, -6.600994903882189568, -6.405260161108500050, -6.335246464236609754, -5.648730639708280599, -4.892201118308060259, -4.020974890406479929, -3.062118867579999737 ),
 .UNSPECIFIED. ) ;
#28567=EDGE_CURVE ( 'NONE', #78311, #22689, #94356, .T. ) ;
#28575=CARTESIAN_POINT ( 'NONE',  ( 7.031363022279999875, 1494.605019377190047, 219.3119659920989761 ) ) ;
#28583=CARTESIAN_POINT ( 'NONE',  ( -5.122105890483237722, 1419.728707206990748, 194.5792988059779702 ) ) ;
#28597=ORIENTED_EDGE ( 'NONE', *, *, #6407, .T. ) ;
#28598=ORIENTED_EDGE ( 'NONE', *, *, #39971, .T. ) ;
#28601=CARTESIAN_POINT ( 'NONE',  ( 2.144541734774120023, 1498.044082580750000, 197.8976195832460121 ) ) ;
#28603=CARTESIAN_POINT ( 'NONE',  ( -7.548376016692439627, 1471.189479627299988, 215.9520417340509937 ) ) ;
#28609=CARTESIAN_POINT ( 'NONE',  ( 8.556723711100000074, 1492.088035619889979, 216.2210623239989786 ) ) ;
#28612=CARTESIAN_POINT ( 'NONE',  ( -18.15983708720000323, 1504.845299867989979, 208.9729485910140170 ) ) ;
#28615=CARTESIAN_POINT ( 'NONE',  ( -9.953599203913679361, 1439.570906027390038, 208.2134350005999863 ) ) ;
#28619=VECTOR ( 'NONE', #103309, 1000.000000000000000 ) ;
#28624=LINE ( 'NONE', #46547, #13327 ) ;
#28625=CARTESIAN_POINT ( 'NONE',  ( -16.91019554306700101, 1419.805496799009916, 208.4777216397309871 ) ) ;
#28627=CARTESIAN_POINT ( 'NONE',  ( -16.53125420670000167, 1418.541487540729804, 202.7561987471289910 ) ) ;
#28630=CARTESIAN_POINT ( 'NONE',  ( -6.430337163319999050, 1460.599122871690042, 209.4294524016669925 ) ) ;
#28637=CARTESIAN_POINT ( 'NONE',  ( -15.93611219510135690, 1463.426168696786590, 221.8455668742993225 ) ) ;
#28645=B_SPLINE_SURFACE_WITH_KNOTS ( 'NONE', 5, 1, ( 
 ( #32318, #67589 ),
 ( #41268, #58630 ),
 ( #50239, #37706 ),
 ( #53992, #43902 ),
 ( #36600, #45031 ),
 ( #71907, #27105 ),
 ( #70799, #29298 ),
 ( #45583, #27649 ),
 ( #52869, #61835 ) ),
 .UNSPECIFIED., .F., .F., .F.,
 ( 6, 3, 6 ),
 ( 2, 2 ),
 ( 0.000000000000000000, 3.961384672979999966, 7.908240876339999836 ),
 ( 0.000000000000000000, 14.00000000000000000 ),
 .UNSPECIFIED. ) ;
#28676=EDGE_CURVE ( 'NONE', #97154, #37608, #43613, .T. ) ;
#28681=CARTESIAN_POINT ( 'NONE',  ( -3.873647543780000202, 1495.674801125089971, 219.6259912128990095 ) ) ;
#28684=CARTESIAN_POINT ( 'NONE',  ( -0.3528731710729979820, 1421.448950200250010, 193.6845254781989922 ) ) ;
#28689=CARTESIAN_POINT ( 'NONE',  ( -9.866420828029999868, 1449.262144085689897, 190.8627134521989888 ) ) ;
#28691=CARTESIAN_POINT ( 'NONE',  ( 4.789673499540000101, 1465.867933640490037, 219.0700355186390027 ) ) ;
#28695=CARTESIAN_POINT ( 'NONE',  ( -11.40503451100000021, 1490.739837095889925, 209.6941766733859822 ) ) ;
#28701=CARTESIAN_POINT ( 'NONE',  ( -9.255392140700001491, 1423.205578550119753, 209.4023171091370159 ) ) ;
#28702=CARTESIAN_POINT ( 'NONE',  ( -11.88408465604287656, 1421.854389613024978, 210.6434707533515507 ) ) ;
#28705=VERTEX_POINT ( 'NONE', #97847 ) ;
#28708=CARTESIAN_POINT ( 'NONE',  ( 1.145290945507940084, 1458.110487998910003, 199.6352770989870180 ) ) ;
#28718=CARTESIAN_POINT ( 'NONE',  ( -6.016306044853139134, 1426.646534911480103, 205.6760721705690003 ) ) ;
#28721=CARTESIAN_POINT ( 'NONE',  ( -3.005258425510039633, 1450.300055283400070, 188.5532298547360028 ) ) ;
#28722=CARTESIAN_POINT ( 'NONE',  ( -2.071979039770960096, 1431.299421665210275, 200.9961302677540118 ) ) ;
#28731=CARTESIAN_POINT ( 'NONE',  ( 9.750232545500001180, 1462.891281938590282, 208.5260954797809916 ) ) ;
#28735=B_SPLINE_CURVE_WITH_KNOTS ( 'NONE', 3,
 ( #59891, #16725, #110264, #42511, #32472, #50388 ),
 .UNSPECIFIED., .F., .F.,
 ( 4, 2, 4 ),
 ( 0.000000000000000000, 0.5000000000000000000, 1.000000000000000000 ),
 .UNSPECIFIED. ) ;
#28747=LINE ( 'NONE', #45576, #11608 ) ;
#28748=B_SPLINE_CURVE_WITH_KNOTS ( 'NONE', 3,
 ( #60070, #9630, #43258, #102029, #110449, #51656, #167, #94187, #85795, #51107, #8525, #710, #109901, #1258, #18026, #42701, #92531, #34289, #76857, #52219, #68471, #102573 ),
 .UNSPECIFIED., .F., .F.,
 ( 4, 3, 3, 3, 3, 3, 3, 4 ),
 ( -15.61491491670000009, -14.96471882913919949, -13.64186865260530013, -12.35990197051819983, -12.10144895473209914, -11.03773465448690061, -9.945779857935429291, -9.104900364405690283 ),
 .UNSPECIFIED. ) ;
#28749=CARTESIAN_POINT ( 'NONE',  ( -8.789510382754970763, 1436.967902467539943, 213.5031532571800028 ) ) ;
#28755=CARTESIAN_POINT ( 'NONE',  ( 17.78284146230000218, 1432.724246433989947, 213.5810953123289835 ) ) ;
#28763=CARTESIAN_POINT ( 'NONE',  ( -3.283955654634000076, 1483.490552537069789, 198.9754571030750014 ) ) ;
#28765=ORIENTED_EDGE ( 'NONE', *, *, #7765, .F. ) ;
#28771=CARTESIAN_POINT ( 'NONE',  ( -14.42895189880000117, 1415.865101995610075, 203.8800253788289751 ) ) ;
#28778=CARTESIAN_POINT ( 'NONE',  ( -8.736970513497151813, 1448.822091765960067, 211.8396115544819907 ) ) ;
#28784=CARTESIAN_POINT ( 'NONE',  ( -0.008453540501490530365, 1515.389376838289991, 213.4149486290589834 ) ) ;
#28787=B_SPLINE_CURVE_WITH_KNOTS ( 'NONE', 3,
 ( #17457, #58407, #51657, #42702, #51109, #6882, #85233, #100923, #41036, #75215, #16360, #109902, #60072, #24758, #93625, #15800, #84138, #7438, #8526, #59513, #50559, #67921, #76858, #25869, #33182, #67372 ),
 .UNSPECIFIED., .F., .F.,
 ( 4, 2, 1, 1, 1, 1, 1, 2, 2, 2, 2, 1, 1, 1, 2, 2, 4 ),
 ( 0.000000000000000000, 0.1249999999996812827, 0.1874999999995336231, 0.2187499999994684807, 0.2343749999994343414, 0.2421874999993992028, 0.2460937499993816058, 0.2480468749993638977, 0.2499999999993462174, 0.3749999999998965827, 0.4375000000001806888, 0.4687500000003306244, 0.4843750000004123923, 0.4921875000004532485, 0.4960937500004726219, 0.5000000000004920508, 1.000000000000000000 ),
 .UNSPECIFIED. ) ;
#28790=B_SPLINE_CURVE_WITH_KNOTS ( 'NONE', 5,
 ( #67142, #48127, #32952, #100168, #14494, #75541 ),
 .UNSPECIFIED., .F., .F.,
 ( 6, 6 ),
 ( 0.000000000000000000, 1.000000000000000000 ),
 .UNSPECIFIED. ) ;
#28794=CARTESIAN_POINT ( 'NONE',  ( 0.6956281545320009974, 1431.241352936390058, 200.3845806967489978 ) ) ;
#28796=CARTESIAN_POINT ( 'NONE',  ( 1.946416182649999937, 1507.064669603390030, 220.8001475467989962 ) ) ;
#28797=CARTESIAN_POINT ( 'NONE',  ( -4.290508147089998836, 1515.379315998089851, 209.1218459616989946 ) ) ;
#28799=AXIS2_PLACEMENT_3D ( 'NONE', #93886, #23917, #68183 ) ;
#28802=CARTESIAN_POINT ( 'NONE',  ( 10.12295999200579999, 1469.488668891520092, 206.2402591453380012 ) ) ;
#28809=CARTESIAN_POINT ( 'NONE',  ( -8.899263831619999010, 1482.224852125390044, 203.1955085269790118 ) ) ;
#28813=VECTOR ( 'NONE', #93606, 1000.000000000000000 ) ;
#28820=CARTESIAN_POINT ( 'NONE',  ( -15.59907717326891330, 1415.960253477549941, 208.0471002303526689 ) ) ;
#28827=CARTESIAN_POINT ( 'NONE',  ( 7.916532357550000398, 1425.151355441629903, 211.5881757975789981 ) ) ;
#28841=CARTESIAN_POINT ( 'NONE',  ( -1.732266665236295466, 1442.302600356889116, 200.4062168750837145 ) ) ;
#28871=CARTESIAN_POINT ( 'NONE',  ( -12.23489732466240021, 1490.237667237379810, 209.6383001084460034 ) ) ;
#28876=CARTESIAN_POINT ( 'NONE',  ( 0.000000000000000000, 1512.051704408390151, 209.1218459616989946 ) ) ;
#28877=CARTESIAN_POINT ( 'NONE',  ( 3.346707516019999940, 1443.005054410889898, 217.3642451189890323 ) ) ;
#28886=CARTESIAN_POINT ( 'NONE',  ( 16.50820735058650257, 1494.476772471000004, 193.0249898974809923 ) ) ;
#28897=CARTESIAN_POINT ( 'NONE',  ( -3.209303788360000187, 1428.804527045590021, 200.3203052568389921 ) ) ;
#28906=CARTESIAN_POINT ( 'NONE',  ( 10.02037163873229986, 1469.310947271520035, 208.3108194760559968 ) ) ;
#28907=ORIENTED_EDGE ( 'NONE', *, *, #72168, .T. ) ;
#28909=CYLINDRICAL_SURFACE ( 'NONE', #83842, 0.5000000000000022204 ) ;
#28918=CARTESIAN_POINT ( 'NONE',  ( -0.09849533087990110236, 1444.626931724390033, 218.0966844286490129 ) ) ;
#28923=CARTESIAN_POINT ( 'NONE',  ( -4.643169496351990055, 1464.538216081999963, 199.1279085030210183 ) ) ;
#28930=CARTESIAN_POINT ( 'NONE',  ( -9.420366384649998537, 1508.551704410389902, 218.6205651585790122 ) ) ;
#28938=( GEOMETRIC_REPRESENTATION_CONTEXT ( 3 ) GLOBAL_UNCERTAINTY_ASSIGNED_CONTEXT ( ( #27808 ) ) GLOBAL_UNIT_ASSIGNED_CONTEXT ( ( #24282, #67431, #34900 ) ) REPRESENTATION_CONTEXT ( 'NONE', 'WORKASPACE' ) );
#28942=CARTESIAN_POINT ( 'NONE',  ( -10.07725390801599907, 1490.597947965959975, 213.5248140628600027 ) ) ;
#28943=CARTESIAN_POINT ( 'NONE',  ( 20.33642835536319993, 1475.138372969219972, 218.0161211975080278 ) ) ;
#28946=CARTESIAN_POINT ( 'NONE',  ( 8.454779184179999518, 1428.363642554090120, 213.4110050395389919 ) ) ;
#28952=ORIENTED_EDGE ( 'NONE', *, *, #52749, .F. ) ;
#28953=CARTESIAN_POINT ( 'NONE',  ( -20.52849295349999892, 1487.269269018690011, 206.0837407197489881 ) ) ;
#28955=CARTESIAN_POINT ( 'NONE',  ( 4.780307568339999591, 1467.625956517089890, 217.8721402715589761 ) ) ;
#28958=CARTESIAN_POINT ( 'NONE',  ( 8.631804350130249048, 1438.018828263250043, 210.0183207127990102 ) ) ;
#28965=CARTESIAN_POINT ( 'NONE',  ( -0.4426438243505830261, 1515.147163425719782, 213.4491377890840056 ) ) ;
#28969=EDGE_CURVE ( 'NONE', #58146, #94338, #88639, .T. ) ;
#28970=CARTESIAN_POINT ( 'NONE',  ( 1.784426211945118412, 1474.496765829112519, 219.6664114916495691 ) ) ;
#28973=CARTESIAN_POINT ( 'NONE',  ( -12.40530867719999897, 1506.963233163389987, 209.0163269402000026 ) ) ;
#28975=CARTESIAN_POINT ( 'NONE',  ( 16.60194679285929809, 1493.289934017370115, 193.2049637902070174 ) ) ;
#28981=CARTESIAN_POINT ( 'NONE',  ( 4.328122124485929589, 1515.115455661490159, 210.0391460303160045 ) ) ;
#28986=EDGE_LOOP ( 'NONE', ( #2796, #77479, #47513, #78232 ) ) ;
#28988=ORIENTED_EDGE ( 'NONE', *, *, #45020, .F. ) ;
#28995=CARTESIAN_POINT ( 'NONE',  ( 0.3312367761006819733, 1496.117391023140044, 221.4620161682219930 ) ) ;
#28996=ORIENTED_EDGE ( 'NONE', *, *, #32906, .F. ) ;
#29002=CARTESIAN_POINT ( 'NONE',  ( 6.665264545140000330, 1472.962710687689878, 217.4318328743790119 ) ) ;
#29003=CARTESIAN_POINT ( 'NONE',  ( -8.178320334364201472, 1439.186072014569845, 206.0664576276559785 ) ) ;
#29007=CARTESIAN_POINT ( 'NONE',  ( 8.650215806398520613, 1435.966538205339930, 207.8981607294979881 ) ) ;
#29010=ORIENTED_EDGE ( 'NONE', *, *, #17348, .T. ) ;
#29023=ORIENTED_EDGE ( 'NONE', *, *, #102194, .T. ) ;
#29024=CARTESIAN_POINT ( 'NONE',  ( -4.682234856550000046, 1438.893385222290135, 227.1256850459990062 ) ) ;
#29026=ORIENTED_EDGE ( 'NONE', *, *, #87183, .T. ) ;
#29037=DIRECTION ( 'NONE',  ( 0.2046277826698074953, 0.9081497821047129770, -0.3652279340669334906 ) ) ;
#29038=ADVANCED_FACE ( 'NONE', ( #86427 ), #95659, .T. ) ;
#29043=CARTESIAN_POINT ( 'NONE',  ( -17.43298349350000009, 1417.731752926339823, 206.9848508551290251 ) ) ;
#29044=CARTESIAN_POINT ( 'NONE',  ( 2.792568477009999661, 1462.433237919889962, 228.6456570646990087 ) ) ;
#29056=CARTESIAN_POINT ( 'NONE',  ( 11.35984264028680002, 1500.240320957290123, 205.8139343689259988 ) ) ;
#29058=EDGE_CURVE ( 'NONE', #108309, #9292, #61798, .T. ) ;
#29062=CARTESIAN_POINT ( 'NONE',  ( -0.9617952840779990797, 1442.613780569990013, 200.2933273620589887 ) ) ;
#29063=CARTESIAN_POINT ( 'NONE',  ( -4.980815112767512431, 1491.198183695671787, 188.8376021758186027 ) ) ;
#29066=CARTESIAN_POINT ( 'NONE',  ( -16.45294080079732879, 1420.118435820799732, 208.7595929061371578 ) ) ;
#29079=CARTESIAN_POINT ( 'NONE',  ( -4.354842003205010137, 1481.954780407009821, 231.1149995741479870 ) ) ;
#29085=CARTESIAN_POINT ( 'NONE',  ( -0.2725765502280009800, 1430.103961438589977, 217.4715266419189845 ) ) ;
#29086=CARTESIAN_POINT ( 'NONE',  ( -10.19055345377419997, 1472.389342895980008, 207.1730495706439967 ) ) ;
#29092=CARTESIAN_POINT ( 'NONE',  ( 11.28832168721960016, 1491.057081966879878, 207.3180782202140051 ) ) ;
#29097=CARTESIAN_POINT ( 'NONE',  ( -3.049988319169830042, 1495.700618439620030, 197.1733382635540011 ) ) ;
#29110=CARTESIAN_POINT ( 'NONE',  ( -7.799115399243870428, 1493.006526667940079, 207.9966609151059913 ) ) ;
#29117=( BOUNDED_CURVE ( )  B_SPLINE_CURVE ( 3, ( #78959, #71125, #60502, #36380 ),
 .UNSPECIFIED., .F., .F. ) 
 B_SPLINE_CURVE_WITH_KNOTS ( ( 4, 4 ),
 ( 4.156210927873500438, 5.268567114269190554 ),
 .UNSPECIFIED. ) 
 CURVE ( )  GEOMETRIC_REPRESENTATION_ITEM ( )  RATIONAL_B_SPLINE_CURVE ( ( 1.000000000000000000, 0.8995193748706308279, 0.8995193748706308279, 1.000000000000000000 ) ) 
 REPRESENTATION_ITEM ( '' )  );
#29120=CARTESIAN_POINT ( 'NONE',  ( 2.033801735519999987, 1486.167426692489926, 219.8516060156989909 ) ) ;
#29121=CARTESIAN_POINT ( 'NONE',  ( 11.26937793039999924, 1478.652698499990038, 205.8601898034189901 ) ) ;
#29124=CARTESIAN_POINT ( 'NONE',  ( 9.796230887720000169, 1493.843361169789887, 216.7872332751290116 ) ) ;
#29130=CARTESIAN_POINT ( 'NONE',  ( 6.434481945890000887, 1424.403579311469912, 194.2120374376990242 ) ) ;
#29137=EDGE_LOOP ( 'NONE', ( #35531, #65068, #30212, #35840 ) ) ;
#29144=ORIENTED_EDGE ( 'NONE', *, *, #45494, .T. ) ;
#29151=EDGE_CURVE ( 'NONE', #21797, #12639, #82441, .T. ) ;
#29152=CARTESIAN_POINT ( 'NONE',  ( -3.225889381169420034, 1508.257277731970134, 220.7239406431660029 ) ) ;
#29153=CARTESIAN_POINT ( 'NONE',  ( 18.29188182340000068, 1431.768652859389704, 209.1218459616989946 ) ) ;
#29154=CARTESIAN_POINT ( 'NONE',  ( -8.425552351598220469, 1471.460212197980127, 214.8702615395930025 ) ) ;
#29157=CARTESIAN_POINT ( 'NONE',  ( -2.712002233883790137, 1476.204657457879875, 220.2613469579490015 ) ) ;
#29161=CARTESIAN_POINT ( 'NONE',  ( -12.72512470610000079, 1502.960342028389960, 208.6669139330979874 ) ) ;
#29171=EDGE_CURVE ( 'NONE', #84750, #78311, #60883, .T. ) ;
#29174=CARTESIAN_POINT ( 'NONE',  ( -15.10325504049999878, 1415.737031090589880, 211.5641457255090359 ) ) ;
#29180=CARTESIAN_POINT ( 'NONE',  ( -1.189564560608550092, 1429.854023961810071, 199.8020812351830102 ) ) ;
#29187=CARTESIAN_POINT ( 'NONE',  ( 9.837386292569160418, 1469.761137999260200, 211.2461267937810305 ) ) ;
#29198=CARTESIAN_POINT ( 'NONE',  ( -14.49162069865310087, 1417.292349856110150, 203.2575443744490258 ) ) ;
#29204=CARTESIAN_POINT ( 'NONE',  ( -4.261736551909999449, 1515.372048949689997, 207.2788837304390199 ) ) ;
#29212=FACE_OUTER_BOUND ( 'NONE', #38640, .T. ) ;
#29214=CARTESIAN_POINT ( 'NONE',  ( 17.74170650421104511, 1432.761001460916759, 213.7496100754616180 ) ) ;
#29232=CARTESIAN_POINT ( 'NONE',  ( -2.022208241610000012, 1421.024495610020040, 193.8502730733989949 ) ) ;
#29235=CARTESIAN_POINT ( 'NONE',  ( 1.046130468810000158, 1463.550315089890091, 230.5479457569989847 ) ) ;
#29245=CARTESIAN_POINT ( 'NONE',  ( -13.34370645066865713, 1422.266645666820523, 196.3187566567426359 ) ) ;
#29247=CARTESIAN_POINT ( 'NONE',  ( 7163.889423669126700, 5182.767774292100512, -7818.362407857699509 ) ) ;
#29248=CARTESIAN_POINT ( 'NONE',  ( -11.07527852154495385, 1422.183102189465899, 210.6367496950426244 ) ) ;
#29253=ORIENTED_EDGE ( 'NONE', *, *, #72026, .T. ) ;
#29261=CARTESIAN_POINT ( 'NONE',  ( 10.24022436676090031, 1482.543054787119900, 212.0614503867469978 ) ) ;
#29265=CARTESIAN_POINT ( 'NONE',  ( -20.60448988230000111, 1484.737042837089803, 209.1218459616989946 ) ) ;
#29267=CARTESIAN_POINT ( 'NONE',  ( -16.83568192250000095, 1418.884533543920043, 201.2565368162689765 ) ) ;
#29268=CARTESIAN_POINT ( 'NONE',  ( 10.03186001745409150, 1491.455176020307590, 213.8859670922726650 ) ) ;
#29276=CARTESIAN_POINT ( 'NONE',  ( 9.706405685860000077, 1463.133235100189950, 210.3097023741290172 ) ) ;
#29279=CARTESIAN_POINT ( 'NONE',  ( -1.062448666549999921, 1463.820984688390126, 199.3576882633090008 ) ) ;
#29287=ORIENTED_EDGE ( 'NONE', *, *, #65339, .T. ) ;
#29290=CARTESIAN_POINT ( 'NONE',  ( -17.36568713798484609, 1508.455955994650367, 212.8023812719880254 ) ) ;
#29293=CARTESIAN_POINT ( 'NONE',  ( -7.530771855114540614, 1435.872963818640073, 215.3039292562540084 ) ) ;
#29296=CARTESIAN_POINT ( 'NONE',  ( -7.617720993269999852, 1508.534261654589955, 219.3295389908989819 ) ) ;
#29298=CARTESIAN_POINT ( 'NONE',  ( 3.184944912390000216, 1492.459204846589955, 188.3860389383989968 ) ) ;
#29312=CARTESIAN_POINT ( 'NONE',  ( -11.28980188229558657, 1489.194859813259427, 213.7481022665220678 ) ) ;
#29313=CARTESIAN_POINT ( 'NONE',  ( -15.33967589549999921, 1415.677402202029953, 209.0176008730730075 ) ) ;
#29318=CARTESIAN_POINT ( 'NONE',  ( -9.258624140391589208, 1449.585829297850069, 207.9796510681429709 ) ) ;
#29323=CARTESIAN_POINT ( 'NONE',  ( 1.460285906039999970, 1515.203804957989860, 213.4476545592490027 ) ) ;
#29325=CARTESIAN_POINT ( 'NONE',  ( 1.662080245303283021, 1464.065906623968203, 199.4475712355095425 ) ) ;
#29327=CARTESIAN_POINT ( 'NONE',  ( -9.915381109698630624, 1446.894009479360193, 211.9680447833129904 ) ) ;
#29336=CARTESIAN_POINT ( 'NONE',  ( 10.10666311268190043, 1469.215464056610017, 203.9609526372169910 ) ) ;
#29344=CARTESIAN_POINT ( 'NONE',  ( 12.19805618840440076, 1491.617858633879905, 207.5154424382099876 ) ) ;
#29350=ORIENTED_EDGE ( 'NONE', *, *, #19123, .F. ) ;
#29353=CARTESIAN_POINT ( 'NONE',  ( -3.677613769069999778E-16, 1378.413060387289988, 209.1218459616989946 ) ) ;
#29359=CARTESIAN_POINT ( 'NONE',  ( 7.300163574239999065, 1426.919040555409993, 212.8503364413490146 ) ) ;
#29367=B_SPLINE_CURVE_WITH_KNOTS ( 'NONE', 3,
 ( #77125, #91287, #95017, #99667, #48758, #86061, #43521, #42397, #60891, #8784, #52479, #18285, #6176, #68733, #59772, #8230, #86607, #44070, #40329 ),
 .UNSPECIFIED., .F., .F.,
 ( 4, 2, 2, 2, 1, 1, 1, 2, 2, 2, 4 ),
 ( 0.000000000000000000, 0.2499999999994982902, 0.3749999999992473243, 0.4374999999991323052, 0.4687499999990772936, 0.4843749999990471511, 0.4921874999990320521, 0.4960937499990347166, 0.4999999999990373256, 0.7499999999995186073, 1.000000000000000000 ),
 .UNSPECIFIED. ) ;
#29374=CARTESIAN_POINT ( 'NONE',  ( -21.52163278259530088, 1505.754112708010098, 209.2478060993030056 ) ) ;
#29387=ORIENTED_EDGE ( 'NONE', *, *, #83127, .F. ) ;
#29399=CARTESIAN_POINT ( 'NONE',  ( -12.12929454590999967, 1489.942571554460073, 210.7157588992720321 ) ) ;
#29406=B_SPLINE_CURVE_WITH_KNOTS ( 'NONE', 5,
 ( #95384, #86973, #10264, #19193, #71883, #37679 ),
 .UNSPECIFIED., .F., .F.,
 ( 6, 6 ),
 ( 0.000000000000000000, 1.000000000000000000 ),
 .UNSPECIFIED. ) ;
#29420=( BOUNDED_CURVE ( )  B_SPLINE_CURVE ( 3, ( #41981, #76131, #110272, #43088 ),
 .UNSPECIFIED., .F., .T. ) 
 B_SPLINE_CURVE_WITH_KNOTS ( ( 4, 4 ),
 ( 1.309525232983709930, 2.739590174588970140 ),
 .UNSPECIFIED. ) 
 CURVE ( )  GEOMETRIC_REPRESENTATION_ITEM ( )  RATIONAL_B_SPLINE_CURVE ( ( 1.000000000000000000, 0.8367146349265004446, 0.8367146349265004446, 1.000000000000000000 ) ) 
 REPRESENTATION_ITEM ( '' )  );
#29426=ORIENTED_EDGE ( 'NONE', *, *, #2116, .T. ) ;
#29428=CARTESIAN_POINT ( 'NONE',  ( -4.487249770485409961, 1509.038615931769982, 206.6339108289169815 ) ) ;
#29432=CARTESIAN_POINT ( 'NONE',  ( -4.442976950240000278, 1500.747712884389784, 229.9760442845989985 ) ) ;
#29438=CARTESIAN_POINT ( 'NONE',  ( 10.03880117160240104, 1469.015768458370076, 208.9124404369970023 ) ) ;
#29441=CARTESIAN_POINT ( 'NONE',  ( 10.52837420263239920, 1481.199010226290284, 208.2608686310830137 ) ) ;
#29445=CARTESIAN_POINT ( 'NONE',  ( 8.383305398618512427, 1424.402938891004396, 195.8285644112468447 ) ) ;
#29448=CARTESIAN_POINT ( 'NONE',  ( 2.552069496900000178, 1442.069545149990063, 217.9835893629989982 ) ) ;
#29454=CARTESIAN_POINT ( 'NONE',  ( -3.623165609177270152, 1464.721259246360205, 198.7228523319660098 ) ) ;
#29459=ORIENTED_EDGE ( 'NONE', *, *, #54906, .F. ) ;
#29461=CARTESIAN_POINT ( 'NONE',  ( -13.06308345429999918, 1508.551704408389924, 216.6557220756489812 ) ) ;
#29465=CARTESIAN_POINT ( 'NONE',  ( 11.26595443788370154, 1470.492046862490042, 207.5653086360470070 ) ) ;
#29467=CARTESIAN_POINT ( 'NONE',  ( -15.62861149524349891, 1418.244676918490086, 203.0179538217920197 ) ) ;
#29470=B_SPLINE_SURFACE_WITH_KNOTS ( 'NONE', 5, 5, ( 
 ( #19768, #45006, #43880, #52848, #86423, #104886 ),
 ( #61811, #9713, #28177, #95933, #78024, #62363 ),
 ( #28731, #62936, #36577, #70775, #18103, #2461 ),
 ( #86975, #46108, #10265, #1901, #44441, #19194 ),
 ( #82826, #92881, #16158, #66615, #37680, #101255 ),
 ( #91232, #15053, #106000, #108587, #100718, #80238 ),
 ( #108024, #67157, #92324, #6674, #91775, #83931 ),
 ( #71884, #29276, #24554, #63468, #14512, #49250 ),
 ( #31873, #24000, #3557, #58742, #31321, #97587 ) ),
 .UNSPECIFIED., .F., .F., .F.,
 ( 6, 3, 6 ),
 ( 6, 6 ),
 ( 3.085444082959999612, 5.308104825929999215, 7.530765568899999707 ),
 ( 0.000000000000000000, 2.000000000000000000 ),
 .UNSPECIFIED. ) ;
#29472=CARTESIAN_POINT ( 'NONE',  ( 4.524905829305170712, 1494.978413301719911, 220.1958960354820078 ) ) ;
#29473=CARTESIAN_POINT ( 'NONE',  ( 20.56230369369999877, 1477.111288992490017, 217.7195332328089989 ) ) ;
#29477=CARTESIAN_POINT ( 'NONE',  ( 2.828342949539999651, 1493.511444851789975, 217.0450404263189910 ) ) ;
#29478=ORIENTED_EDGE ( 'NONE', *, *, #81740, .T. ) ;
#29481=ORIENTED_EDGE ( 'NONE', *, *, #15810, .T. ) ;
#29482=ORIENTED_EDGE ( 'NONE', *, *, #73247, .F. ) ;
#29489=CARTESIAN_POINT ( 'NONE',  ( 8.647870999238421064, 1437.913672787270116, 209.8191767245930066 ) ) ;
#29497=CARTESIAN_POINT ( 'NONE',  ( 0.3081309748295429918, 1515.153045852129935, 213.4489837523270239 ) ) ;
#29499=CARTESIAN_POINT ( 'NONE',  ( -8.683283342131749905, 1478.809903676939939, 216.8972849895139916 ) ) ;
#29504=CARTESIAN_POINT ( 'NONE',  ( -11.46284668979999921, 1503.757050468389934, 207.6153425473289929 ) ) ;
#29507=CARTESIAN_POINT ( 'NONE',  ( -21.51493310030000217, 1488.287434706290014, 202.1454994110590064 ) ) ;
#29521=ORIENTED_EDGE ( 'NONE', *, *, #11777, .T. ) ;
#29524=EDGE_LOOP ( 'NONE', ( #12332, #55487, #65515, #20643 ) ) ;
#29527=CARTESIAN_POINT ( 'NONE',  ( -9.533255814881970380, 1446.965757609550110, 212.1719659162569940 ) ) ;
#29542=CARTESIAN_POINT ( 'NONE',  ( 8.931424042116880457, 1435.562258453619961, 207.9893077555419723 ) ) ;
#29545=VERTEX_POINT ( 'NONE', #63864 ) ;
#29548=CARTESIAN_POINT ( 'NONE',  ( 11.21674625111110046, 1471.567453512700240, 211.3061429236929882 ) ) ;
#29551=EDGE_CURVE ( 'NONE', #76640, #91618, #27543, .T. ) ;
#29561=ORIENTED_EDGE ( 'NONE', *, *, #42858, .F. ) ;
#29565=CARTESIAN_POINT ( 'NONE',  ( -9.018403443429999555, 1415.839591758850020, 205.4133982750190057 ) ) ;
#29574=CARTESIAN_POINT ( 'NONE',  ( -17.54173488089999822, 1417.696455080029864, 206.2934839100489910 ) ) ;
#29596=CARTESIAN_POINT ( 'NONE',  ( -10.47547176029999960, 1491.367109134090015, 212.5025952234090028 ) ) ;
#29600=CARTESIAN_POINT ( 'NONE',  ( -21.46486174681220049, 1504.440211022489848, 215.6677628791860286 ) ) ;
#29602=CARTESIAN_POINT ( 'NONE',  ( -11.61854873712450065, 1501.724215307040140, 208.7855428323910019 ) ) ;
#29610=CARTESIAN_POINT ( 'NONE',  ( 4.271224532216500336, 1508.551704408389924, 204.8816808314769844 ) ) ;
#29613=CARTESIAN_POINT ( 'NONE',  ( -19.73708167012179970, 1467.795432308010049, 204.3773359938460032 ) ) ;
#29618=DIRECTION ( 'NONE',  ( -0.9049609225110241129, -0.3874052256307211062, 0.1759628366502599961 ) ) ;
#29619=ADVANCED_FACE ( 'NONE', ( #48158 ), #79616, .T. ) ;
#29622=CARTESIAN_POINT ( 'NONE',  ( 4.639337580630000346, 1465.928856497889910, 219.1434977748990036 ) ) ;
#29629=CARTESIAN_POINT ( 'NONE',  ( 11.77882348100120069, 1491.514007103689892, 207.7369858202129933 ) ) ;
#29631=ORIENTED_EDGE ( 'NONE', *, *, #90099, .F. ) ;
#29635=CARTESIAN_POINT ( 'NONE',  ( 1.723570287401249956, 1496.958110707269952, 196.8512198874990133 ) ) ;
#29637=CARTESIAN_POINT ( 'NONE',  ( 12.85540944714700018, 1420.911466006700039, 202.8798040533630171 ) ) ;
#29651=CARTESIAN_POINT ( 'NONE',  ( 1.316858285199999923, 1498.792501773990125, 197.8475787186989976 ) ) ;
#29652=CARTESIAN_POINT ( 'NONE',  ( -7.245822883755549171, 1494.393323836579839, 205.4491147294489792 ) ) ;
#29653=EDGE_CURVE ( 'NONE', #13254, #88852, #92976, .T. ) ;
#29655=ORIENTED_EDGE ( 'NONE', *, *, #8571, .F. ) ;
#29663=CARTESIAN_POINT ( 'NONE',  ( 0.8530558503729990250, 1485.832915321789869, 220.6087224736990038 ) ) ;
#29674=ORIENTED_EDGE ( 'NONE', *, *, #55600, .T. ) ;
#29675=CARTESIAN_POINT ( 'NONE',  ( -1.479980094498569931, 1442.001091641500125, 203.0964119015820017 ) ) ;
#29694=CARTESIAN_POINT ( 'NONE',  ( 2.257484783599780442, 1497.637221951559923, 197.6769359036259743 ) ) ;
#29695=CARTESIAN_POINT ( 'NONE',  ( -9.558539228608021077, 1469.579548421909976, 215.2843844815280079 ) ) ;
#29696=B_SPLINE_CURVE_WITH_KNOTS ( 'NONE', 3,
 ( #38819, #100387, #66270, #22541, #108234, #57317, #23672, #13599, #83574, #79877, #91444, #98729, #74652, #23113, #6867, #65701 ),
 .UNSPECIFIED., .F., .F.,
 ( 4, 3, 3, 3, 3, 4 ),
 ( -7.748406663631770108, -7.197925092369000133, -6.190671629245319885, -5.186465823511379192, -4.183578071707561463, -3.182527802580000120 ),
 .UNSPECIFIED. ) ;
#29700=CARTESIAN_POINT ( 'NONE',  ( -6.178279419090149993, 1494.593908523239861, 198.4675342823039728 ) ) ;
#29703=CARTESIAN_POINT ( 'NONE',  ( -18.24261182150000238, 1504.557842952090141, 209.1081479311360170 ) ) ;
#29705=CARTESIAN_POINT ( 'NONE',  ( 11.63005500354680066, 1422.115563547319880, 207.2156999536339868 ) ) ;
#29712=B_SPLINE_CURVE_WITH_KNOTS ( 'NONE', 3,
 ( #10513, #44687, #2143, #9408, #96175, #19450, #53649, #36821, #71011, #45800, #3250, #37376, #71577, #105698, #28981, #14353, #74300, #73750, #90519, #72641, #30622, #12719, #21094, #97815, #13795, #107873, #108431, #39578, #30058, #47435, #55297 ),
 .UNSPECIFIED., .F., .F.,
 ( 4, 3, 3, 3, 3, 3, 3, 3, 3, 3, 4 ),
 ( 2.324858856890000158, 2.629659992665080104, 2.924842189028200146, 3.130565735590880028, 3.432172540380809878, 3.731439316892459779, 4.025646101128260490, 4.318556006019989901, 4.608870341565640238, 4.895817131713270598, 4.991117563570000470 ),
 .UNSPECIFIED. ) ;
#29714=CARTESIAN_POINT ( 'NONE',  ( 4.046802277660000335, 1505.460036802790000, 221.2327940266990254 ) ) ;
#29716=CARTESIAN_POINT ( 'NONE',  ( -16.92376582506389937, 1419.669853879900074, 208.5035371377049955 ) ) ;
#29718=CARTESIAN_POINT ( 'NONE',  ( -17.00797328670000397, 1417.537217351680056, 207.7155449971589860 ) ) ;
#29720=CARTESIAN_POINT ( 'NONE',  ( -16.51698475970000146, 1416.970002106650099, 207.7815561879389747 ) ) ;
#29721=CARTESIAN_POINT ( 'NONE',  ( 0.9458865576463879599, 1430.745089220539967, 199.7241109523880027 ) ) ;
#29724=CARTESIAN_POINT ( 'NONE',  ( 9.357303305019659234, 1435.432409049479929, 208.4554647895430151 ) ) ;
#29733=CARTESIAN_POINT ( 'NONE',  ( -7.469899998879999892, 1491.463634741090118, 211.3946206457289918 ) ) ;
#29741=CARTESIAN_POINT ( 'NONE',  ( -4.175275161990000150, 1515.456650324490056, 207.6382005906990003 ) ) ;
#29750=CARTESIAN_POINT ( 'NONE',  ( -11.05457274329999784, 1492.346892589090203, 209.2220259002270097 ) ) ;
#29752=CARTESIAN_POINT ( 'NONE',  ( -8.724201442159989384, 1437.633719118000045, 210.3032200441300290 ) ) ;
#29753=CARTESIAN_POINT ( 'NONE',  ( -4.992640508427165003, 1391.632012742867346, 214.6223054488346236 ) ) ;
#29755=CARTESIAN_POINT ( 'NONE',  ( -11.86216586729469924, 1481.732520156779856, 209.5386625665159954 ) ) ;
#29756=CARTESIAN_POINT ( 'NONE',  ( 8.000564228190230054, 1425.311446220280004, 211.1882531427259835 ) ) ;
#29760=CARTESIAN_POINT ( 'NONE',  ( -12.02051106306990036, 1491.153688555679992, 206.6632162730240054 ) ) ;
#29761=CARTESIAN_POINT ( 'NONE',  ( -4.986960336344659517, 1508.551704408389924, 206.6058482952879842 ) ) ;
#29776=CARTESIAN_POINT ( 'NONE',  ( -13.16170070989210039, 1468.332209647859827, 191.9366023383940103 ) ) ;
#29790=ORIENTED_EDGE ( 'NONE', *, *, #24089, .F. ) ;
#29791=CARTESIAN_POINT ( 'NONE',  ( 7327.379741814554109, -2339.246371527899555, 11093.44175848640407 ) ) ;
#29792=CARTESIAN_POINT ( 'NONE',  ( -13.59271798984216595, 1421.161248306587140, 210.6331271337394639 ) ) ;
#29796=VERTEX_POINT ( 'NONE', #107911 ) ;
#29799=CARTESIAN_POINT ( 'NONE',  ( -0.4215141012316919733, 1485.982418546980171, 221.0094681181439853 ) ) ;
#29807=CARTESIAN_POINT ( 'NONE',  ( 10.38372441944459901, 1482.290969074429995, 211.4067775984080129 ) ) ;
#29813=CARTESIAN_POINT ( 'NONE',  ( -1.624243150411039949, 1431.539686916680012, 200.8843740557090030 ) ) ;
#29815=ORIENTED_EDGE ( 'NONE', *, *, #1905, .T. ) ;
#29816=EDGE_LOOP ( 'NONE', ( #6264, #61447, #83967, #79508 ) ) ;
#29818=DIRECTION ( 'NONE',  ( -6.505213034913001952E-16, 0.02617694830786544691, 0.9996573249755575929 ) ) ;
#29819=CARTESIAN_POINT ( 'NONE',  ( 12.68801083313210043, 1500.413651417279880, 208.6561539661539939 ) ) ;
#29821=ADVANCED_FACE ( 'NONE', ( #101148 ), #28645, .T. ) ;
#29825=CARTESIAN_POINT ( 'NONE',  ( -1.828147983170000046, 1464.537159857190090, 199.0653224421989762 ) ) ;
#29859=CARTESIAN_POINT ( 'NONE',  ( 7.883259769432120478, 1484.453481079082849, 216.4154215447759952 ) ) ;
#29860=CARTESIAN_POINT ( 'NONE',  ( -15.33402440699999936, 1415.677402176539999, 208.4399661241280057 ) ) ;
#29863=CARTESIAN_POINT ( 'NONE',  ( -17.26825932613299841, 1442.367707598380093, 217.4786320952890151 ) ) ;
#29871=CARTESIAN_POINT ( 'NONE',  ( -0.008839278001780500119, 1515.608558013090033, 213.1832674503789917 ) ) ;
#29873=CARTESIAN_POINT ( 'NONE',  ( -0.7930666024419980031, 1471.115585716789838, 188.9853875966990131 ) ) ;
#29875=CARTESIAN_POINT ( 'NONE',  ( -4.227540919128129460, 1441.218328383909920, 201.3833897788859986 ) ) ;
#29892=CARTESIAN_POINT ( 'NONE',  ( -3.162549882268320012, 1508.551704408389924, 204.2260922363450106 ) ) ;
#29894=EDGE_CURVE ( 'NONE', #46415, #101100, #95727, .T. ) ;
#29896=CARTESIAN_POINT ( 'NONE',  ( -11.38947975027659787, 1501.228585066793357, 208.0670107266517732 ) ) ;
#29903=CARTESIAN_POINT ( 'NONE',  ( -9.269849887880001305, 1450.024127290490014, 206.2237698193690107 ) ) ;
#29905=CARTESIAN_POINT ( 'NONE',  ( 8.192509002470000468, 1427.073616020289819, 211.9190997776489951 ) ) ;
#29926=ADVANCED_FACE ( 'NONE', ( #19791 ), #11656, .T. ) ;
#29939=CARTESIAN_POINT ( 'NONE',  ( -17.44267318540000034, 1419.899571665260055, 205.5533046883089980 ) ) ;
#29940=CARTESIAN_POINT ( 'NONE',  ( -11.39446592756109844, 1470.674086296440009, 209.5209556861319982 ) ) ;
#29945=ORIENTED_EDGE ( 'NONE', *, *, #2868, .T. ) ;
#29946=CARTESIAN_POINT ( 'NONE',  ( -16.73264916879790221, 1508.541854165810037, 213.2276336401049832 ) ) ;
#29949=EDGE_CURVE ( 'NONE', #76707, #3640, #39435, .T. ) ;
#29958=VERTEX_POINT ( 'NONE', #97614 ) ;
#29963=CARTESIAN_POINT ( 'NONE',  ( 9.788141164739998956, 1471.003676181789842, 212.2094840332690069 ) ) ;
#29967=CIRCLE ( 'NONE', #67568, 8.800000000000000711 ) ;
#29970=CARTESIAN_POINT ( 'NONE',  ( 7.950009656035348371, 1425.337175471099954, 192.9554219782069993 ) ) ;
#29978=CARTESIAN_POINT ( 'NONE',  ( -3.132406423129999951, 1429.005220112589996, 200.6955266824789987 ) ) ;
#29980=CARTESIAN_POINT ( 'NONE',  ( 4.491293115488566023, 1508.884207226183435, 206.6339108108618348 ) ) ;
#29982=CARTESIAN_POINT ( 'NONE',  ( 10.78087825220000084, 1423.795965465850031, 203.9512493351290061 ) ) ;
#29987=CARTESIAN_POINT ( 'NONE',  ( 10.23249966253590060, 1470.172983095430254, 209.3814011399140043 ) ) ;
#29994=CARTESIAN_POINT ( 'NONE',  ( 18.21091508359999978, 1429.914989560089907, 210.0150344289870077 ) ) ;
#29995=CARTESIAN_POINT ( 'NONE',  ( 7.571416212307459759, 1423.019345442000031, 195.7264161909869813 ) ) ;
#29996=CARTESIAN_POINT ( 'NONE',  ( 2.906162801440000276, 1443.249005831489967, 217.5410957172989868 ) ) ;
#30000=CARTESIAN_POINT ( 'NONE',  ( 5.255993420997609356, 1486.130296503567479, 199.6624549764852361 ) ) ;
#30008=CARTESIAN_POINT ( 'NONE',  ( -16.32163428129999971, 1508.551704408389924, 213.4489811870489859 ) ) ;
#30012=CARTESIAN_POINT ( 'NONE',  ( -3.994321347890000151, 1485.012103865790095, 198.3399482330989940 ) ) ;
#30018=CARTESIAN_POINT ( 'NONE',  ( -21.47379552819999660, 1487.892728108790152, 202.0847255913190281 ) ) ;
#30019=CARTESIAN_POINT ( 'NONE',  ( -14.49777094512960041, 1415.677402205530143, 205.4885795654869867 ) ) ;
#30021=CARTESIAN_POINT ( 'NONE',  ( 5.055176732809999685, 1428.911752091890094, 215.9094460472589958 ) ) ;
#30023=ORIENTED_EDGE ( 'NONE', *, *, #89234, .F. ) ;
#30028=CARTESIAN_POINT ( 'NONE',  ( -7.841538985989999766, 1492.606015770189970, 208.7602525851700079 ) ) ;
#30033=CARTESIAN_POINT ( 'NONE',  ( 8.716659895241020806, 1437.048749725669950, 210.1866992012669755 ) ) ;
#30039=CARTESIAN_POINT ( 'NONE',  ( 9.120893397559440174, 1464.802252829569852, 212.8346682668349956 ) ) ;
#30042=CARTESIAN_POINT ( 'NONE',  ( 0.5056391278744889473, 1515.143808641159922, 213.4492256370539849 ) ) ;
#30044=CARTESIAN_POINT ( 'NONE',  ( -8.819768609920290103, 1478.884144629650109, 216.7505662143140057 ) ) ;
#30053=CARTESIAN_POINT ( 'NONE',  ( -21.45322466873749789, 1487.695354916500037, 202.0543356184059860 ) ) ;
#30055=CARTESIAN_POINT ( 'NONE',  ( 9.209290677350001175, 1421.000200739789989, 196.8939171836989885 ) ) ;
#30058=CARTESIAN_POINT ( 'NONE',  ( 4.326994892130289649, 1515.158502928330108, 209.1643610636710093 ) ) ;
#30061=CARTESIAN_POINT ( 'NONE',  ( -3.316807713620000264, 1457.277897877190071, 218.1845740658989996 ) ) ;
#30072=FILL_AREA_STYLE_COLOUR ( '', #79422 ) ;
#30086=ORIENTED_EDGE ( 'NONE', *, *, #32618, .F. ) ;
#30088=CARTESIAN_POINT ( 'NONE',  ( -3.076366055149999834, 1424.853903601579987, 191.3970713258989917 ) ) ;
#30089=CARTESIAN_POINT ( 'NONE',  ( 19.21983641119999930, 1456.858306478489794, 206.3357454782189677 ) ) ;
#30094=CARTESIAN_POINT ( 'NONE',  ( 5.456719627610000067, 1455.595244131089885, 218.2350948550090095 ) ) ;
#30101=CARTESIAN_POINT ( 'NONE',  ( -7.514943502936695552, 1426.327996137914170, 205.9160340660706652 ) ) ;
#30103=EDGE_LOOP ( 'NONE', ( #93430, #86946, #42384, #104737 ) ) ;
#30111=FACE_OUTER_BOUND ( 'NONE', #90658, .T. ) ;
#30134=CARTESIAN_POINT ( 'NONE',  ( -10.42483197617790047, 1470.891264593049982, 210.8225716954860047 ) ) ;
#30139=CARTESIAN_POINT ( 'NONE',  ( 12.40037417066400138, 1501.289366441759967, 211.7106409669050038 ) ) ;
#30144=CARTESIAN_POINT ( 'NONE',  ( -4.303235863005570039, 1508.728292324839913, 205.3335050028159969 ) ) ;
#30154=CARTESIAN_POINT ( 'NONE',  ( 2.885329903193750045, 1508.551704408389924, 204.1651163175990007 ) ) ;
#30155=LINE ( 'NONE', #5522, #109136 ) ;
#30157=CARTESIAN_POINT ( 'NONE',  ( -19.58883200382760137, 1465.811229466620034, 204.1485211371180242 ) ) ;
#30162=CARTESIAN_POINT ( 'NONE',  ( -10.76610293753739889, 1461.751116445120033, 211.3389343603909936 ) ) ;
#30165=CARTESIAN_POINT ( 'NONE',  ( -5.819613099869999751, 1462.361531754390171, 201.2907114160189792 ) ) ;
#30170=CARTESIAN_POINT ( 'NONE',  ( 4.637787270109999582, 1462.124489585889933, 228.1829287868989979 ) ) ;
#30180=CARTESIAN_POINT ( 'NONE',  ( -15.30918010269999918, 1420.444122943519915, 211.1786203771790156 ) ) ;
#30187=CARTESIAN_POINT ( 'NONE',  ( -9.109439661327298765, 1447.385667508870029, 211.8713842478840093 ) ) ;
#30192=CARTESIAN_POINT ( 'NONE',  ( -1.531858734065989602E-13, 1515.051704408389924, 205.2922258481490303 ) ) ;
#30193=CARTESIAN_POINT ( 'NONE',  ( 7.526607499040649962, 1425.472659576630122, 212.1966582396349850 ) ) ;
#30194=AXIS2_PLACEMENT_3D ( 'NONE', #82728, #50249, #41822 ) ;
#30195=CARTESIAN_POINT ( 'NONE',  ( -6.415996146495579922, 1495.304407762119808, 203.8734489153730181 ) ) ;
#30203=B_SPLINE_CURVE_WITH_KNOTS ( 'NONE', 5,
 ( #106577, #39372, #99255, #47231, #14712, #107682 ),
 .UNSPECIFIED., .F., .F.,
 ( 6, 6 ),
 ( -2.000000000000000000, 0.000000000000000000 ),
 .UNSPECIFIED. ) ;
#30205=CARTESIAN_POINT ( 'NONE',  ( 1.977078070039999913, 1485.260289170789974, 220.8317664630990294 ) ) ;
#30206=CARTESIAN_POINT ( 'NONE',  ( -4.994775864380000208, 1391.713558696990049, 214.4361776263990009 ) ) ;
#30209=CARTESIAN_POINT ( 'NONE',  ( 8.502412689479999841, 1494.223831056089921, 218.1490364173589853 ) ) ;
#30212=ORIENTED_EDGE ( 'NONE', *, *, #83137, .F. ) ;
#30219=CIRCLE ( 'NONE', #19433, 3.458500000000000352 ) ;
#30227=CARTESIAN_POINT ( 'NONE',  ( -7.211414364699999524, 1427.415731310709816, 205.0259060341190320 ) ) ;
#30230=CARTESIAN_POINT ( 'NONE',  ( 9.695302103464010557, 1481.887598573820014, 215.8648280851800223 ) ) ;
#30231=EDGE_CURVE ( 'NONE', #41801, #25418, #76699, .T. ) ;
#30235=CARTESIAN_POINT ( 'NONE',  ( -11.42573944687380028, 1481.783086644220020, 208.8678723980630139 ) ) ;
#30236=CARTESIAN_POINT ( 'NONE',  ( -2.701523881276569838, 1508.230667595090154, 220.7992134743510064 ) ) ;
#30240=CARTESIAN_POINT ( 'NONE',  ( 12.49185799700000032, 1420.539304375840175, 200.4619042918790228 ) ) ;
#30242=CARTESIAN_POINT ( 'NONE',  ( -6.653371456881099988, 1494.411565237649938, 198.7567593804810144 ) ) ;
#30243=CARTESIAN_POINT ( 'NONE',  ( 11.21925624861339976, 1478.674995329209878, 205.8722235859200111 ) ) ;
#30247=CARTESIAN_POINT ( 'NONE',  ( 12.09770740671049971, 1421.784375224090127, 207.3870252319539986 ) ) ;
#30248=CARTESIAN_POINT ( 'NONE',  ( -9.843485560008819135, 1439.940105572409948, 207.3006424506950225 ) ) ;
#30251=ORIENTED_EDGE ( 'NONE', *, *, #29058, .T. ) ;
#30252=CARTESIAN_POINT ( 'NONE',  ( 12.96503937710000010, 1476.856299447390029, 225.6431713718990011 ) ) ;
#30259=CARTESIAN_POINT ( 'NONE',  ( -15.62936356099999990, 1415.849185049640028, 210.3397193722490215 ) ) ;
#30260=CARTESIAN_POINT ( 'NONE',  ( -17.21782089171700036, 1419.893479116660046, 207.5604823166399910 ) ) ;
#30261=EDGE_LOOP ( 'NONE', ( #22116, #36918, #66490, #80621 ) ) ;
#30263=CARTESIAN_POINT ( 'NONE',  ( -16.90409255678397571, 1417.172264864735780, 207.4840029039214357 ) ) ;
#30266=CARTESIAN_POINT ( 'NONE',  ( -7.892061334917592319, 1477.019624418719332, 215.8670058585243794 ) ) ;
#30267=CARTESIAN_POINT ( 'NONE',  ( -19.56156973859999937, 1464.807986927590036, 211.9767427593990021 ) ) ;
#30270=CARTESIAN_POINT ( 'NONE',  ( 6.193779543994120118, 1460.064517498830128, 201.5421853323860262 ) ) ;
#30283=CARTESIAN_POINT ( 'NONE',  ( 0.008608266560750518770, 1515.483924129489878, 204.8869941145489975 ) ) ;
#30284=CARTESIAN_POINT ( 'NONE',  ( -14.70760701499460055, 1417.599750256749985, 203.2440078780049646 ) ) ;
#30290=CARTESIAN_POINT ( 'NONE',  ( 1.988539752888069279, 1484.903804446283630, 198.5396525162173305 ) ) ;
#30296=CARTESIAN_POINT ( 'NONE',  ( 4.757611653739999724, 1476.697157691990014, 198.4937409947989977 ) ) ;
#30298=CARTESIAN_POINT ( 'NONE',  ( -11.15721983490000113, 1491.329444167089832, 209.2379587012340210 ) ) ;
#30305=EDGE_CURVE ( 'NONE', #26067, #100027, #71404, .T. ) ;
#30309=CARTESIAN_POINT ( 'NONE',  ( -12.17471863065270021, 1490.831372364329809, 207.6427668900300034 ) ) ;
#30314=CARTESIAN_POINT ( 'NONE',  ( -3.123993097060000057, 1502.556458247589944, 230.3127639627990106 ) ) ;
#30317=CARTESIAN_POINT ( 'NONE',  ( 9.787859445082000676, 1471.003474910739897, 212.2097121542219895 ) ) ;
#30324=CARTESIAN_POINT ( 'NONE',  ( -18.29499256740350077, 1465.862032733680053, 217.7259485429990207 ) ) ;
#30330=CARTESIAN_POINT ( 'NONE',  ( -8.881784197000000993E-16, 1392.213060387289943, 209.1218459616989946 ) ) ;
#30339=ORIENTED_EDGE ( 'NONE', *, *, #72317, .T. ) ;
#30343=CARTESIAN_POINT ( 'NONE',  ( -2.222806802245810065, 1486.444619701660031, 220.8419180854079968 ) ) ;
#30344=CARTESIAN_POINT ( 'NONE',  ( 12.65031558649999965, 1500.263532149289858, 208.0494375133089875 ) ) ;
#30352=CARTESIAN_POINT ( 'NONE',  ( 10.02771185788900077, 1481.745846822699832, 215.6032939566460129 ) ) ;
#30360=ORIENTED_EDGE ( 'NONE', *, *, #86358, .T. ) ;
#30361=ORIENTED_EDGE ( 'NONE', *, *, #80365, .F. ) ;
#30364=ADVANCED_FACE ( 'NONE', ( #105320 ), #7955, .T. ) ;
#30366=CARTESIAN_POINT ( 'NONE',  ( 12.61145490078909859, 1500.191570443869978, 207.7439650073710027 ) ) ;
#30371=CARTESIAN_POINT ( 'NONE',  ( -1.625943548539999783, 1463.710935416889924, 199.4574233753289718 ) ) ;
#30386=CARTESIAN_POINT ( 'NONE',  ( 20.78707005949999953, 1497.559210495389834, 213.2326338321889807 ) ) ;
#30388=EDGE_CURVE ( 'NONE', #234, #32360, #35921, .T. ) ;
#30389=LINE ( 'NONE', #56151, #35015 ) ;
#30395=B_SPLINE_SURFACE_WITH_KNOTS ( 'NONE', 5, 5, ( 
 ( #10118, #44290, #639, #104180, #94113, #27464 ),
 ( #69507, #93556, #35320, #61652, #103057, #17384 ),
 ( #78434, #76775, #95231, #9011, #103629, #1746 ),
 ( #101955, #42623, #26927, #91, #95779, #35884 ),
 ( #61116, #68955, #85715, #43728, #77881, #34216 ),
 ( #19046, #52140, #16828, #1189, #70068, #86272 ),
 ( #26355, #60551, #51029, #18495, #17944, #53248 ),
 ( #51583, #52691, #86827, #10684, #87389, #44852 ),
 ( #79004, #33650, #67844, #25242, #9558, #85164 ) ),
 .UNSPECIFIED., .F., .F., .F.,
 ( 6, 3, 6 ),
 ( 6, 6 ),
 ( 3.013220511892180209, 5.186741360400000111, 7.360262208917820459 ),
 ( -0.0004429328978235130116, 2.000000000000000000 ),
 .UNSPECIFIED. ) ;
#30397=CARTESIAN_POINT ( 'NONE',  ( -5.788280361890000059, 1452.919697783089987, 200.3898760574089977 ) ) ;
#30401=CARTESIAN_POINT ( 'NONE',  ( 4.324121571198490166, 1515.222544082249897, 212.0786725323009989 ) ) ;
#30410=CARTESIAN_POINT ( 'NONE',  ( -14.50231995610000091, 1415.734965818289993, 204.4815369236590072 ) ) ;
#30420=ORIENTED_EDGE ( 'NONE', *, *, #3458, .T. ) ;
#30423=CARTESIAN_POINT ( 'NONE',  ( 1.485893011569999977, 1515.551703577890066, 213.0284692437889760 ) ) ;
#30429=CARTESIAN_POINT ( 'NONE',  ( -10.03515428011349897, 1447.044425249150208, 211.5514612114130273 ) ) ;
#30434=CARTESIAN_POINT ( 'NONE',  ( -2.252606381920000178, 1507.752798261690032, 221.0168201868989968 ) ) ;
#30442=CARTESIAN_POINT ( 'NONE',  ( -4.660393612750000081, 1436.848553822789881, 227.0391165213990234 ) ) ;
#30448=CARTESIAN_POINT ( 'NONE',  ( 3.116143480280765043, 1509.034509700538138, 213.6092031811108711 ) ) ;
#30449=CARTESIAN_POINT ( 'NONE',  ( 12.33307560294760030, 1492.131889311669966, 209.3605306458800044 ) ) ;
#30458=CARTESIAN_POINT ( 'NONE',  ( -13.59279696885990063, 1508.107997983119958, 209.5096475415970190 ) ) ;
#30463=CARTESIAN_POINT ( 'NONE',  ( -5.516115361319998911, 1453.414288957689905, 201.0820915901090018 ) ) ;
#30466=CARTESIAN_POINT ( 'NONE',  ( 11.57530253392429920, 1501.342159829270031, 208.5271154928819897 ) ) ;
#30467=CARTESIAN_POINT ( 'NONE',  ( 19.12715434829999950, 1496.834837384790035, 222.0421819495990121 ) ) ;
#30473=ORIENTED_EDGE ( 'NONE', *, *, #77232, .T. ) ;
#30480=CARTESIAN_POINT ( 'NONE',  ( 2.329898369991009854, 1515.064791341159889, 204.7923971587090080 ) ) ;
#30496=CARTESIAN_POINT ( 'NONE',  ( -2.795964621609999590, 1422.864594294989956, 191.4386244948990168 ) ) ;
#30503=CARTESIAN_POINT ( 'NONE',  ( -18.44775390838900009, 1508.456898729019940, 211.1927022132439902 ) ) ;
#30511=CARTESIAN_POINT ( 'NONE',  ( -9.051869799378589931, 1451.060085121989914, 207.2134550054099975 ) ) ;
#30520=CARTESIAN_POINT ( 'NONE',  ( 20.72173035919999506, 1494.363728635189773, 205.4654988462689857 ) ) ;
#30542=CARTESIAN_POINT ( 'NONE',  ( 2.615357652070000150, 1499.621979779589992, 230.2633180907990038 ) ) ;
#30543=CARTESIAN_POINT ( 'NONE',  ( 11.53794409400000021, 1426.017383558870051, 204.7551399598289947 ) ) ;
#30552=CARTESIAN_POINT ( 'NONE',  ( 10.24368108368489949, 1480.724658557739986, 206.6208660495449863 ) ) ;
#30553=EDGE_LOOP ( 'NONE', ( #1148, #72651, #80576, #28468 ) ) ;
#30559=CARTESIAN_POINT ( 'NONE',  ( 9.488876987856384559, 1425.357746453355048, 195.5402808110155775 ) ) ;
#30560=CARTESIAN_POINT ( 'NONE',  ( 1.169937655020000022, 1444.094766671090156, 217.9969059596489842 ) ) ;
#30564=CARTESIAN_POINT ( 'NONE',  ( 3.629220049600000220, 1485.493215689190038, 199.0019176958990101 ) ) ;
#30570=ORIENTED_EDGE ( 'NONE', *, *, #55358, .F. ) ;
#30572=CARTESIAN_POINT ( 'NONE',  ( -11.40093083319999856, 1508.517784003389806, 218.0167457774089996 ) ) ;
#30574=CARTESIAN_POINT ( 'NONE',  ( 11.27050504314370016, 1470.501325604160229, 207.5937458527450019 ) ) ;
#30581=CARTESIAN_POINT ( 'NONE',  ( 5.274922050350429714, 1494.803973017990074, 219.8410646961100099 ) ) ;
#30583=CARTESIAN_POINT ( 'NONE',  ( -15.20693464918219995, 1415.677402202029953, 208.3693492345659877 ) ) ;
#30584=CARTESIAN_POINT ( 'NONE',  ( -9.555044808816591129, 1460.091378345289968, 210.4134086466189899 ) ) ;
#30586=ADVANCED_FACE ( 'NONE', ( #41426 ), #99130, .F. ) ;
#30594=CARTESIAN_POINT ( 'NONE',  ( -11.61544799540000028, 1501.735044459389883, 209.3067194099380117 ) ) ;
#30600=B_SPLINE_CURVE_WITH_KNOTS ( 'NONE', 5,
 ( #108979, #101644, #93265, #24932, #94352, #33905 ),
 .UNSPECIFIED., .F., .F.,
 ( 6, 6 ),
 ( 1.920081532330000192E-14, 6.607473203730000577 ),
 .UNSPECIFIED. ) ;
#30602=DIRECTION ( 'NONE',  ( -9.341989762165448955E-47, 1.000000000000000000, -1.836970198721029688E-16 ) ) ;
#30608=CARTESIAN_POINT ( 'NONE',  ( -11.22044638126500082, 1480.603378457079998, 212.7473660371869926 ) ) ;
#30609=CIRCLE ( 'NONE', #27019, 11.23850026409999892 ) ;
#30615=CARTESIAN_POINT ( 'NONE',  ( -11.42745732190000041, 1504.700167813889948, 207.1863490741189935 ) ) ;
#30616=CARTESIAN_POINT ( 'NONE',  ( -18.73651826089999872, 1506.305784642089975, 222.7068728818989882 ) ) ;
#30622=CARTESIAN_POINT ( 'NONE',  ( 4.327392289583150031, 1515.143326931930005, 209.6385377796920011 ) ) ;
#30623=DIRECTION ( 'NONE',  ( 1.224646799147350002E-16, -1.836970198721029688E-16, -1.000000000000000000 ) ) ;
#30625=CARTESIAN_POINT ( 'NONE',  ( 9.932426370723289821, 1468.626893526349932, 207.8384836896190109 ) ) ;
#30626=CARTESIAN_POINT ( 'NONE',  ( -4.244495231940000224, 1458.029848581590159, 218.1181198957289951 ) ) ;
#30629=VERTEX_POINT ( 'NONE', #59346 ) ;
#30648=CARTESIAN_POINT ( 'NONE',  ( -4.848921205238590382, 1489.192137552770191, 188.8958419331429752 ) ) ;
#30654=CARTESIAN_POINT ( 'NONE',  ( -1.157887263654020060, 1425.290045511299695, 191.1461690046699857 ) ) ;
#30659=CARTESIAN_POINT ( 'NONE',  ( 6.013193143143904074, 1460.021089919706810, 201.5886256082018519 ) ) ;
#30661=CARTESIAN_POINT ( 'NONE',  ( 8.762903475094349304, 1437.482247596529760, 212.7253735826240018 ) ) ;
#30665=ORIENTED_EDGE ( 'NONE', *, *, #81740, .F. ) ;
#30680=EDGE_LOOP ( 'NONE', ( #36733, #14259, #47946, #81349 ) ) ;
#30685=CARTESIAN_POINT ( 'NONE',  ( 0.000000000000000000, 1516.051704408390151, 209.1218459616989946 ) ) ;
#30686=CARTESIAN_POINT ( 'NONE',  ( -3.247593561700000020, 1474.689375161690123, 218.8843939287889953 ) ) ;
#30694=CARTESIAN_POINT ( 'NONE',  ( -10.00165394283440001, 1471.801449162250037, 210.9121004031800055 ) ) ;
#30698=CARTESIAN_POINT ( 'NONE',  ( 10.57774485012819810, 1481.435663256220096, 209.0131183278130038 ) ) ;
#30700=VECTOR ( 'NONE', #49758, 1000.000000000000114 ) ;
#30701=CARTESIAN_POINT ( 'NONE',  ( -1.590368490799999979, 1443.733141016789887, 199.9573130278289739 ) ) ;
#30702=CARTESIAN_POINT ( 'NONE',  ( 8.279741772999999583, 1424.453333272249893, 195.9250968994990103 ) ) ;
#30703=CARTESIAN_POINT ( 'NONE',  ( -10.94904004810000053, 1491.926361048389936, 210.5558081329789957 ) ) ;
#30704=CARTESIAN_POINT ( 'NONE',  ( 0.5203691551014211214, 1508.551704408389924, 219.9487978885150028 ) ) ;
#30708=CARTESIAN_POINT ( 'NONE',  ( -11.42597592515710048, 1501.110059307680103, 208.6216570093839948 ) ) ;
#30715=CARTESIAN_POINT ( 'NONE',  ( 4.504070374249360853, 1508.551704408389924, 205.1553644208390210 ) ) ;
#30718=CARTESIAN_POINT ( 'NONE',  ( -13.32685356434600088, 1469.522677642460167, 191.9925945811579879 ) ) ;
#30721=CARTESIAN_POINT ( 'NONE',  ( -3.586321559908030032, 1515.071394777460000, 205.0390677611139836 ) ) ;
#30722=DIRECTION ( 'NONE',  ( -6.922360974429999144E-17, -1.000000000000000000, 2.302693041820029802E-16 ) ) ;
#30723=CARTESIAN_POINT ( 'NONE',  ( -6.138624675819999155, 1464.038710366590067, 200.4690805114690022 ) ) ;
#30724=CARTESIAN_POINT ( 'NONE',  ( -15.20804204212620725, 1420.041555928045000, 212.2965765635398157 ) ) ;
#30725=CARTESIAN_POINT ( 'NONE',  ( 7.654612949109999676, 1489.887860909490200, 207.9968670573389886 ) ) ;
#30729=DIRECTION ( 'NONE',  ( 1.000000000000000000, 0.000000000000000000, 0.000000000000000000 ) ) ;
#30740=CARTESIAN_POINT ( 'NONE',  ( 12.48571605687039998, 1420.624698929089845, 200.8204384990370102 ) ) ;
#30749=CARTESIAN_POINT ( 'NONE',  ( -9.488257380476161629, 1447.075045628219868, 211.9049835964190152 ) ) ;
#30754=CARTESIAN_POINT ( 'NONE',  ( 6.901445711767499880, 1424.875821108860237, 213.3711103352979990 ) ) ;
#30755=ORIENTED_EDGE ( 'NONE', *, *, #64522, .F. ) ;
#30758=CARTESIAN_POINT ( 'NONE',  ( -11.76686801360590096, 1491.289303165600131, 206.7423971511180127 ) ) ;
#30760=EDGE_CURVE ( 'NONE', #45555, #77955, #49141, .T. ) ;
#30765=EDGE_CURVE ( 'NONE', #20110, #3002, #28735, .T. ) ;
#30777=CARTESIAN_POINT ( 'NONE',  ( -8.366077765514660314, 1446.966787759040017, 191.6214120380429904 ) ) ;
#30784=CARTESIAN_POINT ( 'NONE',  ( -7.217365652099999807, 1426.227155235339978, 204.3687986179290021 ) ) ;
#30787=CARTESIAN_POINT ( 'NONE',  ( 5.170554601400000116, 1484.055082523290139, 219.7711189574989703 ) ) ;
#30789=CARTESIAN_POINT ( 'NONE',  ( 3.701853738749347755, 1478.468837479528020, 199.3102443334512657 ) ) ;
#30792=CARTESIAN_POINT ( 'NONE',  ( -11.88168803400450102, 1481.931231228029901, 208.8867617824080014 ) ) ;
#30795=CARTESIAN_POINT ( 'NONE',  ( -10.12185763815729977, 1470.644638848689965, 212.0624009803890146 ) ) ;
#30796=CARTESIAN_POINT ( 'NONE',  ( 12.10295653074440025, 1501.689262389139913, 213.0402934496359819 ) ) ;
#30797=CARTESIAN_POINT ( 'NONE',  ( 11.67962703000000069, 1420.525946465979814, 199.2877884308990133 ) ) ;
#30798=CARTESIAN_POINT ( 'NONE',  ( -1.017302442628150061, 1475.632587704960088, 220.5137673393959972 ) ) ;
#30804=CARTESIAN_POINT ( 'NONE',  ( 12.28210492449239943, 1427.001931710319923, 206.6181840418510092 ) ) ;
#30805=CARTESIAN_POINT ( 'NONE',  ( -9.869059709240291411, 1439.877441815369821, 207.4585820634549975 ) ) ;
#30813=CARTESIAN_POINT ( 'NONE',  ( 19.64599270300000100, 1476.662575758389949, 214.0395835971089866 ) ) ;
#30814=CARTESIAN_POINT ( 'NONE',  ( -16.25293001547770189, 1420.173544245570156, 209.1081125830500014 ) ) ;
#30816=CARTESIAN_POINT ( 'NONE',  ( 1.734314904639999932, 1429.316081142190114, 217.2477305841389921 ) ) ;
#30818=CARTESIAN_POINT ( 'NONE',  ( -17.01462546559999822, 1417.417564138139824, 207.6637930894090118 ) ) ;
#30822=B_SPLINE_CURVE_WITH_KNOTS ( 'NONE', 3,
 ( #34936, #1355, #78046, #86449, #33274, #85895, #101569, #9201, #35495, #26536, #43362, #77508, #18128, #69122, #84777, #8622, #93719, #42798, #52326, #25410, #76958, #16995, #267, #10288, #103809, #60161, #93183, #51195, #16450, #50647, #94282, #102666, #33832, #43905, #85326, #110544, #61293, #95411, #18675, #34392, #17559, #60732, #44466, #8074, #67465, #42244 ),
 .UNSPECIFIED., .F., .F.,
 ( 4, 3, 3, 3, 3, 3, 3, 3, 3, 3, 3, 3, 3, 3, 3, 4 ),
 ( -22.34240630152029894, -22.26676910785790042, -22.11540990129389783, -21.96056640200000132, -21.94306335083159709, -21.76802964484999947, -21.57549288769999762, -21.37216274998920085, -21.15253510981440144, -20.96805652687310229, -20.80534586139999931, -20.76768359745410208, -20.56671237214550274, -20.32807888289099907, -19.85081190438209831, -19.61749528909999896 ),
 .UNSPECIFIED. ) ;
#30824=CARTESIAN_POINT ( 'NONE',  ( 2.506833295396249994, 1457.656460922180031, 199.7250060859690279 ) ) ;
#30825=CARTESIAN_POINT ( 'NONE',  ( 8.093510796512729755, 1424.956611240659868, 194.6959284516389914 ) ) ;
#30836=CARTESIAN_POINT ( 'NONE',  ( -3.005246163384160063, 1450.300006441359983, 188.5532306313729975 ) ) ;
#30844=CARTESIAN_POINT ( 'NONE',  ( -3.244182695775085890, 1430.599155961690030, 201.4114353244786457 ) ) ;
#30849=CARTESIAN_POINT ( 'NONE',  ( -10.94209138219999922, 1492.979990466090157, 207.3926136405989951 ) ) ;
#30851=CARTESIAN_POINT ( 'NONE',  ( 4.617353517619999792, 1460.098150474590057, 228.0971968620989969 ) ) ;
#30854=CARTESIAN_POINT ( 'NONE',  ( -16.64894006880174615, 1482.394100643090269, 222.3169130686996198 ) ) ;
#30858=CARTESIAN_POINT ( 'NONE',  ( -12.20945877950170022, 1490.723361035459902, 207.9880844395189854 ) ) ;
#30866=CARTESIAN_POINT ( 'NONE',  ( 9.740043262020458670, 1470.413801779320011, 211.7848579975940027 ) ) ;
#30873=CARTESIAN_POINT ( 'NONE',  ( -18.32377947901730053, 1464.077717911239915, 217.4721370783159955 ) ) ;
#30876=CARTESIAN_POINT ( 'NONE',  ( 7.287315400159999790, 1481.177127506090073, 208.3645142728410065 ) ) ;
#30891=CARTESIAN_POINT ( 'NONE',  ( 3.394586470828380165, 1484.752177860970050, 220.4731790445629827 ) ) ;
#30893=CARTESIAN_POINT ( 'NONE',  ( 11.97278235750000164, 1500.105384839889894, 206.6109453941589607 ) ) ;
#30902=CARTESIAN_POINT ( 'NONE',  ( 11.20313537261820080, 1480.728593169510077, 212.9248304369289713 ) ) ;
#30908=CARTESIAN_POINT ( 'NONE',  ( 20.56230944797239957, 1477.111339253379811, 217.7195256771020127 ) ) ;
#30909=CARTESIAN_POINT ( 'NONE',  ( -1.838822892484560212, 1431.425781269919980, 200.9354431986780014 ) ) ;
#30914=CYLINDRICAL_SURFACE ( 'NONE', #16952, 2.000000000000007550 ) ;
#30916=CARTESIAN_POINT ( 'NONE',  ( -16.87986946983459546, 1508.249863702309995, 209.5894333877659790 ) ) ;
#30920=CARTESIAN_POINT ( 'NONE',  ( -0.9802168924079989187, 1463.379214693789891, 199.3683684440489685 ) ) ;
#30921=B_SPLINE_CURVE_WITH_KNOTS ( 'NONE', 5,
 ( #99462, #22740, #89432, #81028, #108993, #108434 ),
 .UNSPECIFIED., .F., .F.,
 ( 6, 6 ),
 ( 0.000000000000000000, 1.000000000000000000 ),
 .UNSPECIFIED. ) ;
#30929=B_SPLINE_CURVE_WITH_KNOTS ( 'NONE', 3,
 ( #13111, #89838, #31030, #106096, #47294, #22050, #106635, #29374, #48411, #56801, #63574, #98788 ),
 .UNSPECIFIED., .F., .F.,
 ( 4, 2, 2, 2, 2, 4 ),
 ( 0.000000000000000000, 0.01073386081903290011, 0.02153086504656569894, 0.04175192121145759883, 0.06241451806017900283, 0.08155783388473800133 ),
 .UNSPECIFIED. ) ;
#30934=CARTESIAN_POINT ( 'NONE',  ( -16.70830179842720042, 1417.149226859160080, 207.3570905742490140 ) ) ;
#30936=CARTESIAN_POINT ( 'NONE',  ( -17.92257945210411307, 1508.456862604705293, 212.0064218226281127 ) ) ;
#30937=ADVANCED_FACE ( 'NONE', ( #30111 ), #92889, .T. ) ;
#30939=CARTESIAN_POINT ( 'NONE',  ( -7.399624460160000083, 1435.775033902190216, 215.4503904880270113 ) ) ;
#30955=CARTESIAN_POINT ( 'NONE',  ( 2.329920892869609794, 1515.492270357739926, 213.2601720494629944 ) ) ;
#30957=CARTESIAN_POINT ( 'NONE',  ( -11.60674135321730027, 1507.508082919659955, 207.5537295141489835 ) ) ;
#30962=CARTESIAN_POINT ( 'NONE',  ( -2.351149531359999489, 1431.454776817389984, 214.3229504429189944 ) ) ;
#30963=CARTESIAN_POINT ( 'NONE',  ( -8.138947185354830083, 1440.565483764919918, 204.7812048973189860 ) ) ;
#30964=CARTESIAN_POINT ( 'NONE',  ( -18.84390534926900074, 1444.419481533549970, 208.3496837893860061 ) ) ;
#30965=CARTESIAN_POINT ( 'NONE',  ( -14.45258105951289807, 1415.677402202029953, 212.7925583759839867 ) ) ;
#30966=CARTESIAN_POINT ( 'NONE',  ( -0.3646785447090010179, 1445.165625506690048, 215.3775911874990072 ) ) ;
#30968=CARTESIAN_POINT ( 'NONE',  ( -10.08936239315010042, 1480.949542027630059, 206.0194718485379894 ) ) ;
#30970=ORIENTED_EDGE ( 'NONE', *, *, #3181, .F. ) ;
#30980=CARTESIAN_POINT ( 'NONE',  ( -6.580058596648179936, 1439.972221953270719, 203.3337447694734408 ) ) ;
#30985=CARTESIAN_POINT ( 'NONE',  ( -11.39360664199999995, 1501.071473187889978, 211.1722694393789936 ) ) ;
#31007=CARTESIAN_POINT ( 'NONE',  ( -18.65942492963539934, 1468.219830252329984, 201.0822089472089829 ) ) ;
#31014=CARTESIAN_POINT ( 'NONE',  ( 7.739519778090000024, 1427.631386558690110, 212.7537242539289934 ) ) ;
#31015=CARTESIAN_POINT ( 'NONE',  ( 0.000000000000000000, 1402.913060387289988, 209.1218459616989946 ) ) ;
#31028=CARTESIAN_POINT ( 'NONE',  ( 2.329957323386949941, 1515.551704201149960, 205.2926810894529979 ) ) ;
#31030=CARTESIAN_POINT ( 'NONE',  ( -21.50621374580559930, 1505.483499709200032, 209.5478608782210301 ) ) ;
#31038=ORIENTED_EDGE ( 'NONE', *, *, #33035, .F. ) ;
#31042=EDGE_LOOP ( 'NONE', ( #9845, #97683, #60558, #56239 ) ) ;
#31087=DIRECTION ( 'NONE',  ( -0.000000000000000000, 1.836970198721029688E-16, 1.000000000000000000 ) ) ;
#31090=CARTESIAN_POINT ( 'NONE',  ( 11.36300084380000008, 1422.238049685370015, 206.7577474052189928 ) ) ;
#31095=CARTESIAN_POINT ( 'NONE',  ( -2.926343479570000294, 1461.299900799990155, 228.5762336084989954 ) ) ;
#31096=CARTESIAN_POINT ( 'NONE',  ( -0.3106507924581433655, 1515.598599846415254, 205.0832686031015157 ) ) ;
#31107=CARTESIAN_POINT ( 'NONE',  ( 9.343973014947424716, 1425.273178258202051, 195.5824969410661538 ) ) ;
#31108=CARTESIAN_POINT ( 'NONE',  ( 2.620959656609999744, 1442.441462711689837, 217.7270133417389957 ) ) ;
#31112=CARTESIAN_POINT ( 'NONE',  ( 8.342125760907268983, 1487.569189912864431, 202.1972327929222502 ) ) ;
#31119=CARTESIAN_POINT ( 'NONE',  ( -3.994937574034520100, 1430.106198372560129, 201.8091617894969829 ) ) ;
#31124=AXIS2_PLACEMENT_3D ( 'NONE', #75417, #50215, #1892 ) ;
#31128=CARTESIAN_POINT ( 'NONE',  ( -14.09290554161880138, 1415.677402202029953, 204.2440491414689916 ) ) ;
#31135=ORIENTED_EDGE ( 'NONE', *, *, #81481, .F. ) ;
#31139=CARTESIAN_POINT ( 'NONE',  ( 4.461864229229999701, 1454.855724705989815, 217.5673509250489985 ) ) ;
#31147=CARTESIAN_POINT ( 'NONE',  ( 0.8282867551300300279, 1515.122054816080208, 213.4497952811889832 ) ) ;
#31149=CARTESIAN_POINT ( 'NONE',  ( -6.355761515339399814, 1477.685937564089954, 218.7950034472659979 ) ) ;
#31154=ORIENTED_EDGE ( 'NONE', *, *, #105176, .F. ) ;
#31156=CARTESIAN_POINT ( 'NONE',  ( -18.77469242039999742, 1505.713855622889923, 222.6051356488989938 ) ) ;
#31163=CARTESIAN_POINT ( 'NONE',  ( 18.22204802156040060, 1431.452345132420078, 207.6392317545619903 ) ) ;
#31164=CARTESIAN_POINT ( 'NONE',  ( -3.957900269260000048, 1458.284989000489986, 219.0746905126889885 ) ) ;
#31167=EDGE_CURVE ( 'NONE', #25915, #77692, #87434, .T. ) ;
#31178=CARTESIAN_POINT ( 'NONE',  ( -17.62371441874761047, 1419.748654031750903, 206.8646141850265963 ) ) ;
#31184=ORIENTED_EDGE ( 'NONE', *, *, #73400, .F. ) ;
#31199=CARTESIAN_POINT ( 'NONE',  ( -20.69303424980000372, 1486.764600954290017, 209.1218459616989946 ) ) ;
#31212=ORIENTED_EDGE ( 'NONE', *, *, #51476, .T. ) ;
#31217=VERTEX_POINT ( 'NONE', #33288 ) ;
#31224=CARTESIAN_POINT ( 'NONE',  ( 12.03449221500000199, 1491.353386477190043, 206.6667661068590292 ) ) ;
#31228=CARTESIAN_POINT ( 'NONE',  ( 17.99277867620000038, 1432.534352819589913, 212.7098897757189775 ) ) ;
#31235=CARTESIAN_POINT ( 'NONE',  ( 1.146125081599999929, 1474.496542508589982, 219.7253671311989933 ) ) ;
#31241=CARTESIAN_POINT ( 'NONE',  ( -1.776356839399999804E-15, 1414.661898229710005, 209.1218459616989946 ) ) ;
#31243=CARTESIAN_POINT ( 'NONE',  ( -9.772455935529970716, 1472.076110283059961, 211.9302343523150114 ) ) ;
#31244=CARTESIAN_POINT ( 'NONE',  ( 9.907316696420009450, 1469.648968762289996, 210.8737231108960088 ) ) ;
#31251=CARTESIAN_POINT ( 'NONE',  ( -1.843107666119999877, 1444.183210091189949, 199.2363500995090249 ) ) ;
#31252=CARTESIAN_POINT ( 'NONE',  ( 8.270286460330000367, 1424.455427991309989, 195.9054154081989907 ) ) ;
#31258=CARTESIAN_POINT ( 'NONE',  ( -0.4832821051016459868, 1508.551704408389924, 220.0496842192639804 ) ) ;
#31262=CARTESIAN_POINT ( 'NONE',  ( -12.56112213346830053, 1502.620980619200054, 209.0016574251579868 ) ) ;
#31264=CARTESIAN_POINT ( 'NONE',  ( -3.163820906539999811, 1456.764302747290003, 218.0770706517390067 ) ) ;
#31268=CARTESIAN_POINT ( 'NONE',  ( 4.554659021567319499, 1508.551704408389924, 205.2297450218139829 ) ) ;
#31273=CARTESIAN_POINT ( 'NONE',  ( -3.665756888920000289, 1509.051704408389924, 204.1347675262390169 ) ) ;
#31293=CARTESIAN_POINT ( 'NONE',  ( -15.31114377250000125, 1420.272718699760162, 211.9351904690790036 ) ) ;
#31303=CARTESIAN_POINT ( 'NONE',  ( 6.942384827123182056, 1508.551704408389924, 200.9625026564361292 ) ) ;
#31304=CARTESIAN_POINT ( 'NONE',  ( 7.275136103057380232, 1425.000205421479905, 212.7055067982740013 ) ) ;
#31314=EDGE_CURVE ( 'NONE', #103948, #46147, #79421, .T. ) ;
#31320=DIRECTION ( 'NONE',  ( 0.000000000000000000, -1.836970198721029688E-16, -1.000000000000000000 ) ) ;
#31321=CARTESIAN_POINT ( 'NONE',  ( 10.36617021350000023, 1462.084514122090013, 211.0499682573590121 ) ) ;
#31326=ORIENTED_EDGE ( 'NONE', *, *, #33065, .T. ) ;
#31329=CARTESIAN_POINT ( 'NONE',  ( 2.487923749338929902, 1508.731372610989865, 213.6767948862569995 ) ) ;
#31335=ADVANCED_FACE ( 'NONE', ( #90992 ), #93794, .F. ) ;
#31336=VERTEX_POINT ( 'NONE', #22475 ) ;
#31337=CARTESIAN_POINT ( 'NONE',  ( 11.48584737056929939, 1480.327931592909863, 211.7937108438270002 ) ) ;
#31346=CARTESIAN_POINT ( 'NONE',  ( 8.841553233067839912, 1503.647460366240011, 218.3045275839649833 ) ) ;
#31347=CARTESIAN_POINT ( 'NONE',  ( 9.568810912189999129, 1420.789473812500091, 197.0881969165990029 ) ) ;
#31351=CARTESIAN_POINT ( 'NONE',  ( -5.264762213780000089, 1496.215614374990082, 199.2138355340389921 ) ) ;
#31355=CARTESIAN_POINT ( 'NONE',  ( 11.18609796984200067, 1425.994771849919971, 206.4955550758209881 ) ) ;
#31360=CARTESIAN_POINT ( 'NONE',  ( -17.18283320249707913, 1417.508594224242870, 206.5901238511499400 ) ) ;
#31364=CARTESIAN_POINT ( 'NONE',  ( -15.74296179209999913, 1415.733199231679919, 209.6832678893589730 ) ) ;
#31365=CARTESIAN_POINT ( 'NONE',  ( 11.26951302955830059, 1422.439921091280212, 203.3658004337269745 ) ) ;
#31366=EDGE_LOOP ( 'NONE', ( #74837, #32664, #104506, #103877, #95505 ) ) ;
#31369=CARTESIAN_POINT ( 'NONE',  ( -16.33362175549999762, 1416.748655660220038, 208.2080258544030187 ) ) ;
#31382=CARTESIAN_POINT ( 'NONE',  ( 4.649753459270000278, 1460.482125307190017, 203.9966562023689676 ) ) ;
#31387=CARTESIAN_POINT ( 'NONE',  ( -17.65532977206540011, 1419.497220819440145, 207.2321560918570071 ) ) ;
#31400=CARTESIAN_POINT ( 'NONE',  ( 4.114426077449999219, 1478.089653320190109, 199.4391987246589792 ) ) ;
#31402=CARTESIAN_POINT ( 'NONE',  ( -11.05734857760000089, 1492.520961800689975, 208.6928883350419994 ) ) ;
#31403=CARTESIAN_POINT ( 'NONE',  ( 0.8634109271070009584, 1463.906666237789977, 202.1056695248490200 ) ) ;
#31408=CARTESIAN_POINT ( 'NONE',  ( -12.24666832539229944, 1490.299283743809838, 209.4193319484280096 ) ) ;
#31410=VERTEX_POINT ( 'NONE', #4617 ) ;
#31417=CARTESIAN_POINT ( 'NONE',  ( 9.985337640048900454, 1470.806041673749860, 211.4815898445349944 ) ) ;
#31418=CARTESIAN_POINT ( 'NONE',  ( 17.89866715925209917, 1430.472632720380034, 212.6087062095869840 ) ) ;
#31425=CARTESIAN_POINT ( 'NONE',  ( -9.746793100592970660, 1463.060628619970203, 228.0587242826289867 ) ) ;
#31429=CARTESIAN_POINT ( 'NONE',  ( 6.906779328069999835, 1480.511272950890088, 206.6585084482690036 ) ) ;
#31432=CARTESIAN_POINT ( 'NONE',  ( -13.31089767776890120, 1503.456584347970193, 208.6977459380580058 ) ) ;
#31434=B_SPLINE_CURVE_WITH_KNOTS ( 'NONE', 3,
 ( #9749, #278, #93729, #17008, #77520, #43915, #51207, #49149, #820, #60742, #40728, #85336, #18139, #52882, #52335, #86458 ),
 .UNSPECIFIED., .F., .F.,
 ( 4, 3, 3, 3, 3, 4 ),
 ( -7.874164595100000774, -7.551475176867179506, -6.470576537018629892, -5.390579508517740592, -4.310775221818579972, -3.231130238939999622 ),
 .UNSPECIFIED. ) ;
#31443=CARTESIAN_POINT ( 'NONE',  ( -0.5979661643004559046, 1486.030882971970186, 221.0048940962329880 ) ) ;
#31445=CARTESIAN_POINT ( 'NONE',  ( 11.39601957930000076, 1501.670084141789857, 207.8884637162790057 ) ) ;
#31450=FACE_OUTER_BOUND ( 'NONE', #110584, .T. ) ;
#31451=CARTESIAN_POINT ( 'NONE',  ( 12.45552494207550076, 1501.256435928469955, 211.6864728236859889 ) ) ;
#31453=CARTESIAN_POINT ( 'NONE',  ( 4.968825510885260144, 1508.551704408389924, 211.9229860405860109 ) ) ;
#31458=CARTESIAN_POINT ( 'NONE',  ( 18.32583792955789903, 1473.764139442630039, 194.8973871065419985 ) ) ;
#31459=CARTESIAN_POINT ( 'NONE',  ( 1.396945595908719806, 1473.097535771269804, 219.2356281669150064 ) ) ;
#31463=CARTESIAN_POINT ( 'NONE',  ( 10.48842339441639915, 1452.980979821939854, 210.6446836343209839 ) ) ;
#31465=CARTESIAN_POINT ( 'NONE',  ( -15.31790971930000111, 1507.704306114589826, 209.3792549816630242 ) ) ;
#31469=CARTESIAN_POINT ( 'NONE',  ( 6.942384827123173174, 1507.551704408389924, 200.9625026564361292 ) ) ;
#31495=CARTESIAN_POINT ( 'NONE',  ( -9.972208786350000409, 1449.536236232390138, 205.8362451147190200 ) ) ;
#31496=CARTESIAN_POINT ( 'NONE',  ( -10.13268345264436476, 1480.912692742363561, 206.1544537871127432 ) ) ;
#31502=CARTESIAN_POINT ( 'NONE',  ( -11.36293846883789804, 1500.786239116730030, 211.0742332070699945 ) ) ;
#31505=CARTESIAN_POINT ( 'NONE',  ( 3.410547590470000223, 1507.830663321090015, 220.3411986762989727 ) ) ;
#31511=FACE_OUTER_BOUND ( 'NONE', #52943, .T. ) ;
#31522=EDGE_CURVE ( 'NONE', #43603, #4789, #86152, .T. ) ;
#31528=DIRECTION ( 'NONE',  ( 0.000000000000000000, -1.000000000000000000, 1.836970198721029688E-16 ) ) ;
#31535=CARTESIAN_POINT ( 'NONE',  ( -11.17096468969999812, 1500.478073591689963, 215.5530715242690007 ) ) ;
#31541=CARTESIAN_POINT ( 'NONE',  ( -9.096596473720000020, 1440.282624608189963, 206.1069770705490214 ) ) ;
#31551=CARTESIAN_POINT ( 'NONE',  ( 12.69964242394170029, 1421.449485046359996, 206.4738677144460155 ) ) ;
#31555=CARTESIAN_POINT ( 'NONE',  ( -13.59314176670009999, 1508.069786739810070, 209.4864804417960329 ) ) ;
#31556=ADVANCED_FACE ( 'NONE', ( #33144 ), #34830, .T. ) ;
#31557=CARTESIAN_POINT ( 'NONE',  ( -19.86622908376359931, 1443.388396254009876, 213.1207183147250248 ) ) ;
#31558=CARTESIAN_POINT ( 'NONE',  ( -16.56054082451800014, 1417.106265379630031, 208.4979211302300257 ) ) ;
#31564=CARTESIAN_POINT ( 'NONE',  ( -4.222077288720000432, 1454.203574068490298, 200.3246332720389944 ) ) ;
#31566=CARTESIAN_POINT ( 'NONE',  ( 8.413970532630001387, 1428.089005924990033, 212.8939830477889927 ) ) ;
#31569=CARTESIAN_POINT ( 'NONE',  ( -21.78529113934020245, 1417.868803632889922, 208.5446529662619923 ) ) ;
#31584=CARTESIAN_POINT ( 'NONE',  ( -4.776356492423380118, 1463.978274100160206, 200.0897609657779981 ) ) ;
#31594=ORIENTED_EDGE ( 'NONE', *, *, #2736, .T. ) ;
#31597=CARTESIAN_POINT ( 'NONE',  ( 21.05586012649999716, 1495.072013869990087, 210.1549089269589956 ) ) ;
#31603=CARTESIAN_POINT ( 'NONE',  ( -11.32042714269999983, 1502.674858046290183, 207.0911706105389953 ) ) ;
#31608=ORIENTED_EDGE ( 'NONE', *, *, #35189, .F. ) ;
#31611=CARTESIAN_POINT ( 'NONE',  ( -7.721313575298860421, 1452.995439927550024, 203.8751428730399766 ) ) ;
#31620=ADVANCED_FACE ( 'NONE', ( #56714 ), #101431, .F. ) ;
#31626=CARTESIAN_POINT ( 'NONE',  ( 12.19154428201109930, 1492.561849750740066, 211.0960655454310029 ) ) ;
#31640=CARTESIAN_POINT ( 'NONE',  ( 7.243833416339904296, 1473.411017056090031, 218.0151120354588556 ) ) ;
#31641=CARTESIAN_POINT ( 'NONE',  ( 11.97204719289999986, 1426.674835027849895, 205.8341005045690224 ) ) ;
#31642=CARTESIAN_POINT ( 'NONE',  ( -3.617573937782270210, 1497.333809982809953, 198.4503636364750037 ) ) ;
#31645=CARTESIAN_POINT ( 'NONE',  ( -2.664535259099999805E-15, 1422.937291763169924, 209.1218459616989946 ) ) ;
#31654=CARTESIAN_POINT ( 'NONE',  ( 10.83576136632169984, 1461.764785210480113, 210.8453021311209739 ) ) ;
#31655=CARTESIAN_POINT ( 'NONE',  ( 9.169705329756888901, 1425.158430046457852, 195.6334031360315748 ) ) ;
#31656=CARTESIAN_POINT ( 'NONE',  ( 4.438328147020000003, 1466.438991376089916, 218.4230750687189868 ) ) ;
#31658=EDGE_CURVE ( 'NONE', #21410, #101374, #24180, .T. ) ;
#31661=CARTESIAN_POINT ( 'NONE',  ( 8.305536275772812616, 1487.549204498889594, 202.1547115178333058 ) ) ;
#31666=ORIENTED_EDGE ( 'NONE', *, *, #54207, .F. ) ;
#31667=CARTESIAN_POINT ( 'NONE',  ( -8.039518803556870097, 1439.999387722500160, 205.2469398296260010 ) ) ;
#31670=CARTESIAN_POINT ( 'NONE',  ( 11.21799561054379879, 1470.401428587849978, 207.2916120790159766 ) ) ;
#31675=CARTESIAN_POINT ( 'NONE',  ( -3.586360116007019982, 1515.071395204220153, 213.2046256369000048 ) ) ;
#31678=CARTESIAN_POINT ( 'NONE',  ( -14.69797768358330003, 1415.677402203350084, 206.1947793185709941 ) ) ;
#31685=ORIENTED_EDGE ( 'NONE', *, *, #107727, .F. ) ;
#31688=CARTESIAN_POINT ( 'NONE',  ( 9.717824533310780666, 1463.678478211699939, 210.3770741684630252 ) ) ;
#31689=CARTESIAN_POINT ( 'NONE',  ( 3.845501273690000055, 1455.043435614390091, 217.8764266887590111 ) ) ;
#31691=CARTESIAN_POINT ( 'NONE',  ( -2.540028566810000221, 1444.571278203389966, 217.8835225073589754 ) ) ;
#31705=VERTEX_POINT ( 'NONE', #53286 ) ;
#31708=CARTESIAN_POINT ( 'NONE',  ( 16.43010731360000065, 1495.465599852389914, 192.8750426889990024 ) ) ;
#31716=CARTESIAN_POINT ( 'NONE',  ( -4.394233624539999994, 1456.808182323690062, 217.5515244654889955 ) ) ;
#31720=CARTESIAN_POINT ( 'NONE',  ( -4.328845283827259749, 1515.087839320550074, 210.3999710242079857 ) ) ;
#31725=CARTESIAN_POINT ( 'NONE',  ( -8.650355960269319411, 1448.128899224820088, 212.2110593161760050 ) ) ;
#31728=CARTESIAN_POINT ( 'NONE',  ( -17.64855902048280356, 1419.508594242146955, 207.1654737734966147 ) ) ;
#31732=FACE_OUTER_BOUND ( 'NONE', #94231, .T. ) ;
#31738=CARTESIAN_POINT ( 'NONE',  ( -9.638891686394590153, 1503.623617614200384, 228.8110675621960013 ) ) ;
#31740=CARTESIAN_POINT ( 'NONE',  ( -18.66351252432520269, 1486.318487979379825, 199.8022941382239992 ) ) ;
#31747=CARTESIAN_POINT ( 'NONE',  ( 10.78618902296759963, 1460.496538158609837, 207.3635337098189950 ) ) ;
#31755=CARTESIAN_POINT ( 'NONE',  ( 8.475509682807949474, 1437.831708687899891, 211.6527867693390306 ) ) ;
#31761=CARTESIAN_POINT ( 'NONE',  ( -11.31317986880000070, 1471.144533718689900, 207.5705785899590126 ) ) ;
#31765=EDGE_CURVE ( 'NONE', #93538, #44452, #44728, .T. ) ;
#31768=CARTESIAN_POINT ( 'NONE',  ( -9.643453033020000120, 1414.681692383400105, 208.0622029686790029 ) ) ;
#31771=CARTESIAN_POINT ( 'NONE',  ( 6.914811870799999483, 1487.329785955590069, 200.7563842756789825 ) ) ;
#31782=CARTESIAN_POINT ( 'NONE',  ( -16.93017999142119834, 1508.551704408389924, 212.6742212789120003 ) ) ;
#31783=CARTESIAN_POINT ( 'NONE',  ( -16.54713268119330039, 1508.454488439769875, 213.8523356813170153 ) ) ;
#31784=CARTESIAN_POINT ( 'NONE',  ( -2.620218387640000035, 1476.166204755790204, 220.2952108551989738 ) ) ;
#31786=CARTESIAN_POINT ( 'NONE',  ( -11.39965473667389873, 1470.700470268689969, 209.4027647874690103 ) ) ;
#31787=CARTESIAN_POINT ( 'NONE',  ( -6.423569254462077716, 1508.337306375136222, 219.9732112918911753 ) ) ;
#31789=CARTESIAN_POINT ( 'NONE',  ( 1.085795944719189832, 1456.124699793469972, 198.6100061673760138 ) ) ;
#31791=DIRECTION ( 'NONE',  ( -1.000000000000000000, 0.000000000000000000, 0.000000000000000000 ) ) ;
#31793=CARTESIAN_POINT ( 'NONE',  ( -10.57951331165799935, 1470.368418028770066, 211.8757554959190088 ) ) ;
#31798=ORIENTED_EDGE ( 'NONE', *, *, #76199, .F. ) ;
#31799=CARTESIAN_POINT ( 'NONE',  ( 7.491611919662470420, 1440.071325087319565, 213.7318617617365248 ) ) ;
#31804=CARTESIAN_POINT ( 'NONE',  ( 8.250335230039999246, 1424.462285376320096, 195.8663749243990253 ) ) ;
#31806=CARTESIAN_POINT ( 'NONE',  ( 11.09879666485499961, 1422.175572497959820, 210.6094381644089992 ) ) ;
#31809=CARTESIAN_POINT ( 'NONE',  ( -2.044097970649489948, 1508.551704408389924, 220.0684391793160160 ) ) ;
#31815=CARTESIAN_POINT ( 'NONE',  ( 11.63699242075930051, 1492.551924726440120, 211.6216904535779975 ) ) ;
#31816=CARTESIAN_POINT ( 'NONE',  ( -2.764335539890000248, 1457.844979587290027, 219.4374305647990013 ) ) ;
#31820=CARTESIAN_POINT ( 'NONE',  ( 4.771130221510349934, 1508.551704408389924, 205.6145743722929922 ) ) ;
#31824=CARTESIAN_POINT ( 'NONE',  ( -2.329906356571839865, 1515.372228416479857, 204.8601837680460278 ) ) ;
#31830=CARTESIAN_POINT ( 'NONE',  ( -13.28196447587500018, 1508.551704408389924, 216.3748897397299800 ) ) ;
#31836=CARTESIAN_POINT ( 'NONE',  ( 7.743638678103569539, 1435.911626056160003, 205.3099362470069877 ) ) ;
#31858=CARTESIAN_POINT ( 'NONE',  ( 7.261033881273809776, 1424.990117404329794, 212.7330084483390067 ) ) ;
#31859=ORIENTED_EDGE ( 'NONE', *, *, #19031, .F. ) ;
#31873=CARTESIAN_POINT ( 'NONE',  ( 9.717822231039999537, 1463.678487757089897, 210.3770952454989924 ) ) ;
#31889=CARTESIAN_POINT ( 'NONE',  ( -5.881379503709999845, 1428.766218426890191, 203.1321793329989873 ) ) ;
#31893=AXIS2_PLACEMENT_3D ( 'NONE', #30192, #36945, #62187 ) ;
#31895=CARTESIAN_POINT ( 'NONE',  ( 9.293666974126480795, 1480.089863132871187, 204.1131580292703802 ) ) ;
#31897=CARTESIAN_POINT ( 'NONE',  ( -10.63047325564510004, 1480.584009184299930, 210.2203730784849824 ) ) ;
#31900=CARTESIAN_POINT ( 'NONE',  ( 7.461990519024649160, 1504.220424024579870, 219.4654900686530254 ) ) ;
#31901=CARTESIAN_POINT ( 'NONE',  ( 7.782527000790000038, 1421.790398246840141, 195.8641137985989928 ) ) ;
#31903=CARTESIAN_POINT ( 'NONE',  ( -9.819355888608599869, 1492.974921486040103, 201.7186537263710022 ) ) ;
#31904=CARTESIAN_POINT ( 'NONE',  ( -4.321803588699999921, 1496.124825247590024, 198.6279956811989962 ) ) ;
#31908=CARTESIAN_POINT ( 'NONE',  ( 10.66776494214329851, 1424.286285492139996, 206.6302606398689932 ) ) ;
#31916=CARTESIAN_POINT ( 'NONE',  ( 9.802591111456759876, 1422.649162510939959, 211.3555123156029936 ) ) ;
#31917=CARTESIAN_POINT ( 'NONE',  ( 11.58812742166940168, 1425.640754144680159, 202.9099269016940070 ) ) ;
#31918=B_SPLINE_CURVE_WITH_KNOTS ( 'NONE', 3,
 ( #33824, #26529, #60725, #60156, #69119, #51191 ),
 .UNSPECIFIED., .F., .F.,
 ( 4, 2, 4 ),
 ( 0.000000000000000000, 0.5000000000000000000, 1.000000000000000000 ),
 .UNSPECIFIED. ) ;
#31921=CARTESIAN_POINT ( 'NONE',  ( -7.795091205023656933, 1476.960015112429573, 215.9744489608353319 ) ) ;
#31926=CARTESIAN_POINT ( 'NONE',  ( -16.77179453697938527, 1420.486811422051233, 203.1613059882370180 ) ) ;
#31929=CARTESIAN_POINT ( 'NONE',  ( 0.8775825618903729808, 1398.755125754900064, 208.6424204230947907 ) ) ;
#31930=CARTESIAN_POINT ( 'NONE',  ( 4.223612416888080645, 1474.237109173149975, 219.7333844760279931 ) ) ;
#31939=CARTESIAN_POINT ( 'NONE',  ( -17.51440549372729905, 1442.103934404829943, 219.2287673605049747 ) ) ;
#31942=CARTESIAN_POINT ( 'NONE',  ( 8.293154156760014217, 1466.896286154528752, 203.5718718306909523 ) ) ;
#31946=CARTESIAN_POINT ( 'NONE',  ( -0.8748704360600072505, 1484.083060082853308, 198.4676730996152969 ) ) ;
#31949=CARTESIAN_POINT ( 'NONE',  ( -3.628052555810424629, 1430.352677179689636, 201.5964689278353035 ) ) ;
#31956=CARTESIAN_POINT ( 'NONE',  ( 2.516232255349999836, 1464.674062122390069, 202.5523636628589941 ) ) ;
#31967=CONICAL_SURFACE ( 'NONE', #89209, 7.500000000000000000, 0.02617993877989872875 ) ;
#31970=CARTESIAN_POINT ( 'NONE',  ( -18.74729292449999818, 1442.199705176290081, 209.1218459616989946 ) ) ;
#31972=CARTESIAN_POINT ( 'NONE',  ( 5.826428076080000906, 1473.811884028689974, 218.9454251420289950 ) ) ;
#31974=CARTESIAN_POINT ( 'NONE',  ( 10.18019783711949877, 1471.338426166499858, 211.9712393461159934 ) ) ;
#31984=CARTESIAN_POINT ( 'NONE',  ( 7.244363788860000319, 1481.023503507690066, 208.0198210207190073 ) ) ;
#31996=ORIENTED_EDGE ( 'NONE', *, *, #57059, .F. ) ;
#32000=CARTESIAN_POINT ( 'NONE',  ( 2.396857868302820105, 1485.113936978040101, 220.7346362247920126 ) ) ;
#32008=CARTESIAN_POINT ( 'NONE',  ( 12.70100719244910081, 1500.608200984970154, 209.4159698383299997 ) ) ;
#32013=CARTESIAN_POINT ( 'NONE',  ( -21.44637752539939868, 1506.412652546340269, 216.0243762360449864 ) ) ;
#32018=CARTESIAN_POINT ( 'NONE',  ( 10.28174319281220050, 1453.348041341110047, 211.7471195966300002 ) ) ;
#32021=CARTESIAN_POINT ( 'NONE',  ( -20.35947145212350051, 1508.252440922349933, 209.6500315394189897 ) ) ;
#32023=CARTESIAN_POINT ( 'NONE',  ( 2.330134126767420266, 1515.064792882699976, 204.7923971855439902 ) ) ;
#32031=ORIENTED_EDGE ( 'NONE', *, *, #26512, .F. ) ;
#32034=ORIENTED_EDGE ( 'NONE', *, *, #22923, .F. ) ;
#32039=DIRECTION ( 'NONE',  ( -7.436362843295819681E-17, 1.000000000000000000, -1.457576885956999882E-16 ) ) ;
#32040=CARTESIAN_POINT ( 'NONE',  ( 8.454790733525280544, 1428.363638633589972, 213.4109935021670026 ) ) ;
#32041=CARTESIAN_POINT ( 'NONE',  ( -17.02817110700241443, 1508.455360531000224, 213.2597695858250404 ) ) ;
#32042=CARTESIAN_POINT ( 'NONE',  ( -10.69637384178539996, 1462.945480530389887, 206.3136169826919968 ) ) ;
#32044=CARTESIAN_POINT ( 'NONE',  ( 10.63889126261920026, 1470.011729377750044, 207.0794648040029813 ) ) ;
#32062=CARTESIAN_POINT ( 'NONE',  ( -12.48995958582669985, 1501.883328869510024, 211.6213070116990025 ) ) ;
#32065=CARTESIAN_POINT ( 'NONE',  ( 2.810679194570000039, 1508.430220233089813, 220.1167136484990010 ) ) ;
#32074=CARTESIAN_POINT ( 'NONE',  ( 6.575517168109999311, 1463.094441317690098, 208.8281860452259764 ) ) ;
#32082=EDGE_CURVE ( 'NONE', #57781, #19417, #109478, .T. ) ;
#32087=CARTESIAN_POINT ( 'NONE',  ( -3.440623305239999929, 1458.093607836889760, 219.2469823057990084 ) ) ;
#32090=ADVANCED_FACE ( 'NONE', ( #20598 ), #100512, .T. ) ;
#32092=CARTESIAN_POINT ( 'NONE',  ( -5.445054425793269814, 1494.866999379700246, 198.0707246423999948 ) ) ;
#32101=CARTESIAN_POINT ( 'NONE',  ( -11.21638122688047368, 1414.413060387330006, 208.4170904300009113 ) ) ;
#32106=B_SPLINE_SURFACE_WITH_KNOTS ( 'NONE', 5, 1, ( 
 ( #100670, #41881 ),
 ( #109641, #92279 ),
 ( #15548, #7181 ),
 ( #76040, #41338 ),
 ( #67658, #101766 ),
 ( #53061, #60351 ) ),
 .UNSPECIFIED., .F., .F., .F.,
 ( 6, 6 ),
 ( 2, 2 ),
 ( 0.000000000000000000, 4.002909968980000066 ),
 ( 8.881784197000000007E-16, 14.00000000000000000 ),
 .UNSPECIFIED. ) ;
#32110=CARTESIAN_POINT ( 'NONE',  ( 4.229167303610000594, 1436.983388288790138, 227.1518914930990150 ) ) ;
#32115=B_SPLINE_SURFACE_WITH_KNOTS ( 'NONE', 5, 5, ( 
 ( #48894, #31505, #74636, #40461, #81907, #5212 ),
 ( #39366, #49435, #108771, #32065, #66254, #100373 ),
 ( #23658, #82477, #83557, #107675, #65135, #38257 ),
 ( #99248, #22525, #56727, #8500, #60601, #24734 ),
 ( #84114, #58931, #102005, #33702, #84659, #76830 ),
 ( #85210, #16336, #49977, #16879, #41578, #50535 ),
 ( #60044, #92508, #144, #66798, #7959, #42126 ),
 ( #76274, #6850, #75734, #109878, #33157, #7413 ),
 ( #110423, #41011, #67897, #94722, #93601, #9067 ) ),
 .UNSPECIFIED., .F., .F., .F.,
 ( 6, 3, 6 ),
 ( 6, 6 ),
 ( 0.000000000000000000, 4.751561961960000247, 10.41361588720000064 ),
 ( 0.000000000000000000, 1.000000000000000000 ),
 .UNSPECIFIED. ) ;
#32117=CARTESIAN_POINT ( 'NONE',  ( -13.59471078833350077, 1507.829393183870025, 209.3810580891559994 ) ) ;
#32118=CARTESIAN_POINT ( 'NONE',  ( -2.775555821678710178, 1468.867611629940257, 187.4507004058289965 ) ) ;
#32124=CARTESIAN_POINT ( 'NONE',  ( -5.349442052910000633, 1454.859441816789968, 201.3532327490590035 ) ) ;
#32129=CARTESIAN_POINT ( 'NONE',  ( -17.02234413428539739, 1420.211165650439852, 204.6962164606919998 ) ) ;
#32141=CARTESIAN_POINT ( 'NONE',  ( 2.919790884400000230, 1445.755750970590043, 200.1990502211790215 ) ) ;
#32144=CARTESIAN_POINT ( 'NONE',  ( -4.591854502347329614, 1463.586371817870031, 200.3131754724250015 ) ) ;
#32145=CARTESIAN_POINT ( 'NONE',  ( -17.50950631050429962, 1417.908328417909843, 206.9179188249679839 ) ) ;
#32161=CARTESIAN_POINT ( 'NONE',  ( -11.68017202480000094, 1503.190160464489963, 208.0141257398589971 ) ) ;
#32179=CARTESIAN_POINT ( 'NONE',  ( 21.03867822700000190, 1494.819670719790111, 208.4793431422329775 ) ) ;
#32180=B_SPLINE_CURVE_WITH_KNOTS ( 'NONE', 5,
 ( #87028, #44492, #1952, #70274, #34420, #80297, #81928, #64062, #3612 ),
 .UNSPECIFIED., .F., .F.,
 ( 6, 3, 6 ),
 ( 429.4216791289999833, 432.6128460950000090, 434.5419185690000177 ),
 .UNSPECIFIED. ) ;
#32185=CARTESIAN_POINT ( 'NONE',  ( 11.90847486998620042, 1492.860655245649923, 212.4217341398910150 ) ) ;
#32199=( BOUNDED_CURVE ( )  B_SPLINE_CURVE ( 3, ( #107077, #64553, #11924, #46104 ),
 .UNSPECIFIED., .F., .F. ) 
 B_SPLINE_CURVE_WITH_KNOTS ( ( 4, 4 ),
 ( 0.9985734095396142651, 2.143019256287069574 ),
 .UNSPECIFIED. ) 
 CURVE ( )  GEOMETRIC_REPRESENTATION_ITEM ( )  RATIONAL_B_SPLINE_CURVE ( ( 1.000000000000000000, 0.8937995569179151278, 0.8937995569179151278, 1.000000000000000000 ) ) 
 REPRESENTATION_ITEM ( '' )  );
#32201=CARTESIAN_POINT ( 'NONE',  ( 5.027849746001829878, 1485.388521802679861, 218.6205834690780136 ) ) ;
#32203=CARTESIAN_POINT ( 'NONE',  ( 1.513089995879569383, 1498.833490213426558, 197.8872906115371109 ) ) ;
#32215=CARTESIAN_POINT ( 'NONE',  ( 10.84428623605119846, 1461.742173074219863, 210.7892283924740013 ) ) ;
#32216=LINE ( 'NONE', #50138, #71756 ) ;
#32217=CARTESIAN_POINT ( 'NONE',  ( 4.575325728500000189, 1466.769487727290198, 218.0849816997290134 ) ) ;
#32221=CARTESIAN_POINT ( 'NONE',  ( 8.033473906835755685, 1487.403589905162789, 201.8500708422530749 ) ) ;
#32232=CARTESIAN_POINT ( 'NONE',  ( -5.668006973570000717, 1484.831902833290087, 198.6468248041990137 ) ) ;
#32237=CARTESIAN_POINT ( 'NONE',  ( -8.671125672311569943, 1437.958062009570085, 208.7129840011259887 ) ) ;
#32244=ORIENTED_EDGE ( 'NONE', *, *, #78050, .T. ) ;
#32254=CARTESIAN_POINT ( 'NONE',  ( -2.975911813860000255, 1445.219193664589966, 217.6412520525290120 ) ) ;
#32257=CARTESIAN_POINT ( 'NONE',  ( 2.220446049249999755E-16, 1516.051704408390151, 209.1218459616989946 ) ) ;
#32261=CARTESIAN_POINT ( 'NONE',  ( -3.782764153885679992, 1454.025518203000047, 199.3518729501290068 ) ) ;
#32262=CARTESIAN_POINT ( 'NONE',  ( -11.47171006529080017, 1480.905530949450167, 211.9467558702930035 ) ) ;
#32267=VERTEX_POINT ( 'NONE', #67605 ) ;
#32269=CARTESIAN_POINT ( 'NONE',  ( 0.03745370349719699676, 1502.433616705189934, 233.2734988771990174 ) ) ;
#32273=CARTESIAN_POINT ( 'NONE',  ( -9.902323404119773187, 1422.657237248887441, 210.6700027881538233 ) ) ;
#32276=CARTESIAN_POINT ( 'NONE',  ( -20.53044877720000372, 1484.405134138590029, 211.1019867995989898 ) ) ;
#32283=CARTESIAN_POINT ( 'NONE',  ( 10.41177662488709998, 1460.024663752159995, 205.9063130872220029 ) ) ;
#32291=CARTESIAN_POINT ( 'NONE',  ( -17.63831374727218915, 1419.677598567774794, 207.0084533942130349 ) ) ;
#32299=CARTESIAN_POINT ( 'NONE',  ( 10.95098223739999987, 1471.837422851889869, 212.3987393883689947 ) ) ;
#32302=DIRECTION ( 'NONE',  ( 9.341989762165448955E-47, -1.000000000000000000, 1.836970198721029688E-16 ) ) ;
#32312=CARTESIAN_POINT ( 'NONE',  ( 4.138599669886909638, 1426.481420035549945, 191.5413917934459960 ) ) ;
#32316=EDGE_CURVE ( 'NONE', #43735, #37252, #6031, .T. ) ;
#32318=CARTESIAN_POINT ( 'NONE',  ( -2.832196849119999804, 1497.533045831589789, 201.1364434386690050 ) ) ;
#32319=CARTESIAN_POINT ( 'NONE',  ( 8.993477303732159811, 1437.143916695869848, 212.0776306990970284 ) ) ;
#32325=CARTESIAN_POINT ( 'NONE',  ( -8.628995479883890596, 1437.624223205020144, 208.3388049724410109 ) ) ;
#32334=CARTESIAN_POINT ( 'NONE',  ( -9.306860583259998876, 1415.471543658610017, 206.2851672951890123 ) ) ;
#32337=CARTESIAN_POINT ( 'NONE',  ( 5.247705765879999262, 1487.053368902190186, 199.5049302458390059 ) ) ;
#32341=CARTESIAN_POINT ( 'NONE',  ( -13.74003952106156135, 1447.587101742432196, 195.3179347002435122 ) ) ;
#32345=CARTESIAN_POINT ( 'NONE',  ( -16.50397793950000036, 1420.609998909190153, 203.2697724632589882 ) ) ;
#32350=CARTESIAN_POINT ( 'NONE',  ( -11.26841194160630089, 1471.218450017450095, 207.2998296250100054 ) ) ;
#32351=CARTESIAN_POINT ( 'NONE',  ( -5.004574234055505499, 1508.230405643570293, 220.4208381782240735 ) ) ;
#32353=CARTESIAN_POINT ( 'NONE',  ( -2.690862365372829856, 1454.581388717919936, 198.9826033966560033 ) ) ;
#32358=CARTESIAN_POINT ( 'NONE',  ( -1.200707496499999971, 1481.436145357489977, 229.6922108031990035 ) ) ;
#32360=VERTEX_POINT ( 'NONE', #53012 ) ;
#32361=CARTESIAN_POINT ( 'NONE',  ( 3.628818056492709943, 1505.602008419380127, 221.3635114792730292 ) ) ;
#32363=CARTESIAN_POINT ( 'NONE',  ( -2.048534905309999932, 1444.110401950890036, 199.2775038477390126 ) ) ;
#32364=CARTESIAN_POINT ( 'NONE',  ( 11.56811101928649954, 1502.082184429209974, 211.3526444203309893 ) ) ;
#32365=CARTESIAN_POINT ( 'NONE',  ( -295.4396879434189600, -8387.357407334295203, -1814.563882277197763 ) ) ;
#32368=CARTESIAN_POINT ( 'NONE',  ( -0.1127505383448819953, 1508.551704408389924, 220.0210036674560001 ) ) ;
#32369=CARTESIAN_POINT ( 'NONE',  ( -4.138543391159999807, 1515.492058413689847, 207.2788837304390199 ) ) ;
#32375=CARTESIAN_POINT ( 'NONE',  ( 11.16165179841680022, 1492.334248400359911, 211.8614833883839879 ) ) ;
#32376=CARTESIAN_POINT ( 'NONE',  ( 0.02062240259779879806, 1456.497060068189967, 219.0045627830490105 ) ) ;
#32380=CARTESIAN_POINT ( 'NONE',  ( 4.980141907642230414, 1508.551704408389924, 206.4478324081339906 ) ) ;
#32382=ORIENTED_EDGE ( 'NONE', *, *, #36587, .T. ) ;
#32387=CARTESIAN_POINT ( 'NONE',  ( -7.935787006710000036, 1461.796959919690153, 203.3733083132490265 ) ) ;
#32391=VECTOR ( 'NONE', #106601, 1000.000000000000000 ) ;
#32392=CARTESIAN_POINT ( 'NONE',  ( -9.648630365757211891, 1508.551704408389924, 218.4115283752189782 ) ) ;
#32395=CARTESIAN_POINT ( 'NONE',  ( 16.09101509135354036, 1459.755789917567654, 220.7358767599917542 ) ) ;
#32396=CARTESIAN_POINT ( 'NONE',  ( 1.914129829356669976, 1431.087911108530079, 199.8421603670449826 ) ) ;
#32401=CARTESIAN_POINT ( 'NONE',  ( 0.000000000000000000, 1420.584111001019892, 209.1218459616989946 ) ) ;
#32407=CARTESIAN_POINT ( 'NONE',  ( 1.550613581710394095, 1515.551704304084751, 213.0145121093438547 ) ) ;
#32408=CARTESIAN_POINT ( 'NONE',  ( -15.05020751920000066, 1420.512178086570202, 211.8108503490890087 ) ) ;
#32416=CARTESIAN_POINT ( 'NONE',  ( -7.807919481659999938, 1426.371178030289911, 206.6874965076690103 ) ) ;
#32417=B_SPLINE_CURVE_WITH_KNOTS ( 'NONE', 3,
 ( #93042, #41559, #7394, #75714, #123, #102532, #91948, #34247, #109860, #32044, #85747, #43216, #32603, #92486, #67876, #100879, #66233, #16316, #58912, #67326, #50517, #25272, #75170, #100352, #8480, #23640, #68430, #16859, #15756, #33137, #109320, #6831, #40991, #24714 ),
 .UNSPECIFIED., .F., .F.,
 ( 4, 3, 3, 3, 3, 3, 3, 3, 3, 3, 3, 4 ),
 ( -1.999999957325899969, -1.874565698771090139, -1.690129705517909864, -1.503459105586989919, -1.315598157701630022, -1.126271480114729995, -0.9365167983017219644, -0.7468004907161611694, -0.5575843769484218893, -0.3700485060396170311, -0.1840983994498410770, 0.000000000000000000 ),
 .UNSPECIFIED. ) ;
#32421=CARTESIAN_POINT ( 'NONE',  ( 7.246758094710430420, 1424.980848950539894, 212.7605380421140069 ) ) ;
#32441=ORIENTED_EDGE ( 'NONE', *, *, #53536, .T. ) ;
#32448=EDGE_CURVE ( 'NONE', #73065, #82244, #25832, .T. ) ;
#32460=CARTESIAN_POINT ( 'NONE',  ( 4.541133981099999772, 1426.446980476019917, 211.3175313703289930 ) ) ;
#32466=CARTESIAN_POINT ( 'NONE',  ( 7.966089429799998456, 1421.435344681000061, 195.9328034231990046 ) ) ;
#32468=CARTESIAN_POINT ( 'NONE',  ( 0.3404198581328219952, 1431.708939325159918, 218.6080673264870029 ) ) ;
#32469=CARTESIAN_POINT ( 'NONE',  ( -4.329448776040000446, 1515.064792882589927, 209.0973262533439936 ) ) ;
#32472=CARTESIAN_POINT ( 'NONE',  ( 4.038582000521929061, 1515.598601297060441, 209.4325486173436843 ) ) ;
#32473=CARTESIAN_POINT ( 'NONE',  ( 10.66776494060489888, 1424.286284153560018, 206.6302608488180113 ) ) ;
#32479=CARTESIAN_POINT ( 'NONE',  ( 2.340571794239999726, 1472.604797962090061, 216.2450463976489914 ) ) ;
#32483=CARTESIAN_POINT ( 'NONE',  ( 9.799993285045120572, 1423.431501241479964, 209.4821564460780223 ) ) ;
#32484=CARTESIAN_POINT ( 'NONE',  ( 10.94471713272500146, 1423.681646166069868, 203.2258399444270083 ) ) ;
#32485=CARTESIAN_POINT ( 'NONE',  ( 1.727284872639999858, 1431.232427857390121, 218.4620812309590008 ) ) ;
#32490=CARTESIAN_POINT ( 'NONE',  ( 1.914156610164409855, 1431.087920293139859, 199.8421651263110164 ) ) ;
#32494=CARTESIAN_POINT ( 'NONE',  ( 8.536750983910001978, 1465.433596956489964, 214.1723092710689968 ) ) ;
#32499=CARTESIAN_POINT ( 'NONE',  ( -8.117665312093365060, 1425.422482083973136, 208.7068306292352986 ) ) ;
#32501=B_SPLINE_CURVE_WITH_KNOTS ( 'NONE', 5,
 ( #83454, #17331, #92402, #84564, #59946, #6748, #94062, #101337, #32521 ),
 .UNSPECIFIED., .F., .F.,
 ( 6, 3, 6 ),
 ( 0.000000000000000000, 0.5111911274250463544, 1.000000000000000000 ),
 .UNSPECIFIED. ) ;
#32502=CARTESIAN_POINT ( 'NONE',  ( -1.808747093880000101, 1474.298755092390138, 216.4373183392189617 ) ) ;
#32504=CARTESIAN_POINT ( 'NONE',  ( 0.7420515760630009838, 1515.368784161290250, 204.8340560411189699 ) ) ;
#32506=CARTESIAN_POINT ( 'NONE',  ( -13.97985289466289949, 1420.196174639120045, 195.9955836006969889 ) ) ;
#32520=CARTESIAN_POINT ( 'NONE',  ( 20.54545170502450446, 1497.714248496870141, 214.2325552634220003 ) ) ;
#32521=CARTESIAN_POINT ( 'NONE',  ( 3.628818056492709943, 1505.602008419380127, 221.3635114792730292 ) ) ;
#32523=CARTESIAN_POINT ( 'NONE',  ( -14.91281678549999867, 1416.540137034410009, 213.0067496813389880 ) ) ;
#32528=CARTESIAN_POINT ( 'NONE',  ( 11.82645876916039995, 1426.795760154579966, 206.5338053568990233 ) ) ;
#32534=CARTESIAN_POINT ( 'NONE',  ( 2.484906683780000236, 1472.794382616990106, 219.0213525527389891 ) ) ;
#32535=CARTESIAN_POINT ( 'NONE',  ( 10.20292507491700107, 1470.367289678880070, 209.9988428381880112 ) ) ;
#32538=B_SPLINE_CURVE_WITH_KNOTS ( 'NONE', 3,
 ( #13542, #29268, #63460, #97579, #55046, #89174 ),
 .UNSPECIFIED., .F., .F.,
 ( 4, 2, 4 ),
 ( 0.000000000000000000, 0.5000000000000000000, 1.000000000000000000 ),
 .UNSPECIFIED. ) ;
#32539=CARTESIAN_POINT ( 'NONE',  ( -11.09323634000895353, 1492.391963403851150, 209.0647905715161698 ) ) ;
#32556=CARTESIAN_POINT ( 'NONE',  ( -17.54118812318929699, 1417.910349704349983, 206.8634943573240150 ) ) ;
#32559=CARTESIAN_POINT ( 'NONE',  ( 11.36069158549999969, 1501.598968272789989, 207.6205322127590023 ) ) ;
#32573=CARTESIAN_POINT ( 'NONE',  ( 18.46110511450000047, 1471.786120934990095, 195.2229451476989937 ) ) ;
#32575=VERTEX_POINT ( 'NONE', #99941 ) ;
#32578=CARTESIAN_POINT ( 'NONE',  ( 10.42032938315659862, 1453.131236670619955, 211.0854769158530360 ) ) ;
#32580=CARTESIAN_POINT ( 'NONE',  ( -20.34501938112269670, 1508.551704408389924, 210.4487953478319753 ) ) ;
#32583=CARTESIAN_POINT ( 'NONE',  ( 4.329448776040000446, 1515.064792882589927, 210.9648081929590262 ) ) ;
#32599=CARTESIAN_POINT ( 'NONE',  ( 6.884066909838960413, 1429.271425755099926, 215.6498002703089867 ) ) ;
#32601=CARTESIAN_POINT ( 'NONE',  ( -10.24974442935089947, 1462.794995015260156, 206.4145582120489735 ) ) ;
#32603=CARTESIAN_POINT ( 'NONE',  ( 10.47538074031769995, 1469.876780579760180, 207.1493381432659930 ) ) ;
#32617=CARTESIAN_POINT ( 'NONE',  ( 2.956827888069309740, 1515.222544093250008, 213.4459675459839900 ) ) ;
#32618=EDGE_CURVE ( 'NONE', #40693, #88887, #92680, .T. ) ;
#32620=CARTESIAN_POINT ( 'NONE',  ( -11.98797817168060043, 1501.622048148490194, 211.4516665317300124 ) ) ;
#32622=CARTESIAN_POINT ( 'NONE',  ( -15.55913749090388087, 1415.687746563815381, 209.6140629208140922 ) ) ;
#32625=CARTESIAN_POINT ( 'NONE',  ( -6.095125402108049428, 1441.837371024610093, 202.1071835498420057 ) ) ;
#32627=CARTESIAN_POINT ( 'NONE',  ( -7.602521990106799521, 1425.809942238630128, 203.7442148849289936 ) ) ;
#32628=CARTESIAN_POINT ( 'NONE',  ( 6.906779373730000060, 1480.511273071390178, 206.6585084174489850 ) ) ;
#32638=CARTESIAN_POINT ( 'NONE',  ( 2.003572920832760396, 1454.623075833809935, 218.3091034149879874 ) ) ;
#32641=CARTESIAN_POINT ( 'NONE',  ( -15.22265112240000029, 1415.931502849980234, 206.6367959904590066 ) ) ;
#32644=CARTESIAN_POINT ( 'NONE',  ( 9.181100887863649973, 1450.964097471789955, 210.1935140534000084 ) ) ;
#32648=CARTESIAN_POINT ( 'NONE',  ( -12.90006350071139885, 1507.961479924099876, 209.2725772594830005 ) ) ;
#32663=CARTESIAN_POINT ( 'NONE',  ( 10.32403803707900103, 1479.706866225239992, 206.5120394917040301 ) ) ;
#32664=ORIENTED_EDGE ( 'NONE', *, *, #35867, .F. ) ;
#32666=CARTESIAN_POINT ( 'NONE',  ( -19.16799087484339736, 1444.936066881249872, 199.7607002489500019 ) ) ;
#32668=CARTESIAN_POINT ( 'NONE',  ( 20.10528729596699904, 1430.878053334959986, 215.1856554786780009 ) ) ;
#32672=CYLINDRICAL_SURFACE ( 'NONE', #63439, 0.5000000000000026645 ) ;
#32683=ORIENTED_EDGE ( 'NONE', *, *, #3458, .F. ) ;
#32691=CARTESIAN_POINT ( 'NONE',  ( 3.829164871872719811, 1515.551704201149960, 206.7918886313289875 ) ) ;
#32695=CARTESIAN_POINT ( 'NONE',  ( -4.990022623493119980, 1464.266792026490066, 199.7730999070479925 ) ) ;
#32696=CARTESIAN_POINT ( 'NONE',  ( 1.690753242990000071, 1418.551567007509902, 204.1881961068189923 ) ) ;
#32702=ORIENTED_EDGE ( 'NONE', *, *, #56884, .F. ) ;
#32704=ORIENTED_EDGE ( 'NONE', *, *, #86501, .F. ) ;
#32712=CARTESIAN_POINT ( 'NONE',  ( -12.75671326420000007, 1503.496710435090108, 208.6968438420659879 ) ) ;
#32716=( BOUNDED_SURFACE ( )  B_SPLINE_SURFACE ( 1, 2, ( 
 ( #78205, #104514, #35650, #103958, #27255, #78766, #2082 ),
 ( #102834, #96110, #70955, #19384, #105070, #28359, #26128 ) ),
 .UNSPECIFIED., .F., .F., .F. ) 
 B_SPLINE_SURFACE_WITH_KNOTS ( ( 2, 2 ),
 ( 3, 2, 2, 3 ),
 ( -10000.00000000000000, 10000.00000000000000 ),
 ( 2.628620570831615044, 3.141592653589790007, 4.712388980384689674, 5.770213224422409581 ),
 .UNSPECIFIED. ) 
 GEOMETRIC_REPRESENTATION_ITEM ( )  RATIONAL_B_SPLINE_SURFACE ( (
 ( 0.8711730262221800691, 0.9043503973637049276, 1.000000000000000000, 0.7071067811865480168, 1.000000000000000000, 0.8027563838226560167, 0.8711730262223089660),
 ( 0.8711730262221800691, 0.9043503973637049276, 1.000000000000000000, 0.7071067811865480168, 1.000000000000000000, 0.8027563838226560167, 0.8711730262223089660) ) ) 
 REPRESENTATION_ITEM ( '' )  SURFACE ( )  );
#32719=ORIENTED_EDGE ( 'NONE', *, *, #11821, .F. ) ;
#32728=CARTESIAN_POINT ( 'NONE',  ( -14.95528230852240092, 1508.551704408389924, 210.3622119209300081 ) ) ;
#32734=CARTESIAN_POINT ( 'NONE',  ( 11.71533056565333197, 1414.421228241719973, 209.8579518281819674 ) ) ;
#32735=CARTESIAN_POINT ( 'NONE',  ( 1.542378980109999853, 1442.042834985789796, 218.9497927206290058 ) ) ;
#32747=CARTESIAN_POINT ( 'NONE',  ( 10.70463268489986142, 1472.030523703590006, 213.2176825260488613 ) ) ;
#32748=CARTESIAN_POINT ( 'NONE',  ( 11.92256370189999792, 1421.800997465520140, 206.9479557017089917 ) ) ;
#32760=CARTESIAN_POINT ( 'NONE',  ( -0.4215884677550009729, 1444.753357002690109, 218.0930000387590155 ) ) ;
#32771=CARTESIAN_POINT ( 'NONE',  ( -8.178306764501339643, 1439.185977283359989, 206.0664987394139871 ) ) ;
#32777=CARTESIAN_POINT ( 'NONE',  ( -9.062501693986670048, 1438.222286192869888, 210.0833190316829757 ) ) ;
#32778=CARTESIAN_POINT ( 'NONE',  ( -2.898098007869549964, 1515.492902828930028, 213.2585957736860109 ) ) ;
#32782=CARTESIAN_POINT ( 'NONE',  ( -4.532544388959999893, 1433.779930133089920, 212.7417843401189828 ) ) ;
#32784=ORIENTED_EDGE ( 'NONE', *, *, #35850, .F. ) ;
#32787=VERTEX_POINT ( 'NONE', #33290 ) ;
#32789=FACE_OUTER_BOUND ( 'NONE', #40150, .T. ) ;
#32791=CARTESIAN_POINT ( 'NONE',  ( 1.660254716250000095, 1454.717553612689926, 218.3876423414490091 ) ) ;
#32796=CARTESIAN_POINT ( 'NONE',  ( 9.624923068494529943, 1463.973964823269853, 211.0293340011560019 ) ) ;
#32797=CARTESIAN_POINT ( 'NONE',  ( 7.368463984539999956, 1423.734805372980190, 213.0570616533089776 ) ) ;
#32799=CARTESIAN_POINT ( 'NONE',  ( -3.345456442099850047, 1454.253772392629799, 199.1892521207759899 ) ) ;
#32805=ORIENTED_EDGE ( 'NONE', *, *, #35047, .F. ) ;
#32807=CARTESIAN_POINT ( 'NONE',  ( -18.90194474967839966, 1503.740679335620143, 222.2659978651250015 ) ) ;
#32809=CARTESIAN_POINT ( 'NONE',  ( 0.4943681453122752423, 1473.359364695990507, 219.3321834821998664 ) ) ;
#32811=CARTESIAN_POINT ( 'NONE',  ( -14.61959290290118041, 1420.357143390019928, 213.8552925859152367 ) ) ;
#32814=CARTESIAN_POINT ( 'NONE',  ( 18.29188182340000068, 1431.768652859389704, 209.1218459616989946 ) ) ;
#32817=CARTESIAN_POINT ( 'NONE',  ( -9.152553986288870291, 1448.325309252199986, 210.6317879819130212 ) ) ;
#32821=CARTESIAN_POINT ( 'NONE',  ( -4.329089011153670619, 1515.078531749479907, 210.5455323891260093 ) ) ;
#32825=CARTESIAN_POINT ( 'NONE',  ( 7.596893798666170206, 1424.854153163179944, 194.2789038821860288 ) ) ;
#32835=B_SPLINE_CURVE_WITH_KNOTS ( 'NONE', 3,
 ( #21069, #46874, #81002, #38436, #27289, #70432 ),
 .UNSPECIFIED., .F., .F.,
 ( 4, 2, 4 ),
 ( 0.000000000000000000, 0.4821770457261087550, 0.9643540914522175100 ),
 .UNSPECIFIED. ) ;
#32839=CARTESIAN_POINT ( 'NONE',  ( 11.27867428310018560, 1425.794442006550980, 197.9026106389715380 ) ) ;
#32855=CARTESIAN_POINT ( 'NONE',  ( -10.24275455859999973, 1472.071912135389994, 207.8889228267089777 ) ) ;
#32857=ORIENTED_EDGE ( 'NONE', *, *, #78858, .T. ) ;
#32862=CARTESIAN_POINT ( 'NONE',  ( -9.467443545490001000, 1415.183427459279983, 206.9475390216489927 ) ) ;
#32865=CARTESIAN_POINT ( 'NONE',  ( 6.435066429969999113, 1488.114327637990073, 199.4146561316890143 ) ) ;
#32876=CARTESIAN_POINT ( 'NONE',  ( -17.16826720739999956, 1420.250473903940019, 203.6854009021189995 ) ) ;
#32879=CARTESIAN_POINT ( 'NONE',  ( -2.829326390389999890, 1474.515727672689991, 219.0106651408090102 ) ) ;
#32881=CARTESIAN_POINT ( 'NONE',  ( -21.47567121439999838, 1505.309716411789850, 210.5476439721289807 ) ) ;
#32882=CARTESIAN_POINT ( 'NONE',  ( -11.28893270251630021, 1471.181900745179746, 207.4356590764699888 ) ) ;
#32883=CARTESIAN_POINT ( 'NONE',  ( -5.592450460805372003, 1508.275704380422212, 220.2479065938019573 ) ) ;
#32885=CARTESIAN_POINT ( 'NONE',  ( -2.409034624560000282, 1512.051704408390151, 204.7134966871890072 ) ) ;
#32887=CARTESIAN_POINT ( 'NONE',  ( -14.20981681145070041, 1419.004817284329874, 200.1611811227300279 ) ) ;
#32888=CARTESIAN_POINT ( 'NONE',  ( 3.206304093069999972, 1492.460538144390057, 188.3278363003989853 ) ) ;
#32889=CARTESIAN_POINT ( 'NONE',  ( 4.709520687179999499, 1480.407452823689937, 228.9869292435990076 ) ) ;
#32893=CARTESIAN_POINT ( 'NONE',  ( -15.31790971930000111, 1507.704306114589826, 209.3792549816630242 ) ) ;
#32894=CARTESIAN_POINT ( 'NONE',  ( 7.854266064069999942, 1423.715025901959962, 195.8676021965990230 ) ) ;
#32895=CARTESIAN_POINT ( 'NONE',  ( -1966.210325831229966, 11216.44053380570040, -21.67665461820280015 ) ) ;
#32899=CARTESIAN_POINT ( 'NONE',  ( -4.217997304759999899, 1515.470303964289997, 208.3798484374839859 ) ) ;
#32905=CARTESIAN_POINT ( 'NONE',  ( 10.89683788740839887, 1490.584122941180112, 210.4541128349080168 ) ) ;
#32906=EDGE_CURVE ( 'NONE', #15707, #21322, #84533, .T. ) ;
#32907=CARTESIAN_POINT ( 'NONE',  ( 1.538502245710000160, 1455.675329834489958, 218.5739180266590154 ) ) ;
#32911=EDGE_CURVE ( 'NONE', #76707, #29958, #35170, .T. ) ;
#32912=CARTESIAN_POINT ( 'NONE',  ( 4.987078442593329441, 1508.551704408389924, 206.6339108768089829 ) ) ;
#32913=ORIENTED_EDGE ( 'NONE', *, *, #61460, .T. ) ;
#32916=FACE_OUTER_BOUND ( 'NONE', #6822, .T. ) ;
#32917=CARTESIAN_POINT ( 'NONE',  ( -4.082779675200169933, 1515.071395204220153, 205.5354858456919942 ) ) ;
#32919=CARTESIAN_POINT ( 'NONE',  ( 3.092979971720000165, 1469.622821628089923, 189.3242126552989930 ) ) ;
#32921=CARTESIAN_POINT ( 'NONE',  ( -8.728835042969999236, 1462.533594714489936, 204.2920097199789780 ) ) ;
#32924=B_SPLINE_CURVE_WITH_KNOTS ( 'NONE', 3,
 ( #14318, #31128, #6484, #107839, #64210, #23271, #74265, #30019, #21056, #38967, #13209, #31678, #14868, #55815, #39540, #40636, #47942, #82647, #74808, #89393, #99978, #48509, #90483, #4822, #40085, #91031, #5939, #65859, #30583, #56351, #83196, #13758, #108952, #63666, #55261, #97780, #46862, #80992, #4298, #38425, #72601, #106729, #98333 ),
 .UNSPECIFIED., .F., .F.,
 ( 4, 3, 3, 3, 3, 3, 3, 3, 3, 3, 3, 3, 3, 3, 4 ),
 ( 3.966820340228049968, 5.122032127245899957, 6.221263424738429748, 7.257200153960000399, 8.081244681909998562, 8.905289209860001165, 9.318356587769999422, 10.01723044449550137, 10.55754830240000075, 11.31812075668910111, 12.00342336190689885, 12.22175150850000058, 12.83982335616149939, 13.41885480076430071, 13.57487840009213897 ),
 .UNSPECIFIED. ) ;
#32926=CARTESIAN_POINT ( 'NONE',  ( -16.05960259768179910, 1508.551704408389924, 213.7616175704369823 ) ) ;
#32937=CARTESIAN_POINT ( 'NONE',  ( -4.552706710259999845, 1475.816573717389929, 203.2240324946190242 ) ) ;
#32941=CARTESIAN_POINT ( 'NONE',  ( -3.072927222099999689, 1475.870007387389933, 199.1238673863090014 ) ) ;
#32947=CARTESIAN_POINT ( 'NONE',  ( 2.907323806750489847, 1428.844561383579958, 216.8721538760840133 ) ) ;
#32948=CARTESIAN_POINT ( 'NONE',  ( -1.843107666119999877, 1444.183210091189949, 199.2363500995090249 ) ) ;
#32949=EDGE_CURVE ( 'NONE', #89343, #69095, #45151, .T. ) ;
#32952=CARTESIAN_POINT ( 'NONE',  ( 4.082703447780033024, 1515.071394417502688, 205.5355069181578358 ) ) ;
#32953=CARTESIAN_POINT ( 'NONE',  ( 7.430468893321169332, 1426.189551463749922, 212.4985856753800135 ) ) ;
#32954=EDGE_CURVE ( 'NONE', #32988, #61245, #80557, .T. ) ;
#32956=EDGE_LOOP ( 'NONE', ( #73074, #13175, #20956, #10272 ) ) ;
#32958=CARTESIAN_POINT ( 'NONE',  ( -11.30037463203350079, 1491.719108927019988, 206.9447153815449951 ) ) ;
#32960=CARTESIAN_POINT ( 'NONE',  ( -19.75595483460000068, 1465.302321228290111, 208.1554333590609929 ) ) ;
#32965=ORIENTED_EDGE ( 'NONE', *, *, #95240, .F. ) ;
#32969=ORIENTED_EDGE ( 'NONE', *, *, #85138, .F. ) ;
#32977=CARTESIAN_POINT ( 'NONE',  ( 4.487359766195160304, 1509.034536885679927, 212.2379737843340024 ) ) ;
#32981=EDGE_CURVE ( 'NONE', #109119, #59235, #77266, .T. ) ;
#32988=VERTEX_POINT ( 'NONE', #62126 ) ;
#32989=DIRECTION ( 'NONE',  ( 0.9989456101410736366, 0.04590932679840484254, 4.114359441837505869E-05 ) ) ;
#32991=CARTESIAN_POINT ( 'NONE',  ( -4.650616333688489590, 1508.551704408389924, 212.8644526986900019 ) ) ;
#32993=CARTESIAN_POINT ( 'NONE',  ( 7.524255332260000095, 1421.856213011689988, 195.6731416337989913 ) ) ;
#32994=CARTESIAN_POINT ( 'NONE',  ( 0.7135751966820839121, 1431.574231143599945, 218.5858100304659786 ) ) ;
#32996=CARTESIAN_POINT ( 'NONE',  ( 10.37029593331170041, 1479.421151158329849, 205.9993793812860190 ) ) ;
#33000=CARTESIAN_POINT ( 'NONE',  ( -3.263114576272079827E-31, 1414.677402202029953, 209.1218459616989946 ) ) ;
#33001=CARTESIAN_POINT ( 'NONE',  ( 11.64198556425840003, 1426.536525572139908, 206.5273548246410087 ) ) ;
#33013=CARTESIAN_POINT ( 'NONE',  ( 9.490676817001279630, 1424.811928784230076, 209.0801198070559792 ) ) ;
#33014=CARTESIAN_POINT ( 'NONE',  ( 12.24717007643060107, 1426.243361053459921, 202.7748164033999956 ) ) ;
#33015=CARTESIAN_POINT ( 'NONE',  ( -10.83720256795320047, 1462.826867853169915, 206.9403819536609888 ) ) ;
#33017=EDGE_CURVE ( 'NONE', #9541, #56950, #8374, .T. ) ;
#33021=B_SPLINE_SURFACE_WITH_KNOTS ( 'NONE', 5, 5, ( 
 ( #100880, #24174, #94144, #34248, #58362, #92487 ),
 ( #15757, #33683, #42655, #49958, #42108, #7395 ),
 ( #76809, #76255, #41560, #75715, #16317, #68431 ),
 ( #50518, #84642, #102533, #67877, #25825, #43217 ),
 ( #77367, #668, #66234, #100353, #34799, #79036 ),
 ( #1218, #88522, #2337, #35916, #10715, #54389 ),
 ( #79578, #96924, #18525, #69540, #94704, #44886 ),
 ( #87419, #11807, #19644, #35353, #53847, #68987 ),
 ( #20191, #60583, #52722, #80110, #87984, #96365 ) ),
 .UNSPECIFIED., .F., .F., .F.,
 ( 6, 3, 6 ),
 ( 6, 6 ),
 ( 8.898683856529999048, 17.98737357839999973, 25.59366590640000183 ),
 ( 0.000000000000000000, 2.000000000000000000 ),
 .UNSPECIFIED. ) ;
#33024=CARTESIAN_POINT ( 'NONE',  ( 8.573315781209160491, 1422.682987794119981, 197.1461458239759850 ) ) ;
#33025=CARTESIAN_POINT ( 'NONE',  ( 9.619266338924012061, 1463.334782415319978, 214.5539088362909865 ) ) ;
#33026=CARTESIAN_POINT ( 'NONE',  ( -11.41675697748640061, 1482.775670443970057, 205.7339590229720159 ) ) ;
#33028=LINE ( 'NONE', #23527, #71410 ) ;
#33030=CARTESIAN_POINT ( 'NONE',  ( 0.7266811281859989480, 1473.184386469690025, 216.5181916793989956 ) ) ;
#33035=EDGE_CURVE ( 'NONE', #27986, #61245, #91149, .T. ) ;
#33036=CARTESIAN_POINT ( 'NONE',  ( -17.51543816364580053, 1417.552355716799866, 206.7803260042529701 ) ) ;
#33038=CARTESIAN_POINT ( 'NONE',  ( -9.278582903680890226, 1424.431248859760217, 204.6907556553629774 ) ) ;
#33049=CARTESIAN_POINT ( 'NONE',  ( -1.024097229660000163, 1484.039857070089965, 198.4653328332990156 ) ) ;
#33051=CARTESIAN_POINT ( 'NONE',  ( 10.03326978499999989, 1480.064307681189803, 205.9776673489490122 ) ) ;
#33054=CARTESIAN_POINT ( 'NONE',  ( -8.569414462087090456, 1437.093887118070143, 211.2561754816580049 ) ) ;
#33062=CARTESIAN_POINT ( 'NONE',  ( 11.90624125940899880, 1421.888678172720120, 209.0552753088340125 ) ) ;
#33065=EDGE_CURVE ( 'NONE', #67895, #94689, #47508, .T. ) ;
#33069=CARTESIAN_POINT ( 'NONE',  ( 5.586191088959999718, 1473.645535070089863, 218.5932301067289814 ) ) ;
#33072=CARTESIAN_POINT ( 'NONE',  ( -10.49051443589999977, 1493.796478401889999, 205.2036621587689922 ) ) ;
#33082=CARTESIAN_POINT ( 'NONE',  ( 0.1599736409740009913, 1457.268902431789911, 199.5796105822190043 ) ) ;
#33093=ORIENTED_EDGE ( 'NONE', *, *, #97304, .T. ) ;
#33102=CARTESIAN_POINT ( 'NONE',  ( 9.659057376369998948, 1477.882669201989984, 202.4105350377390096 ) ) ;
#33108=CARTESIAN_POINT ( 'NONE',  ( -18.47518245119999847, 1466.235720591789914, 200.8822878489689856 ) ) ;
#33113=CARTESIAN_POINT ( 'NONE',  ( -0.9532864999229999636, 1432.163584394390000, 203.4075515145090094 ) ) ;
#33114=CARTESIAN_POINT ( 'NONE',  ( 10.55262952197939974, 1452.742582998889930, 209.9734261203599885 ) ) ;
#33115=CARTESIAN_POINT ( 'NONE',  ( -4.535342621894029591, 1507.667936859109886, 221.1848183489019846 ) ) ;
#33116=CARTESIAN_POINT ( 'NONE',  ( 2.157536728407475568, 1397.913060387289988, 207.9431782750405659 ) ) ;
#33133=CARTESIAN_POINT ( 'NONE',  ( 5.805275416047459558, 1429.751446996589948, 216.6272687077410239 ) ) ;
#33135=CARTESIAN_POINT ( 'NONE',  ( -7.166932940584959333, 1489.833104379089491, 217.3880470055029264 ) ) ;
#33137=CARTESIAN_POINT ( 'NONE',  ( 9.924145419382540467, 1468.837275789919886, 207.5733661434399835 ) ) ;
#33138=CARTESIAN_POINT ( 'NONE',  ( -10.29442985670006117, 1469.837443877088390, 213.9189782992590665 ) ) ;
#33142=CARTESIAN_POINT ( 'NONE',  ( -20.77679319119999946, 1505.353396285190229, 209.2699052164729778 ) ) ;
#33143=CARTESIAN_POINT ( 'NONE',  ( 5.576745036960350177, 1467.101830086349992, 199.5044134152479955 ) ) ;
#33144=FACE_OUTER_BOUND ( 'NONE', #62225, .T. ) ;
#33146=B_SPLINE_SURFACE_WITH_KNOTS ( 'NONE', 5, 1, ( 
 ( #95921, #97576 ),
 ( #98109, #61800 ),
 ( #71873, #46094 ),
 ( #80778, #3544 ),
 ( #106523, #1889 ),
 ( #63998, #29265 ) ),
 .UNSPECIFIED., .F., .F., .F.,
 ( 6, 6 ),
 ( 2, 2 ),
 ( 0.000000000000000000, 3.864159766120000228 ),
 ( 0.000000000000000000, 14.00000000000000000 ),
 .UNSPECIFIED. ) ;
#33154=CARTESIAN_POINT ( 'NONE',  ( -11.51256439133040033, 1501.104924895310205, 211.2032020787609952 ) ) ;
#33157=CARTESIAN_POINT ( 'NONE',  ( -1.563447624619999976, 1508.551704408389924, 220.3217919041989887 ) ) ;
#33163=CARTESIAN_POINT ( 'NONE',  ( -6.198495147294970309, 1426.943711827879952, 202.1453469996679928 ) ) ;
#33178=CARTESIAN_POINT ( 'NONE',  ( -14.56536539080000026, 1417.270466440329983, 203.6292502051090025 ) ) ;
#33181=B_SPLINE_SURFACE_WITH_KNOTS ( 'NONE', 5, 1, ( 
 ( #83198, #74268 ),
 ( #92145, #56901 ),
 ( #101622, #73717 ),
 ( #32782, #99981 ),
 ( #108955, #14321 ),
 ( #58010, #58560 ) ),
 .UNSPECIFIED., .F., .F., .F.,
 ( 6, 6 ),
 ( 2, 2 ),
 ( 0.000000000000000000, 15.56462730289999996 ),
 ( 0.000000000000000000, 14.00000000000000000 ),
 .UNSPECIFIED. ) ;
#33182=CARTESIAN_POINT ( 'NONE',  ( -17.33706400627729138, 1419.403770296549055, 207.7192493357346450 ) ) ;
#33184=EDGE_CURVE ( 'NONE', #19773, #77131, #78961, .T. ) ;
#33187=CARTESIAN_POINT ( 'NONE',  ( -11.50563130876499862, 1508.158931577909925, 207.5673837874410026 ) ) ;
#33200=CARTESIAN_POINT ( 'NONE',  ( -2.302358205752170317, 1507.635233240290063, 221.1829251670985741 ) ) ;
#33204=CARTESIAN_POINT ( 'NONE',  ( 12.47858532031530032, 1421.602759672520051, 207.4039838217449869 ) ) ;
#33205=CARTESIAN_POINT ( 'NONE',  ( 10.38589783937220012, 1479.770266300000003, 206.7566811546030010 ) ) ;
#33206=FACE_OUTER_BOUND ( 'NONE', #90712, .T. ) ;
#33207=CARTESIAN_POINT ( 'NONE',  ( 4.677539293532180231, 1434.888973739250105, 228.7640143593589812 ) ) ;
#33210=CARTESIAN_POINT ( 'NONE',  ( -20.36853080836219831, 1464.956632874939942, 210.9458194777220115 ) ) ;
#33211=CARTESIAN_POINT ( 'NONE',  ( -16.17592491924940035, 1416.577882651939944, 209.2335455203370032 ) ) ;
#33212=CARTESIAN_POINT ( 'NONE',  ( -2.487935118526678480, 1508.884207228051082, 204.6305528479420843 ) ) ;
#33216=CARTESIAN_POINT ( 'NONE',  ( -1.920602012799999869, 1420.567466289690174, 193.8392733480989989 ) ) ;
#33220=FACE_OUTER_BOUND ( 'NONE', #91897, .T. ) ;
#33235=CARTESIAN_POINT ( 'NONE',  ( 1.285642914329999886, 1444.921654895390020, 199.8418900409189973 ) ) ;
#33242=CARTESIAN_POINT ( 'NONE',  ( 10.65114734267110030, 1480.262814529339948, 208.4911516818010284 ) ) ;
#33255=CARTESIAN_POINT ( 'NONE',  ( -11.92155900329999874, 1502.317141431590017, 208.8109435272550058 ) ) ;
#33270=CARTESIAN_POINT ( 'NONE',  ( -16.31523981255880074, 1508.551704408389924, 210.3829298100710048 ) ) ;
#33274=CARTESIAN_POINT ( 'NONE',  ( -2.543708339781890260, 1429.172938267450036, 200.1013465518929877 ) ) ;
#33279=CARTESIAN_POINT ( 'NONE',  ( 9.710109577146511128, 1434.985020983699997, 207.7973431748550013 ) ) ;
#33283=VERTEX_POINT ( 'NONE', #41849 ) ;
#33288=CARTESIAN_POINT ( 'NONE',  ( 7.799999999999999822, 1412.913060387329779, 209.1218459616989946 ) ) ;
#33290=CARTESIAN_POINT ( 'NONE',  ( 4.987078416198220232, 1508.551704408389924, 211.6097810847190033 ) ) ;
#33293=CARTESIAN_POINT ( 'NONE',  ( -9.190572780844979306, 1449.577780504580005, 209.0393402580440068 ) ) ;
#33300=CARTESIAN_POINT ( 'NONE',  ( -9.124411009920782689, 1461.277107961660022, 205.8277251432190837 ) ) ;
#33301=CARTESIAN_POINT ( 'NONE',  ( 4.334458048930000196, 1466.050308755590095, 219.2818749650989787 ) ) ;
#33307=ADVANCED_FACE ( 'NONE', ( #84938 ), #1675, .F. ) ;
#33309=CARTESIAN_POINT ( 'NONE',  ( 4.704564003757560009, 1507.026338954369976, 219.8246688803149880 ) ) ;
#33314=DIRECTION ( 'NONE',  ( -0.8393249826168291960, -0.3829000781212070215, -0.3859029719113770129 ) ) ;
#33316=CARTESIAN_POINT ( 'NONE',  ( 11.46786347449999965, 1502.092859008989990, 211.0284006470890006 ) ) ;
#33318=CARTESIAN_POINT ( 'NONE',  ( -9.831691212836640048, 1438.525609616689962, 210.5507346167850073 ) ) ;
#33321=PLANE ( 'NONE',  #34257 ) ;
#33327=ORIENTED_EDGE ( 'NONE', *, *, #2899, .T. ) ;
#33332=ORIENTED_EDGE ( 'NONE', *, *, #11217, .T. ) ;
#33333=CARTESIAN_POINT ( 'NONE',  ( 4.208240993269999564, 1434.939300248989866, 227.0651965576989824 ) ) ;
#33335=CARTESIAN_POINT ( 'NONE',  ( 4.301794564619999761, 1454.418299454290036, 217.4807569431989975 ) ) ;
#33337=CARTESIAN_POINT ( 'NONE',  ( -7.305751433210000201, 1447.589639846790078, 214.8024071067289924 ) ) ;
#33342=CARTESIAN_POINT ( 'NONE',  ( 7.346975979479999808, 1425.060309264630177, 212.5630391892889861 ) ) ;
#33359=FACE_OUTER_BOUND ( 'NONE', #49634, .T. ) ;
#33363=CARTESIAN_POINT ( 'NONE',  ( -8.662982322953059366, 1448.248813715330016, 211.9993685260630230 ) ) ;
#33369=ORIENTED_EDGE ( 'NONE', *, *, #950, .T. ) ;
#33375=EDGE_LOOP ( 'NONE', ( #33434, #1191, #106655, #11382 ) ) ;
#33388=CARTESIAN_POINT ( 'NONE',  ( 2.236830499208590339, 1495.676457082710158, 221.2569898128769807 ) ) ;
#33395=CARTESIAN_POINT ( 'NONE',  ( -5.970282146669999790, 1449.727869094690050, 209.8750552241949947 ) ) ;
#33400=CARTESIAN_POINT ( 'NONE',  ( -10.79543140439999860, 1471.481918345589975, 207.1280613816090010 ) ) ;
#33403=PLANE ( 'NONE',  #30194 ) ;
#33408=CARTESIAN_POINT ( 'NONE',  ( 9.702207697720000468, 1489.235137281590141, 203.6117652758089775 ) ) ;
#33412=CARTESIAN_POINT ( 'NONE',  ( -4.487249775048080203, 1509.038615934839981, 211.6097811040130239 ) ) ;
#33417=CARTESIAN_POINT ( 'NONE',  ( -16.54305653649999641, 1420.580047969900079, 203.3927685990690009 ) ) ;
#33418=ORIENTED_EDGE ( 'NONE', *, *, #11184, .F. ) ;
#33424=CARTESIAN_POINT ( 'NONE',  ( -5.066920007859089914, 1508.235255472309291, 220.4033713207047924 ) ) ;
#33430=CARTESIAN_POINT ( 'NONE',  ( -10.55936701243939879, 1471.180347189670101, 209.5615340540499858 ) ) ;
#33434=ORIENTED_EDGE ( 'NONE', *, *, #44069, .T. ) ;
#33439=CARTESIAN_POINT ( 'NONE',  ( 9.651066088509999474, 1425.440658930580184, 195.4941615409990163 ) ) ;
#33441=CARTESIAN_POINT ( 'NONE',  ( 9.971732002342131196, 1422.489342820810180, 212.1848988156249902 ) ) ;
#33444=CARTESIAN_POINT ( 'NONE',  ( 10.37959279779999910, 1453.090483345690018, 190.0119662633989890 ) ) ;
#33448=CARTESIAN_POINT ( 'NONE',  ( 11.44464715210460071, 1491.838548702460230, 209.9183825457590160 ) ) ;
#33449=CARTESIAN_POINT ( 'NONE',  ( -2.280001584889999933, 1457.248781993690045, 218.7633449024490062 ) ) ;
#33450=ORIENTED_EDGE ( 'NONE', *, *, #108159, .F. ) ;
#33453=CARTESIAN_POINT ( 'NONE',  ( -3.100192419969999946, 1431.506313241990028, 216.9304414810590060 ) ) ;
#33456=DIRECTION ( 'NONE',  ( 0.000000000000000000, -0.02617694830808806397, 0.9996573249755517088 ) ) ;
#33460=CARTESIAN_POINT ( 'NONE',  ( -9.771542533679999920, 1462.553261080089896, 206.2413439940889930 ) ) ;
#33461=AXIS2_PLACEMENT_3D ( 'NONE', #31645, #16473, #33850 ) ;
#33465=CARTESIAN_POINT ( 'NONE',  ( -10.41491974136950027, 1508.551704408389924, 218.0827215060540141 ) ) ;
#33468=CARTESIAN_POINT ( 'NONE',  ( -0.4061581754453899573, 1486.016806840350000, 197.2250015105809950 ) ) ;
#33474=CARTESIAN_POINT ( 'NONE',  ( -2.953102495588340481, 1470.057161604909879, 187.4194597744339887 ) ) ;
#33480=CARTESIAN_POINT ( 'NONE',  ( -12.78494549719999895, 1502.727917388590186, 208.9468085136539912 ) ) ;
#33481=CARTESIAN_POINT ( 'NONE',  ( -13.59512407998240135, 1507.703338069740084, 209.3532897553030239 ) ) ;
#33482=CARTESIAN_POINT ( 'NONE',  ( -20.17395953629999994, 1505.644431352489846, 209.1238650338669913 ) ) ;
#33483=CARTESIAN_POINT ( 'NONE',  ( -1.886715933359999875, 1476.714922781289943, 198.9125049787990065 ) ) ;
#33488=CARTESIAN_POINT ( 'NONE',  ( 3.085209382068490047, 1428.771282319309876, 216.8020061943259975 ) ) ;
#33489=CARTESIAN_POINT ( 'NONE',  ( -7.544801320229999497, 1425.914425209869933, 205.6925056590089866 ) ) ;
#33494=CARTESIAN_POINT ( 'NONE',  ( 7.461100860251050015, 1426.110972386630010, 212.4219345183129803 ) ) ;
#33500=CARTESIAN_POINT ( 'NONE',  ( -6.403692060479999171, 1460.996305860290249, 208.5086931504900178 ) ) ;
#33501=CARTESIAN_POINT ( 'NONE',  ( -3.984081755090763011, 1515.551704407335137, 207.2788837462810534 ) ) ;
#33502=CARTESIAN_POINT ( 'NONE',  ( 3.552717040180000119, 1420.594650159299817, 205.3542343418889971 ) ) ;
#33510=EDGE_LOOP ( 'NONE', ( #89919, #98645, #5857, #67774, #761, #31685 ) ) ;
#33518=EDGE_CURVE ( 'NONE', #63746, #21533, #79218, .T. ) ;
#33529=CARTESIAN_POINT ( 'NONE',  ( -11.60381925561519800, 1481.105444724209974, 211.4046900983030071 ) ) ;
#33530=EDGE_CURVE ( 'NONE', #88484, #106272, #5833, .T. ) ;
#33533=CARTESIAN_POINT ( 'NONE',  ( -4.206093650348769586, 1508.551704408389924, 213.4237127473219857 ) ) ;
#33535=CARTESIAN_POINT ( 'NONE',  ( 7.372986420420000186, 1422.271846737719898, 195.5865301424989866 ) ) ;
#33536=CARTESIAN_POINT ( 'NONE',  ( -1.578050994240060012, 1432.480027970319952, 218.5065461788099981 ) ) ;
#33537=CARTESIAN_POINT ( 'NONE',  ( -4.396663909700000872, 1496.560935200589938, 198.7783260529990059 ) ) ;
#33550=CARTESIAN_POINT ( 'NONE',  ( -10.38271356220340103, 1483.373521473610026, 203.2896237654969980 ) ) ;
#33552=CARTESIAN_POINT ( 'NONE',  ( 8.729815835326180107, 1423.787549604110154, 211.0527875084169978 ) ) ;
#33554=CARTESIAN_POINT ( 'NONE',  ( 11.00321081153069969, 1423.193864714949996, 203.2865044889030059 ) ) ;
#33555=B_SPLINE_CURVE_WITH_KNOTS ( 'NONE', 5,
 ( #20826, #19158, #29245, #37090, #96454, #40253 ),
 .UNSPECIFIED., .F., .F.,
 ( 6, 6 ),
 ( 0.000000000000000000, 1.000000000000000000 ),
 .UNSPECIFIED. ) ;
#33556=CARTESIAN_POINT ( 'NONE',  ( 1.338019556329999915, 1431.361302696190023, 218.5179664551590122 ) ) ;
#33565=CARTESIAN_POINT ( 'NONE',  ( 9.076018398308100643, 1424.724030148510110, 196.5059690868249902 ) ) ;
#33567=CARTESIAN_POINT ( 'NONE',  ( 9.777144235831070063, 1463.043760913599954, 213.2472973885180068 ) ) ;
#33573=CARTESIAN_POINT ( 'NONE',  ( -0.2116227187891456529, 1477.625743691535718, 198.7159279415461697 ) ) ;
#33576=CARTESIAN_POINT ( 'NONE',  ( 12.75035444685179975, 1426.659570474229895, 203.9315474661299845 ) ) ;
#33577=CARTESIAN_POINT ( 'NONE',  ( 18.99431337219000326, 1459.501208559760016, 220.3864240110139860 ) ) ;
#33579=CARTESIAN_POINT ( 'NONE',  ( -13.24697265328699913, 1421.521121240300090, 208.1594402398530121 ) ) ;
#33589=CARTESIAN_POINT ( 'NONE',  ( -10.94922717770000098, 1470.861560407889783, 209.5255082979219878 ) ) ;
#33590=CARTESIAN_POINT ( 'NONE',  ( 10.47956906020000112, 1478.583002912489974, 204.7952642272489925 ) ) ;
#33592=CARTESIAN_POINT ( 'NONE',  ( 8.212352435486090840, 1503.127186295949969, 210.4119011823910057 ) ) ;
#33593=CARTESIAN_POINT ( 'NONE',  ( 6.250429024355669938, 1467.523505036979941, 206.1081765850969987 ) ) ;
#33596=CARTESIAN_POINT ( 'NONE',  ( -16.21478424889999559, 1417.659049898350077, 209.2181137195750296 ) ) ;
#33601=CARTESIAN_POINT ( 'NONE',  ( 10.86658986439489816, 1422.901391916879902, 206.8975148066129748 ) ) ;
#33607=CARTESIAN_POINT ( 'NONE',  ( 0.000000000000000000, 1516.051704408390151, 209.1218459616989946 ) ) ;
#33610=CARTESIAN_POINT ( 'NONE',  ( -10.73077433369999945, 1492.937000258489888, 206.1586420614789859 ) ) ;
#33614=CARTESIAN_POINT ( 'NONE',  ( -10855.50032577649290, 5181.793945261120825, 7511.881964575620259 ) ) ;
#33619=CARTESIAN_POINT ( 'NONE',  ( -9.105994434067794074, 1449.807959746201050, 207.8187243124739041 ) ) ;
#33620=ADVANCED_FACE ( 'NONE', ( #52360 ), #6162, .T. ) ;
#33622=AXIS2_PLACEMENT_3D ( 'NONE', #27145, #18713, #45071 ) ;
#33645=CARTESIAN_POINT ( 'NONE',  ( 2.843730423744790237, 1508.551704408389924, 214.0849298366779863 ) ) ;
#33650=CARTESIAN_POINT ( 'NONE',  ( 9.694462811961930271, 1462.254523745029928, 208.2086536884339978 ) ) ;
#33654=CARTESIAN_POINT ( 'NONE',  ( 1.121604517039999971, 1425.801401066219796, 191.0761181822990125 ) ) ;
#33660=CARTESIAN_POINT ( 'NONE',  ( 3.829620113550000315, 1515.551704408389924, 210.9648081929590262 ) ) ;
#33665=CARTESIAN_POINT ( 'NONE',  ( 9.218353480593270532, 1451.410954820720008, 210.0417286664930145 ) ) ;
#33679=CARTESIAN_POINT ( 'NONE',  ( -7.472882595364333191, 1434.765136914032610, 213.3156276624751229 ) ) ;
#33680=CARTESIAN_POINT ( 'NONE',  ( -6.351474700609002433, 1489.557796261735803, 218.0707846636206853 ) ) ;
#33683=CARTESIAN_POINT ( 'NONE',  ( -9.864626116910001130, 1473.082391558989912, 206.3028941057989982 ) ) ;
#33688=CARTESIAN_POINT ( 'NONE',  ( -5.387811863060000483, 1496.648312753189884, 199.2595355468089906 ) ) ;
#33689=CARTESIAN_POINT ( 'NONE',  ( 3.383995498396490387, 1466.337167523709923, 198.5968663170720276 ) ) ;
#33698=CARTESIAN_POINT ( 'NONE',  ( -14.68224860129999954, 1415.739699861750069, 213.1708190345090088 ) ) ;
#33699=CARTESIAN_POINT ( 'NONE',  ( -4.138543391158297169, 1515.492058413688255, 211.4519800883778373 ) ) ;
#33702=CARTESIAN_POINT ( 'NONE',  ( 0.7310778633389990455, 1508.461242302289975, 220.4858708957989961 ) ) ;
#33708=CARTESIAN_POINT ( 'NONE',  ( 21.13734888319999783, 1496.938803861589804, 209.1218459616989946 ) ) ;
#33709=EDGE_CURVE ( 'NONE', #20056, #28187, #85943, .T. ) ;
#33712=CARTESIAN_POINT ( 'NONE',  ( -10.48474031351270064, 1480.275052362939959, 208.2232303084710168 ) ) ;
#33714=ORIENTED_EDGE ( 'NONE', *, *, #68020, .F. ) ;
#33723=CARTESIAN_POINT ( 'NONE',  ( 2.588318195730309856, 1454.459320507460006, 218.1543517672069754 ) ) ;
#33724=CARTESIAN_POINT ( 'NONE',  ( -15.85591190879999779, 1415.880081504350073, 209.4912631162540038 ) ) ;
#33726=CARTESIAN_POINT ( 'NONE',  ( -10.04630323299999972, 1461.008343231690105, 213.6807241916089879 ) ) ;
#33728=CARTESIAN_POINT ( 'NONE',  ( -3.805396659119999914, 1495.647976226690162, 219.6495707272989932 ) ) ;
#33729=CARTESIAN_POINT ( 'NONE',  ( -8.638504774626840188, 1437.522490713840170, 208.5429851243989958 ) ) ;
#33733=CARTESIAN_POINT ( 'NONE',  ( -1.842962231260000028, 1515.064792882589927, 213.4512947377390049 ) ) ;
#33750=CARTESIAN_POINT ( 'NONE',  ( 4.825596943430000785, 1484.194153470290075, 219.9364766577990054 ) ) ;
#33753=CARTESIAN_POINT ( 'NONE',  ( -19.04698835603899809, 1444.155774679960132, 199.5979800297200200 ) ) ;
#33754=CARTESIAN_POINT ( 'NONE',  ( -3.829619994797929916, 1515.551704292389786, 210.9648097401420159 ) ) ;
#33761=CARTESIAN_POINT ( 'NONE',  ( 4.616666844463280128, 1447.066147660239949, 200.0483904391570036 ) ) ;
#33775=EDGE_LOOP ( 'NONE', ( #74056, #26478, #108291, #70463, #16830 ) ) ;
#33778=EDGE_LOOP ( 'NONE', ( #71547, #37546, #50488, #16699, #9439, #30339 ) ) ;
#33781=CARTESIAN_POINT ( 'NONE',  ( 3.644351594699349661, 1515.551704204689941, 205.8497219879369879 ) ) ;
#33785=VECTOR ( 'NONE', #59283, 1000.000000000000000 ) ;
#33807=CARTESIAN_POINT ( 'NONE',  ( 12.33374228401319961, 1421.685547970650077, 207.8899185667679888 ) ) ;
#33815=ADVANCED_FACE ( 'NONE', ( #81788 ), #15097, .T. ) ;
#33817=B_SPLINE_CURVE_WITH_KNOTS ( 'NONE', 5,
 ( #20273, #1862, #46066, #89145, #2969, #19731 ),
 .UNSPECIFIED., .F., .F.,
 ( 6, 6 ),
 ( 0.000000000000000000, 1.000000000000000000 ),
 .UNSPECIFIED. ) ;
#33821=EDGE_LOOP ( 'NONE', ( #32913, #6803, #71895, #109249 ) ) ;
#33824=CARTESIAN_POINT ( 'NONE',  ( -3.829620113550000315, 1515.551704408389924, 207.2788837304390199 ) ) ;
#33826=ADVANCED_FACE ( 'NONE', ( #25597 ), #50941, .F. ) ;
#33832=CARTESIAN_POINT ( 'NONE',  ( -3.253889150190400148, 1428.778859686050055, 200.3401300163330063 ) ) ;
#33837=CARTESIAN_POINT ( 'NONE',  ( -11.86441352026110074, 1482.079730296919934, 208.3752912375910284 ) ) ;
#33846=CARTESIAN_POINT ( 'NONE',  ( 12.45662329989999861, 1427.088120873819889, 206.6493142630589830 ) ) ;
#33850=DIRECTION ( 'NONE',  ( -1.000000000000000000, 0.000000000000000000, 0.000000000000000000 ) ) ;
#33851=CARTESIAN_POINT ( 'NONE',  ( -1.550613577669627485, 1515.551704304084296, 205.2291798131859935 ) ) ;
#33854=CARTESIAN_POINT ( 'NONE',  ( -8.654560031179620694, 1508.432825899400086, 219.2516281120300050 ) ) ;
#33856=CARTESIAN_POINT ( 'NONE',  ( 4.987078416198220232, 1508.551704408389924, 211.6097810847190033 ) ) ;
#33858=CARTESIAN_POINT ( 'NONE',  ( 10.94310694154670038, 1460.970394390260026, 208.7352916610030320 ) ) ;
#33859=CARTESIAN_POINT ( 'NONE',  ( -13.31089767776890120, 1503.456584347970193, 208.6977459380580058 ) ) ;
#33860=CARTESIAN_POINT ( 'NONE',  ( 3.869834123409999993, 1466.682401882589829, 218.6841892407390162 ) ) ;
#33868=CARTESIAN_POINT ( 'NONE',  ( -9.105545352350659982, 1449.059046520889979, 210.1350150939630055 ) ) ;
#33876=CARTESIAN_POINT ( 'NONE',  ( 12.26398290010000025, 1500.757830321889969, 209.2458525896959998 ) ) ;
#33877=CARTESIAN_POINT ( 'NONE',  ( -4.623067421070000016, 1470.601194648889987, 189.6761541078989808 ) ) ;
#33879=CARTESIAN_POINT ( 'NONE',  ( 7.565836366640000143, 1425.419877822159833, 211.6547584071689982 ) ) ;
#33890=CARTESIAN_POINT ( 'NONE',  ( -5.311724842150000292, 1500.891271500089942, 229.7588813323989996 ) ) ;
#33891=CARTESIAN_POINT ( 'NONE',  ( -15.49932866405858789, 1415.988126884580197, 207.5283249126204907 ) ) ;
#33894=CARTESIAN_POINT ( 'NONE',  ( -8.557208171940001051, 1448.617778667089851, 212.3361775886790213 ) ) ;
#33901=DIRECTION ( 'NONE',  ( -0.9243714516270737924, -0.3790700632520799807, -0.04293374620179828127 ) ) ;
#33902=CARTESIAN_POINT ( 'NONE',  ( 1.860632309006911456, 1494.734257013992419, 220.1210481096561580 ) ) ;
#33905=CARTESIAN_POINT ( 'NONE',  ( 2.236830499208590339, 1495.676457082710158, 221.2569898128769807 ) ) ;
#33912=DIRECTION ( 'NONE',  ( 0.06309892600015151731, -0.9660070198143602127, -0.2506969549216855886 ) ) ;
#33916=CARTESIAN_POINT ( 'NONE',  ( 2.326513286163319538, 1476.258183507229887, 197.8633931498989966 ) ) ;
#33920=CARTESIAN_POINT ( 'NONE',  ( -9.244740828173918956, 1448.612708514039923, 209.9868122805330017 ) ) ;
#33923=ORIENTED_EDGE ( 'NONE', *, *, #6332, .F. ) ;
#33928=EDGE_LOOP ( 'NONE', ( #56587, #38847, #83555, #72605, #57626, #41742, #46894, #49633 ) ) ;
#33930=CARTESIAN_POINT ( 'NONE',  ( -18.83642247210000065, 1444.248298674089938, 209.1218459616989946 ) ) ;
#33933=DIRECTION ( 'NONE',  ( -1.000000000000000000, 0.000000000000000000, 0.000000000000000000 ) ) ;
#33943=B_SPLINE_SURFACE_WITH_KNOTS ( 'NONE', 5, 1, ( 
 ( #23529, #39797 ),
 ( #29733, #73956 ),
 ( #99673, #91294 ),
 ( #22965, #57172 ),
 ( #82891, #6182 ),
 ( #40335, #74516 ) ),
 .UNSPECIFIED., .F., .F., .F.,
 ( 6, 6 ),
 ( 2, 2 ),
 ( 0.000000000000000000, 3.835535759499999919 ),
 ( 0.000000000000000000, 14.00000000000000000 ),
 .UNSPECIFIED. ) ;
#33950=ORIENTED_EDGE ( 'NONE', *, *, #94120, .F. ) ;
#33954=CARTESIAN_POINT ( 'NONE',  ( -6.031288452957631385, 1442.578928665805051, 201.0498015145549573 ) ) ;
#33960=CARTESIAN_POINT ( 'NONE',  ( 3.066583199566000534E-32, 1507.508085020990166, 209.1218459616989946 ) ) ;
#33963=EDGE_LOOP ( 'NONE', ( #96374, #24432, #52417, #80912, #64004, #85765, #19903, #65146 ) ) ;
#33969=CARTESIAN_POINT ( 'NONE',  ( -3.994937584009999654, 1430.106198397690150, 201.8091617978890042 ) ) ;
#33972=CARTESIAN_POINT ( 'NONE',  ( -6.929999671550000073, 1413.957734829029960, 207.7807066811290042 ) ) ;
#33974=CARTESIAN_POINT ( 'NONE',  ( 5.288836944179999833, 1486.626846567689881, 199.6980016761590093 ) ) ;
#33975=FACE_OUTER_BOUND ( 'NONE', #25684, .T. ) ;
#33979=CARTESIAN_POINT ( 'NONE',  ( -10.97132182545054846, 1448.375239271800638, 192.9928798521789304 ) ) ;
#33993=CARTESIAN_POINT ( 'NONE',  ( -11.24713962180850046, 1471.253631266729826, 207.1712745178000148 ) ) ;
#34000=CARTESIAN_POINT ( 'NONE',  ( -1.920586321285300047, 1420.567450626859909, 193.8392714366590326 ) ) ;
#34001=DIRECTION ( 'NONE',  ( 0.8774038027816709606, -0.3849049474659920200, 0.2863751879623379626 ) ) ;
#34032=VECTOR ( 'NONE', #106227, 1000.000000000000000 ) ;
#34033=CARTESIAN_POINT ( 'NONE',  ( -8.930212406729999941, 1461.403864792989907, 205.1993326667990232 ) ) ;
#34040=CARTESIAN_POINT ( 'NONE',  ( 1.248280726178319977, 1432.832982257020149, 200.7627227404510108 ) ) ;
#34046=CARTESIAN_POINT ( 'NONE',  ( 20.67523678790000119, 1478.097707044290019, 217.5712452575990028 ) ) ;
#34050=CARTESIAN_POINT ( 'NONE',  ( 3.066583199566000534E-32, 1507.508085020990166, 209.1218459616989946 ) ) ;
#34055=CARTESIAN_POINT ( 'NONE',  ( 0.8317469223220009811, 1476.953783366089965, 198.6245987969989812 ) ) ;
#34060=CARTESIAN_POINT ( 'NONE',  ( 0.7301090186228299528, 1429.703966172960008, 217.4049395672290075 ) ) ;
#34061=CARTESIAN_POINT ( 'NONE',  ( -7.604290685550000539, 1426.735974020640015, 206.0921002386889995 ) ) ;
#34066=B_SPLINE_SURFACE_WITH_KNOTS ( 'NONE', 5, 5, ( 
 ( #81516, #40083, #63129, #72074, #97231, #4820 ),
 ( #46316, #106727, #38423, #106189, #30581, #4295 ),
 ( #3759, #72598, #98881, #37891, #29472, #63664 ),
 ( #21054, #55258, #12680, #5381, #21608, #46860 ),
 ( #80989, #55813, #22148, #41191, #74263, #100534 ),
 ( #110596, #93236, #57465, #67516, #59659, #66417 ) ),
 .UNSPECIFIED., .F., .F., .F.,
 ( 6, 6 ),
 ( 6, 6 ),
 ( -1.600009832348449890E-05, 6.607489203828340152 ),
 ( -1.600009834268530264E-05, 2.000000000000000000 ),
 .UNSPECIFIED. ) ;
#34068=CARTESIAN_POINT ( 'NONE',  ( 7.474209936774370178, 1426.071330082020040, 212.3877608208809704 ) ) ;
#34080=ORIENTED_EDGE ( 'NONE', *, *, #74621, .F. ) ;
#34091=CARTESIAN_POINT ( 'NONE',  ( 4.556906905527969620, 1508.729448404669938, 212.2592272162939935 ) ) ;
#34099=CARTESIAN_POINT ( 'NONE',  ( -1.156571746234419829, 1444.424822986080017, 199.1343848052200087 ) ) ;
#34104=CARTESIAN_POINT ( 'NONE',  ( 5.589575339105699925, 1434.643108874500058, 202.6764547222993258 ) ) ;
#34106=CARTESIAN_POINT ( 'NONE',  ( -4.391179462891900087, 1508.551704408389924, 213.2284805894280169 ) ) ;
#34108=CARTESIAN_POINT ( 'NONE',  ( 7.549774212029999987, 1421.876882727210159, 195.6872530139989976 ) ) ;
#34109=CARTESIAN_POINT ( 'NONE',  ( -2.427052486703370260, 1432.867848442830109, 218.3435047856359859 ) ) ;
#34110=CARTESIAN_POINT ( 'NONE',  ( -3.467940584279999960, 1495.562067875890079, 197.2905559997990110 ) ) ;
#34124=CARTESIAN_POINT ( 'NONE',  ( 9.741659962066350431, 1422.546270596229988, 212.4615314579379799 ) ) ;
#34128=CARTESIAN_POINT ( 'NONE',  ( 1.124949149999999953, 1430.908435203989939, 217.7868727458690046 ) ) ;
#34136=B_SPLINE_CURVE_WITH_KNOTS ( 'NONE', 3,
 ( #91747, #49221, #83347, #109665, #40799, #74978, #76610, #109126, #32407, #15568 ),
 .UNSPECIFIED., .F., .F.,
 ( 4, 2, 2, 2, 4 ),
 ( 0.000000000000000000, 0.2499999999999998890, 0.4999999999999998890, 0.7499999999999998890, 1.000000000000000000 ),
 .UNSPECIFIED. ) ;
#34137=CARTESIAN_POINT ( 'NONE',  ( 10.53309060615429793, 1424.587086563600224, 199.9078566869370093 ) ) ;
#34138=CARTESIAN_POINT ( 'NONE',  ( 9.224637020051591918, 1464.192156177939978, 212.6135812687480211 ) ) ;
#34147=CARTESIAN_POINT ( 'NONE',  ( -1.485893011569999977, 1515.551703577890066, 205.2152226796090133 ) ) ;
#34149=CARTESIAN_POINT ( 'NONE',  ( -21.47379561725159647, 1487.892728963219952, 202.0847257228780052 ) ) ;
#34151=CARTESIAN_POINT ( 'NONE',  ( -21.23871617420000391, 1418.070708022229837, 210.0663963951400319 ) ) ;
#34154=ORIENTED_EDGE ( 'NONE', *, *, #35626, .F. ) ;
#34156=CARTESIAN_POINT ( 'NONE',  ( -12.09621839340030824, 1446.031655959586260, 193.6906851894976853 ) ) ;
#34160=ORIENTED_EDGE ( 'NONE', *, *, #10728, .F. ) ;
#34161=CARTESIAN_POINT ( 'NONE',  ( -10.57294294639999954, 1471.242314994889966, 209.3037664082490323 ) ) ;
#34163=CARTESIAN_POINT ( 'NONE',  ( 7.224377867204991865, 1447.376750353422722, 203.6098548312575929 ) ) ;
#34165=CARTESIAN_POINT ( 'NONE',  ( -8.498308697023119862, 1436.913760846189916, 212.4344101014090143 ) ) ;
#34172=CARTESIAN_POINT ( 'NONE',  ( 11.59960881601659999, 1426.963225802300030, 207.4389891066049927 ) ) ;
#34173=VERTEX_POINT ( 'NONE', #24906 ) ;
#34178=CARTESIAN_POINT ( 'NONE',  ( 5.242187580730000462, 1473.743341493890057, 218.7973554873690034 ) ) ;
#34180=CARTESIAN_POINT ( 'NONE',  ( 19.31452971239999883, 1455.192177364190002, 208.1916251275950174 ) ) ;
#34188=CARTESIAN_POINT ( 'NONE',  ( 5.981358413060000601, 1447.780665424890003, 201.2187644437790084 ) ) ;
#34197=CARTESIAN_POINT ( 'NONE',  ( -3.126045989589999685, 1496.690033224690069, 220.3233446123989836 ) ) ;
#34198=ORIENTED_EDGE ( 'NONE', *, *, #96968, .F. ) ;
#34212=CARTESIAN_POINT ( 'NONE',  ( 4.530018341142350025, 1508.551704408389924, 213.0522568375050128 ) ) ;
#34216=CARTESIAN_POINT ( 'NONE',  ( 10.76124213208149882, 1460.439160552989961, 207.1949203455349959 ) ) ;
#34220=CARTESIAN_POINT ( 'NONE',  ( -0.5698918850559979710, 1425.422772561009879, 191.0863376515989955 ) ) ;
#34224=CARTESIAN_POINT ( 'NONE',  ( -14.20525283303160080, 1416.384016890880048, 203.1489016136929706 ) ) ;
#34229=CARTESIAN_POINT ( 'NONE',  ( 10.44647102983249987, 1451.860058722380018, 207.7484592784610129 ) ) ;
#34232=ORIENTED_EDGE ( 'NONE', *, *, #89960, .F. ) ;
#34239=ORIENTED_EDGE ( 'NONE', *, *, #14729, .F. ) ;
#34241=ADVANCED_FACE ( 'NONE', ( #42852, #110597 ), #33321, .F. ) ;
#34243=CARTESIAN_POINT ( 'NONE',  ( -4.329341231296617742, 1515.068899845850183, 212.0800850781405131 ) ) ;
#34245=CARTESIAN_POINT ( 'NONE',  ( -3.672026810689013931, 1488.783744143340982, 219.3790594625757819 ) ) ;
#34247=CARTESIAN_POINT ( 'NONE',  ( 10.75512883408480036, 1470.091788688690031, 207.0349106889550228 ) ) ;
#34248=CARTESIAN_POINT ( 'NONE',  ( -10.38017158409999929, 1471.876108471190037, 207.0077964733490035 ) ) ;
#34255=CARTESIAN_POINT ( 'NONE',  ( -5.311690196159160493, 1500.891276851109978, 229.7589207481180154 ) ) ;
#34257=AXIS2_PLACEMENT_3D ( 'NONE', #93768, #318, #101618 ) ;
#34261=CARTESIAN_POINT ( 'NONE',  ( -14.60558113189999929, 1415.677402202029953, 212.8314178170890045 ) ) ;
#34262=CARTESIAN_POINT ( 'NONE',  ( 0.6417514479943100536, 1515.135428326259898, 204.7942468399390066 ) ) ;
#34263=ORIENTED_EDGE ( 'NONE', *, *, #24188, .F. ) ;
#34268=CARTESIAN_POINT ( 'NONE',  ( -10.90851772964620103, 1461.964075312410159, 210.6186257616180058 ) ) ;
#34270=CARTESIAN_POINT ( 'NONE',  ( -5.838032942621479648, 1427.197080586870015, 201.8313282331189953 ) ) ;
#34272=CARTESIAN_POINT ( 'NONE',  ( 13.12523828760000022, 1473.126683452290081, 192.9578767172990013 ) ) ;
#34275=CARTESIAN_POINT ( 'NONE',  ( -10.28629954290000015, 1479.827768412789965, 212.1118048706690047 ) ) ;
#34287=CARTESIAN_POINT ( 'NONE',  ( -15.25967915520000062, 1416.619611601430051, 206.0080059597690081 ) ) ;
#34289=CARTESIAN_POINT ( 'NONE',  ( -2.917647860963519690, 1485.453250951370137, 197.5824647639669820 ) ) ;
#34295=CARTESIAN_POINT ( 'NONE',  ( 10.52837420263239920, 1481.199010226290284, 208.2608686310830137 ) ) ;
#34307=CARTESIAN_POINT ( 'NONE',  ( -2.664535259099999805E-15, 1422.937291763169924, 209.1218459616989946 ) ) ;
#34310=ADVANCED_FACE ( 'NONE', ( #91261 ), #92923, .F. ) ;
#34314=CARTESIAN_POINT ( 'NONE',  ( 5.009762976649999366, 1485.882962529690076, 218.6550994417989671 ) ) ;
#34315=CARTESIAN_POINT ( 'NONE',  ( 4.482879682490001017, 1422.721247146459973, 194.3586833993989842 ) ) ;
#34318=EDGE_CURVE ( 'NONE', #11716, #90525, #36869, .T. ) ;
#34319=CARTESIAN_POINT ( 'NONE',  ( 11.78523210350000028, 1435.905840746989952, 225.6005139738989840 ) ) ;
#34321=CARTESIAN_POINT ( 'NONE',  ( 10.59813991437289893, 1477.524080021249802, 229.9254213493549912 ) ) ;
#34325=CARTESIAN_POINT ( 'NONE',  ( 9.764985867364520900, 1436.011985270369905, 210.2792758222440170 ) ) ;
#34326=CARTESIAN_POINT ( 'NONE',  ( -10.69722738760000169, 1491.094497843389945, 211.6881357245790127 ) ) ;
#34327=CARTESIAN_POINT ( 'NONE',  ( 9.159631730552030504, 1450.106319786690165, 204.1877701249059953 ) ) ;
#34345=LINE ( 'NONE', #85282, #17624 ) ;
#34356=CARTESIAN_POINT ( 'NONE',  ( 10.51790268500719883, 1480.734060164550101, 208.3818872041500185 ) ) ;
#34366=EDGE_LOOP ( 'NONE', ( #7931, #49399, #103898, #66972 ) ) ;
#34378=ORIENTED_EDGE ( 'NONE', *, *, #37865, .F. ) ;
#34392=CARTESIAN_POINT ( 'NONE',  ( -3.472682794772799841, 1428.654985552910148, 200.4267480108129860 ) ) ;
#34411=CARTESIAN_POINT ( 'NONE',  ( -9.105402976021849781, 1449.059321480550125, 210.1353435409779991 ) ) ;
#34419=CARTESIAN_POINT ( 'NONE',  ( -8.554652906407122614, 1461.548920753501307, 204.5271286160454167 ) ) ;
#34420=CARTESIAN_POINT ( 'NONE',  ( 21.02847232690000467, 1496.614785848189968, 206.9633919846189940 ) ) ;
#34421=CARTESIAN_POINT ( 'NONE',  ( 12.49401126939999962, 1451.800774058590150, 193.6953293048989906 ) ) ;
#34423=EDGE_CURVE ( 'NONE', #49356, #75164, #13849, .T. ) ;
#34426=CARTESIAN_POINT ( 'NONE',  ( -2.096701719259999930, 1429.602646753990030, 200.3590733686490069 ) ) ;
#34428=CARTESIAN_POINT ( 'NONE',  ( 10.86111838972819932, 1480.525208337349795, 210.6924698787690033 ) ) ;
#34430=CARTESIAN_POINT ( 'NONE',  ( -10.33299300126450149, 1447.717326489380184, 209.8084994042759774 ) ) ;
#34434=CARTESIAN_POINT ( 'NONE',  ( 2.109745707098269918, 1456.459472160349833, 219.5317045544409780 ) ) ;
#34441=CARTESIAN_POINT ( 'NONE',  ( 9.722209888710001024, 1428.114071763990069, 212.2005363753689835 ) ) ;
#34445=CARTESIAN_POINT ( 'NONE',  ( -5.787664699130000479, 1484.577383496389984, 199.2118460601089964 ) ) ;
#34447=EDGE_CURVE ( 'NONE', #47729, #106390, #39631, .T. ) ;
#34454=ORIENTED_EDGE ( 'NONE', *, *, #5630, .T. ) ;
#34458=CARTESIAN_POINT ( 'NONE',  ( -1.427750768948659932, 1457.410439390729834, 219.6702089923480230 ) ) ;
#34463=CARTESIAN_POINT ( 'NONE',  ( 7.458660324640000283, 1423.927228631740036, 212.7475639799289979 ) ) ;
#34464=CARTESIAN_POINT ( 'NONE',  ( 10.75631864630000045, 1451.138109685189875, 190.3409053448989994 ) ) ;
#34469=ADVANCED_FACE ( 'NONE', ( #12210 ), #5249, .T. ) ;
#34487=ORIENTED_EDGE ( 'NONE', *, *, #65149, .F. ) ;
#34516=CARTESIAN_POINT ( 'NONE',  ( 18.59085833919679942, 1477.390785077480132, 218.3860272671680320 ) ) ;
#34524=CARTESIAN_POINT ( 'NONE',  ( -3.710825917439999788, 1429.315763692190103, 201.5588532918390001 ) ) ;
#34538=FACE_OUTER_BOUND ( 'NONE', #87743, .T. ) ;
#34540=CARTESIAN_POINT ( 'NONE',  ( 5.752297360424160289, 1487.277805609919824, 203.3775840806389965 ) ) ;
#34553=CARTESIAN_POINT ( 'NONE',  ( -13.61671581806340114, 1417.869541547810059, 201.5013355043030003 ) ) ;
#34554=CARTESIAN_POINT ( 'NONE',  ( -5.098507870328135461, 1391.860130066733973, 203.6232600018305163 ) ) ;
#34562=CARTESIAN_POINT ( 'NONE',  ( 8.880307795244190672, 1425.079377176630032, 195.6786652326489957 ) ) ;
#34563=CARTESIAN_POINT ( 'NONE',  ( 4.971111079171492975, 1423.228780049225634, 194.5224207974501951 ) ) ;
#34565=CARTESIAN_POINT ( 'NONE',  ( -2.851657392136500047, 1487.618571494400157, 219.7563995687149827 ) ) ;
#34576=CARTESIAN_POINT ( 'NONE',  ( 8.440216524157060363, 1436.746754282560005, 207.3499268363860040 ) ) ;
#34580=CARTESIAN_POINT ( 'NONE',  ( -4.859106712929900596, 1457.993497594239898, 213.8797617162830136 ) ) ;
#34585=CARTESIAN_POINT ( 'NONE',  ( 8.765059777696018628, 1436.630117689859844, 209.3499172591779995 ) ) ;
#34593=CARTESIAN_POINT ( 'NONE',  ( -9.173749095941850840, 1450.559996438570124, 208.1432995907519796 ) ) ;
#34594=CARTESIAN_POINT ( 'NONE',  ( -14.05984932083289962, 1421.816753890520204, 203.6799934543310258 ) ) ;
#34598=ORIENTED_EDGE ( 'NONE', *, *, #85923, .T. ) ;
#34599=CARTESIAN_POINT ( 'NONE',  ( 10.83350752517260140, 1478.706377548199953, 229.8680168337830025 ) ) ;
#34603=CARTESIAN_POINT ( 'NONE',  ( -6.915889856759999788, 1473.238612421190055, 208.0311295872689925 ) ) ;
#34608=CARTESIAN_POINT ( 'NONE',  ( 0.4281874960050009449, 1475.888370069490065, 197.6396167722989787 ) ) ;
#34614=CARTESIAN_POINT ( 'NONE',  ( -7.703873474549999933, 1425.539119294559896, 205.4402485642290230 ) ) ;
#34620=CARTESIAN_POINT ( 'NONE',  ( -7.265312330176009858, 1471.117001311926515, 216.1747626545108290 ) ) ;
#34621=CARTESIAN_POINT ( 'NONE',  ( 7.539305306222179759, 1425.626486982010192, 212.1832883622500106 ) ) ;
#34624=CARTESIAN_POINT ( 'NONE',  ( -17.59976141832330043, 1419.797097700060021, 206.6695233765389901 ) ) ;
#34625=CARTESIAN_POINT ( 'NONE',  ( -11.48963409184570139, 1491.507525978150170, 206.8509400678860004 ) ) ;
#34642=CARTESIAN_POINT ( 'NONE',  ( -10.51574440819999978, 1480.737039981889893, 208.3487666310030306 ) ) ;
#34653=CARTESIAN_POINT ( 'NONE',  ( 2.093110410547600164, 1445.759653694790131, 199.2445041395880025 ) ) ;
#34655=ORIENTED_EDGE ( 'NONE', *, *, #17644, .F. ) ;
#34656=CARTESIAN_POINT ( 'NONE',  ( 4.019735481669824750, 1515.589562461881087, 208.4997842682788303 ) ) ;
#34658=CARTESIAN_POINT ( 'NONE',  ( -4.072632511706010483, 1508.551704408389924, 213.5435155163000047 ) ) ;
#34664=CARTESIAN_POINT ( 'NONE',  ( -1.693092047772239983, 1443.235800395060096, 218.9922115469449864 ) ) ;
#34673=CARTESIAN_POINT ( 'NONE',  ( -6.968573436492549789, 1484.503278946609953, 199.4663635475509977 ) ) ;
#34675=CARTESIAN_POINT ( 'NONE',  ( 8.405716135139408962, 1426.718822582190114, 211.2875594345169930 ) ) ;
#34676=( BOUNDED_CURVE ( )  B_SPLINE_CURVE ( 3, ( #8783, #84936, #102294, #101737 ),
 .UNSPECIFIED., .F., .T. ) 
 B_SPLINE_CURVE_WITH_KNOTS ( ( 4, 4 ),
 ( 0.9946974666264819520, 2.146895183780889838 ),
 .UNSPECIFIED. ) 
 CURVE ( )  GEOMETRIC_REPRESENTATION_ITEM ( )  RATIONAL_B_SPLINE_CURVE ( ( 1.000000000000000000, 0.8923961322389445394, 0.8923961322389445394, 1.000000000000000000 ) ) 
 REPRESENTATION_ITEM ( '' )  );
#34677=CARTESIAN_POINT ( 'NONE',  ( 12.58719134636679904, 1426.438815673830049, 202.7206058308819934 ) ) ;
#34684=CARTESIAN_POINT ( 'NONE',  ( -9.713507356099999157, 1424.012636679030038, 192.3806507662989702 ) ) ;
#34685=CARTESIAN_POINT ( 'NONE',  ( 9.816351554025828818, 1424.339539135469977, 198.3139274869160147 ) ) ;
#34687=CARTESIAN_POINT ( 'NONE',  ( 8.441029897509530144, 1464.999488427009965, 214.2962224928130297 ) ) ;
#34691=CARTESIAN_POINT ( 'NONE',  ( -7.604289863101939773, 1426.735970264149955, 206.0920986175900111 ) ) ;
#34694=CARTESIAN_POINT ( 'NONE',  ( 3.401869620952525874, 1507.778041293768410, 220.3126522683182316 ) ) ;
#34696=CARTESIAN_POINT ( 'NONE',  ( -9.609628611790521191, 1464.248357633179921, 228.1965958858790202 ) ) ;
#34698=CARTESIAN_POINT ( 'NONE',  ( -10.53793291988730019, 1423.359083101020133, 205.8279893113830212 ) ) ;
#34699=CARTESIAN_POINT ( 'NONE',  ( -2.330134126739549671, 1515.219201591195770, 204.7964405199902842 ) ) ;
#34700=CARTESIAN_POINT ( 'NONE',  ( 18.12237639339999973, 1431.228556021990016, 206.5934752596589874 ) ) ;
#34705=LINE ( 'NONE', #8948, #108668 ) ;
#34708=ORIENTED_EDGE ( 'NONE', *, *, #32906, .T. ) ;
#34709=B_SPLINE_SURFACE_WITH_KNOTS ( 'NONE', 5, 5, ( 
 ( #79751, #54020, #12529, #46709, #80837, #90320 ),
 ( #81366, #3608, #4679, #104938, #21991, #37731 ),
 ( #80292, #88150, #11438, #37184, #28226, #62413 ),
 ( #19814, #45610, #107132, #62984, #97639, #71934 ),
 ( #20908, #96540, #28784, #63524, #71382, #29871 ),
 ( #47787, #13598, #3059, #72995, #56182, #21448 ),
 ( #54566, #89235, #105492, #97095, #46162, #106046 ),
 ( #2507, #29323, #88699, #55110, #11980, #30423 ),
 ( #36629, #4145, #38818, #38269, #70827, #72455 ) ),
 .UNSPECIFIED., .F., .F., .F.,
 ( 6, 3, 6 ),
 ( 6, 6 ),
 ( 2.324858856890000158, 4.970096098099999971, 7.657659707949999728 ),
 ( 0.000000000000000000, 0.5000000000000000000 ),
 .UNSPECIFIED. ) ;
#34713=CARTESIAN_POINT ( 'NONE',  ( 8.044362178399680374, 1504.012373259569813, 212.2082695997949884 ) ) ;
#34714=CARTESIAN_POINT ( 'NONE',  ( -6.982434334785139640, 1435.340673196930084, 214.9240378055680196 ) ) ;
#34716=CARTESIAN_POINT ( 'NONE',  ( -15.11179371579999930, 1419.704522818860141, 212.3545469124089777 ) ) ;
#34719=B_SPLINE_SURFACE_WITH_KNOTS ( 'NONE', 5, 1, ( 
 ( #33592, #32520 ),
 ( #34713, #41477 ),
 ( #101897, #50438 ),
 ( #17329, #8956 ),
 ( #43129, #8397 ),
 ( #42567, #77288 ) ),
 .UNSPECIFIED., .F., .F., .F.,
 ( 6, 6 ),
 ( 2, 2 ),
 ( -9.395743872997430171E-05, 18.06269844883869879 ),
 ( 0.000000000000000000, 14.00009395743870044 ),
 .UNSPECIFIED. ) ;
#34722=CARTESIAN_POINT ( 'NONE',  ( 10.95716479804320009, 1427.278218707250062, 209.1113885757679896 ) ) ;
#34725=EDGE_CURVE ( 'NONE', #10311, #88376, #49657, .T. ) ;
#34729=ORIENTED_EDGE ( 'NONE', *, *, #27407, .F. ) ;
#34730=CARTESIAN_POINT ( 'NONE',  ( 1.842962214296182122, 1515.219201590508419, 204.7964405199711280 ) ) ;
#34732=CARTESIAN_POINT ( 'NONE',  ( -10.68791968979999929, 1492.481557180890150, 204.6992124531689967 ) ) ;
#34741=CARTESIAN_POINT ( 'NONE',  ( -1.337878788439999855, 1456.624765931489947, 199.6947203986289878 ) ) ;
#34745=B_SPLINE_SURFACE_WITH_KNOTS ( 'NONE', 5, 1, ( 
 ( #66572, #6630 ),
 ( #49754, #75514 ),
 ( #50314, #36121 ),
 ( #92834, #27711 ),
 ( #7189, #109647 ),
 ( #83884, #70305 ),
 ( #83334, #41888 ),
 ( #59264, #87064 ),
 ( #61897, #41344 ) ),
 .UNSPECIFIED., .F., .F., .F.,
 ( 6, 3, 6 ),
 ( 2, 2 ),
 ( 0.000000000000000000, 3.592628445999999975, 7.162337568599999926 ),
 ( 0.000000000000000000, 14.00000000000000000 ),
 .UNSPECIFIED. ) ;
#34746=DIRECTION ( 'NONE',  ( -1.000000000000000000, 0.000000000000000000, 0.000000000000000000 ) ) ;
#34747=CARTESIAN_POINT ( 'NONE',  ( -2.112801085030000081, 1497.385224591190081, 198.0352397674990073 ) ) ;
#34748=CARTESIAN_POINT ( 'NONE',  ( 0.7246754490289990525, 1495.521260695290039, 220.6941092417989978 ) ) ;
#34749=ORIENTED_EDGE ( 'NONE', *, *, #41104, .T. ) ;
#34751=ORIENTED_EDGE ( 'NONE', *, *, #38524, .T. ) ;
#34764=CARTESIAN_POINT ( 'NONE',  ( 4.363515742428809574, 1508.551704408389924, 213.2628643576499883 ) ) ;
#34768=CARTESIAN_POINT ( 'NONE',  ( -19.73883108929999963, 1465.087274007090173, 209.8242536915520020 ) ) ;
#34770=VERTEX_POINT ( 'NONE', #80405 ) ;
#34771=VERTEX_POINT ( 'NONE', #72562 ) ;
#34778=CARTESIAN_POINT ( 'NONE',  ( -10.58718094483835337, 1418.062149160418812, 197.9312562613863520 ) ) ;
#34779=CARTESIAN_POINT ( 'NONE',  ( -1.019681180111194907, 1443.417322147287450, 200.2632829245056314 ) ) ;
#34782=CARTESIAN_POINT ( 'NONE',  ( 9.144930279399812179, 1450.428525763479911, 207.9341771728810215 ) ) ;
#34783=LINE ( 'NONE', #77350, #80738 ) ;
#34785=ORIENTED_EDGE ( 'NONE', *, *, #83533, .T. ) ;
#34795=CARTESIAN_POINT ( 'NONE',  ( -7.514677712297311629, 1489.952809768607949, 217.0828538730388857 ) ) ;
#34798=CARTESIAN_POINT ( 'NONE',  ( 9.214423736713580837, 1450.766440915549992, 209.7350477037440157 ) ) ;
#34799=CARTESIAN_POINT ( 'NONE',  ( -8.617927921830000670, 1473.119234900290166, 202.1039715580190261 ) ) ;
#34804=CARTESIAN_POINT ( 'NONE',  ( 4.098642029037120160, 1466.578069225399986, 198.8310470422320009 ) ) ;
#34806=CARTESIAN_POINT ( 'NONE',  ( 11.95229909155720094, 1492.825378593110145, 212.2580762583590115 ) ) ;
#34807=AXIS2_PLACEMENT_3D ( 'NONE', #45538, #71860, #79677 ) ;
#34811=CARTESIAN_POINT ( 'NONE',  ( 2.719262146893400038E-32, 1524.051704408389924, 209.1218459616989946 ) ) ;
#34813=CARTESIAN_POINT ( 'NONE',  ( -14.59826557239999900, 1415.739699861750069, 213.4694186940990051 ) ) ;
#34814=CARTESIAN_POINT ( 'NONE',  ( -0.6516344982487189963, 1515.134688985600178, 204.7942274797200071 ) ) ;
#34825=CARTESIAN_POINT ( 'NONE',  ( -10.46710872037930073, 1480.356471093349910, 207.9758824041080061 ) ) ;
#34830=B_SPLINE_SURFACE_WITH_KNOTS ( 'NONE', 5, 1, ( 
 ( #67333, #66786 ),
 ( #39352, #23646 ),
 ( #40447, #49964 ),
 ( #22512, #14693 ),
 ( #24722, #91416 ),
 ( #23082, #49420 ) ),
 .UNSPECIFIED., .F., .F., .F.,
 ( 6, 6 ),
 ( 2, 2 ),
 ( 0.000000000000000000, 3.773583235669999869 ),
 ( 0.000000000000000000, 14.00000000000000000 ),
 .UNSPECIFIED. ) ;
#34834=CARTESIAN_POINT ( 'NONE',  ( -15.27212236273409829, 1418.081934325779912, 203.1274159867730020 ) ) ;
#34837=CARTESIAN_POINT ( 'NONE',  ( -14.43176891870000134, 1417.361915031260196, 203.3004091609390116 ) ) ;
#34841=CARTESIAN_POINT ( 'NONE',  ( -9.163890685529999303, 1498.531675235289867, 216.1508746217490113 ) ) ;
#34842=VERTEX_POINT ( 'NONE', #106689 ) ;
#34846=AXIS2_PLACEMENT_3D ( 'NONE', #52847, #242, #25943 ) ;
#34847=CARTESIAN_POINT ( 'NONE',  ( -11.76846763270469864, 1508.551704408290107, 209.7988299663460339 ) ) ;
#34864=CARTESIAN_POINT ( 'NONE',  ( 4.252899391840000654, 1485.733079649889987, 219.0121294742889972 ) ) ;
#34868=CARTESIAN_POINT ( 'NONE',  ( 20.24316163930199863, 1432.051856502529972, 214.9276842344050067 ) ) ;
#34870=CARTESIAN_POINT ( 'NONE',  ( 24.11200242905490043, 1496.633641595180052, 206.8275340915270135 ) ) ;
#34875=CARTESIAN_POINT ( 'NONE',  ( -10.77749580200000068, 1490.550318827689807, 211.8705906801690162 ) ) ;
#34876=CARTESIAN_POINT ( 'NONE',  ( 7.961513149873700179, 1449.132914919729956, 202.5404456399149922 ) ) ;
#34879=CARTESIAN_POINT ( 'NONE',  ( -4.794426340529999386, 1463.608615258990085, 228.2108236244990280 ) ) ;
#34883=CARTESIAN_POINT ( 'NONE',  ( -10.16358567940831747, 1422.552167032401030, 210.6545967428373842 ) ) ;
#34892=CARTESIAN_POINT ( 'NONE',  ( -10.33299300126450149, 1447.717326489380184, 209.8084994042759774 ) ) ;
#34893=CARTESIAN_POINT ( 'NONE',  ( 4.259777698987599948, 1515.374151778960140, 206.1850281986660036 ) ) ;
#34898=CARTESIAN_POINT ( 'NONE',  ( 3.235048537869999574, 1466.472015836390028, 219.6884158037989891 ) ) ;
#34900=( NAMED_UNIT ( * ) SI_UNIT ( $, .STERADIAN. ) SOLID_ANGLE_UNIT ( ) );
#34906=EDGE_LOOP ( 'NONE', ( #55869, #104182 ) ) ;
#34914=CARTESIAN_POINT ( 'NONE',  ( -8.251582857397114168, 1474.733389988602312, 202.9883399646709279 ) ) ;
#34916=CARTESIAN_POINT ( 'NONE',  ( 0.2753775948021700004, 1465.468850400709925, 198.1161068840000041 ) ) ;
#34917=CARTESIAN_POINT ( 'NONE',  ( 11.32781805967280064, 1422.100515973739903, 210.2113672716099870 ) ) ;
#34922=EDGE_LOOP ( 'NONE', ( #71484, #66988, #34239, #109558 ) ) ;
#34931=CARTESIAN_POINT ( 'NONE',  ( -17.83658993330359976, 1508.551704408389924, 210.4067863104130254 ) ) ;
#34932=CARTESIAN_POINT ( 'NONE',  ( 1.363474410897823397, 1457.370847949542167, 199.6942262104683437 ) ) ;
#34936=CARTESIAN_POINT ( 'NONE',  ( -2.480175250669919951, 1429.207669930499833, 200.0830571243679969 ) ) ;
#34941=EDGE_CURVE ( 'NONE', #26525, #66058, #64731, .T. ) ;
#34946=ORIENTED_EDGE ( 'NONE', *, *, #110287, .F. ) ;
#34956=CARTESIAN_POINT ( 'NONE',  ( -9.922530801272239742, 1448.008349691420108, 209.5732083501220018 ) ) ;
#34960=CARTESIAN_POINT ( 'NONE',  ( -12.71621933285400097, 1508.444018394370232, 217.3234386178750128 ) ) ;
#34964=DIRECTION ( 'NONE',  ( -1.156023075842281927E-31, 1.000000000000000000, -1.698192320643030073E-16 ) ) ;
#34966=CARTESIAN_POINT ( 'NONE',  ( -19.23853081770000273, 1466.576780668189940, 213.8528554934590034 ) ) ;
#34972=CARTESIAN_POINT ( 'NONE',  ( 10.55550475196309890, 1481.771801338060186, 210.0110538323510241 ) ) ;
#34977=ORIENTED_EDGE ( 'NONE', *, *, #24711, .T. ) ;
#34981=CARTESIAN_POINT ( 'NONE',  ( 3.436083655040000018, 1486.341471508789937, 198.7604659685989645 ) ) ;
#34984=CARTESIAN_POINT ( 'NONE',  ( 11.60325616329999932, 1501.577980218590028, 209.3671369954699912 ) ) ;
#34987=CARTESIAN_POINT ( 'NONE',  ( 7.537605568320000060, 1427.603033106790008, 212.6450987096289964 ) ) ;
#34998=ORIENTED_EDGE ( 'NONE', *, *, #99444, .T. ) ;
#35000=CARTESIAN_POINT ( 'NONE',  ( 1.083797102072519891, 1435.612377985999956, 227.5537550227259942 ) ) ;
#35002=CARTESIAN_POINT ( 'NONE',  ( -14.91528134978724651, 1416.112049509652024, 205.1592457836539438 ) ) ;
#35004=CARTESIAN_POINT ( 'NONE',  ( -9.977345552905569903, 1439.328177480719887, 208.7903818577229913 ) ) ;
#35007=CARTESIAN_POINT ( 'NONE',  ( 7.840108726700000474, 1425.497406979299967, 211.6543916462389916 ) ) ;
#35008=CARTESIAN_POINT ( 'NONE',  ( 19.03958014020000178, 1453.804227313890124, 200.7927590370090059 ) ) ;
#35013=ORIENTED_EDGE ( 'NONE', *, *, #85004, .F. ) ;
#35014=ORIENTED_EDGE ( 'NONE', *, *, #3285, .T. ) ;
#35015=VECTOR ( 'NONE', #99228, 999.9999999999998863 ) ;
#35020=CARTESIAN_POINT ( 'NONE',  ( 8.055079858170127949, 1500.429113765004331, 201.0492220431988812 ) ) ;
#35023=CARTESIAN_POINT ( 'NONE',  ( -2.617907763213700001, 1475.116115922490053, 197.9881756648049986 ) ) ;
#35035=ORIENTED_EDGE ( 'NONE', *, *, #86810, .T. ) ;
#35038=DIRECTION ( 'NONE',  ( 9.156846217086110244E-47, -1.000000000000000000, 1.836970198721029688E-16 ) ) ;
#35047=EDGE_CURVE ( 'NONE', #30629, #2493, #12348, .T. ) ;
#35057=CARTESIAN_POINT ( 'NONE',  ( 12.55308716756742626, 1426.311334306029721, 201.5587213662597037 ) ) ;
#35059=CARTESIAN_POINT ( 'NONE',  ( 10.70400544403340071, 1460.361839742069833, 206.9582489332520083 ) ) ;
#35069=ORIENTED_EDGE ( 'NONE', *, *, #33530, .F. ) ;
#35074=EDGE_LOOP ( 'NONE', ( #66808, #80245, #70423, #81989, #48589 ) ) ;
#35076=CARTESIAN_POINT ( 'NONE',  ( -3.492373078290000432, 1428.790505188590032, 200.8458585022190164 ) ) ;
#35088=ORIENTED_EDGE ( 'NONE', *, *, #45953, .F. ) ;
#35091=ORIENTED_EDGE ( 'NONE', *, *, #62581, .T. ) ;
#35094=CARTESIAN_POINT ( 'NONE',  ( -17.28313798789999822, 1509.292373661990041, 209.6576118363560113 ) ) ;
#35095=FACE_OUTER_BOUND ( 'NONE', #64487, .T. ) ;
#35096=CARTESIAN_POINT ( 'NONE',  ( 2.975355613810000133, 1441.383001986190038, 218.5845790346389776 ) ) ;
#35101=CARTESIAN_POINT ( 'NONE',  ( 9.529616216263738337, 1459.343410895429997, 203.7689765404180093 ) ) ;
#35102=CARTESIAN_POINT ( 'NONE',  ( -8844.044327685292956, -2339.359351152911131, 3014.028579042705587 ) ) ;
#35104=CARTESIAN_POINT ( 'NONE',  ( -14.75778311606660154, 1417.788083049279976, 203.2704335446259734 ) ) ;
#35105=CARTESIAN_POINT ( 'NONE',  ( -4.993214560040000194, 1391.653934889589891, 203.5347113830289913 ) ) ;
#35108=CARTESIAN_POINT ( 'NONE',  ( -8.308282170169999148, 1508.515045414190126, 219.1793389093990072 ) ) ;
#35117=CARTESIAN_POINT ( 'NONE',  ( -3.522358130609859916, 1488.738444080139971, 219.4891182003030110 ) ) ;
#35119=CARTESIAN_POINT ( 'NONE',  ( -9.573037224950001089, 1423.427965722019962, 192.3355728592989919 ) ) ;
#35122=LINE ( 'NONE', #59791, #62496 ) ;
#35131=ORIENTED_EDGE ( 'NONE', *, *, #56222, .T. ) ;
#35143=CARTESIAN_POINT ( 'NONE',  ( 1.443775278116770089, 1486.508325946929972, 197.2873345197639878 ) ) ;
#35145=CARTESIAN_POINT ( 'NONE',  ( -9.127884186257210430, 1449.574596975079885, 210.1377844312270042 ) ) ;
#35146=CARTESIAN_POINT ( 'NONE',  ( -15.39552638457469946, 1421.149667150770028, 203.4478981028480007 ) ) ;
#35149=VERTEX_POINT ( 'NONE', #104929 ) ;
#35151=CARTESIAN_POINT ( 'NONE',  ( -3.041881798304169937, 1470.651976562600112, 187.4038384089669762 ) ) ;
#35157=CARTESIAN_POINT ( 'NONE',  ( -20.53092383730000137, 1484.406264705989997, 211.0952521839789711 ) ) ;
#35165=CARTESIAN_POINT ( 'NONE',  ( -8.375770438119999994, 1423.465221721570060, 210.4663274327489830 ) ) ;
#35170=B_SPLINE_CURVE_WITH_KNOTS ( 'NONE', 5,
 ( #14010, #40325, #73946, #16203, #7280, #49849, #14565, #83980, #32490 ),
 .UNSPECIFIED., .F., .F.,
 ( 6, 3, 6 ),
 ( 0.000000000000000000, 0.4794969076149564469, 1.000000000000000000 ),
 .UNSPECIFIED. ) ;
#35172=CARTESIAN_POINT ( 'NONE',  ( 7.529301028092720394, 1425.491244692560031, 212.1922084480190165 ) ) ;
#35173=AXIS2_PLACEMENT_3D ( 'NONE', #79074, #62280, #61727 ) ;
#35179=CARTESIAN_POINT ( 'NONE',  ( 2.115993288544910200, 1487.070543772652172, 219.7330506709243707 ) ) ;
#35180=CARTESIAN_POINT ( 'NONE',  ( -17.46391305203579947, 1508.455563235159843, 212.6812038778440126 ) ) ;
#35182=CARTESIAN_POINT ( 'NONE',  ( 1.818941110869999989, 1460.558667203089954, 228.6206250013989916 ) ) ;
#35183=CARTESIAN_POINT ( 'NONE',  ( -9.096589177653610747, 1440.282626970159754, 206.1069680632970176 ) ) ;
#35184=ORIENTED_EDGE ( 'NONE', *, *, #69186, .T. ) ;
#35189=EDGE_CURVE ( 'NONE', #23187, #53058, #45496, .T. ) ;
#35201=CARTESIAN_POINT ( 'NONE',  ( -4.736739505650000126, 1428.640587360089967, 202.0925030146489974 ) ) ;
#35203=VERTEX_POINT ( 'NONE', #93067 ) ;
#35211=CARTESIAN_POINT ( 'NONE',  ( -4.973792553552699225, 1508.551704408389924, 211.8808810681379953 ) ) ;
#35215=CARTESIAN_POINT ( 'NONE',  ( 11.76014420379719994, 1479.338752705380102, 208.6264958516850072 ) ) ;
#35217=CARTESIAN_POINT ( 'NONE',  ( -1.285566754106051146, 1444.251790938402337, 217.9819968700315940 ) ) ;
#35231=CARTESIAN_POINT ( 'NONE',  ( 1.647872562449680167, 1421.485654266244183, 193.8027845224808914 ) ) ;
#35232=CARTESIAN_POINT ( 'NONE',  ( -10.81837133496780012, 1462.844907795940117, 206.8474244494269954 ) ) ;
#35239=CARTESIAN_POINT ( 'NONE',  ( 18.32584553287430040, 1429.337180726220140, 201.2167037691079940 ) ) ;
#35240=EDGE_CURVE ( 'NONE', #72871, #23842, #16019, .T. ) ;
#35249=CARTESIAN_POINT ( 'NONE',  ( -0.5646469274638281632, 1477.536569817737927, 198.7333153465972373 ) ) ;
#35251=CARTESIAN_POINT ( 'NONE',  ( 3.298919637249711379, 1508.340401136613082, 219.9739890455120985 ) ) ;
#35252=CARTESIAN_POINT ( 'NONE',  ( -18.29179382875269866, 1466.060301896490046, 217.7541515181700049 ) ) ;
#35255=CARTESIAN_POINT ( 'NONE',  ( -14.88318523122000059, 1421.206373356060112, 205.0325180053320082 ) ) ;
#35260=CARTESIAN_POINT ( 'NONE',  ( -4.629662637760000088, 1475.320779598089985, 199.7646424499390037 ) ) ;
#35263=CARTESIAN_POINT ( 'NONE',  ( -3.818868948821170228, 1508.551704408389924, 219.8880244334079919 ) ) ;
#35266=B_SPLINE_CURVE_WITH_KNOTS ( 'NONE', 5,
 ( #108988, #75399, #32811, #44412, #19161, #94228 ),
 .UNSPECIFIED., .F., .F.,
 ( 6, 6 ),
 ( 0.000000000000000000, 1.000000000000000000 ),
 .UNSPECIFIED. ) ;
#35267=DIRECTION ( 'NONE',  ( -1.000000000000000000, 0.000000000000000000, 0.000000000000000000 ) ) ;
#35271=CARTESIAN_POINT ( 'NONE',  ( -1.191415256510000020, 1432.303667401890152, 218.5821185343490072 ) ) ;
#35272=CARTESIAN_POINT ( 'NONE',  ( -11.11751878483429934, 1471.394268115599971, 206.7642780669090143 ) ) ;
#35284=ORIENTED_EDGE ( 'NONE', *, *, #35393, .T. ) ;
#35287=CARTESIAN_POINT ( 'NONE',  ( -11.59964765079999971, 1491.341587899690012, 206.7829323850089907 ) ) ;
#35289=CARTESIAN_POINT ( 'NONE',  ( 12.41707514731779938, 1427.120553744379777, 206.8353885506759866 ) ) ;
#35291=CARTESIAN_POINT ( 'NONE',  ( -9108.204429824800172, -2340.220200558880151, -1569.808522337019895 ) ) ;
#35293=CARTESIAN_POINT ( 'NONE',  ( -21.34331888389999676, 1507.003414196590029, 212.5301348003789883 ) ) ;
#35295=CARTESIAN_POINT ( 'NONE',  ( 0.3001670315860009430, 1456.850937440089865, 199.4793357935189988 ) ) ;
#35299=CARTESIAN_POINT ( 'NONE',  ( 849.7329242730789929, 1438.581626214380094, 209.1374421084189805 ) ) ;
#35300=CARTESIAN_POINT ( 'NONE',  ( -2.580029938729999639, 1497.232914682590035, 198.1414743728990118 ) ) ;
#35301=CARTESIAN_POINT ( 'NONE',  ( -3.216334032309999813, 1497.139726794089711, 221.0989039285990145 ) ) ;
#35304=EDGE_LOOP ( 'NONE', ( #66636, #23949, #14099, #3676 ) ) ;
#35316=CARTESIAN_POINT ( 'NONE',  ( 4.301866786085239980, 1508.551704408389924, 213.3279396115709687 ) ) ;
#35318=ORIENTED_EDGE ( 'NONE', *, *, #54487, .T. ) ;
#35320=CARTESIAN_POINT ( 'NONE',  ( 9.404417543028079862, 1461.021834069670149, 206.2633287157840130 ) ) ;
#35327=ORIENTED_EDGE ( 'NONE', *, *, #100700, .T. ) ;
#35328=CARTESIAN_POINT ( 'NONE',  ( -7.526713224480260145, 1508.370997529450051, 219.6556564864339975 ) ) ;
#35329=CARTESIAN_POINT ( 'NONE',  ( -14.72917304848470010, 1508.551704408389924, 210.3587638926149737 ) ) ;
#35334=CARTESIAN_POINT ( 'NONE',  ( 9.279213122865108687, 1450.852794977289932, 207.7366403636850123 ) ) ;
#35335=CARTESIAN_POINT ( 'NONE',  ( 19.22058768450000343, 1456.859121009089904, 206.3396914917290133 ) ) ;
#35349=CARTESIAN_POINT ( 'NONE',  ( -10.56724066066260015, 1462.360737918739915, 208.4611404715059848 ) ) ;
#35353=CARTESIAN_POINT ( 'NONE',  ( -5.592037798779999846, 1474.580918538189962, 199.9913374685289966 ) ) ;
#35354=CARTESIAN_POINT ( 'NONE',  ( 10.51054125589999977, 1491.593346108490096, 212.4262192567589693 ) ) ;
#35360=TOROIDAL_SURFACE ( 'NONE', #10263, 3.250000000000000000, 0.5000000000000000000 ) ;
#35369=CARTESIAN_POINT ( 'NONE',  ( -0.6118612317751669361, 1515.137305168459989, 204.7942959869070023 ) ) ;
#35371=CARTESIAN_POINT ( 'NONE',  ( -15.65670116826264113, 1415.721358585960843, 209.6507542426478494 ) ) ;
#35372=CARTESIAN_POINT ( 'NONE',  ( 20.14609246460000236, 1475.555345410090013, 207.1883922094089883 ) ) ;
#35375=CARTESIAN_POINT ( 'NONE',  ( -11.03553767863800061, 1462.348513829580043, 209.1377274935910009 ) ) ;
#35377=CARTESIAN_POINT ( 'NONE',  ( -9.783936650027678539, 1438.409968310599879, 210.7790528106160082 ) ) ;
#35380=CARTESIAN_POINT ( 'NONE',  ( -8.049345161460001563, 1477.536138853090051, 215.9441310019589935 ) ) ;
#35393=EDGE_CURVE ( 'NONE', #103755, #1788, #6777, .T. ) ;
#35395=CARTESIAN_POINT ( 'NONE',  ( -15.57670388880000090, 1415.694330284400166, 209.2552609234499812 ) ) ;
#35399=FACE_OUTER_BOUND ( 'NONE', #73423, .T. ) ;
#35414=CIRCLE ( 'NONE', #3313, 2.458500000000000352 ) ;
#35417=CARTESIAN_POINT ( 'NONE',  ( 4.282693164180000345, 1515.349926011190064, 208.0213331141290212 ) ) ;
#35422=CARTESIAN_POINT ( 'NONE',  ( 3.910001326520000209, 1486.362971887289859, 219.1796580760989741 ) ) ;
#35423=CARTESIAN_POINT ( 'NONE',  ( 10.91379151888849819, 1479.765342082039979, 208.3165719332679942 ) ) ;
#35425=CARTESIAN_POINT ( 'NONE',  ( 20.78241041049849969, 1455.840303560959910, 207.1559588098690199 ) ) ;
#35427=CARTESIAN_POINT ( 'NONE',  ( 19.12715434814980142, 1496.834837383639979, 222.0421819497279898 ) ) ;
#35430=CARTESIAN_POINT ( 'NONE',  ( -5.026419929959999422, 1391.797186054590156, 203.6610981513489946 ) ) ;
#35431=CARTESIAN_POINT ( 'NONE',  ( 9.803321272836790001, 1435.322606278559988, 208.6575614323569994 ) ) ;
#35432=CARTESIAN_POINT ( 'NONE',  ( -10.69044905890000052, 1491.561357479690059, 211.7988311077089918 ) ) ;
#35433=CARTESIAN_POINT ( 'NONE',  ( 10.16318987985490097, 1451.293190031329914, 206.5284763887880217 ) ) ;
#35434=CARTESIAN_POINT ( 'NONE',  ( 3.829620113550000315, 1515.551704408389924, 206.7917118356089929 ) ) ;
#35441=CARTESIAN_POINT ( 'NONE',  ( -11.53006918210525278, 1506.266512897565917, 207.3910517571966068 ) ) ;
#35457=( LENGTH_UNIT ( ) NAMED_UNIT ( * ) SI_UNIT ( .MILLI., .METRE. ) );
#35460=CARTESIAN_POINT ( 'NONE',  ( -9.110776130009609730, 1423.030562184250130, 209.7485040796009912 ) ) ;
#35462=VERTEX_POINT ( 'NONE', #18005 ) ;
#35464=( NAMED_UNIT ( * ) SI_UNIT ( $, .STERADIAN. ) SOLID_ANGLE_UNIT ( ) );
#35465=ORIENTED_EDGE ( 'NONE', *, *, #5484, .T. ) ;
#35469=CARTESIAN_POINT ( 'NONE',  ( -8.142296919120433074, 1474.791439460570473, 202.8386750668462923 ) ) ;
#35471=CARTESIAN_POINT ( 'NONE',  ( -0.7542027323512070502, 1465.241414061940077, 198.1437931916329944 ) ) ;
#35472=CARTESIAN_POINT ( 'NONE',  ( 11.25476890810059949, 1422.124858124740058, 210.3410537449459810 ) ) ;
#35474=CARTESIAN_POINT ( 'NONE',  ( 3.238415943299999711, 1465.057015839789983, 199.8093003563689933 ) ) ;
#35485=CARTESIAN_POINT ( 'NONE',  ( 1.044682716639319997, 1423.188007962369966, 192.5288407937300121 ) ) ;
#35491=CARTESIAN_POINT ( 'NONE',  ( 9.327651199099038948, 1434.415569083649871, 206.2244204008570136 ) ) ;
#35494=TOROIDAL_SURFACE ( 'NONE', #3382, 14.90133124319999780, 0.5000000000000000000 ) ;
#35495=CARTESIAN_POINT ( 'NONE',  ( -2.646857175475319846, 1429.116376473109995, 200.1321371505179911 ) ) ;
#35498=AXIS2_PLACEMENT_3D ( 'NONE', #84105, #50527, #7405 ) ;
#35501=CARTESIAN_POINT ( 'NONE',  ( -11.85130961024979968, 1482.142199958030233, 208.1561019704090256 ) ) ;
#35522=CARTESIAN_POINT ( 'NONE',  ( 3.317744430799999922, 1467.314064772389884, 218.6468771502790105 ) ) ;
#35523=CARTESIAN_POINT ( 'NONE',  ( 5.981720629350000706, 1449.156460935289942, 207.4142490612589995 ) ) ;
#35528=CARTESIAN_POINT ( 'NONE',  ( 10.50869459094269942, 1481.949074847140082, 210.5032414321599958 ) ) ;
#35529=CARTESIAN_POINT ( 'NONE',  ( 3.005897003519999888, 1505.999189604289995, 221.1413980816990090 ) ) ;
#35530=CARTESIAN_POINT ( 'NONE',  ( -8.557209110492459914, 1448.617779613390212, 212.3361752075699940 ) ) ;
#35531=ORIENTED_EDGE ( 'NONE', *, *, #73425, .T. ) ;
#35534=CARTESIAN_POINT ( 'NONE',  ( 9.755929852662839963, 1468.207539460409862, 206.7555844597239911 ) ) ;
#35536=FACE_OUTER_BOUND ( 'NONE', #72105, .T. ) ;
#35538=CARTESIAN_POINT ( 'NONE',  ( 7.721630276590000008, 1426.874396221100142, 211.9998969879490289 ) ) ;
#35540=B_SPLINE_SURFACE_WITH_KNOTS ( 'NONE', 5, 1, ( 
 ( #85340, #84252 ),
 ( #84791, #101585 ),
 ( #76405, #8637 ),
 ( #75862, #66928 ),
 ( #42813, #51775 ),
 ( #23782, #59078 ) ),
 .UNSPECIFIED., .F., .F., .F.,
 ( 6, 6 ),
 ( 2, 2 ),
 ( 0.000000000000000000, 16.39065553909999906 ),
 ( 0.000000000000000000, 14.00000000000000000 ),
 .UNSPECIFIED. ) ;
#35542=CARTESIAN_POINT ( 'NONE',  ( -9.721170047090000210, 1481.243685225789932, 204.9479232781289966 ) ) ;
#35548=VERTEX_POINT ( 'NONE', #35941 ) ;
#35549=ORIENTED_EDGE ( 'NONE', *, *, #68125, .T. ) ;
#35550=CARTESIAN_POINT ( 'NONE',  ( 4.900006679340000559, 1499.255191946190052, 229.7873568473989963 ) ) ;
#35553=CARTESIAN_POINT ( 'NONE',  ( 0.9724418386591719976, 1456.734366788370153, 219.6981812980549762 ) ) ;
#35557=CONICAL_SURFACE ( 'NONE', #81993, 6.911399307709998219, 0.04363323129990067523 ) ;
#35558=CARTESIAN_POINT ( 'NONE',  ( 7.526645696320000134, 1425.452156459670050, 212.1942742985490042 ) ) ;
#35559=CARTESIAN_POINT ( 'NONE',  ( -3.005245951399999615, 1450.300005596989877, 188.5532306447990152 ) ) ;
#35563=CARTESIAN_POINT ( 'NONE',  ( 7.016154481710000113, 1454.841981631690032, 216.5674988146290048 ) ) ;
#35564=ORIENTED_EDGE ( 'NONE', *, *, #64522, .T. ) ;
#35571=CARTESIAN_POINT ( 'NONE',  ( 7.253697669526002478, 1500.197240720463924, 200.3293451155131493 ) ) ;
#35576=CARTESIAN_POINT ( 'NONE',  ( 0.5358887729754751028, 1475.906136617699985, 197.6669786481479889 ) ) ;
#35585=EDGE_LOOP ( 'NONE', ( #82727, #101837, #20281, #17507, #99184 ) ) ;
#35604=CARTESIAN_POINT ( 'NONE',  ( -10.16240527536719895, 1472.558926193989919, 209.8189312950259762 ) ) ;
#35613=DIRECTION ( 'NONE',  ( -1.000000000000000000, 0.000000000000000000, 0.000000000000000000 ) ) ;
#35615=CARTESIAN_POINT ( 'NONE',  ( -21.51338411143810347, 1505.551551846900111, 209.1218200089510333 ) ) ;
#35624=CARTESIAN_POINT ( 'NONE',  ( -11.82942659101509975, 1491.433867479470109, 205.8513465834750207 ) ) ;
#35626=EDGE_CURVE ( 'NONE', #76715, #27116, #57587, .T. ) ;
#35645=CARTESIAN_POINT ( 'NONE',  ( -8.169799973510000868, 1501.392344667289990, 208.3166649180830063 ) ) ;
#35648=CARTESIAN_POINT ( 'NONE',  ( 3.745877440767119815, 1424.347276005310050, 191.5446012222820116 ) ) ;
#35650=CARTESIAN_POINT ( 'NONE',  ( 230.7985005798999794, 11216.44053380570040, -1757.088479869530147 ) ) ;
#35664=CARTESIAN_POINT ( 'NONE',  ( 9.651066088509999474, 1425.440658930580184, 195.4941615409990163 ) ) ;
#35669=CARTESIAN_POINT ( 'NONE',  ( -11.39266988268109948, 1470.664952754889782, 209.5618712138449951 ) ) ;
#35671=CARTESIAN_POINT ( 'NONE',  ( -8.627771016562100215, 1437.492617161759881, 228.3379561119689924 ) ) ;
#35680=CARTESIAN_POINT ( 'NONE',  ( -14.72209156862839841, 1419.171754436449874, 213.6412557114610138 ) ) ;
#35684=CARTESIAN_POINT ( 'NONE',  ( 9.698064461892839105, 1462.705242386489999, 208.0596150282290182 ) ) ;
#35689=CARTESIAN_POINT ( 'NONE',  ( -4.535936068263819898, 1495.192894671210070, 197.6626227834830161 ) ) ;
#35697=CARTESIAN_POINT ( 'NONE',  ( -9.204027750931148333, 1450.286637959580048, 208.6661583415359758 ) ) ;
#35698=CARTESIAN_POINT ( 'NONE',  ( -16.40172556159690131, 1420.659342363810083, 203.2854767675109997 ) ) ;
#35700=CARTESIAN_POINT ( 'NONE',  ( 3.195005116169999937, 1472.592485613090048, 218.8132852216689912 ) ) ;
#35702=FACE_OUTER_BOUND ( 'NONE', #56549, .T. ) ;
#35704=CARTESIAN_POINT ( 'NONE',  ( 18.25820950609999826, 1474.753073108990066, 194.7346205266990182 ) ) ;
#35710=VECTOR ( 'NONE', #68500, 1000.000000000000227 ) ;
#35719=DIRECTION ( 'NONE',  ( -0.9531156431133573914, 0.2972425205391840963, 0.05672261309322752798 ) ) ;
#35720=AXIS2_PLACEMENT_3D ( 'NONE', #44554, #10951, #61931 ) ;
#35723=EDGE_CURVE ( 'NONE', #104032, #42951, #44299, .T. ) ;
#35726=CARTESIAN_POINT ( 'NONE',  ( -6.694418385159999652, 1473.791160286789818, 199.7891180969089930 ) ) ;
#35730=CARTESIAN_POINT ( 'NONE',  ( -2.128846521502799849, 1496.797177652799974, 221.3100224611679891 ) ) ;
#35731=ORIENTED_EDGE ( 'NONE', *, *, #78858, .F. ) ;
#35739=EDGE_CURVE ( 'NONE', #36610, #104032, #53586, .T. ) ;
#35740=CARTESIAN_POINT ( 'NONE',  ( -9.731514810505409230, 1440.165830278139993, 206.7233373073800067 ) ) ;
#35741=ORIENTED_EDGE ( 'NONE', *, *, #7683, .T. ) ;
#35747=EDGE_LOOP ( 'NONE', ( #70987, #79939, #30361, #29790, #10706 ) ) ;
#35749=ADVANCED_FACE ( 'NONE', ( #17712 ), #41050, .T. ) ;
#35762=ORIENTED_EDGE ( 'NONE', *, *, #76649, .F. ) ;
#35772=CARTESIAN_POINT ( 'NONE',  ( 7.406484258469999915, 1423.002001740159812, 195.5970099228989909 ) ) ;
#35775=CARTESIAN_POINT ( 'NONE',  ( -3.980933278039999745, 1495.557870970189924, 197.8745908229989823 ) ) ;
#35785=CARTESIAN_POINT ( 'NONE',  ( -16.95354638770000122, 1417.269256936009924, 207.1959995758089974 ) ) ;
#35787=CARTESIAN_POINT ( 'NONE',  ( -6.736062857916709667, 1484.563701159229822, 199.3070513110980073 ) ) ;
#35789=ADVANCED_FACE ( 'NONE', ( #101052 ), #74128, .T. ) ;
#35791=CARTESIAN_POINT ( 'NONE',  ( -4.328122124485859423, 1515.115455661490159, 208.2045458931170003 ) ) ;
#35797=B_SPLINE_SURFACE_WITH_KNOTS ( 'NONE', 5, 5, ( 
 ( #57746, #91866, #85112, #7856, #40910, #15140 ),
 ( #49330, #110322, #33596, #67791, #109239, #102459 ),
 ( #48792, #6206, #6751, #25193, #59396, #32523 ),
 ( #93507, #66695, #16779, #50983, #8400, #26877 ),
 ( #45359, #43133, #103575, #96287, #34716, #79498 ),
 ( #8962, #77291, #94618, #53770, #19564, #95183 ) ),
 .UNSPECIFIED., .F., .F., .F.,
 ( 6, 6 ),
 ( 6, 6 ),
 ( 0.5468448937290000256, 9.215064474420000096 ),
 ( 0.000000000000000000, 20.00000000000000000 ),
 .UNSPECIFIED. ) ;
#35800=CARTESIAN_POINT ( 'NONE',  ( -9.760330733150000881, 1424.207526998040066, 192.3956767351990038 ) ) ;
#35810=CARTESIAN_POINT ( 'NONE',  ( -16.62238355811029322, 1420.074002544102314, 208.4323893795217089 ) ) ;
#35813=CARTESIAN_POINT ( 'NONE',  ( 19.12715430460800192, 1496.834837051899967, 222.0421819869680178 ) ) ;
#35822=CARTESIAN_POINT ( 'NONE',  ( -4.376458691559999892, 1474.728570106689858, 198.9952830931989922 ) ) ;
#35825=CARTESIAN_POINT ( 'NONE',  ( -4.661699225921780432, 1508.551704408389924, 219.7406003995500043 ) ) ;
#35830=EDGE_CURVE ( 'NONE', #86670, #22363, #108337, .T. ) ;
#35832=CARTESIAN_POINT ( 'NONE',  ( 0.7162863658319988946, 1429.709265593189912, 217.4063670190490143 ) ) ;
#35840=ORIENTED_EDGE ( 'NONE', *, *, #46991, .F. ) ;
#35844=CARTESIAN_POINT ( 'NONE',  ( 7.492689511757870235, 1466.181183281610174, 215.6096703809890016 ) ) ;
#35849=CARTESIAN_POINT ( 'NONE',  ( 2.433505161638750192, 1497.103005101570034, 196.9591516541469787 ) ) ;
#35850=EDGE_CURVE ( 'NONE', #25072, #12462, #32180, .T. ) ;
#35852=CARTESIAN_POINT ( 'NONE',  ( 11.68966055026420037, 1427.510905538520092, 209.0456480543080033 ) ) ;
#35855=CARTESIAN_POINT ( 'NONE',  ( 4.233304266720000264, 1446.747982731589900, 200.2615130837390041 ) ) ;
#35865=CARTESIAN_POINT ( 'NONE',  ( 1.375364450349999990, 1495.360691154489814, 220.6206533883990062 ) ) ;
#35867=EDGE_CURVE ( 'NONE', #86830, #61012, #62980, .T. ) ;
#35875=AXIS2_PLACEMENT_3D ( 'NONE', #51593, #60564, #94684 ) ;
#35880=CARTESIAN_POINT ( 'NONE',  ( -5.222641443459999699, 1391.931189958289906, 214.6468068300290213 ) ) ;
#35884=CARTESIAN_POINT ( 'NONE',  ( 10.64147525944390082, 1460.268832998469861, 206.6760994863940084 ) ) ;
#35889=CARTESIAN_POINT ( 'NONE',  ( 9.894842273953122103, 1453.125045676060154, 211.4470279248059796 ) ) ;
#35890=CARTESIAN_POINT ( 'NONE',  ( 8.453089846490000170, 1424.727987169319931, 195.6886735564989976 ) ) ;
#35891=EDGE_LOOP ( 'NONE', ( #81713, #64444, #57029, #41431 ) ) ;
#35893=CARTESIAN_POINT ( 'NONE',  ( -2.409034624560000282, 1512.051704408390151, 213.5301952362090105 ) ) ;
#35900=CARTESIAN_POINT ( 'NONE',  ( -14.17232384770000131, 1420.119835273649869, 215.1506258166890007 ) ) ;
#35904=VERTEX_POINT ( 'NONE', #46168 ) ;
#35912=CARTESIAN_POINT ( 'NONE',  ( -9.346796821772709762, 1471.356213985179920, 213.0927830673160202 ) ) ;
#35915=CARTESIAN_POINT ( 'NONE',  ( 9.181100887863649973, 1450.964097471789955, 210.1935140534000084 ) ) ;
#35916=CARTESIAN_POINT ( 'NONE',  ( -7.009441893950000058, 1474.031553669390178, 201.0250566641990133 ) ) ;
#35917=CARTESIAN_POINT ( 'NONE',  ( 10.76609234380000046, 1492.646438831789965, 213.2464151773390029 ) ) ;
#35920=CARTESIAN_POINT ( 'NONE',  ( -19.14812029890000034, 1505.318613837190014, 209.0594768593419985 ) ) ;
#35921=LINE ( 'NONE', #62244, #36582 ) ;
#35923=CIRCLE ( 'NONE', #98478, 3.750000000000000000 ) ;
#35924=CARTESIAN_POINT ( 'NONE',  ( -9.959708506167800124, 1439.533817592069909, 208.3028740885160062 ) ) ;
#35930=CARTESIAN_POINT ( 'NONE',  ( 4.944374238289999113, 1505.309208253089992, 220.4536355099990033 ) ) ;
#35931=CARTESIAN_POINT ( 'NONE',  ( -14.47420009890000081, 1416.181292664740113, 214.4142689833190047 ) ) ;
#35932=CARTESIAN_POINT ( 'NONE',  ( 1.548360550803739910, 1515.071586600679893, 204.7925750858499896 ) ) ;
#35934=CARTESIAN_POINT ( 'NONE',  ( 4.781276783620000081, 1452.020048942890071, 190.5513815401990030 ) ) ;
#35937=CARTESIAN_POINT ( 'NONE',  ( -16.52551917950000160, 1417.103176096179823, 208.5467600217809832 ) ) ;
#35939=CARTESIAN_POINT ( 'NONE',  ( 1.007052846431199411, 1444.164410995541857, 218.0138153337278482 ) ) ;
#35941=CARTESIAN_POINT ( 'NONE',  ( -2.170627987649289992, 1485.611815795640041, 197.4219879416550327 ) ) ;
#35945=CARTESIAN_POINT ( 'NONE',  ( -11.39043170617670064, 1482.032881333110026, 208.0372395411779962 ) ) ;
#35953=CARTESIAN_POINT ( 'NONE',  ( 2.768651645099999836, 1478.720412810289872, 229.3713484223989951 ) ) ;
#35954=CARTESIAN_POINT ( 'NONE',  ( -14.97307836811019932, 1417.870019438920053, 203.2001793081319931 ) ) ;
#35957=CARTESIAN_POINT ( 'NONE',  ( -15.88408514909999880, 1416.392489341679948, 208.4668446563049997 ) ) ;
#35965=CARTESIAN_POINT ( 'NONE',  ( 11.63974220683948779, 1435.319261371113043, 224.2611706537471719 ) ) ;
#35977=CARTESIAN_POINT ( 'NONE',  ( -11.03352569490000157, 1462.446813036689946, 208.7213868678359745 ) ) ;
#35978=CARTESIAN_POINT ( 'NONE',  ( 4.329448813750000014, 1515.064791442790010, 207.6699222060090051 ) ) ;
#35984=CARTESIAN_POINT ( 'NONE',  ( -14.20525283303160080, 1416.384016890880048, 203.1489016136929706 ) ) ;
#35985=CARTESIAN_POINT ( 'NONE',  ( 5.145337980659999921, 1422.426138373190042, 194.5914561771990066 ) ) ;
#35988=CARTESIAN_POINT ( 'NONE',  ( -9.913669495620000660, 1449.457131675590063, 190.8767303025989861 ) ) ;
#35990=CARTESIAN_POINT ( 'NONE',  ( -12.04602610265449947, 1481.198043685850052, 227.9689298190359921 ) ) ;
#35993=CARTESIAN_POINT ( 'NONE',  ( -5.028436728809999146, 1391.796861381390045, 203.7103736513389833 ) ) ;
#35994=CARTESIAN_POINT ( 'NONE',  ( 9.796705758833221367, 1435.283077638600162, 208.5591499206929882 ) ) ;
#35995=CARTESIAN_POINT ( 'NONE',  ( -10.90499273530000046, 1491.392513267690219, 210.6662861634189881 ) ) ;
#36002=CARTESIAN_POINT ( 'NONE',  ( 10.70119619629079999, 1502.850065394879948, 214.5617076214280132 ) ) ;
#36003=CARTESIAN_POINT ( 'NONE',  ( -9.434181852818266378, 1422.844516205027048, 210.7101302893215120 ) ) ;
#36018=B_SPLINE_CURVE_WITH_KNOTS ( 'NONE', 5,
 ( #77188, #83354, #41372, #57641, #42460, #8298, #32948, #49229, #59836 ),
 .UNSPECIFIED., .F., .F.,
 ( 6, 3, 6 ),
 ( 0.000000000000000000, 0.7482103374986269761, 1.000000000000000000 ),
 .UNSPECIFIED. ) ;
#36020=CARTESIAN_POINT ( 'NONE',  ( -0.5477602106990010489, 1469.061648626090118, 219.1663329555989890 ) ) ;
#36024=CARTESIAN_POINT ( 'NONE',  ( -8.279722129557768540, 1423.369210425909841, 209.8234668683010113 ) ) ;
#36030=ORIENTED_EDGE ( 'NONE', *, *, #1511, .F. ) ;
#36031=VERTEX_POINT ( 'NONE', #33724 ) ;
#36037=CARTESIAN_POINT ( 'NONE',  ( 0.08355061096887030081, 1465.424449796589897, 198.1142439294760038 ) ) ;
#36044=CARTESIAN_POINT ( 'NONE',  ( 8.651090045271681461, 1437.459470016739942, 208.9048937552290113 ) ) ;
#36047=VERTEX_POINT ( 'NONE', #49455 ) ;
#36055=CARTESIAN_POINT ( 'NONE',  ( -0.2452586311791360163, 1422.882060582030135, 192.4945411992279958 ) ) ;
#36059=CARTESIAN_POINT ( 'NONE',  ( -7.354862284149999319, 1508.833542331989975, 219.0557158588990205 ) ) ;
#36060=LINE ( 'NONE', #50645, #105793 ) ;
#36061=CARTESIAN_POINT ( 'NONE',  ( 8.909957024879078702, 1434.607635241320168, 206.3240561870909744 ) ) ;
#36085=CARTESIAN_POINT ( 'NONE',  ( -8.949166976945781116, 1508.433673422140146, 219.1618437498449907 ) ) ;
#36089=CARTESIAN_POINT ( 'NONE',  ( -19.82380892210000312, 1467.090503478189930, 209.9302942427229937 ) ) ;
#36090=CARTESIAN_POINT ( 'NONE',  ( 0.5135905785996027761, 1469.225700524577405, 219.1587014438361223 ) ) ;
#36095=CARTESIAN_POINT ( 'NONE',  ( -0.06016446275539899524, 1431.826830952890077, 200.6931156591689955 ) ) ;
#36096=CARTESIAN_POINT ( 'NONE',  ( -15.85591190879999779, 1415.880081504350073, 209.4912631162540038 ) ) ;
#36097=CARTESIAN_POINT ( 'NONE',  ( -0.9486860776340020340, 1507.879202551890103, 220.9616002900989997 ) ) ;
#36098=CARTESIAN_POINT ( 'NONE',  ( 1.582067810090000045E-15, 1508.551704408389924, 209.1218459616989946 ) ) ;
#36102=CARTESIAN_POINT ( 'NONE',  ( -0.1560728617379990024, 1485.890437600389760, 197.6029597742989949 ) ) ;
#36103=CARTESIAN_POINT ( 'NONE',  ( 6.487764263893970096, 1466.799890030109964, 201.2724796736299879 ) ) ;
#36105=DIRECTION ( 'NONE',  ( -1.000000000000000000, 0.000000000000000000, 0.000000000000000000 ) ) ;
#36107=CARTESIAN_POINT ( 'NONE',  ( 8.482143754180000883, 1423.325759885000025, 211.9865062201690193 ) ) ;
#36111=CARTESIAN_POINT ( 'NONE',  ( -10.28192841989999984, 1482.564960466189859, 205.0245988223590246 ) ) ;
#36114=ORIENTED_EDGE ( 'NONE', *, *, #13931, .F. ) ;
#36119=CARTESIAN_POINT ( 'NONE',  ( -11.39431203569762552, 1501.174835975778933, 208.1498517562084487 ) ) ;
#36120=CARTESIAN_POINT ( 'NONE',  ( -13.58681706775159981, 1508.455392534539897, 209.9114426240880107 ) ) ;
#36121=CARTESIAN_POINT ( 'NONE',  ( 2.963088497139999777, 1449.560975490390092, 190.2511718989990186 ) ) ;
#36123=CARTESIAN_POINT ( 'NONE',  ( -9.842956191871440552, 1438.561763663640022, 210.4747371474470015 ) ) ;
#36125=CARTESIAN_POINT ( 'NONE',  ( -8.835157404840000339, 1450.736626986090187, 204.9140208344290102 ) ) ;
#36127=CARTESIAN_POINT ( 'NONE',  ( 7.774392068240000064, 1425.884050503550270, 211.7695909195089996 ) ) ;
#36128=CARTESIAN_POINT ( 'NONE',  ( -19.04700360180000374, 1444.155872993190087, 199.5980005317190091 ) ) ;
#36140=CARTESIAN_POINT ( 'NONE',  ( 6.271138058716076991, 1499.936577760534874, 199.6202075728144507 ) ) ;
#36143=CARTESIAN_POINT ( 'NONE',  ( 2.239840163258520089, 1476.242923025720074, 197.8476420570929974 ) ) ;
#36156=CARTESIAN_POINT ( 'NONE',  ( -3.205906119050000225, 1454.493865833489963, 199.5427769187489844 ) ) ;
#36169=CARTESIAN_POINT ( 'NONE',  ( 9.213513262295309758, 1461.925794281050003, 206.0128988621550263 ) ) ;
#36174=CARTESIAN_POINT ( 'NONE',  ( -12.02051104499999923, 1491.153688735689911, 206.6632163132790083 ) ) ;
#36182=CARTESIAN_POINT ( 'NONE',  ( 13.69810584925325259, 1494.139388547490398, 192.1978378177635705 ) ) ;
#36209=CARTESIAN_POINT ( 'NONE',  ( 2.736568218950000020, 1441.973427766389932, 217.9247250662190254 ) ) ;
#36210=CARTESIAN_POINT ( 'NONE',  ( -3.271538019026510202, 1454.292002138270163, 199.1638778078030043 ) ) ;
#36226=CARTESIAN_POINT ( 'NONE',  ( -10.43765270066229967, 1479.571382516360018, 210.2075621104870038 ) ) ;
#36229=CARTESIAN_POINT ( 'NONE',  ( -4.376494698527389815, 1488.973636533830131, 219.1697672411899873 ) ) ;
#36230=CARTESIAN_POINT ( 'NONE',  ( -0.3862383889521530111, 1500.063189114229999, 233.1571762794760048 ) ) ;
#36235=DIRECTION ( 'NONE',  ( -1.000000000000000000, 0.000000000000000000, 0.000000000000000000 ) ) ;
#36236=VERTEX_POINT ( 'NONE', #91447 ) ;
#36247=CARTESIAN_POINT ( 'NONE',  ( 8.754875282535529379, 1436.430644587890129, 208.9268862815009982 ) ) ;
#36249=CARTESIAN_POINT ( 'NONE',  ( 0.1543026821579989993, 1487.992631772989853, 217.2489902802990116 ) ) ;
#36254=CARTESIAN_POINT ( 'NONE',  ( -9.204572690731579243, 1450.041973421969942, 209.1554608508139950 ) ) ;
#36257=ORIENTED_EDGE ( 'NONE', *, *, #7650, .T. ) ;
#36258=CARTESIAN_POINT ( 'NONE',  ( -3.224549562455830021, 1508.551704408489968, 213.9552827710969893 ) ) ;
#36259=CARTESIAN_POINT ( 'NONE',  ( 9.992014340670891670, 1491.422427633320012, 188.4943361087159985 ) ) ;
#36272=CARTESIAN_POINT ( 'NONE',  ( -8.782009155840000858, 1423.187680728870191, 210.2326933490990086 ) ) ;
#36278=DIRECTION ( 'NONE',  ( 0.9999994573234139983, 9.540975887252238799E-32, -0.001041802705676339504 ) ) ;
#36284=CARTESIAN_POINT ( 'NONE',  ( -16.32084964895840073, 1508.551704408389924, 213.4499384416680243 ) ) ;
#36285=CARTESIAN_POINT ( 'NONE',  ( 9.986106302860001449, 1472.420748959189950, 214.7747459013789921 ) ) ;
#36286=CARTESIAN_POINT ( 'NONE',  ( -9.105587270462899951, 1439.161147590870087, 208.1449012116760002 ) ) ;
#36291=CARTESIAN_POINT ( 'NONE',  ( 8.899191358356040027, 1435.476522257870101, 207.7847561027849963 ) ) ;
#36296=EDGE_CURVE ( 'NONE', #38904, #43913, #109359, .T. ) ;
#36314=CARTESIAN_POINT ( 'NONE',  ( 7.571416214730000149, 1423.019345440409779, 195.7264161940989879 ) ) ;
#36316=CARTESIAN_POINT ( 'NONE',  ( -4.037927790559999508, 1496.698780035289928, 198.6284372844990003 ) ) ;
#36320=CARTESIAN_POINT ( 'NONE',  ( 2.175409717514719593E-31, 1397.551704408390151, 209.1218459616989946 ) ) ;
#36330=EDGE_CURVE ( 'NONE', #101391, #52522, #52228, .T. ) ;
#36331=CARTESIAN_POINT ( 'NONE',  ( -1.288421119806714588, 1420.729263807338157, 193.7694644859544724 ) ) ;
#36333=CARTESIAN_POINT ( 'NONE',  ( 19.41976554590000248, 1457.605858504690104, 210.0668255001349962 ) ) ;
#36338=CARTESIAN_POINT ( 'NONE',  ( 4.163336342339999869E-15, 1416.181292664740113, 209.1218459616989946 ) ) ;
#36339=CARTESIAN_POINT ( 'NONE',  ( -10.82576510151410076, 1461.830236086719879, 211.0839844832650272 ) ) ;
#36342=CARTESIAN_POINT ( 'NONE',  ( -9.385734277025909122, 1422.648365155559986, 192.2754659541220121 ) ) ;
#36343=VERTEX_POINT ( 'NONE', #25309 ) ;
#36348=CARTESIAN_POINT ( 'NONE',  ( -4.925340228020513855, 1491.207026113694155, 188.8237031222513451 ) ) ;
#36350=CARTESIAN_POINT ( 'NONE',  ( -16.47688868883378888, 1420.112172641060852, 208.7131226723711848 ) ) ;
#36358=CARTESIAN_POINT ( 'NONE',  ( 3.626340809789999842, 1441.877721644789972, 217.3328878409490130 ) ) ;
#36365=CARTESIAN_POINT ( 'NONE',  ( 18.38166776770140132, 1428.164217240339894, 201.4944361684150067 ) ) ;
#36367=ADVANCED_FACE ( 'NONE', ( #28093 ), #62856, .T. ) ;
#36370=CARTESIAN_POINT ( 'NONE',  ( -2.487935123020000194, 1508.551704408389924, 214.1089243778970115 ) ) ;
#36374=CARTESIAN_POINT ( 'NONE',  ( -0.6139455675770010279, 1430.723786662589873, 217.4810676936089919 ) ) ;
#36375=CARTESIAN_POINT ( 'NONE',  ( -10.28050713296510033, 1472.193390648910054, 207.1071822515270071 ) ) ;
#36380=CARTESIAN_POINT ( 'NONE',  ( -3.657993755839999750, 1474.872004365689918, 218.7367895275489786 ) ) ;
#36389=CARTESIAN_POINT ( 'NONE',  ( 1.887268207041509882, 1496.992342273679924, 196.8733779563050064 ) ) ;
#36401=CARTESIAN_POINT ( 'NONE',  ( -2.697707841769999781, 1496.152875393589966, 220.1550137170989956 ) ) ;
#36409=FACE_OUTER_BOUND ( 'NONE', #35585, .T. ) ;
#36412=CARTESIAN_POINT ( 'NONE',  ( 3.347837012790000344, 1485.651792710489872, 219.4796433975990055 ) ) ;
#36414=DIRECTION ( 'NONE',  ( 0.9072248115955994230, -0.3865001137603080728, -0.1660144671063280564 ) ) ;
#36422=CARTESIAN_POINT ( 'NONE',  ( 8.853608006785520956, 1452.164931631960144, 211.9660445263369866 ) ) ;
#36423=CARTESIAN_POINT ( 'NONE',  ( 8.607172403139999872, 1425.024168402240093, 195.3267954577989940 ) ) ;
#36427=CARTESIAN_POINT ( 'NONE',  ( -6.349477754588637168, 1419.387435849262829, 195.0908289166754059 ) ) ;
#36436=ORIENTED_EDGE ( 'NONE', *, *, #106284, .F. ) ;
#36438=EDGE_CURVE ( 'NONE', #73608, #26364, #99128, .T. ) ;
#36442=CARTESIAN_POINT ( 'NONE',  ( -6.558694315301119460, 1508.421471884069888, 219.8384412560889984 ) ) ;
#36444=( BOUNDED_SURFACE ( )  B_SPLINE_SURFACE ( 1, 2, ( 
 ( #39295, #21363, #5139, #13518, #37648, #29247, #38735 ),
 ( #71853, #73467, #28141, #29791, #62332, #2975, #89695 ) ),
 .UNSPECIFIED., .F., .F., .T. ) 
 B_SPLINE_SURFACE_WITH_KNOTS ( ( 2, 2 ),
 ( 3, 2, 2, 3 ),
 ( -10000.00000000000000, 10000.00000000000000 ),
 ( 2.609770915052339824, 3.141592653589790007, 4.712388980384689674, 5.770213224332369606 ),
 .UNSPECIFIED. ) 
 GEOMETRIC_REPRESENTATION_ITEM ( )  RATIONAL_B_SPLINE_SURFACE ( (
 ( 0.8688191111210129547, 0.9008356601183090673, 1.000000000000000000, 0.7071067811865480168, 1.000000000000000000, 0.8027563838394459195, 0.8711730262106620604),
 ( 0.8688191111210129547, 0.9008356601183090673, 1.000000000000000000, 0.7071067811865480168, 1.000000000000000000, 0.8027563838394459195, 0.8711730262106620604) ) ) 
 REPRESENTATION_ITEM ( '' )  SURFACE ( )  );
#36445=CARTESIAN_POINT ( 'NONE',  ( -4.824314178002369502, 1468.483533977829893, 219.2782425545100011 ) ) ;
#36450=CARTESIAN_POINT ( 'NONE',  ( -2.449516837986489559, 1422.315028397099923, 192.7719440642819961 ) ) ;
#36453=CARTESIAN_POINT ( 'NONE',  ( 7.443246446248299009, 1423.092341332710021, 195.6161848952980051 ) ) ;
#36454=CARTESIAN_POINT ( 'NONE',  ( -20.30540503779999995, 1505.205473082589833, 209.2397414641690148 ) ) ;
#36457=CARTESIAN_POINT ( 'NONE',  ( -9.932527294720630451, 1439.673512841460024, 207.9640247163430047 ) ) ;
#36463=B_SPLINE_CURVE_WITH_KNOTS ( 'NONE', 3,
 ( #50010, #41606, #26438, #93093, #16909, #67928, #16364, #51114, #15804, #77958, #717, #109907, #59518, #9099, #100929, #34295 ),
 .UNSPECIFIED., .F., .F.,
 ( 4, 3, 3, 3, 3, 4 ),
 ( -7.690120649562800281, -7.200842779664780480, -6.186030432389340028, -5.174050502141839480, -4.163300565000019660, -3.154256035599999564 ),
 .UNSPECIFIED. ) ;
#36468=CARTESIAN_POINT ( 'NONE',  ( 5.123510356189999726, 1506.385164154990207, 219.6030550502989911 ) ) ;
#36470=CARTESIAN_POINT ( 'NONE',  ( -1.700207153400070004, 1515.066230056300128, 204.7924348194040078 ) ) ;
#36474=CARTESIAN_POINT ( 'NONE',  ( -15.89685123880000006, 1415.918798422770124, 209.5438913505039977 ) ) ;
#36475=CARTESIAN_POINT ( 'NONE',  ( -6.436826263860000452, 1460.741096996990109, 209.1237132485140080 ) ) ;
#36484=CARTESIAN_POINT ( 'NONE',  ( -4.652798870049999813, 1476.958451974490117, 219.7229608691989995 ) ) ;
#36492=EDGE_CURVE ( 'NONE', #37425, #73065, #92551, .T. ) ;
#36494=CARTESIAN_POINT ( 'NONE',  ( -1.197716701820000118, 1479.406703890490007, 229.6030852470990169 ) ) ;
#36498=CARTESIAN_POINT ( 'NONE',  ( 18.83903520582832414, 1477.219481574037900, 217.3633840002517843 ) ) ;
#36505=ORIENTED_EDGE ( 'NONE', *, *, #61441, .F. ) ;
#36510=CARTESIAN_POINT ( 'NONE',  ( -13.59448967766789806, 1507.983772107289951, 209.3963046402899977 ) ) ;
#36515=ADVANCED_FACE ( 'NONE', ( #15658 ), #75949, .F. ) ;
#36522=CARTESIAN_POINT ( 'NONE',  ( -10.63631708518249752, 1493.561200479843819, 205.8325361800690132 ) ) ;
#36523=CARTESIAN_POINT ( 'NONE',  ( 3.984081798389999651, 1515.551704150889918, 207.2788819995389815 ) ) ;
#36528=CARTESIAN_POINT ( 'NONE',  ( 2.021030077200000274, 1421.580652348860212, 193.8043510613990179 ) ) ;
#36531=CARTESIAN_POINT ( 'NONE',  ( 18.90005065560000119, 1456.739796555589919, 200.1223556290190118 ) ) ;
#36537=CARTESIAN_POINT ( 'NONE',  ( -11.95245250920000046, 1489.692386819589956, 211.6783199228790124 ) ) ;
#36543=CARTESIAN_POINT ( 'NONE',  ( 7.287626706846419999, 1504.670790707109973, 218.7321252575409858 ) ) ;
#36552=CARTESIAN_POINT ( 'NONE',  ( -2.401759440763739040, 1456.579829547543568, 199.9421882610167245 ) ) ;
#36553=CARTESIAN_POINT ( 'NONE',  ( 11.07826983750000061, 1500.667907230989840, 205.8218841770989798 ) ) ;
#36558=CARTESIAN_POINT ( 'NONE',  ( 0.03360429821169879511, 1468.905055714589935, 219.1740298947989913 ) ) ;
#36564=CARTESIAN_POINT ( 'NONE',  ( -12.95799293189999979, 1421.417920776069877, 210.6553815501089844 ) ) ;
#36568=CARTESIAN_POINT ( 'NONE',  ( -12.14766904159599825, 1440.691551917680044, 223.4139461185880009 ) ) ;
#36574=EDGE_CURVE ( 'NONE', #49356, #34770, #12452, .T. ) ;
#36577=CARTESIAN_POINT ( 'NONE',  ( 9.870105591850000692, 1461.985261895689973, 208.8208347412080172 ) ) ;
#36578=CARTESIAN_POINT ( 'NONE',  ( -18.40330103019589814, 1508.551701338139992, 210.4131062939880223 ) ) ;
#36582=VECTOR ( 'NONE', #70653, 1000.000000000000000 ) ;
#36587=EDGE_CURVE ( 'NONE', #109446, #58146, #104642, .T. ) ;
#36600=CARTESIAN_POINT ( 'NONE',  ( -0.8415958139899989421, 1498.413741156690094, 200.5784037818789898 ) ) ;
#36603=CARTESIAN_POINT ( 'NONE',  ( -0.06914114004050241069, 1462.882045625689898, 228.8295648571990171 ) ) ;
#36607=CARTESIAN_POINT ( 'NONE',  ( -11.49316453475270094, 1482.710248906200150, 206.0058552507379943 ) ) ;
#36610=VERTEX_POINT ( 'NONE', #98459 ) ;
#36615=CARTESIAN_POINT ( 'NONE',  ( -14.31200009510000015, 1415.739699867260015, 203.9225122001990087 ) ) ;
#36620=ADVANCED_FACE ( 'NONE', ( #2240 ), #14188, .T. ) ;
#36623=CARTESIAN_POINT ( 'NONE',  ( -9.466486982440619258, 1449.314193870430017, 207.5699851590599962 ) ) ;
#36629=CARTESIAN_POINT ( 'NONE',  ( 1.842963219479999859, 1515.064792519189950, 213.4512947472589985 ) ) ;
#36635=CARTESIAN_POINT ( 'NONE',  ( 3.135857944719999679, 1466.984112378690043, 218.9566967715590238 ) ) ;
#36638=DIRECTION ( 'NONE',  ( -0.1481527700395769420, 0.3686965082634817703, 0.9176675005272424412 ) ) ;
#36639=CARTESIAN_POINT ( 'NONE',  ( 0.4140934722930009748, 1432.034230537489975, 200.6936621557090064 ) ) ;
#36640=CARTESIAN_POINT ( 'NONE',  ( 9.183393462700504273, 1463.661249169792200, 215.2717992091796475 ) ) ;
#36641=CARTESIAN_POINT ( 'NONE',  ( 0.7301356836779989701, 1507.011728406289876, 221.2028043055989883 ) ) ;
#36642=CARTESIAN_POINT ( 'NONE',  ( -18.60492040140000114, 1442.815685133389934, 206.3625141719689964 ) ) ;
#36646=CARTESIAN_POINT ( 'NONE',  ( 4.498205314171340952, 1465.056958170999906, 200.2655687005689913 ) ) ;
#36654=CARTESIAN_POINT ( 'NONE',  ( -10.43759599350000045, 1482.453041218790077, 205.4625892378089986 ) ) ;
#36656=AXIS2_PLACEMENT_3D ( 'NONE', #85424, #58604, #17658 ) ;
#36659=( BOUNDED_CURVE ( )  B_SPLINE_CURVE ( 3, ( #103168, #26470, #1295, #60664 ),
 .UNSPECIFIED., .F., .T. ) 
 B_SPLINE_CURVE_WITH_KNOTS ( ( 4, 4 ),
 ( 1.006279808626920014, 2.135312847049839924 ),
 .UNSPECIFIED. ) 
 CURVE ( )  GEOMETRIC_REPRESENTATION_ITEM ( )  RATIONAL_B_SPLINE_CURVE ( ( 1.000000000000000000, 0.8965649099742322159, 0.8965649099742322159, 1.000000000000000000 ) ) 
 REPRESENTATION_ITEM ( '' )  );
#36660=CARTESIAN_POINT ( 'NONE',  ( -2.825661703002820158, 1508.551704408389924, 204.1562177343460007 ) ) ;
#36664=CARTESIAN_POINT ( 'NONE',  ( -11.37084677945475164, 1501.461804469615572, 207.7930807248614258 ) ) ;
#36665=CARTESIAN_POINT ( 'NONE',  ( -13.58041510073769942, 1508.551704408389924, 210.3416170870220014 ) ) ;
#36673=CARTESIAN_POINT ( 'NONE',  ( 7.539740262130000481, 1425.605416228270087, 212.1797667491989898 ) ) ;
#36674=CARTESIAN_POINT ( 'NONE',  ( -9.838224505759999516, 1462.268909614690074, 227.9668215275989667 ) ) ;
#36679=CARTESIAN_POINT ( 'NONE',  ( 8.040162348720000907, 1454.435424808689959, 215.4819357908390316 ) ) ;
#36681=EDGE_LOOP ( 'NONE', ( #48848, #36030, #53598, #106424 ) ) ;
#36687=CARTESIAN_POINT ( 'NONE',  ( 21.13734888319999783, 1496.938803861589804, 209.1218459616989946 ) ) ;
#36701=CARTESIAN_POINT ( 'NONE',  ( -3.668914018200000182, 1454.923457869790127, 200.3099103192890027 ) ) ;
#36706=FACE_OUTER_BOUND ( 'NONE', #1192, .T. ) ;
#36712=B_SPLINE_CURVE_WITH_KNOTS ( 'NONE', 5,
 ( #105970, #63437, #38191, #96456, #97555, #37093, #20829, #55024, #105408, #28701, #53937, #62906, #97017, #106502, #89151 ),
 .UNSPECIFIED., .F., .F.,
 ( 6, 3, 3, 3, 6 ),
 ( 0.000000000000000000, 0.2761287575458264421, 0.5540238061273354830, 0.8350199265002417048, 1.000000000000000000 ),
 .UNSPECIFIED. ) ;
#36713=CARTESIAN_POINT ( 'NONE',  ( 2.330134126090000368, 1515.551704408389924, 212.9514660752490158 ) ) ;
#36723=CARTESIAN_POINT ( 'NONE',  ( -4.460976907891178733, 1441.968611084702388, 201.4736981887971865 ) ) ;
#36729=CARTESIAN_POINT ( 'NONE',  ( 16.37089355035010030, 1427.986872975570122, 201.3297975146790009 ) ) ;
#36730=VECTOR ( 'NONE', #73825, 1000.000000000000000 ) ;
#36731=CARTESIAN_POINT ( 'NONE',  ( 9.738306733412100513, 1493.400156934610095, 188.2659883396410123 ) ) ;
#36733=ORIENTED_EDGE ( 'NONE', *, *, #40371, .T. ) ;
#36750=CARTESIAN_POINT ( 'NONE',  ( 10.94246130620789970, 1470.964434095790239, 209.6243324065490015 ) ) ;
#36757=CARTESIAN_POINT ( 'NONE',  ( 4.629464564640000113, 1426.297974515259966, 211.0805667635490011 ) ) ;
#36759=CARTESIAN_POINT ( 'NONE',  ( 3.149572309329999875, 1442.624013563290191, 217.4256031491790111 ) ) ;
#36762=B_SPLINE_CURVE_WITH_KNOTS ( 'NONE', 5,
 ( #2330, #104755, #19636, #53838, #87977, #90137, #99634, #99086, #90693 ),
 .UNSPECIFIED., .F., .F.,
 ( 6, 3, 6 ),
 ( 0.000000000000000000, 0.5437164176757826040, 1.000000000000000000 ),
 .UNSPECIFIED. ) ;
#36776=CARTESIAN_POINT ( 'NONE',  ( -3.428557866510000274, 1483.455582133289909, 199.0092266202990174 ) ) ;
#36777=CARTESIAN_POINT ( 'NONE',  ( -16.42371717981465906, 1417.596043028402619, 205.5727573974847076 ) ) ;
#36781=CARTESIAN_POINT ( 'NONE',  ( -11.24888976860679968, 1470.384811285099886, 210.8887443170019935 ) ) ;
#36782=CARTESIAN_POINT ( 'NONE',  ( -7.501016434054790238, 1489.462053520290056, 217.1422798885779741 ) ) ;
#36783=CARTESIAN_POINT ( 'NONE',  ( -0.03315926146910300187, 1502.038558776489936, 233.2541124319990047 ) ) ;
#36790=ORIENTED_EDGE ( 'NONE', *, *, #96767, .F. ) ;
#36801=CARTESIAN_POINT ( 'NONE',  ( -5.187859588409159173, 1494.961024232720092, 197.9425774163800327 ) ) ;
#36804=CARTESIAN_POINT ( 'NONE',  ( -0.6387392339020010468, 1488.293180997690115, 217.2118250028790101 ) ) ;
#36808=CARTESIAN_POINT ( 'NONE',  ( -1.694729585588290011, 1515.066341861390129, 213.4512541762859996 ) ) ;
#36810=CARTESIAN_POINT ( 'NONE',  ( -9.641170858363588891, 1424.230922240009932, 204.6135712703660090 ) ) ;
#36814=CARTESIAN_POINT ( 'NONE',  ( -11.93942137219999999, 1507.056495409390209, 208.6096073126149975 ) ) ;
#36816=CARTESIAN_POINT ( 'NONE',  ( -5.659004368249999750, 1491.641286619889797, 185.8655773011990107 ) ) ;
#36821=CARTESIAN_POINT ( 'NONE',  ( 4.328991615394299330, 1515.082251143320036, 210.4834250158149871 ) ) ;
#36824=CARTESIAN_POINT ( 'NONE',  ( -6.802668042220000544, 1459.333277144890189, 216.9857242932490067 ) ) ;
#36832=CARTESIAN_POINT ( 'NONE',  ( -5.898813458170000246, 1474.065724237490031, 199.2881457417290108 ) ) ;
#36833=CARTESIAN_POINT ( 'NONE',  ( -3.313501335607589748, 1397.551704408390151, 203.0565224509919915 ) ) ;
#36837=CARTESIAN_POINT ( 'NONE',  ( 3.775314256393730084, 1507.374707593759922, 220.2027404254530154 ) ) ;
#36839=CARTESIAN_POINT ( 'NONE',  ( -18.51989805858369920, 1508.551704408389924, 210.2057868587989731 ) ) ;
#36841=CARTESIAN_POINT ( 'NONE',  ( -9.510122433503239492, 1439.432175621480155, 208.1922871124760093 ) ) ;
#36842=ORIENTED_EDGE ( 'NONE', *, *, #51525, .T. ) ;
#36851=CARTESIAN_POINT ( 'NONE',  ( 2.324366880823700132, 1466.792378440680068, 219.9346284353489978 ) ) ;
#36865=CARTESIAN_POINT ( 'NONE',  ( 3.116127822634939815, 1509.034536885679927, 204.6344861955039960 ) ) ;
#36869=LINE ( 'NONE', #87278, #43140 ) ;
#36879=CARTESIAN_POINT ( 'NONE',  ( -17.01462653269999947, 1417.417567022180037, 207.6637925360890051 ) ) ;
#36881=CARTESIAN_POINT ( 'NONE',  ( -7.637723194635209545, 1484.320820859400101, 199.9856414351459932 ) ) ;
#36897=CARTESIAN_POINT ( 'NONE',  ( 9.576461961311400373, 1463.549209214470011, 211.2185630534640097 ) ) ;
#36900=CARTESIAN_POINT ( 'NONE',  ( -19.06177932457689295, 1488.336581673826686, 199.7544505207700070 ) ) ;
#36902=DIRECTION ( 'NONE',  ( 1.000000000000000000, 0.000000000000000000, 0.000000000000000000 ) ) ;
#36908=CARTESIAN_POINT ( 'NONE',  ( 8.781724162916820120, 1451.721506209049949, 212.1163246891099732 ) ) ;
#36912=B_SPLINE_CURVE_WITH_KNOTS ( 'NONE', 3,
 ( #32062, #100895, #24192, #57301, #6311, #67343, #74085, #40457, #84110, #32620, #57837, #6847, #108214, #66795, #58379, #75731, #91427, #109875, #50532, #33154, #58928, #93059, #16333, #42123, #31502, #110420, #67894, #102001, #65682, #59488, #93598, #17996, #17429, #18544 ),
 .UNSPECIFIED., .F., .F.,
 ( 4, 3, 3, 3, 3, 3, 3, 3, 3, 3, 3, 4 ),
 ( -2.000000000000000000, -1.872502022310899905, -1.688267240139549985, -1.501795031034689920, -1.314134592350729935, -1.125010883417350005, -0.9354619354659259312, -0.7459537259483131066, -0.5569474984532378770, -0.3696240495077129928, -0.1838865046504070122, 0.000000000000000000 ),
 .UNSPECIFIED. ) ;
#36917=CARTESIAN_POINT ( 'NONE',  ( 18.28862841063420319, 1430.119204692329959, 201.0315373977480249 ) ) ;
#36918=ORIENTED_EDGE ( 'NONE', *, *, #110319, .T. ) ;
#36929=CARTESIAN_POINT ( 'NONE',  ( 10.97962301462450085, 1490.622470617079898, 207.3477770736940045 ) ) ;
#36930=DIRECTION ( 'NONE',  ( 1.000000000000000000, 0.000000000000000000, 0.000000000000000000 ) ) ;
#36933=CARTESIAN_POINT ( 'NONE',  ( -18.73498386431730012, 1442.071135603129960, 209.6995629687959877 ) ) ;
#36934=CARTESIAN_POINT ( 'NONE',  ( 2.391961498639229688, 1497.094853944359784, 196.9517835458970012 ) ) ;
#36936=CARTESIAN_POINT ( 'NONE',  ( 11.84247987984260142, 1427.444780555890020, 208.6785203155049828 ) ) ;
#36939=CARTESIAN_POINT ( 'NONE',  ( 3.279726742559999852, 1445.963864114290118, 200.3213863680089730 ) ) ;
#36945=DIRECTION ( 'NONE',  ( 1.000000000000000000, 1.810374147724000060E-32, 1.224646799147351975E-16 ) ) ;
#36946=CARTESIAN_POINT ( 'NONE',  ( 2.475018574370000390, 1497.111080388990104, 196.9667223758990247 ) ) ;
#36947=CARTESIAN_POINT ( 'NONE',  ( -20.11389898556769751, 1487.601351896439837, 204.1067778117269995 ) ) ;
#36952=ADVANCED_FACE ( 'NONE', ( #38154 ), #57150, .T. ) ;
#36970=DIRECTION ( 'NONE',  ( 0.4794255386042031719, 0.000000000000000000, 0.8775825618903726477 ) ) ;
#36973=CARTESIAN_POINT ( 'NONE',  ( 9.993125864493370258, 1452.958822306690081, 210.9634216041149841 ) ) ;
#36974=CARTESIAN_POINT ( 'NONE',  ( 4.993613116619998848, 1423.332947890779906, 194.3851836586989918 ) ) ;
#36997=CARTESIAN_POINT ( 'NONE',  ( -9.702159690257650126, 1471.556315755829928, 212.0784607202180041 ) ) ;
#37001=CARTESIAN_POINT ( 'NONE',  ( -12.74742477238099880, 1502.424001303030082, 209.9689629893190101 ) ) ;
#37002=CARTESIAN_POINT ( 'NONE',  ( 10.81377540340000110, 1493.463431426289844, 215.2021047779490175 ) ) ;
#37004=CARTESIAN_POINT ( 'NONE',  ( 8.507717558044577189, 1424.620342978096460, 195.7232110867650192 ) ) ;
#37005=CARTESIAN_POINT ( 'NONE',  ( -17.70257496129999808, 1504.298185088789978, 209.2114294917570021 ) ) ;
#37006=DIRECTION ( 'NONE',  ( 1.000000000000000000, 0.000000000000000000, 0.000000000000000000 ) ) ;
#37008=CARTESIAN_POINT ( 'NONE',  ( -9.965372901819408824, 1439.491959218489910, 208.4032164217179854 ) ) ;
#37010=ORIENTED_EDGE ( 'NONE', *, *, #11224, .F. ) ;
#37016=CARTESIAN_POINT ( 'NONE',  ( 5.466273243599998999, 1504.965088730989919, 220.6538119101990105 ) ) ;
#37017=CARTESIAN_POINT ( 'NONE',  ( -15.51438564200000059, 1415.734451527310057, 210.2992275438789989 ) ) ;
#37018=CARTESIAN_POINT ( 'NONE',  ( 12.60620919525579886, 1421.114752853880191, 203.4337117396169958 ) ) ;
#37020=CARTESIAN_POINT ( 'NONE',  ( -15.61900273229925418, 1415.705855514175028, 209.6365545205262890 ) ) ;
#37023=CARTESIAN_POINT ( 'NONE',  ( 4.124127541549999165, 1440.791920158089852, 218.1322488136489994 ) ) ;
#37024=ADVANCED_FACE ( 'NONE', ( #100269 ), #13496, .F. ) ;
#37031=CARTESIAN_POINT ( 'NONE',  ( -4.648405679570000615, 1475.312747251090059, 218.3805770009889784 ) ) ;
#37048=CARTESIAN_POINT ( 'NONE',  ( 3.727273714354999878, 1456.064331771540083, 219.0685001699370105 ) ) ;
#37076=CARTESIAN_POINT ( 'NONE',  ( 0.5871476172820019324, 1421.209716202029767, 193.6933393547989795 ) ) ;
#37079=CARTESIAN_POINT ( 'NONE',  ( -9.724670062538070425, 1448.677161661070159, 190.8206614882809902 ) ) ;
#37085=FACE_OUTER_BOUND ( 'NONE', #46932, .T. ) ;
#37090=CARTESIAN_POINT ( 'NONE',  ( -10.33691510611295072, 1423.136607578389885, 193.7437805996329416 ) ) ;
#37093=CARTESIAN_POINT ( 'NONE',  ( -9.093965512229999604, 1423.880366148619942, 207.4491482849089721 ) ) ;
#37094=CARTESIAN_POINT ( 'NONE',  ( -14.41017938444479185, 1420.830237651402740, 210.6135021038660966 ) ) ;
#37102=CARTESIAN_POINT ( 'NONE',  ( 0.2886576936755593792, 1457.782815465476006, 199.5840498596436134 ) ) ;
#37109=CARTESIAN_POINT ( 'NONE',  ( -0.6482359200730010151, 1468.620574178790093, 219.2670886169990183 ) ) ;
#37114=CARTESIAN_POINT ( 'NONE',  ( -9.200421498919999053, 1422.937291500389847, 210.7384572914190244 ) ) ;
#37118=CARTESIAN_POINT ( 'NONE',  ( -19.04700360180000374, 1444.155872993190087, 199.5980005317190091 ) ) ;
#37119=CARTESIAN_POINT ( 'NONE',  ( -2.645191157576220142, 1430.969724324070285, 201.1795969678530014 ) ) ;
#37120=ORIENTED_EDGE ( 'NONE', *, *, #79567, .F. ) ;
#37123=EDGE_CURVE ( 'NONE', #20110, #86208, #72529, .T. ) ;
#37146=ADVANCED_FACE ( 'NONE', ( #32916 ), #83877, .F. ) ;
#37147=CARTESIAN_POINT ( 'NONE',  ( 8.248015215549999724, 1502.411902838189917, 208.8103458818409877 ) ) ;
#37154=EDGE_CURVE ( 'NONE', #106272, #49433, #49748, .T. ) ;
#37158=CARTESIAN_POINT ( 'NONE',  ( 17.99277867620000038, 1432.534352819589913, 212.7098897757189775 ) ) ;
#37172=CARTESIAN_POINT ( 'NONE',  ( -3.276492809264478723, 1486.691461902717947, 220.6577066230676962 ) ) ;
#37173=CARTESIAN_POINT ( 'NONE',  ( -1.794934993283609614, 1484.669492803836192, 198.5571763550413209 ) ) ;
#37179=CARTESIAN_POINT ( 'NONE',  ( -9.499594844283979711, 1449.194695334430207, 207.7958694408430063 ) ) ;
#37184=CARTESIAN_POINT ( 'NONE',  ( -1.117126662530000036, 1515.456827602489966, 213.3225888563989940 ) ) ;
#37189=ADVANCED_FACE ( 'NONE', ( #99564 ), #32106, .T. ) ;
#37197=CARTESIAN_POINT ( 'NONE',  ( 1.871941823660000059, 1506.355489675189801, 221.3883213455989960 ) ) ;
#37198=CARTESIAN_POINT ( 'NONE',  ( -4.324092179320000007, 1515.269353058490196, 209.4836008490580070 ) ) ;
#37202=CARTESIAN_POINT ( 'NONE',  ( 6.578458372278979560, 1465.931120787709915, 201.5766924354090293 ) ) ;
#37204=CARTESIAN_POINT ( 'NONE',  ( 13.67970179620000160, 1494.136271315190015, 192.1856007679989773 ) ) ;
#37210=CARTESIAN_POINT ( 'NONE',  ( -10.97570620389999974, 1482.624300749189842, 205.8415958148989944 ) ) ;
#37223=DIRECTION ( 'NONE',  ( 9.120238070098449704E-47, -1.000000000000000000, 1.836970198721029688E-16 ) ) ;
#37224=ADVANCED_FACE ( 'NONE', ( #458 ), #107156, .T. ) ;
#37228=CARTESIAN_POINT ( 'NONE',  ( 7.467907613800000455, 1424.983389225890051, 212.2844559904590085 ) ) ;
#37229=CARTESIAN_POINT ( 'NONE',  ( -4.354856984870000502, 1481.954696296189923, 231.1149923864989830 ) ) ;
#37245=DIRECTION ( 'NONE',  ( 0.9526631324121143107, 0.2953532403522530769, -0.07210700074307911656 ) ) ;
#37252=VERTEX_POINT ( 'NONE', #35684 ) ;
#37267=CARTESIAN_POINT ( 'NONE',  ( 7.916532357550000398, 1425.151355441629903, 211.5881757975789981 ) ) ;
#37289=CARTESIAN_POINT ( 'NONE',  ( 6.543292404667510276, 1424.997647815940127, 192.3570860859640277 ) ) ;
#37290=CARTESIAN_POINT ( 'NONE',  ( 16.66443952165710130, 1492.498711326890088, 193.3249459387799902 ) ) ;
#37306=CARTESIAN_POINT ( 'NONE',  ( 10.47511427260239891, 1482.040461736080033, 210.7458695605469927 ) ) ;
#37308=CARTESIAN_POINT ( 'NONE',  ( 10.52924840420589980, 1470.684170504899839, 209.6686858039719823 ) ) ;
#37314=B_SPLINE_CURVE_WITH_KNOTS ( 'NONE', 5,
 ( #21845, #29724, #13452, #81769, #90729, #39789 ),
 .UNSPECIFIED., .F., .F.,
 ( 6, 6 ),
 ( -1.999999509065029990, -6.779759595954004681E-07 ),
 .UNSPECIFIED. ) ;
#37315=CARTESIAN_POINT ( 'NONE',  ( 4.824051484379999977, 1425.779874028899940, 210.3687978271890131 ) ) ;
#37317=CARTESIAN_POINT ( 'NONE',  ( 2.003345808180000187, 1442.032355148490069, 218.4647324736090184 ) ) ;
#37322=CARTESIAN_POINT ( 'NONE',  ( -19.18813880309999931, 1465.797355387890093, 204.3301597990889888 ) ) ;
#37329=CARTESIAN_POINT ( 'NONE',  ( -8.954648243350000314, 1508.433707402489972, 219.1777012664989854 ) ) ;
#37331=CARTESIAN_POINT ( 'NONE',  ( -16.88275388290000123, 1507.705444072489854, 209.4032267757409898 ) ) ;
#37332=CARTESIAN_POINT ( 'NONE',  ( -3.520005857620000178, 1483.900612090289997, 199.0196415985990086 ) ) ;
#37335=CARTESIAN_POINT ( 'NONE',  ( 1.779428962334640207, 1456.357349043589920, 198.6855221538999956 ) ) ;
#37339=CARTESIAN_POINT ( 'NONE',  ( -9.092716900757949361, 1490.074253787619909, 215.3417004495109950 ) ) ;
#37340=CARTESIAN_POINT ( 'NONE',  ( -20.36852816458540261, 1464.956552523959999, 210.9458084407719980 ) ) ;
#37343=CARTESIAN_POINT ( 'NONE',  ( 7.360592667339999728, 1427.547308638959976, 213.0878291651189897 ) ) ;
#37344=CARTESIAN_POINT ( 'NONE',  ( -18.75058736031470019, 1443.878575118040089, 210.7892154803369920 ) ) ;
#37359=AXIS2_PLACEMENT_3D ( 'NONE', #74601, #49941, #84079 ) ;
#37362=CARTESIAN_POINT ( 'NONE',  ( -0.6417514479877001188, 1515.135428326259898, 213.4494450834599775 ) ) ;
#37366=CARTESIAN_POINT ( 'NONE',  ( 4.221033085759999359, 1472.290285735790121, 218.3905899716789918 ) ) ;
#37369=CARTESIAN_POINT ( 'NONE',  ( -2.487923159525530004, 1508.611354624159958, 213.7999901551609980 ) ) ;
#37370=CARTESIAN_POINT ( 'NONE',  ( -5.221937430894320720, 1489.269441483490027, 185.8916500386229984 ) ) ;
#37374=CARTESIAN_POINT ( 'NONE',  ( -2.483162210680000204, 1476.934831334089949, 201.9767984825489862 ) ) ;
#37376=CARTESIAN_POINT ( 'NONE',  ( 4.328546746085200070, 1515.099240016830208, 210.2463711844760041 ) ) ;
#37379=CARTESIAN_POINT ( 'NONE',  ( -6.214213076750000120, 1457.627299019590282, 216.3771072480390103 ) ) ;
#37382=EDGE_LOOP ( 'NONE', ( #13410, #45965, #3687, #39545 ) ) ;
#37383=CARTESIAN_POINT ( 'NONE',  ( -8.001908350489999933, 1424.415893222990007, 210.2813077655789868 ) ) ;
#37386=CARTESIAN_POINT ( 'NONE',  ( -9.791236033121871074, 1446.818000420939825, 212.2240223532789969 ) ) ;
#37391=DIRECTION ( 'NONE',  ( -1.913759484722300243E-19, 1.000000000000000000, -1.836968204960139822E-16 ) ) ;
#37392=B_SPLINE_SURFACE_WITH_KNOTS ( 'NONE', 5, 5, ( 
 ( #37114, #86962, #27613, #10253, #70215, #78573 ),
 ( #88090, #36024, #79689, #11377, #19755, #44992 ),
 ( #71315, #35460, #104319, #1888, #95920, #45549 ),
 ( #79139, #52834, #2448, #69650, #105429, #28163 ),
 ( #36564, #104873, #62351, #9701, #96475, #28718 ),
 ( #60692, #53956, #26496, #18091, #103771, #94815 ),
 ( #43869, #78012, #27073, #61257, #95372, #18636 ),
 ( #76704, #84550, #33579, #17, #34698, #33038 ),
 ( #67227, #68890, #50965, #69439, #68336, #94596 ),
 ( #103554, #110304, #16220, #9496, #59379, #51509 ),
 ( #101323, #59931, #85642, #17314, #52072, #85093 ),
 ( #86205, #8942, #43115, #43663, #35255, #93491 ),
 ( #25729, #24613, #77274, #58808, #77815, #1124 ),
 ( #34151, #572, #67771, #102443, #94048, #92948 ),
 ( #26857, #102992, #41462, #50424, #16762, #92387 ),
 ( #8384, #42553, #75624, #26289, #60478, #15660 ),
 ( #76156, #17875, #49864, #83998, #7298, #109758 ),
 ( #7839, #42007, #101884, #25175, #32129, #108282 ),
 ( #22583, #98774, #100431, #82540, #100967, #99863 ),
 ( #57899, #73602, #66314, #23714, #90925, #83623 ),
 ( #6920, #92034, #81404, #49498, #15306, #41076 ),
 ( #13097, #57362, #83084, #5270, #109403, #22036 ),
 ( #13641, #91486, #56233, #6377, #90363, #75254 ),
 ( #40523, #31569, #74701, #65197, #23160, #14766 ) ),
 .UNSPECIFIED., .F., .F., .F.,
 ( 6, 3, 3, 3, 3, 3, 3, 6 ),
 ( 6, 6 ),
 ( 7.502205049999999709, 15.58712854470000053, 20.12010233590000041, 26.07035490390000021, 28.80892602879999842, 30.17821159120000019, 30.86285437249999930, 31.55357349654520149 ),
 ( -1.110223024629999900E-16, 53.14935204510580036 ),
 .UNSPECIFIED. ) ;
#37398=LINE ( 'NONE', #95644, #87482 ) ;
#37399=CARTESIAN_POINT ( 'NONE',  ( -8.831974440303309137, 1439.830871220620111, 206.5957406833990149 ) ) ;
#37409=CARTESIAN_POINT ( 'NONE',  ( 11.39677682778439838, 1471.132186382680175, 209.6872533683069832 ) ) ;
#37414=CARTESIAN_POINT ( 'NONE',  ( 2.664535259099999805E-15, 1420.121162737279974, 209.1218459616989946 ) ) ;
#37423=CARTESIAN_POINT ( 'NONE',  ( -2.023055664010000143, 1438.317420438290128, 227.6217140021989849 ) ) ;
#37425=VERTEX_POINT ( 'NONE', #72088 ) ;
#37434=CARTESIAN_POINT ( 'NONE',  ( 11.72865777870000059, 1490.920838208090117, 205.3345067772989978 ) ) ;
#37441=CARTESIAN_POINT ( 'NONE',  ( -17.18995323200000058, 1417.426350748869936, 207.0509207859589935 ) ) ;
#37442=CARTESIAN_POINT ( 'NONE',  ( -4.794426340529999386, 1463.608615258990085, 228.2108236244990280 ) ) ;
#37451=CARTESIAN_POINT ( 'NONE',  ( -10.43128891525519997, 1461.757356303399774, 210.7313694234769912 ) ) ;
#37453=CARTESIAN_POINT ( 'NONE',  ( 10.06226723659419875, 1500.632405250589954, 203.5390182893460178 ) ) ;
#37454=ORIENTED_EDGE ( 'NONE', *, *, #15824, .T. ) ;
#37461=CARTESIAN_POINT ( 'NONE',  ( -16.41917143159986026, 1420.127254725630564, 208.8252928080606807 ) ) ;
#37464=CARTESIAN_POINT ( 'NONE',  ( -3.116127437694289792, 1509.034538005060085, 204.6344859856109792 ) ) ;
#37475=CARTESIAN_POINT ( 'NONE',  ( -14.38098269158279940, 1422.143816687460003, 196.2925691453790193 ) ) ;
#37476=ORIENTED_EDGE ( 'NONE', *, *, #44754, .T. ) ;
#37484=CARTESIAN_POINT ( 'NONE',  ( -10.06543680052650203, 1473.157550441890180, 207.3953233922799768 ) ) ;
#37490=CIRCLE ( 'NONE', #19573, 0.2999999999999669598 ) ;
#37491=CARTESIAN_POINT ( 'NONE',  ( 10.91851345119660088, 1489.922152752260217, 208.2558192066160245 ) ) ;
#37493=ORIENTED_EDGE ( 'NONE', *, *, #61812, .F. ) ;
#37497=CARTESIAN_POINT ( 'NONE',  ( 11.48693412901199906, 1427.591069643789979, 209.4851071871740089 ) ) ;
#37509=CARTESIAN_POINT ( 'NONE',  ( 2.257543447819999827, 1497.637321272190093, 197.6769954692990154 ) ) ;
#37521=CARTESIAN_POINT ( 'NONE',  ( 2.137002880650000325, 1486.596861473290119, 219.7231104124990111 ) ) ;
#37523=CARTESIAN_POINT ( 'NONE',  ( 19.75716384889999944, 1473.226869026490021, 205.2905475991589981 ) ) ;
#37530=ORIENTED_EDGE ( 'NONE', *, *, #4050, .F. ) ;
#37533=EDGE_LOOP ( 'NONE', ( #22610, #77926, #9260, #11699 ) ) ;
#37534=CARTESIAN_POINT ( 'NONE',  ( -3.660374594542989968, 1507.478316997890033, 221.4607952786410010 ) ) ;
#37546=ORIENTED_EDGE ( 'NONE', *, *, #42400, .F. ) ;
#37551=ORIENTED_EDGE ( 'NONE', *, *, #10943, .F. ) ;
#37552=VERTEX_POINT ( 'NONE', #47952 ) ;
#37555=CARTESIAN_POINT ( 'NONE',  ( 7.795806952825950376, 1499.846699301729814, 200.6023917261699978 ) ) ;
#37556=CARTESIAN_POINT ( 'NONE',  ( -7.344976460507339766, 1469.674713007590071, 216.6639152125200098 ) ) ;
#37558=VECTOR ( 'NONE', #52004, 1000.000000000000227 ) ;
#37562=DIRECTION ( 'NONE',  ( -9.066331650111889066E-17, 1.000000000000000000, -7.714096702464409664E-17 ) ) ;
#37563=CARTESIAN_POINT ( 'NONE',  ( -18.26050052379999755, 1504.444625823090064, 209.3988868026209786 ) ) ;
#37573=CARTESIAN_POINT ( 'NONE',  ( 5.300910123630000470, 1506.315325122790000, 219.5100740960989754 ) ) ;
#37575=CARTESIAN_POINT ( 'NONE',  ( -17.70335225402379820, 1419.745088214420093, 206.7394850893050204 ) ) ;
#37577=CARTESIAN_POINT ( 'NONE',  ( -15.92643154291071461, 1416.091409276738204, 209.7524194240169777 ) ) ;
#37578=CARTESIAN_POINT ( 'NONE',  ( 19.84405992990000200, 1475.251132489289830, 205.2734896568690033 ) ) ;
#37583=CARTESIAN_POINT ( 'NONE',  ( 7.294923696395279933, 1458.268530975320118, 201.0098625615580090 ) ) ;
#37596=DIRECTION ( 'NONE',  ( 0.02091224828123190022, 0.9990482215818557998, 0.03827961371219716635 ) ) ;
#37598=CARTESIAN_POINT ( 'NONE',  ( 12.51530806464030121, 1427.043259357019906, 206.3792954839019842 ) ) ;
#37605=CARTESIAN_POINT ( 'NONE',  ( 3.992841683700380617, 1455.996149397760064, 218.9659736531049816 ) ) ;
#37608=VERTEX_POINT ( 'NONE', #92154 ) ;
#37612=CARTESIAN_POINT ( 'NONE',  ( -13.35927778977159974, 1507.978183412450107, 209.3898014577139861 ) ) ;
#37616=CARTESIAN_POINT ( 'NONE',  ( 9.722207004026980570, 1428.114070666289763, 212.2005352792010058 ) ) ;
#37623=CARTESIAN_POINT ( 'NONE',  ( 3.829620175029999629, 1515.551704176389876, 207.2788819937790095 ) ) ;
#37624=VERTEX_POINT ( 'NONE', #31688 ) ;
#37627=( BOUNDED_CURVE ( )  B_SPLINE_CURVE ( 3, ( #84957, #102858, #94461, #58138 ),
 .UNSPECIFIED., .F., .T. ) 
 B_SPLINE_CURVE_WITH_KNOTS ( ( 4, 4 ),
 ( 4.131751671967750283, 5.293027011176480556 ),
 .UNSPECIFIED. ) 
 CURVE ( )  GEOMETRIC_REPRESENTATION_ITEM ( )  RATIONAL_B_SPLINE_CURVE ( ( 1.000000000000000000, 0.8907420144464277545, 0.8907420144464277545, 1.000000000000000000 ) ) 
 REPRESENTATION_ITEM ( '' )  );
#37630=CARTESIAN_POINT ( 'NONE',  ( 1.758980145960000074, 1423.182207406469843, 192.9748505280989832 ) ) ;
#37632=B_SPLINE_SURFACE_WITH_KNOTS ( 'NONE', 5, 5, ( 
 ( #96520, #62965, #97077, #41006, #90858, #58377 ),
 ( #100893, #30401, #99243, #48889, #14145, #48332 ),
 ( #4661, #64592, #24189, #66248, #83017, #98711 ),
 ( #75184, #15770, #6309, #109334, #57298, #13581 ),
 ( #14700, #32617, #40455, #66793, #49972, #15238 ),
 ( #22520, #92503, #90300, #30955, #38799, #107113 ) ),
 .UNSPECIFIED., .F., .F., .F.,
 ( 6, 6 ),
 ( 6, 6 ),
 ( 5.893388375715320038, 9.819929736134680454 ),
 ( 0.000000000000000000, 0.5002947206946759540 ),
 .UNSPECIFIED. ) ;
#37634=CARTESIAN_POINT ( 'NONE',  ( 18.96326924193710184, 1459.304563651490071, 220.4161041720870173 ) ) ;
#37648=CARTESIAN_POINT ( 'NONE',  ( 1776.830386524950200, 5182.767774292099602, -8872.362978888699217 ) ) ;
#37661=CARTESIAN_POINT ( 'NONE',  ( 0.8333005674559990084, 1467.257208946589799, 220.1998364950989924 ) ) ;
#37663=CARTESIAN_POINT ( 'NONE',  ( 9.424585447077209466, 1482.249723839049921, 215.0732731526550197 ) ) ;
#37668=CARTESIAN_POINT ( 'NONE',  ( 17.76546875260000036, 1430.865606781589804, 204.9340536459789917 ) ) ;
#37670=CARTESIAN_POINT ( 'NONE',  ( 18.99432114591609988, 1459.501257801400243, 220.3864165788380092 ) ) ;
#37671=CYLINDRICAL_SURFACE ( 'NONE', #10119, 0.4999999999999449329 ) ;
#37673=EDGE_LOOP ( 'NONE', ( #109639, #12872, #77054, #52399 ) ) ;
#37679=CARTESIAN_POINT ( 'NONE',  ( -2.487935121788300119, 1509.038615937200120, 204.6345961869410246 ) ) ;
#37680=CARTESIAN_POINT ( 'NONE',  ( 10.51639688740000089, 1461.562446843690168, 209.7842554828359880 ) ) ;
#37683=CARTESIAN_POINT ( 'NONE',  ( -0.09961128158209880956, 1464.896202565289968, 198.8671910008989983 ) ) ;
#37687=B_SPLINE_CURVE_WITH_KNOTS ( 'NONE', 5,
 ( #49203, #83331, #6627, #79361, #60354, #26168, #26734, #9388, #9934 ),
 .UNSPECIFIED., .F., .F.,
 ( 6, 3, 6 ),
 ( -3.121899836449999910, -2.731662331479999928, 4.440892098500626162E-16 ),
 .UNSPECIFIED. ) ;
#37690=CIRCLE ( 'NONE', #102004, 11.73843354579999954 ) ;
#37691=CARTESIAN_POINT ( 'NONE',  ( 11.66147129757649914, 1479.066346190409831, 207.6019141534899859 ) ) ;
#37703=FACE_OUTER_BOUND ( 'NONE', #77599, .T. ) ;
#37706=CARTESIAN_POINT ( 'NONE',  ( -2.889942526720000071, 1491.528343827289973, 188.3843089064990011 ) ) ;
#37708=LINE ( 'NONE', #106562, #78419 ) ;
#37713=CARTESIAN_POINT ( 'NONE',  ( -4.273307515800790490, 1483.235679352140096, 199.3608564754620147 ) ) ;
#37717=CARTESIAN_POINT ( 'NONE',  ( 3.552713678799999608E-15, 1415.677402202029953, 209.1218459616989946 ) ) ;
#37720=CARTESIAN_POINT ( 'NONE',  ( -14.39820424329999859, 1415.677402202029953, 205.1327016663190079 ) ) ;
#37731=CARTESIAN_POINT ( 'NONE',  ( -1.491420627269999910, 1515.551704408389924, 213.0272754455090194 ) ) ;
#37735=CARTESIAN_POINT ( 'NONE',  ( 1.813981524939379364, 1464.111506541877816, 199.4724776592340731 ) ) ;
#37741=CARTESIAN_POINT ( 'NONE',  ( -3.994937574034520100, 1430.106198372560129, 201.8091617894969829 ) ) ;
#37746=CARTESIAN_POINT ( 'NONE',  ( -5.411583886059999848, 1438.069580177289936, 208.0725929255889923 ) ) ;
#37752=CARTESIAN_POINT ( 'NONE',  ( 4.391391641444769789, 1465.488788256659973, 200.1904207473230031 ) ) ;
#37756=CARTESIAN_POINT ( 'NONE',  ( 7.805006001919999825, 1501.592229138889934, 206.4628694236189972 ) ) ;
#37760=CARTESIAN_POINT ( 'NONE',  ( 0.9449119460842639873, 1430.444995504165263, 217.4187635772842100 ) ) ;
#37770=EDGE_CURVE ( 'NONE', #12262, #36031, #104157, .T. ) ;
#37771=DIRECTION ( 'NONE',  ( -1.274053389372359975E-11, 4.864808734250780256E-10, -1.000000000000000000 ) ) ;
#37772=VECTOR ( 'NONE', #70956, 1000.000000000000000 ) ;
#37777=CARTESIAN_POINT ( 'NONE',  ( -9.000838837759999933, 1450.837337738590122, 206.6584664167089898 ) ) ;
#37778=B_SPLINE_CURVE_WITH_KNOTS ( 'NONE', 3,
 ( #49276, #83405, #6701, #40856, #75031, #48730, #109183, #32994, #58772, #108613, #32468, #40303, #41966, #100743, #66089, #109719, #102408, #58227, #68300, #76120, #83959, #110260, #67183, #33536, #92351, #7259, #93451, #16722, #15623, #34109, #67736, #101845, #50923, #85053, #42507, #76667, #110816 ),
 .UNSPECIFIED., .F., .F.,
 ( 4, 3, 3, 3, 3, 3, 3, 3, 3, 3, 3, 3, 4 ),
 ( -12.51705759590000078, -12.22413941043480001, -11.58026520907609935, -10.89731576345280040, -10.17759668157450115, -9.397776376799340525, -8.458468502643359699, -7.545168930068030022, -6.795306101010590183, -5.915671535258179681, -5.141253452723230311, -4.456700984109849273, -3.809711666909999295 ),
 .UNSPECIFIED. ) ;
#37780=CARTESIAN_POINT ( 'NONE',  ( 7.678276105319999267, 1426.141326229849938, 211.9767368881090022 ) ) ;
#37781=CARTESIAN_POINT ( 'NONE',  ( 22.14279730899999876, 1473.984189751590065, 210.1089390466149780 ) ) ;
#37787=CARTESIAN_POINT ( 'NONE',  ( 8.301150669200000110, 1452.680711464789965, 213.4379032366990145 ) ) ;
#37814=EDGE_CURVE ( 'NONE', #9164, #2539, #62754, .T. ) ;
#37819=CIRCLE ( 'NONE', #70059, 3.250000000000000000 ) ;
#37838=CARTESIAN_POINT ( 'NONE',  ( 8.972130450985041250, 1425.592216824180241, 193.4866236545800007 ) ) ;
#37845=VERTEX_POINT ( 'NONE', #15293 ) ;
#37847=AXIS2_PLACEMENT_3D ( 'NONE', #104117, #1679, #77279 ) ;
#37856=CARTESIAN_POINT ( 'NONE',  ( -16.38047698457823032, 1416.780647377006062, 208.1117118038502554 ) ) ;
#37858=CARTESIAN_POINT ( 'NONE',  ( 9.941125970135800571, 1469.097218566779929, 207.7382653174890095 ) ) ;
#37865=EDGE_CURVE ( 'NONE', #34771, #102504, #65345, .T. ) ;
#37869=CARTESIAN_POINT ( 'NONE',  ( 2.780476011279999771, 1442.828392787190069, 217.5657236421889991 ) ) ;
#37882=CARTESIAN_POINT ( 'NONE',  ( -11.26545136039999839, 1508.551704408389924, 217.7655129179189828 ) ) ;
#37884=EDGE_CURVE ( 'NONE', #56179, #9541, #94851, .T. ) ;
#37886=CARTESIAN_POINT ( 'NONE',  ( -4.729727150590000484, 1484.839046518389978, 198.6511715847990160 ) ) ;
#37887=CARTESIAN_POINT ( 'NONE',  ( -15.90344751825240799, 1418.061016069739026, 203.7331501587224238 ) ) ;
#37891=CARTESIAN_POINT ( 'NONE',  ( 4.336695207250549799, 1494.691757117450152, 219.8673055875190130 ) ) ;
#37894=CARTESIAN_POINT ( 'NONE',  ( -6.684245985025539127, 1487.813528818469877, 218.7500381969930174 ) ) ;
#37895=CARTESIAN_POINT ( 'NONE',  ( -9.609628710759999137, 1464.248356776189894, 228.1965957863990013 ) ) ;
#37898=CARTESIAN_POINT ( 'NONE',  ( 5.885377578960000022, 1429.730554523590172, 216.6318111531790009 ) ) ;
#37901=B_SPLINE_CURVE_WITH_KNOTS ( 'NONE', 3,
 ( #43873, #52839, #86966, #19759, #19185, #109555, #53389, #58606, #96479, #44433, #87538, #44998, #7630, #79142, #43330, #69094, #103195, #26500, #60696, #18096, #52291, #14098, #80781, #106526, #71876, #105434, #71319, #98112, #29813, #3548, #30909, #99201, #28722, #11919, #62928, #97039, #20850, #37119, #22480, #81860 ),
 .UNSPECIFIED., .F., .F.,
 ( 4, 3, 3, 3, 3, 3, 3, 3, 3, 3, 3, 3, 3, 4 ),
 ( -12.02648879740000076, -11.98563415181089908, -11.30522982652169972, -10.58397085564349993, -9.831326559260959996, -9.032570767541811207, -8.137609212483280174, -7.249943402468200127, -7.107856609420229788, -6.496713401214210037, -5.822552568774050030, -5.084697154694810095, -4.319144763170720935, -3.650975912550000757 ),
 .UNSPECIFIED. ) ;
#37915=CARTESIAN_POINT ( 'NONE',  ( 4.780307568339999591, 1467.625956517089890, 217.8721402715589761 ) ) ;
#37916=CARTESIAN_POINT ( 'NONE',  ( -3.677001408430000229, 1443.877114344990105, 218.5311880179489776 ) ) ;
#37921=CARTESIAN_POINT ( 'NONE',  ( -6.112747810279289595, 1477.579416776660082, 218.9411244695629932 ) ) ;
#37927=CARTESIAN_POINT ( 'NONE',  ( -21.53550188629999695, 1488.484788005089968, 202.1758863209290098 ) ) ;
#37933=B_SPLINE_CURVE_WITH_KNOTS ( 'NONE', 5,
 ( #110687, #48603, #67060, #109057, #58103, #32341, #33979, #50790, #40181 ),
 .UNSPECIFIED., .F., .F.,
 ( 6, 3, 6 ),
 ( 0.000000000000000000, 0.1586384821461520045, 1.000000000000000000 ),
 .UNSPECIFIED. ) ;
#37937=CARTESIAN_POINT ( 'NONE',  ( -8.571847540900000340, 1459.808793802090122, 213.9952768880189922 ) ) ;
#37945=CARTESIAN_POINT ( 'NONE',  ( -9.718888103667799427, 1446.855032085529956, 212.2079679782489734 ) ) ;
#37950=ORIENTED_EDGE ( 'NONE', *, *, #3143, .T. ) ;
#37958=CARTESIAN_POINT ( 'NONE',  ( 8.561929138950318929, 1436.589287696300062, 208.1473329548439892 ) ) ;
#37963=CARTESIAN_POINT ( 'NONE',  ( 11.39798805746750077, 1471.122479896730056, 209.6527432349059836 ) ) ;
#37980=CARTESIAN_POINT ( 'NONE',  ( -6.544148738009999633, 1414.829190269450010, 206.3506811497689739 ) ) ;
#37990=VERTEX_POINT ( 'NONE', #46470 ) ;
#37991=CARTESIAN_POINT ( 'NONE',  ( -17.13241642390000052, 1417.472910479740221, 206.6641778192989989 ) ) ;
#38001=DIRECTION ( 'NONE',  ( -1.000000000000000000, -2.249639673992789970E-32, -1.224646799147350002E-16 ) ) ;
#38004=CARTESIAN_POINT ( 'NONE',  ( 10.72043382369189857, 1500.413529223420028, 204.6654587861600021 ) ) ;
#38010=CARTESIAN_POINT ( 'NONE',  ( -1.249906575759999861, 1443.441360560090061, 200.1672907908790080 ) ) ;
#38011=CARTESIAN_POINT ( 'NONE',  ( 12.24666786109679961, 1501.370948797369920, 211.6632830822960045 ) ) ;
#38017=CARTESIAN_POINT ( 'NONE',  ( -2.487922500652269608, 1508.611354795260013, 204.4437021699770014 ) ) ;
#38019=CARTESIAN_POINT ( 'NONE',  ( -203.9558787908000284, -8382.262153571269664, 2179.147420460110425 ) ) ;
#38021=CARTESIAN_POINT ( 'NONE',  ( 9.707170653865018650, 1452.234477919450001, 209.8040067783620088 ) ) ;
#38025=CARTESIAN_POINT ( 'NONE',  ( 3.136939361377039770, 1508.551704408389924, 204.2190535551970072 ) ) ;
#38028=CARTESIAN_POINT ( 'NONE',  ( -22.19118223659430100, 1483.601855164859899, 216.8114985404419883 ) ) ;
#38032=CARTESIAN_POINT ( 'NONE',  ( -9.659668719498959888, 1460.930246227030011, 210.9154259961320008 ) ) ;
#38034=CARTESIAN_POINT ( 'NONE',  ( -15.61462149936531496, 1419.935087858347742, 211.2718617567576871 ) ) ;
#38042=CARTESIAN_POINT ( 'NONE',  ( 10.85247041220890019, 1489.752500976519968, 207.7569310478100135 ) ) ;
#38059=CARTESIAN_POINT ( 'NONE',  ( -3.271538019026510202, 1454.292002138270163, 199.1638778078030043 ) ) ;
#38061=CARTESIAN_POINT ( 'NONE',  ( 2.045592726109999759, 1498.492550166889941, 197.9893586035990154 ) ) ;
#38069=CARTESIAN_POINT ( 'NONE',  ( 4.329448776040000446, 1515.064792882589927, 210.9648081929590262 ) ) ;
#38071=CARTESIAN_POINT ( 'NONE',  ( 0.9805682090549989738, 1486.537029112289929, 220.0330171165990123 ) ) ;
#38080=CARTESIAN_POINT ( 'NONE',  ( 9.649574114248718359, 1452.507656576000045, 210.4986084856580248 ) ) ;
#38084=CARTESIAN_POINT ( 'NONE',  ( -0.1314063909958990140, 1442.749369516519891, 202.9452824733500051 ) ) ;
#38085=LINE ( 'NONE', #35893, #13321 ) ;
#38094=CARTESIAN_POINT ( 'NONE',  ( 10.75039077348039918, 1481.132873321739908, 213.9959934367710161 ) ) ;
#38099=CARTESIAN_POINT ( 'NONE',  ( -2.672221962908839732, 1508.496458072200085, 220.4565680788469990 ) ) ;
#38101=CARTESIAN_POINT ( 'NONE',  ( -6.488950515515869988, 1468.824231596619939, 218.3969576502859979 ) ) ;
#38103=CARTESIAN_POINT ( 'NONE',  ( 8.757425179709999341, 1421.002068976639976, 196.4497576583989940 ) ) ;
#38104=CARTESIAN_POINT ( 'NONE',  ( 1.831535152954090195, 1474.831757411260014, 220.3926950305869923 ) ) ;
#38108=CARTESIAN_POINT ( 'NONE',  ( -12.68088003869999980, 1503.103876362690016, 208.6356514325480020 ) ) ;
#38113=VERTEX_POINT ( 'NONE', #93395 ) ;
#38117=CARTESIAN_POINT ( 'NONE',  ( 4.944136252469999881, 1506.455065028490026, 219.6922201799989693 ) ) ;
#38119=CARTESIAN_POINT ( 'NONE',  ( 3.387394683297223708, 1486.863201838490568, 198.4078931434325455 ) ) ;
#38120=VERTEX_POINT ( 'NONE', #42446 ) ;
#38121=CARTESIAN_POINT ( 'NONE',  ( 1.529315676469999774, 1429.868337973490043, 217.3144367521890103 ) ) ;
#38124=CARTESIAN_POINT ( 'NONE',  ( 0.6998493108949769281, 1430.651357711089986, 199.7101808117699875 ) ) ;
#38129=CARTESIAN_POINT ( 'NONE',  ( 4.455250013253990282, 1458.875479649829913, 200.5222135128619811 ) ) ;
#38145=CARTESIAN_POINT ( 'NONE',  ( 9.564625103933238393, 1428.147876255639858, 212.3796509962729715 ) ) ;
#38153=ORIENTED_EDGE ( 'NONE', *, *, #19284, .F. ) ;
#38154=FACE_OUTER_BOUND ( 'NONE', #66898, .T. ) ;
#38156=CARTESIAN_POINT ( 'NONE',  ( -10.99776467329999896, 1492.242005317089934, 208.0361729597790088 ) ) ;
#38157=CARTESIAN_POINT ( 'NONE',  ( -8.589458402129759307, 1436.797986341739943, 209.9032590128110201 ) ) ;
#38165=CARTESIAN_POINT ( 'NONE',  ( -7.980162481601299262, 1424.786834349992887, 210.5240428619318322 ) ) ;
#38176=CARTESIAN_POINT ( 'NONE',  ( -1.412825010259999736, 1422.092295416799743, 193.3406738546989914 ) ) ;
#38179=CARTESIAN_POINT ( 'NONE',  ( 1.080077838119999800, 1463.747891711090006, 230.5571479593990034 ) ) ;
#38191=CARTESIAN_POINT ( 'NONE',  ( -8.619814553459999473, 1424.664384728270079, 205.6756477520589783 ) ) ;
#38192=CARTESIAN_POINT ( 'NONE',  ( -11.41393124623838773, 1422.045517156225287, 210.6385245698202198 ) ) ;
#38194=ORIENTED_EDGE ( 'NONE', *, *, #46003, .F. ) ;
#38198=CARTESIAN_POINT ( 'NONE',  ( 2.994586639156319841, 1484.901524374630299, 220.5882564702210118 ) ) ;
#38206=CARTESIAN_POINT ( 'NONE',  ( 8.208364431944110251, 1484.299506827869891, 216.1663257859750047 ) ) ;
#38211=CARTESIAN_POINT ( 'NONE',  ( 14.17511321471899954, 1428.761346845179787, 195.0897062075739825 ) ) ;
#38223=CARTESIAN_POINT ( 'NONE',  ( 0.8851935269000009709, 1465.434339089689956, 198.5254376396989926 ) ) ;
#38238=CARTESIAN_POINT ( 'NONE',  ( -5.244363409054339620, 1434.381075504319824, 217.2110953212229845 ) ) ;
#38247=CARTESIAN_POINT ( 'NONE',  ( -0.1976107320300010128, 1469.705836264889967, 216.4285800060690121 ) ) ;
#38253=CARTESIAN_POINT ( 'NONE',  ( -4.041144483454799818, 1483.296311158560002, 199.2628329227509880 ) ) ;
#38254=CARTESIAN_POINT ( 'NONE',  ( -16.76078030769999927, 1420.494757909599912, 203.1294657649889928 ) ) ;
#38257=CARTESIAN_POINT ( 'NONE',  ( 2.174183498839999729, 1508.551704408389924, 219.6416074559989795 ) ) ;
#38258=CARTESIAN_POINT ( 'NONE',  ( -8.494709133442391646, 1488.072329454872261, 217.7903042299439562 ) ) ;
#38269=CARTESIAN_POINT ( 'NONE',  ( 1.842963808589999974, 1515.492058141890084, 213.2603893764890017 ) ) ;
#38273=CARTESIAN_POINT ( 'NONE',  ( -0.3555850868473771631, 1463.527481276508070, 199.3363023076782952 ) ) ;
#38276=CARTESIAN_POINT ( 'NONE',  ( -6.057897975499958676, 1440.290016138275178, 202.7497801027471382 ) ) ;
#38277=CARTESIAN_POINT ( 'NONE',  ( -6.617556317490000062, 1459.313145877689976, 217.6703565655190005 ) ) ;
#38281=CARTESIAN_POINT ( 'NONE',  ( -4.329448786299999519, 1515.064792490889886, 210.9648092169189795 ) ) ;
#38284=CIRCLE ( 'NONE', #63347, 7.500000000000000000 ) ;
#38291=AXIS2_PLACEMENT_3D ( 'NONE', #41630, #24256, #85265 ) ;
#38292=B_SPLINE_SURFACE_WITH_KNOTS ( 'NONE', 5, 5, ( 
 ( #58240, #73937, #81759, #41437, #33013, #32483, #57152, #108069, #67199 ),
 ( #99656, #83419, #99108, #66655, #6715, #40871, #24047, #5627, #64990 ),
 ( #22385, #101298, #23512, #82870, #100233, #65547, #75047, #91277, #90160 ),
 ( #109199, #24593, #48747, #13441, #57705, #6164, #56585, #90719, #40318 ),
 ( #74500, #92364, #47631, #15637, #5063, #39210, #14003, #31916, #66108 ),
 ( #42525, #76134, #51485, #102967, #68313, #33552, #61985, #76680, #85615 ),
 ( #16197, #551, #67749, #59356, #8915, #94026, #101241, #102422, #34124 ),
 ( #59905, #101859, #110276, #25703, #17289, #68863, #58786, #92925, #43090 ),
 ( #77251, #41985, #85068, #34675, #27799, #96101, #50398, #25153, #84527 ) ),
 .UNSPECIFIED., .F., .F., .F.,
 ( 6, 3, 6 ),
 ( 6, 3, 6 ),
 ( 3.495303171621910288, 6.017914243079999892, 8.540525314547538827 ),
 ( 0.000000000000000000, 1.500000000000000000, 3.000238679058089719 ),
 .UNSPECIFIED. ) ;
#38293=CARTESIAN_POINT ( 'NONE',  ( 12.05020405772690140, 1491.375760444399930, 206.7358482363899839 ) ) ;
#38297=B_SPLINE_CURVE_WITH_KNOTS ( 'NONE', 3,
 ( #97674, #79792, #54058, #88735 ),
 .UNSPECIFIED., .F., .F.,
 ( 4, 4 ),
 ( -19.11832560899999933, -0.3666095563249989198 ),
 .UNSPECIFIED. ) ;
#38301=CARTESIAN_POINT ( 'NONE',  ( -11.33207981915198204, 1503.013677552742820, 207.0720892954946635 ) ) ;
#38303=CARTESIAN_POINT ( 'NONE',  ( -9.624872151419999966, 1503.621315096290118, 228.8144366447990024 ) ) ;
#38311=CARTESIAN_POINT ( 'NONE',  ( 7.513421685239999981, 1426.406794065100030, 212.3389288288790056 ) ) ;
#38312=CARTESIAN_POINT ( 'NONE',  ( 16.50821402049999875, 1494.476688022989947, 193.0250027032990090 ) ) ;
#38323=DIRECTION ( 'NONE',  ( -1.699538841806929935E-33, 1.000000000000000000, -1.698192320643030073E-16 ) ) ;
#38340=CARTESIAN_POINT ( 'NONE',  ( -4.961196303140000374, 1424.964372189380128, 209.4833162189939912 ) ) ;
#38360=ORIENTED_EDGE ( 'NONE', *, *, #82360, .F. ) ;
#38363=AXIS2_PLACEMENT_3D ( 'NONE', #20858, #55055, #96486 ) ;
#38367=AXIS2_PLACEMENT_3D ( 'NONE', #108078, #38672, #49299 ) ;
#38388=CARTESIAN_POINT ( 'NONE',  ( 11.00924500930000072, 1425.566778448970126, 205.8224405914690180 ) ) ;
#38392=CARTESIAN_POINT ( 'NONE',  ( 4.163173891473259225, 1457.139433440971288, 199.2031176836267718 ) ) ;
#38401=CARTESIAN_POINT ( 'NONE',  ( 7.653560456693386804, 1423.197433329561591, 195.7764355311638269 ) ) ;
#38402=CARTESIAN_POINT ( 'NONE',  ( 2.366397864590000122, 1442.164712771990025, 218.0400648220289952 ) ) ;
#38406=CARTESIAN_POINT ( 'NONE',  ( 8.189759204080917954, 1487.486609484756400, 202.0226346771893589 ) ) ;
#38414=CARTESIAN_POINT ( 'NONE',  ( -11.31089902619999954, 1508.551704403789927, 217.8497850877789972 ) ) ;
#38416=CARTESIAN_POINT ( 'NONE',  ( 11.14978817083719953, 1470.287995331660113, 206.9593417752710138 ) ) ;
#38417=CARTESIAN_POINT ( 'NONE',  ( -2.850336743489999769, 1485.269293374889912, 197.9872958246989754 ) ) ;
#38421=B_SPLINE_SURFACE_WITH_KNOTS ( 'NONE', 5, 1, ( 
 ( #94247, #68533 ),
 ( #93683, #70601 ),
 ( #16962, #85290 ),
 ( #16418, #104719 ),
 ( #75813, #58465 ),
 ( #66878, #230 ) ),
 .UNSPECIFIED., .F., .F., .F.,
 ( 6, 6 ),
 ( 2, 2 ),
 ( 0.000000000000000000, 15.70013102750000122 ),
 ( 0.000000000000000000, 14.00000000000000000 ),
 .UNSPECIFIED. ) ;
#38423=CARTESIAN_POINT ( 'NONE',  ( 4.874616599078260393, 1494.129475450019982, 219.3025786937440103 ) ) ;
#38424=CARTESIAN_POINT ( 'NONE',  ( -3.071476887830000280, 1470.850261538789937, 187.3986309372990036 ) ) ;
#38425=CARTESIAN_POINT ( 'NONE',  ( -15.44282314831900038, 1415.677402202029953, 209.4843333921439807 ) ) ;
#38426=CARTESIAN_POINT ( 'NONE',  ( -9.532366409914120098, 1460.042444853610050, 210.5589214869069963 ) ) ;
#38428=DIRECTION ( 'NONE',  ( 0.000000000000000000, 1.000000000000000000, 0.000000000000000000 ) ) ;
#38436=CARTESIAN_POINT ( 'NONE',  ( 6.925143992711317864, 1424.000660984779415, 213.5535729141376748 ) ) ;
#38440=CARTESIAN_POINT ( 'NONE',  ( 8.594215834125739306, 1437.591654922809994, 210.1985574426290384 ) ) ;
#38445=CARTESIAN_POINT ( 'NONE',  ( 8.370668212402989639, 1465.542310901930023, 214.3762783931849754 ) ) ;
#38449=CARTESIAN_POINT ( 'NONE',  ( -0.3115382522500990126, 1515.152701004710025, 213.4489927825219979 ) ) ;
#38451=CARTESIAN_POINT ( 'NONE',  ( -3.523962699983150149, 1476.511731499819916, 220.0526012347959863 ) ) ;
#38459=CARTESIAN_POINT ( 'NONE',  ( 9.687580767120000047, 1493.795581537490079, 188.2203327861989806 ) ) ;
#38467=CARTESIAN_POINT ( 'NONE',  ( 0.4266141307560009643, 1456.468849147889841, 199.2577416451890144 ) ) ;
#38468=CARTESIAN_POINT ( 'NONE',  ( -3.163822641140000336, 1456.764303476689975, 218.0770700807990181 ) ) ;
#38477=CARTESIAN_POINT ( 'NONE',  ( -17.60576718599832446, 1419.790616927256906, 206.7145629358298606 ) ) ;
#38479=DIRECTION ( 'NONE',  ( -1.156023075842281927E-31, 1.000000000000000000, -1.698192320643030073E-16 ) ) ;
#38484=CARTESIAN_POINT ( 'NONE',  ( 5.530560524640000253, 1471.884652610789999, 217.6741512182190093 ) ) ;
#38490=CARTESIAN_POINT ( 'NONE',  ( 9.712381508628240567, 1434.979473192740215, 207.7851750229139896 ) ) ;
#38496=CARTESIAN_POINT ( 'NONE',  ( 11.07598440222710146, 1471.727447236650050, 211.9431201832250053 ) ) ;
#38520=CARTESIAN_POINT ( 'NONE',  ( -2.469737631213410278, 1507.227429411520006, 221.7265308815400147 ) ) ;
#38524=EDGE_CURVE ( 'NONE', #74404, #60042, #5198, .T. ) ;
#38525=EDGE_LOOP ( 'NONE', ( #874, #45389, #24841, #31326 ) ) ;
#38527=CARTESIAN_POINT ( 'NONE',  ( -4.124924170559999936, 1474.647204749290040, 198.4545245537989899 ) ) ;
#38532=CARTESIAN_POINT ( 'NONE',  ( 19.26336319460000013, 1457.977935815189767, 211.9550914373890009 ) ) ;
#38535=CARTESIAN_POINT ( 'NONE',  ( 0.2249571944082079944, 1455.813922287919922, 198.5778828182170059 ) ) ;
#38540=CARTESIAN_POINT ( 'NONE',  ( -10.01326586723869916, 1481.014341800280135, 205.7823588363200145 ) ) ;
#38541=ORIENTED_EDGE ( 'NONE', *, *, #33709, .T. ) ;
#38542=FACE_OUTER_BOUND ( 'NONE', #80996, .T. ) ;
#38544=CARTESIAN_POINT ( 'NONE',  ( -2.884827118950000102, 1442.301347507789842, 200.7110630097789965 ) ) ;
#38546=CARTESIAN_POINT ( 'NONE',  ( 12.32716906920000000, 1492.190914771690132, 209.5898718715859843 ) ) ;
#38550=CARTESIAN_POINT ( 'NONE',  ( -2.487921567437299863, 1508.551704408389924, 204.2892348438399779 ) ) ;
#38552=CARTESIAN_POINT ( 'NONE',  ( -11.69032781984710034, 1501.851939758080107, 208.8185134538140062 ) ) ;
#38558=CARTESIAN_POINT ( 'NONE',  ( -3.618491329580000304, 1476.620320023590011, 199.4078043363890060 ) ) ;
#38561=CARTESIAN_POINT ( 'NONE',  ( -18.47516819563199775, 1466.235567073390030, 200.8822723802850021 ) ) ;
#38565=CARTESIAN_POINT ( 'NONE',  ( 0.9645253690480010134, 1484.661534505690042, 201.1941721493990372 ) ) ;
#38570=CARTESIAN_POINT ( 'NONE',  ( -10.09235534473100060, 1472.733359838320212, 207.2792504626609968 ) ) ;
#38585=CARTESIAN_POINT ( 'NONE',  ( -3.430374836980000008, 1431.708658569990121, 216.7924588047190184 ) ) ;
#38586=CARTESIAN_POINT ( 'NONE',  ( -14.83290890009999963, 1420.352728576609934, 213.2060141321290132 ) ) ;
#38594=FACE_OUTER_BOUND ( 'NONE', #79429, .T. ) ;
#38599=CARTESIAN_POINT ( 'NONE',  ( 1.037960838350000081, 1497.036773399490130, 197.1546544923990041 ) ) ;
#38606=CIRCLE ( 'NONE', #108322, 0.2999999999999669598 ) ;
#38610=CARTESIAN_POINT ( 'NONE',  ( 2.418224342909999880, 1485.303415267289893, 220.3436431501990000 ) ) ;
#38611=EDGE_CURVE ( 'NONE', #61362, #21533, #4074, .T. ) ;
#38619=ORIENTED_EDGE ( 'NONE', *, *, #71701, .F. ) ;
#38621=CARTESIAN_POINT ( 'NONE',  ( 9.176823589263729986, 1451.591198660380087, 210.4727899134140046 ) ) ;
#38624=ORIENTED_EDGE ( 'NONE', *, *, #5898, .F. ) ;
#38626=CARTESIAN_POINT ( 'NONE',  ( 20.69751568230000061, 1495.539250102490087, 213.2323776579090122 ) ) ;
#38627=ADVANCED_FACE ( 'NONE', ( #95909 ), #75045, .T. ) ;
#38629=CARTESIAN_POINT ( 'NONE',  ( 3.601839739459999912, 1444.840594719589944, 200.9001243581789993 ) ) ;
#38634=CARTESIAN_POINT ( 'NONE',  ( -8.316669917960000546, 1425.055151526479904, 204.9623398779190211 ) ) ;
#38637=CARTESIAN_POINT ( 'NONE',  ( 9.010607138093890356, 1482.289598254839802, 216.7687604371109842 ) ) ;
#38639=ORIENTED_EDGE ( 'NONE', *, *, #31522, .F. ) ;
#38640=EDGE_LOOP ( 'NONE', ( #49747, #104606, #51538, #96494 ) ) ;
#38646=CARTESIAN_POINT ( 'NONE',  ( 11.21940781969999890, 1420.554733691869842, 198.7349279449990149 ) ) ;
#38648=CARTESIAN_POINT ( 'NONE',  ( 0.9567324420246190453, 1475.057211051239847, 220.5008870814820057 ) ) ;
#38649=CARTESIAN_POINT ( 'NONE',  ( -7.566646731243020341, 1494.041882933070156, 199.4137124706639952 ) ) ;
#38654=CARTESIAN_POINT ( 'NONE',  ( 12.01697534725119887, 1421.833474732869945, 207.3587116575859852 ) ) ;
#38655=CARTESIAN_POINT ( 'NONE',  ( -9.835593549186530282, 1439.958152553570017, 207.2549332851669988 ) ) ;
#38664=CARTESIAN_POINT ( 'NONE',  ( -14.87918216340000122, 1415.865102033119911, 212.9009079005989804 ) ) ;
#38665=CARTESIAN_POINT ( 'NONE',  ( -9.183711187100000117, 1463.569275765890097, 202.8257126108990178 ) ) ;
#38666=ORIENTED_EDGE ( 'NONE', *, *, #74806, .F. ) ;
#38667=CARTESIAN_POINT ( 'NONE',  ( 4.110418388699999426, 1430.160170311989987, 217.2245068817190088 ) ) ;
#38670=CARTESIAN_POINT ( 'NONE',  ( 0.2961798576886189305, 1430.492998182000065, 199.6993750702310138 ) ) ;
#38672=DIRECTION ( 'NONE',  ( 0.9996573249755569268, 0.02617694830788839730, 1.176140869340470334E-16 ) ) ;
#38673=CARTESIAN_POINT ( 'NONE',  ( 4.830146310314740177, 1458.041703014179802, 200.3202911288479982 ) ) ;
#38689=CARTESIAN_POINT ( 'NONE',  ( 8.637121918412720589, 1428.330124385589897, 213.2627993150280190 ) ) ;
#38691=CARTESIAN_POINT ( 'NONE',  ( 0.9281737935813634266, 1484.584957263379692, 198.4507462532201032 ) ) ;
#38694=CARTESIAN_POINT ( 'NONE',  ( 4.781276783620000081, 1452.020048942890071, 190.5513815401990030 ) ) ;
#38696=CARTESIAN_POINT ( 'NONE',  ( 0.9988581265890018601, 1485.909730274089952, 197.9875094714990098 ) ) ;
#38697=CARTESIAN_POINT ( 'NONE',  ( 4.229221492309999775, 1477.633992664089874, 199.3656528811089856 ) ) ;
#38699=CARTESIAN_POINT ( 'NONE',  ( -11.81485801620000053, 1490.683346627590026, 208.7791644193250136 ) ) ;
#38700=CARTESIAN_POINT ( 'NONE',  ( 1.543581094750000160, 1464.188004283289956, 202.2270558697589991 ) ) ;
#38716=CARTESIAN_POINT ( 'NONE',  ( -10.81752260999999926, 1499.346262163689971, 213.0012804442189918 ) ) ;
#38718=CARTESIAN_POINT ( 'NONE',  ( -2.472546475879999761, 1422.360492461289823, 192.6709265613989999 ) ) ;
#38722=CARTESIAN_POINT ( 'NONE',  ( -16.53936930417849993, 1465.413251900429941, 220.7146308235560070 ) ) ;
#38735=CARTESIAN_POINT ( 'NONE',  ( 8821.610583169964229, 5182.767774292105059, -2585.458545683866305 ) ) ;
#38760=EDGE_LOOP ( 'NONE', ( #12939, #52816, #97841, #91776 ) ) ;
#38761=VERTEX_POINT ( 'NONE', #65491 ) ;
#38765=CARTESIAN_POINT ( 'NONE',  ( -16.87183719374050028, 1508.551704427820141, 210.1079651444619856 ) ) ;
#38766=B_SPLINE_CURVE_WITH_KNOTS ( 'NONE', 5,
 ( #65167, #14739, #47256, #107149, #73013, #99839 ),
 .UNSPECIFIED., .F., .F.,
 ( 6, 6 ),
 ( -1.999999800030170194, 0.000000000000000000 ),
 .UNSPECIFIED. ) ;
#38780=EDGE_LOOP ( 'NONE', ( #35318, #96769, #16546, #10098 ) ) ;
#38782=CARTESIAN_POINT ( 'NONE',  ( 8.427480802527020032, 1428.383621637630085, 213.4646598519510121 ) ) ;
#38796=CARTESIAN_POINT ( 'NONE',  ( -10.40779544903779197, 1480.508706840727882, 207.4968371392113795 ) ) ;
#38799=CARTESIAN_POINT ( 'NONE',  ( 2.329939114882360052, 1515.551844914359890, 213.1055637607790061 ) ) ;
#38800=EDGE_CURVE ( 'NONE', #74706, #109446, #38606, .T. ) ;
#38807=CARTESIAN_POINT ( 'NONE',  ( -14.53748718939999840, 1415.677402282210096, 205.0892928880890054 ) ) ;
#38809=CARTESIAN_POINT ( 'NONE',  ( -15.06652045519958349, 1415.677402202029953, 210.6308072257622541 ) ) ;
#38818=CARTESIAN_POINT ( 'NONE',  ( 1.842963640640000067, 1515.372048646890107, 213.3835825195990026 ) ) ;
#38819=CARTESIAN_POINT ( 'NONE',  ( 10.79528402730720060, 1489.628194868570063, 207.4012257063180016 ) ) ;
#38821=CARTESIAN_POINT ( 'NONE',  ( 1.356372325302582782, 1463.975736616651602, 199.4023338319472884 ) ) ;
#38823=CARTESIAN_POINT ( 'NONE',  ( -4.817207246935718779, 1440.943601040120939, 201.7191942600521202 ) ) ;
#38828=CARTESIAN_POINT ( 'NONE',  ( -4.175269160410000069, 1515.456655180189955, 210.6055574401990214 ) ) ;
#38831=DIRECTION ( 'NONE',  ( -1.000000000000000000, 0.000000000000000000, 0.000000000000000000 ) ) ;
#38835=CARTESIAN_POINT ( 'NONE',  ( -9.526128307108560733, 1440.436522615020067, 205.9995050262249947 ) ) ;
#38838=CARTESIAN_POINT ( 'NONE',  ( -4.994663984927831812, 1391.700789716822328, 214.7093307040285026 ) ) ;
#38845=CARTESIAN_POINT ( 'NONE',  ( -2.910436537626309939, 1508.551704408389924, 204.1692697258259841 ) ) ;
#38847=ORIENTED_EDGE ( 'NONE', *, *, #96968, .T. ) ;
#38850=DIRECTION ( 'NONE',  ( 0.4229618813980365877, 0.9061474752402244315, 4.354426617128452806E-10 ) ) ;
#38854=CARTESIAN_POINT ( 'NONE',  ( -4.360511200180000380, 1454.978814463989920, 200.7714289439389859 ) ) ;
#38856=CARTESIAN_POINT ( 'NONE',  ( 12.68801083313210043, 1500.413651417279880, 208.6561539661539939 ) ) ;
#38858=CARTESIAN_POINT ( 'NONE',  ( 9.738317565070000015, 1493.400072498489862, 188.2659980885989910 ) ) ;
#38875=CARTESIAN_POINT ( 'NONE',  ( -2.384849065066879881, 1464.024019744329962, 199.4598481641620253 ) ) ;
#38892=CARTESIAN_POINT ( 'NONE',  ( -17.18922504907660098, 1508.551704422510056, 212.4816474524029957 ) ) ;
#38895=ADVANCED_FACE ( 'NONE', ( #73327 ), #49113, .T. ) ;
#38899=CARTESIAN_POINT ( 'NONE',  ( -8.509555873503130030, 1452.079233855630036, 205.3893997472640081 ) ) ;
#38904=VERTEX_POINT ( 'NONE', #2096 ) ;
#38915=CARTESIAN_POINT ( 'NONE',  ( 12.72813482502530036, 1426.626821931249879, 196.2928140043740086 ) ) ;
#38929=CARTESIAN_POINT ( 'NONE',  ( 11.54684311930000007, 1425.837099041209967, 203.6587523742389862 ) ) ;
#38934=CARTESIAN_POINT ( 'NONE',  ( 11.19499699576850027, 1470.359902562939851, 207.1673228584000128 ) ) ;
#38943=CARTESIAN_POINT ( 'NONE',  ( 2.663026065689999999, 1442.012083350790135, 217.9487819464190181 ) ) ;
#38953=CARTESIAN_POINT ( 'NONE',  ( -9.946114271644979965, 1472.218658670100012, 211.2590325883199966 ) ) ;
#38956=CARTESIAN_POINT ( 'NONE',  ( -14.36727199889999973, 1508.541240743890057, 215.8627312463090107 ) ) ;
#38967=CARTESIAN_POINT ( 'NONE',  ( -14.61097672478990006, 1415.677402205059934, 205.8812875983110189 ) ) ;
#38970=CARTESIAN_POINT ( 'NONE',  ( 6.938871378149999991, 1427.890279811890196, 213.8982594654290210 ) ) ;
#38971=CARTESIAN_POINT ( 'NONE',  ( 19.35628570429999940, 1496.398810548190113, 218.7515486585290034 ) ) ;
#38989=CARTESIAN_POINT ( 'NONE',  ( 9.554826419470950682, 1464.136006249749926, 211.3862083144839801 ) ) ;
#38990=CARTESIAN_POINT ( 'NONE',  ( 0.6516344981559789584, 1515.134688985610182, 213.4494644436790054 ) ) ;
#38997=ORIENTED_EDGE ( 'NONE', *, *, #44750, .F. ) ;
#39000=CARTESIAN_POINT ( 'NONE',  ( -18.74924298070000006, 1506.108474969089912, 222.6729604708989996 ) ) ;
#39004=CARTESIAN_POINT ( 'NONE',  ( -11.52816659857622561, 1414.661898229710005, 206.9304423160286888 ) ) ;
#39007=DIRECTION ( 'NONE',  ( -1.000000000000000000, 0.000000000000000000, 0.000000000000000000 ) ) ;
#39008=CARTESIAN_POINT ( 'NONE',  ( -3.345499056600000021, 1457.924539801389983, 218.8450915141490043 ) ) ;
#39014=EDGE_LOOP ( 'NONE', ( #81117, #59701, #35013, #70948 ) ) ;
#39035=CARTESIAN_POINT ( 'NONE',  ( 1.476582328747939821, 1467.059268612629921, 220.0911334793899812 ) ) ;
#39039=CARTESIAN_POINT ( 'NONE',  ( 6.006124716077446024, 1460.017935509939662, 201.5831662601001995 ) ) ;
#39040=CARTESIAN_POINT ( 'NONE',  ( 9.906408661899998691, 1453.734930172990062, 213.0153772767789917 ) ) ;
#39041=CARTESIAN_POINT ( 'NONE',  ( 4.124003890242169845, 1440.791985383939846, 218.1323065870639937 ) ) ;
#39044=VERTEX_POINT ( 'NONE', #70410 ) ;
#39061=EDGE_CURVE ( 'NONE', #103217, #108761, #61354, .T. ) ;
#39077=CARTESIAN_POINT ( 'NONE',  ( -1.165022167831349931, 1455.263797152349980, 198.6710384306789763 ) ) ;
#39080=CARTESIAN_POINT ( 'NONE',  ( -10.07722745004169873, 1471.911775314289798, 210.4363667124119672 ) ) ;
#39082=VERTEX_POINT ( 'NONE', #47391 ) ;
#39083=ORIENTED_EDGE ( 'NONE', *, *, #56184, .F. ) ;
#39084=CARTESIAN_POINT ( 'NONE',  ( 10.55265553690759894, 1480.891686322609985, 208.8870839355319902 ) ) ;
#39086=CARTESIAN_POINT ( 'NONE',  ( -4.553268120680000308, 1442.065311926689901, 201.3752710187589798 ) ) ;
#39092=ADVANCED_FACE ( 'NONE', ( #4815 ), #91088, .T. ) ;
#39096=CARTESIAN_POINT ( 'NONE',  ( -11.44991336099019819, 1501.249626596179951, 208.6595951068130148 ) ) ;
#39104=CARTESIAN_POINT ( 'NONE',  ( 3.219327822800559957, 1508.551704408389924, 204.2443104558009850 ) ) ;
#39107=CARTESIAN_POINT ( 'NONE',  ( -18.32378034181390092, 1464.077664432049914, 217.4721294711199846 ) ) ;
#39111=FACE_OUTER_BOUND ( 'NONE', #87954, .T. ) ;
#39131=CARTESIAN_POINT ( 'NONE',  ( -15.86088303929999910, 1419.980596273840092, 210.7344905958990182 ) ) ;
#39136=CARTESIAN_POINT ( 'NONE',  ( 13.55421397129999939, 1497.816254223590022, 226.3870761728989862 ) ) ;
#39141=DIRECTION ( 'NONE',  ( 0.000000000000000000, 0.000000000000000000, 1.000000000000000000 ) ) ;
#39147=CARTESIAN_POINT ( 'NONE',  ( 7.085131439273410159, 1424.907808281010148, 213.0594611446600197 ) ) ;
#39153=CARTESIAN_POINT ( 'NONE',  ( -3.709420335830000415, 1414.325355622289862, 206.4743713944289709 ) ) ;
#39154=CARTESIAN_POINT ( 'NONE',  ( -11.97564940980980097, 1491.173717386239787, 206.6759772995580136 ) ) ;
#39158=CARTESIAN_POINT ( 'NONE',  ( -1.840591215909999967, 1487.831606858690066, 219.8181691253990095 ) ) ;
#39166=ORIENTED_EDGE ( 'NONE', *, *, #96051, .T. ) ;
#39175=CARTESIAN_POINT ( 'NONE',  ( 2.531901238200000126, 1444.224916984790070, 200.5256934874690273 ) ) ;
#39183=CARTESIAN_POINT ( 'NONE',  ( 10.23003872437689843, 1481.533373258429947, 215.0139943380300167 ) ) ;
#39185=EDGE_LOOP ( 'NONE', ( #78034, #44025, #52083, #107847, #76796 ) ) ;
#39192=CARTESIAN_POINT ( 'NONE',  ( 11.29246402500000102, 1420.389623373509721, 198.6444918639989794 ) ) ;
#39199=CARTESIAN_POINT ( 'NONE',  ( 10.74318624240480169, 1423.607808323160043, 206.7556458220460058 ) ) ;
#39206=CARTESIAN_POINT ( 'NONE',  ( -16.85557438000711272, 1417.264140369140478, 207.1097720217920255 ) ) ;
#39210=CARTESIAN_POINT ( 'NONE',  ( 9.058157503864009641, 1423.689293625850041, 210.6374908749079964 ) ) ;
#39211=CARTESIAN_POINT ( 'NONE',  ( -16.14864212301420210, 1419.744746607639854, 210.0472711449799874 ) ) ;
#39213=CARTESIAN_POINT ( 'NONE',  ( 4.329898783340000001, 1430.328825655489936, 217.5774781053490017 ) ) ;
#39216=ADVANCED_FACE ( 'NONE', ( #40038, #41139 ), #42251, .T. ) ;
#39234=CARTESIAN_POINT ( 'NONE',  ( -0.7050289745649990225, 1515.139588934790027, 204.7943557892189972 ) ) ;
#39235=CARTESIAN_POINT ( 'NONE',  ( -14.20525283303160080, 1416.384016890880048, 203.1489016136929706 ) ) ;
#39238=CARTESIAN_POINT ( 'NONE',  ( 18.38166058516359769, 1428.164368163260178, 201.4944004331299823 ) ) ;
#39242=CARTESIAN_POINT ( 'NONE',  ( 9.070710170037548536, 1428.247707153859892, 212.8796129129519841 ) ) ;
#39248=CARTESIAN_POINT ( 'NONE',  ( -2.847678236428970333, 1430.845636561999981, 201.2564352187889938 ) ) ;
#39253=CARTESIAN_POINT ( 'NONE',  ( -12.07906408490000061, 1491.053577648989858, 206.9546736298989913 ) ) ;
#39263=CARTESIAN_POINT ( 'NONE',  ( -12.09091630672140028, 1491.024750413429956, 207.0451805009280122 ) ) ;
#39264=CARTESIAN_POINT ( 'NONE',  ( -4.174206985259830027, 1508.551704408389924, 204.7881409777949955 ) ) ;
#39273=CARTESIAN_POINT ( 'NONE',  ( 9.623281588457949454, 1470.012648596069994, 212.1148972040010108 ) ) ;
#39277=CARTESIAN_POINT ( 'NONE',  ( -2.265100829110000102, 1421.884435632049872, 193.4623859336989824 ) ) ;
#39281=CARTESIAN_POINT ( 'NONE',  ( -18.30458809710689749, 1465.267267787470018, 217.6413456689680004 ) ) ;
#39285=CARTESIAN_POINT ( 'NONE',  ( 19.60792669039999936, 1475.100271358290229, 204.3343059087790152 ) ) ;
#39288=EDGE_CURVE ( 'NONE', #18748, #97154, #90651, .T. ) ;
#39289=CARTESIAN_POINT ( 'NONE',  ( -14.55659802589999963, 1503.856184377289992, 208.7749621606049857 ) ) ;
#39295=CARTESIAN_POINT ( 'NONE',  ( -8765.422060425717063, 5182.767774292095964, 3175.242030490383513 ) ) ;
#39302=CARTESIAN_POINT ( 'NONE',  ( -3.558358604862239982, 1455.955982659530036, 200.3550966546550001 ) ) ;
#39312=CARTESIAN_POINT ( 'NONE',  ( 10.43358895521959973, 1481.587437876299873, 210.8843897139930164 ) ) ;
#39325=CARTESIAN_POINT ( 'NONE',  ( -20.36287103150000277, 1507.711394158289977, 209.4617748114379765 ) ) ;
#39334=ORIENTED_EDGE ( 'NONE', *, *, #29653, .F. ) ;
#39343=CARTESIAN_POINT ( 'NONE',  ( -18.05280916457315143, 1508.456971748121987, 211.8086596262961621 ) ) ;
#39345=CARTESIAN_POINT ( 'NONE',  ( -7.465741425504200279, 1435.823992893209834, 215.3776685733120075 ) ) ;
#39352=CARTESIAN_POINT ( 'NONE',  ( 6.555273148870000455, 1470.255836705890033, 211.2211195251889819 ) ) ;
#39353=AXIS2_PLACEMENT_3D ( 'NONE', #33607, #84577, #92416 ) ;
#39357=CARTESIAN_POINT ( 'NONE',  ( -10.33191382005590953, 1480.649815741992597, 207.0399858577212910 ) ) ;
#39358=CARTESIAN_POINT ( 'NONE',  ( 3.163495553606223254, 1467.481610648900414, 218.5739468055329837 ) ) ;
#39361=CARTESIAN_POINT ( 'NONE',  ( -3.631597801648350110, 1483.402419362059845, 199.0973728678349914 ) ) ;
#39362=CARTESIAN_POINT ( 'NONE',  ( -11.25664976887165203, 1508.421381615256678, 207.6010284851684276 ) ) ;
#39366=CARTESIAN_POINT ( 'NONE',  ( 2.911802205209999883, 1507.562757914290160, 220.4805861716990023 ) ) ;
#39368=CARTESIAN_POINT ( 'NONE',  ( -15.75672504909999816, 1415.912232267690115, 208.9316401283900291 ) ) ;
#39369=CARTESIAN_POINT ( 'NONE',  ( -6.711227830452440202, 1442.278139609789832, 201.5834457825660024 ) ) ;
#39371=CARTESIAN_POINT ( 'NONE',  ( 8.725351515859999907, 1420.892103511989944, 196.4178243839989761 ) ) ;
#39372=CARTESIAN_POINT ( 'NONE',  ( -9.522388363570000180, 1439.330054399390065, 208.4250942545799887 ) ) ;
#39383=CARTESIAN_POINT ( 'NONE',  ( 0.1095232733706122119, 1463.638598533493223, 199.3170435800446398 ) ) ;
#39384=CARTESIAN_POINT ( 'NONE',  ( 9.545351305817721510, 1500.533481294277635, 228.7109972438295813 ) ) ;
#39392=CARTESIAN_POINT ( 'NONE',  ( -4.045201229639999951, 1515.528102034789981, 210.6102411367990328 ) ) ;
#39395=CARTESIAN_POINT ( 'NONE',  ( -1.073240929390329958E-18, 1414.661898229710005, 209.1218459616989946 ) ) ;
#39403=CIRCLE ( 'NONE', #82324, 15.40132948099999943 ) ;
#39415=CARTESIAN_POINT ( 'NONE',  ( -19.86464710129909861, 1441.435714616360201, 212.6459466280339825 ) ) ;
#39416=CARTESIAN_POINT ( 'NONE',  ( -15.92986207429999901, 1416.139014782290133, 209.7537124246929920 ) ) ;
#39419=CARTESIAN_POINT ( 'NONE',  ( -8.045651973969999204, 1451.834176107089888, 203.9611725415890078 ) ) ;
#39422=CARTESIAN_POINT ( 'NONE',  ( 7.213731313499999409, 1426.540065858099979, 212.9766447227389961 ) ) ;
#39426=CARTESIAN_POINT ( 'NONE',  ( -3.220674668504990290, 1433.265634988960073, 218.1214075394389909 ) ) ;
#39435=B_SPLINE_CURVE_WITH_KNOTS ( 'NONE', 5,
 ( #35491, #36061, #78606, #61291, #104354, #62959 ),
 .UNSPECIFIED., .F., .F.,
 ( 6, 6 ),
 ( -2.000000000000000000, -3.509303492243986966E-08 ),
 .UNSPECIFIED. ) ;
#39439=CARTESIAN_POINT ( 'NONE',  ( 2.329939107268570009, 1515.551844914359890, 205.1381281622049926 ) ) ;
#39440=CARTESIAN_POINT ( 'NONE',  ( 3.279726280340000244, 1445.963863862890094, 200.3213861966889908 ) ) ;
#39457=CARTESIAN_POINT ( 'NONE',  ( 10.96561470309999820, 1490.902452854290004, 209.8193876016359809 ) ) ;
#39463=B_SPLINE_CURVE_WITH_KNOTS ( 'NONE', 3,
 ( #102529, #50514, #101420, #110399, #75710, #33679, #40988, #42103, #68427, #67871 ),
 .UNSPECIFIED., .F., .F.,
 ( 4, 2, 2, 2, 4 ),
 ( 0.000000000000000000, 0.2500000000000000000, 0.5000000000000000000, 0.7500000000000000000, 1.000000000000000000 ),
 .UNSPECIFIED. ) ;
#39465=CARTESIAN_POINT ( 'NONE',  ( -11.41188801179999857, 1502.809396336989948, 207.5688504535389995 ) ) ;
#39473=CARTESIAN_POINT ( 'NONE',  ( -8.599604059879169426, 1451.952372034600103, 205.6084899554880110 ) ) ;
#39489=CARTESIAN_POINT ( 'NONE',  ( 17.25714853236529933, 1428.491813688779757, 203.4901169056299750 ) ) ;
#39502=CARTESIAN_POINT ( 'NONE',  ( 1.451113133880000072, 1499.806239416590188, 230.3830668976989955 ) ) ;
#39503=CARTESIAN_POINT ( 'NONE',  ( 12.91459300150000011, 1421.176040162410118, 204.7063101998089962 ) ) ;
#39508=CARTESIAN_POINT ( 'NONE',  ( 7.294923546887015497, 1458.268531074105567, 201.0098627031420904 ) ) ;
#39517=CARTESIAN_POINT ( 'NONE',  ( 8.950879146035706668, 1424.989091137386595, 195.6957624501638406 ) ) ;
#39518=CARTESIAN_POINT ( 'NONE',  ( 1.480262881429999844, 1443.955256524790002, 217.9442098410289930 ) ) ;
#39521=CARTESIAN_POINT ( 'NONE',  ( 19.52205342210000083, 1473.076230373790168, 204.3554439105789982 ) ) ;
#39528=EDGE_LOOP ( 'NONE', ( #26588, #55188, #56508, #31154 ) ) ;
#39530=CARTESIAN_POINT ( 'NONE',  ( -16.59176436839999980, 1508.492920114390017, 213.6703949458789964 ) ) ;
#39540=CARTESIAN_POINT ( 'NONE',  ( -14.82123553143790140, 1415.677402202029953, 206.6677478258380063 ) ) ;
#39542=CARTESIAN_POINT ( 'NONE',  ( -9.643323296948050682, 1460.351442354390201, 209.5911327240870037 ) ) ;
#39543=CARTESIAN_POINT ( 'NONE',  ( 6.687468864090000409, 1429.390509083689949, 215.9663958518090112 ) ) ;
#39545=ORIENTED_EDGE ( 'NONE', *, *, #78085, .F. ) ;
#39548=EDGE_CURVE ( 'NONE', #77826, #32575, #26395, .T. ) ;
#39551=CARTESIAN_POINT ( 'NONE',  ( -12.78592627679999971, 1502.554352260989845, 209.5469753058839899 ) ) ;
#39553=CARTESIAN_POINT ( 'NONE',  ( 1.991751356299999776, 1454.627457338589920, 218.3211767913890071 ) ) ;
#39555=CARTESIAN_POINT ( 'NONE',  ( 9.339431960871671379, 1436.245858615840007, 210.2893693010520053 ) ) ;
#39557=CARTESIAN_POINT ( 'NONE',  ( -3.116134665872564380, 1509.034509761476556, 213.6092032002669328 ) ) ;
#39561=CARTESIAN_POINT ( 'NONE',  ( -1.273031542849370146, 1515.087982642930001, 213.4506874923570194 ) ) ;
#39563=CARTESIAN_POINT ( 'NONE',  ( -5.619035311959510004, 1477.367051216990149, 219.2138315790730019 ) ) ;
#39571=CARTESIAN_POINT ( 'NONE',  ( 19.12714126967820150, 1496.834737738279955, 222.0421931355600123 ) ) ;
#39578=CARTESIAN_POINT ( 'NONE',  ( 4.326999254989379651, 1515.158336317459998, 209.1856212445070184 ) ) ;
#39580=CARTESIAN_POINT ( 'NONE',  ( 10.00058476560569964, 1468.846443592369724, 208.4342511431520109 ) ) ;
#39581=CARTESIAN_POINT ( 'NONE',  ( -5.024929782580000115, 1457.083462483489939, 217.2019913456090308 ) ) ;
#39587=ORIENTED_EDGE ( 'NONE', *, *, #81068, .F. ) ;
#39590=CARTESIAN_POINT ( 'NONE',  ( -8.993785038736740844, 1447.472150739280096, 212.1283412365259835 ) ) ;
#39608=VERTEX_POINT ( 'NONE', #100894 ) ;
#39625=CARTESIAN_POINT ( 'NONE',  ( -10.19411843490000003, 1472.876058185389866, 208.6040583671850186 ) ) ;
#39631=LINE ( 'NONE', #65403, #86050 ) ;
#39641=CARTESIAN_POINT ( 'NONE',  ( -17.48275921970000013, 1417.637981030829906, 206.6019964927289720 ) ) ;
#39646=CARTESIAN_POINT ( 'NONE',  ( -2.702426668010000199, 1474.936083011690016, 219.0658163223389749 ) ) ;
#39650=CARTESIAN_POINT ( 'NONE',  ( -2.139976072801630380, 1454.838776466839818, 198.8441892363819932 ) ) ;
#39654=CARTESIAN_POINT ( 'NONE',  ( -7.980162481601299262, 1424.786834349992887, 210.5240428619318322 ) ) ;
#39657=B_SPLINE_CURVE_WITH_KNOTS ( 'NONE', 5,
 ( #91344, #48812, #83477, #5695, #82935, #15698, #65609, #99167, #49350 ),
 .UNSPECIFIED., .F., .F.,
 ( 6, 3, 6 ),
 ( 0.000000000000000000, 0.4798557570286712815, 1.000000000000000000 ),
 .UNSPECIFIED. ) ;
#39660=CARTESIAN_POINT ( 'NONE',  ( 1.248319867352440049, 1432.832940376729994, 200.7627304351539976 ) ) ;
#39663=CARTESIAN_POINT ( 'NONE',  ( 11.35500377106789927, 1502.899977923620099, 211.0831124703279897 ) ) ;
#39666=CARTESIAN_POINT ( 'NONE',  ( -1.398163373145720145, 1508.551704408389924, 220.0821830793859704 ) ) ;
#39670=CARTESIAN_POINT ( 'NONE',  ( -11.55818388030770016, 1501.591350514780061, 208.7507439016920046 ) ) ;
#39677=CARTESIAN_POINT ( 'NONE',  ( 3.384752633832900148, 1508.551704408389924, 204.2997876064260083 ) ) ;
#39680=CARTESIAN_POINT ( 'NONE',  ( 10.37957671256920023, 1453.090566707049902, 190.0119522185410119 ) ) ;
#39683=CARTESIAN_POINT ( 'NONE',  ( -3.368571795366160249, 1515.551842517600107, 205.3433056528259897 ) ) ;
#39700=CARTESIAN_POINT ( 'NONE',  ( 12.82316716488450048, 1420.870306943950027, 202.5884333197170122 ) ) ;
#39702=CARTESIAN_POINT ( 'NONE',  ( -14.76729556169999924, 1420.459770328189734, 213.1799085011889758 ) ) ;
#39709=B_SPLINE_CURVE_WITH_KNOTS ( 'NONE', 3,
 ( #43533, #35669, #96130, #44084, #70413, #26710, #96697, #11034, #53044, #36781, #18848, #10471, #9370, #44644, #79896, #60336, #103405, #60904, #45201, #78224, #70973, #95579 ),
 .UNSPECIFIED., .F., .F.,
 ( 4, 3, 3, 3, 3, 3, 3, 4 ),
 ( -7.319250909075099898, -7.125925300183699740, -6.024000583945539944, -5.159116688310800392, -5.076639483430359867, -4.351712499397559775, -3.635277218665780019, -2.998981459959999540 ),
 .UNSPECIFIED. ) ;
#39712=CARTESIAN_POINT ( 'NONE',  ( -9.044119212145819375, 1448.868168609049917, 210.5545963948329984 ) ) ;
#39717=CARTESIAN_POINT ( 'NONE',  ( 7.301066274272970169, 1425.020808777460161, 212.6544105784089993 ) ) ;
#39725=CARTESIAN_POINT ( 'NONE',  ( -4.633397098031163175, 1377.913060387290216, 214.0697612255490014 ) ) ;
#39747=CARTESIAN_POINT ( 'NONE',  ( -7.604266383829999754, 1426.735969319010110, 206.0920978162889980 ) ) ;
#39750=CARTESIAN_POINT ( 'NONE',  ( 11.15342146135749957, 1480.750365135299944, 212.9722137386380041 ) ) ;
#39756=CARTESIAN_POINT ( 'NONE',  ( -10.70297910787769879, 1480.941407630280082, 209.2201545748799845 ) ) ;
#39762=CARTESIAN_POINT ( 'NONE',  ( 9.570877374229999290, 1420.722443590560033, 197.0571623609990297 ) ) ;
#39763=CARTESIAN_POINT ( 'NONE',  ( -2.039945179225050254, 1475.967660246570176, 220.3917608611429841 ) ) ;
#39765=CARTESIAN_POINT ( 'NONE',  ( -4.873188877689999643, 1496.854351603390114, 198.9825648115990191 ) ) ;
#39773=CARTESIAN_POINT ( 'NONE',  ( 6.454036439679999404, 1470.375359702289870, 211.5526527559590022 ) ) ;
#39780=CARTESIAN_POINT ( 'NONE',  ( 11.07287788601909995, 1424.672578760980059, 203.0822791269380332 ) ) ;
#39782=CARTESIAN_POINT ( 'NONE',  ( 2.529870311359999846, 1429.478213350389979, 217.0523039979090072 ) ) ;
#39784=CARTESIAN_POINT ( 'NONE',  ( 1.110223024629999949E-15, 1377.913060387289988, 209.1218459616989946 ) ) ;
#39788=ADVANCED_FACE ( 'NONE', ( #43232 ), #40138, .T. ) ;
#39789=CARTESIAN_POINT ( 'NONE',  ( 8.559858904628349308, 1437.030483964089854, 207.9845584131589931 ) ) ;
#39797=CARTESIAN_POINT ( 'NONE',  ( -20.06562366400000030, 1485.934169092390221, 214.0282076738189971 ) ) ;
#39800=CARTESIAN_POINT ( 'NONE',  ( 1.842962231260000028, 1515.219201591190085, 204.7964405199890336 ) ) ;
#39801=CARTESIAN_POINT ( 'NONE',  ( -14.45615645293159979, 1417.226029900110007, 203.2557612791789836 ) ) ;
#39823=CARTESIAN_POINT ( 'NONE',  ( -12.25193733536140073, 1490.464065053120066, 208.8495834660220112 ) ) ;
#39824=CARTESIAN_POINT ( 'NONE',  ( -4.239735416363259901, 1508.551704408389924, 204.8502244740350022 ) ) ;
#39830=CARTESIAN_POINT ( 'NONE',  ( 11.39055221683119967, 1471.191658448979979, 209.8979774520730075 ) ) ;
#39831=CARTESIAN_POINT ( 'NONE',  ( 18.07341264884579957, 1430.225308298370010, 211.4628600911939884 ) ) ;
#39837=CARTESIAN_POINT ( 'NONE',  ( -20.45989939420000425, 1467.733552288090095, 211.3272550349789753 ) ) ;
#39855=CARTESIAN_POINT ( 'NONE',  ( -17.43675326300159867, 1417.688629928019964, 206.2161178420579972 ) ) ;
#39857=CARTESIAN_POINT ( 'NONE',  ( 3.262212153180289675, 1484.802729046160039, 220.5136830109310040 ) ) ;
#39858=CARTESIAN_POINT ( 'NONE',  ( 12.09108845230000107, 1500.238058980090045, 207.1892423451589877 ) ) ;
#39864=CARTESIAN_POINT ( 'NONE',  ( 10.80507665935240169, 1480.918775577479892, 212.7532992060299932 ) ) ;
#39869=CARTESIAN_POINT ( 'NONE',  ( -2.775555821850000271, 1468.867611631090085, 187.4507004057990116 ) ) ;
#39872=VERTEX_POINT ( 'NONE', #47088 ) ;
#39877=CARTESIAN_POINT ( 'NONE',  ( -2.330134126681665752, 1515.193466806617153, 213.4479252923928243 ) ) ;
#39881=CARTESIAN_POINT ( 'NONE',  ( -1.423096497750000022, 1465.102360927890004, 198.1952834721990087 ) ) ;
#39886=EDGE_LOOP ( 'NONE', ( #24664, #60739, #51287, #48651 ) ) ;
#39889=EDGE_LOOP ( 'NONE', ( #6138, #65966, #14752, #34729, #63140 ) ) ;
#39894=CARTESIAN_POINT ( 'NONE',  ( 8.186040751612090105, 1428.551989710240150, 213.9112982126329996 ) ) ;
#39902=EDGE_CURVE ( 'NONE', #44275, #78311, #28624, .T. ) ;
#39909=CARTESIAN_POINT ( 'NONE',  ( -10.22078022364619976, 1448.827725899079724, 207.2905427559460065 ) ) ;
#39914=( BOUNDED_CURVE ( )  B_SPLINE_CURVE ( 3, ( #49629, #41758, #33902, #8146 ),
 .UNSPECIFIED., .F., .F. ) 
 B_SPLINE_CURVE_WITH_KNOTS ( ( 4, 4 ),
 ( 1.006680279111034082, 2.134912272047150061 ),
 .UNSPECIFIED. ) 
 CURVE ( )  GEOMETRIC_REPRESENTATION_ITEM ( )  RATIONAL_B_SPLINE_CURVE ( ( 1.000000000000000000, 0.8967077198847258623, 0.8967077198847258623, 1.000000000000000000 ) ) 
 REPRESENTATION_ITEM ( '' )  );
#39921=CARTESIAN_POINT ( 'NONE',  ( -1.315891021949999962, 1430.627222964690191, 214.6815279436889909 ) ) ;
#39924=CARTESIAN_POINT ( 'NONE',  ( 9.197260543180000525, 1420.703589484819986, 196.7538032495989739 ) ) ;
#39925=ADVANCED_FACE ( 'NONE', ( #64451 ), #23136, .F. ) ;
#39928=CARTESIAN_POINT ( 'NONE',  ( -20.24460045326980051, 1505.070898157219972, 209.5321939871419943 ) ) ;
#39939=CARTESIAN_POINT ( 'NONE',  ( -10.32330663897819889, 1447.671776642609984, 209.9210912389999919 ) ) ;
#39944=CARTESIAN_POINT ( 'NONE',  ( -10.21665424470000083, 1499.224423270490206, 214.5746271585690010 ) ) ;
#39955=CARTESIAN_POINT ( 'NONE',  ( 12.14869142895439857, 1491.529512745250031, 207.2247900540259877 ) ) ;
#39960=CARTESIAN_POINT ( 'NONE',  ( 10.92186379062459878, 1478.901561184230104, 206.2239204151590286 ) ) ;
#39963=CARTESIAN_POINT ( 'NONE',  ( -3.317807041231336485E-31, 1414.677402202029953, 209.1218459616989946 ) ) ;
#39964=CARTESIAN_POINT ( 'NONE',  ( -19.04700360162490114, 1444.155872992060040, 199.5980005314840184 ) ) ;
#39969=CARTESIAN_POINT ( 'NONE',  ( -5.735785620560000631, 1454.599929374689964, 201.6482604689090010 ) ) ;
#39971=EDGE_CURVE ( 'NONE', #50471, #101391, #85082, .T. ) ;
#39973=CARTESIAN_POINT ( 'NONE',  ( 7.143956740810000205, 1426.607338919389804, 213.1092222816089929 ) ) ;
#39988=FACE_OUTER_BOUND ( 'NONE', #14912, .T. ) ;
#39990=ADVANCED_FACE ( 'NONE', ( #109733 ), #38292, .T. ) ;
#39992=CARTESIAN_POINT ( 'NONE',  ( -4.458786532230819333, 1463.138397474430121, 200.4163687677220196 ) ) ;
#40003=CARTESIAN_POINT ( 'NONE',  ( -6.466996272939999457, 1422.019461440550231, 192.0563668886989888 ) ) ;
#40008=B_SPLINE_SURFACE_WITH_KNOTS ( 'NONE', 5, 5, ( 
 ( #106973, #37575, #12360, #54408, #72301, #71212 ),
 ( #72840, #30260, #64453, #98567, #21836, #106432 ),
 ( #11824, #105334, #80126, #28625, #29716, #64991 ),
 ( #30814, #98015, #63900, #5064, #47632, #45995 ),
 ( #21287, #90161, #81761, #62827, #71776, #39211 ),
 ( #73388, #107524, #105895, #99109, #3445, #56586 ) ),
 .UNSPECIFIED., .F., .F., .F.,
 ( 6, 6 ),
 ( 6, 6 ),
 ( 27.35438305753609711, 59.36386366779180435 ),
 ( -0.0006425587617316530107, 0.5000000000000000000 ),
 .UNSPECIFIED. ) ;
#40010=CARTESIAN_POINT ( 'NONE',  ( -11.42324330920000008, 1503.135554566890050, 207.5366435103790081 ) ) ;
#40016=CARTESIAN_POINT ( 'NONE',  ( -8.890910552086271679, 1451.447161361959843, 206.5067915207390001 ) ) ;
#40022=ORIENTED_EDGE ( 'NONE', *, *, #97876, .F. ) ;
#40030=EDGE_CURVE ( 'NONE', #73642, #86033, #28747, .T. ) ;
#40033=CARTESIAN_POINT ( 'NONE',  ( -1.693092047772239983, 1443.235800395060096, 218.9922115469449864 ) ) ;
#40038=FACE_BOUND ( 'NONE', #63461, .T. ) ;
#40045=CARTESIAN_POINT ( 'NONE',  ( -1.908953967214899405, 1494.973776298109669, 220.1229886510380140 ) ) ;
#40047=CARTESIAN_POINT ( 'NONE',  ( 12.85698489369999997, 1421.301446356600081, 205.5386183585989954 ) ) ;
#40064=CARTESIAN_POINT ( 'NONE',  ( 9.592729112698087590, 1425.412518091523225, 195.5100996857470932 ) ) ;
#40065=CARTESIAN_POINT ( 'NONE',  ( 4.647891285400000072, 1467.686421235989883, 217.9474878197889893 ) ) ;
#40069=CARTESIAN_POINT ( 'NONE',  ( 10.16029637529024399, 1488.802298484208677, 205.1479740240232275 ) ) ;
#40077=CARTESIAN_POINT ( 'NONE',  ( 10.14180306839999801, 1422.829400496329981, 209.7690176243060023 ) ) ;
#40078=CARTESIAN_POINT ( 'NONE',  ( 9.722207004026980570, 1428.114070666289763, 212.2005352792010058 ) ) ;
#40083=CARTESIAN_POINT ( 'NONE',  ( 5.400240006326249897, 1493.509531614239904, 218.8212082968839809 ) ) ;
#40085=CARTESIAN_POINT ( 'NONE',  ( -15.08212675520640111, 1415.677402202029953, 207.7871099719839947 ) ) ;
#40096=CARTESIAN_POINT ( 'NONE',  ( 4.355885920510000453, 1455.333275423389978, 217.9418639333990200 ) ) ;
#40097=CARTESIAN_POINT ( 'NONE',  ( 1.844551928739080138, 1456.521385733330135, 219.5817337447860211 ) ) ;
#40098=CARTESIAN_POINT ( 'NONE',  ( -8.102264060359999576, 1447.655834216490121, 213.4872354334590057 ) ) ;
#40100=DIRECTION ( 'NONE',  ( 9.156846217086110244E-47, -1.000000000000000000, 1.836970198721029688E-16 ) ) ;
#40112=CARTESIAN_POINT ( 'NONE',  ( -13.90061082261569858, 1502.276449099379988, 227.4029592858559852 ) ) ;
#40114=CARTESIAN_POINT ( 'NONE',  ( -2.389513320580931577, 1474.347589592441182, 219.1042510813949775 ) ) ;
#40119=CARTESIAN_POINT ( 'NONE',  ( 9.905242068095489572, 1468.560492227489931, 207.6656469818879884 ) ) ;
#40120=CARTESIAN_POINT ( 'NONE',  ( -3.060197654820000057, 1457.550371045389966, 218.5492501106489840 ) ) ;
#40125=B_SPLINE_SURFACE_WITH_KNOTS ( 'NONE', 5, 5, ( 
 ( #101988, #51614, #16862, #93585, #9045, #85749 ),
 ( #85195, #42656, #43219, #68432, #84643, #102534 ),
 ( #77368, #60584, #17980, #52175, #75172, #100881 ),
 ( #15758, #24175, #7396, #70648, #43761, #96925 ),
 ( #28609, #104766, #44323, #62809, #20192, #45435 ),
 ( #2338, #79037, #26960, #53281, #54390, #37002 ),
 ( #2883, #28050, #95810, #77913, #86858, #78467 ),
 ( #87420, #1780, #1219, #35917, #10150, #45977 ),
 ( #62240, #35354, #88523, #10716, #69541, #103662 ) ),
 .UNSPECIFIED., .F., .F., .F.,
 ( 6, 3, 6 ),
 ( 6, 6 ),
 ( 0.000000000000000000, 7.189919518870000026, 14.37983903770000005 ),
 ( 0.000000000000000000, 2.000000000000000000 ),
 .UNSPECIFIED. ) ;
#40126=B_SPLINE_CURVE_WITH_KNOTS ( 'NONE', 3,
 ( #57259, #13548, #83515, #108731, #39877, #23615 ),
 .UNSPECIFIED., .F., .F.,
 ( 4, 2, 4 ),
 ( 0.000000000000000000, 0.5000000000000000000, 1.000000000000000000 ),
 .UNSPECIFIED. ) ;
#40128=ORIENTED_EDGE ( 'NONE', *, *, #58613, .T. ) ;
#40134=CARTESIAN_POINT ( 'NONE',  ( -17.63951784556396163, 1419.668342365388753, 207.0221617922962878 ) ) ;
#40138=B_SPLINE_SURFACE_WITH_KNOTS ( 'NONE', 5, 5, ( 
 ( #60597, #34261, #1231, #68443, #8496, #103103 ),
 ( #104228, #76270, #33698, #52189, #67893, #86319 ),
 ( #85763, #9603, #34813, #26405, #25286, #16874 ),
 ( #94159, #17428, #61164, #9061, #77380, #43773 ),
 ( #103676, #61702, #59487, #77924, #26975, #95280 ),
 ( #18543, #93597, #51080, #44338, #52737, #35931 ) ),
 .UNSPECIFIED., .F., .F., .F.,
 ( 6, 6 ),
 ( 6, 6 ),
 ( 132.5300310469999943, 134.7130480889999831 ),
 ( 0.000000000000000000, 0.5000000000000000000 ),
 .UNSPECIFIED. ) ;
#40142=ADVANCED_FACE ( 'NONE', ( #70791 ), #65174, .T. ) ;
#40150=EDGE_LOOP ( 'NONE', ( #74322, #108399, #25939, #12911 ) ) ;
#40154=CARTESIAN_POINT ( 'NONE',  ( 10.89952677771999845, 1460.763933248429794, 208.1481502120179812 ) ) ;
#40157=CIRCLE ( 'NONE', #34807, 1.000010375718257460 ) ;
#40176=CARTESIAN_POINT ( 'NONE',  ( -6.964057390120000690, 1413.857113999770036, 207.9404136278890007 ) ) ;
#40179=CARTESIAN_POINT ( 'NONE',  ( 3.735758962120000248, 1487.094197141789891, 198.1822665823990235 ) ) ;
#40181=CARTESIAN_POINT ( 'NONE',  ( -4.390466737189999691, 1449.947854720489886, 190.5483265708990075 ) ) ;
#40187=CARTESIAN_POINT ( 'NONE',  ( -17.55780571682349844, 1508.551704408389924, 211.7873504713069792 ) ) ;
#40192=CARTESIAN_POINT ( 'NONE',  ( -11.36241000037609972, 1471.019701088729789, 208.0608489626829964 ) ) ;
#40193=CARTESIAN_POINT ( 'NONE',  ( -4.300067920883310357, 1508.175884720887780, 220.6014452582427339 ) ) ;
#40195=CARTESIAN_POINT ( 'NONE',  ( 1.351404204432949729, 1456.215857334650082, 198.6335368618340169 ) ) ;
#40198=CARTESIAN_POINT ( 'NONE',  ( -9.899088691764880821, 1472.173087826980009, 211.4694681913989882 ) ) ;
#40199=CARTESIAN_POINT ( 'NONE',  ( -5.742877853539999577, 1477.404484404390132, 219.2478600367990111 ) ) ;
#40201=EDGE_LOOP ( 'NONE', ( #97333, #6312, #98853, #31996 ) ) ;
#40204=CARTESIAN_POINT ( 'NONE',  ( 6.223484587698222548, 1441.168272379637301, 215.3989590944712234 ) ) ;
#40206=CARTESIAN_POINT ( 'NONE',  ( -3.261844206600000184, 1443.084586291889991, 200.4064849727489843 ) ) ;
#40207=CARTESIAN_POINT ( 'NONE',  ( 11.35583702168310083, 1503.040203525480138, 211.0426724955169959 ) ) ;
#40210=CARTESIAN_POINT ( 'NONE',  ( 9.345710454894810226, 1422.635914553260136, 212.8840094578699791 ) ) ;
#40212=CARTESIAN_POINT ( 'NONE',  ( 0.2964407352292510178, 1508.551704408389924, 219.9776655330169888 ) ) ;
#40216=CARTESIAN_POINT ( 'NONE',  ( -12.07091066857769945, 1502.301112229150021, 208.9299697958410036 ) ) ;
#40217=CARTESIAN_POINT ( 'NONE',  ( 10.61162123832369986, 1490.998599246300273, 212.0041548266819973 ) ) ;
#40218=CARTESIAN_POINT ( 'NONE',  ( -0.1769726758110010123, 1455.698884654190124, 218.5933451010789952 ) ) ;
#40222=CARTESIAN_POINT ( 'NONE',  ( 3.053241897432329655, 1508.551704408389924, 204.1980707054060247 ) ) ;
#40226=CARTESIAN_POINT ( 'NONE',  ( -2.898099067781480187, 1515.492902831140100, 204.9850961401090217 ) ) ;
#40229=CARTESIAN_POINT ( 'NONE',  ( -5.727657026459999301, 1464.121933083889871, 200.1990060710790260 ) ) ;
#40232=CARTESIAN_POINT ( 'NONE',  ( -15.83041352305280114, 1508.551704408389924, 214.0237305288890184 ) ) ;
#40236=CARTESIAN_POINT ( 'NONE',  ( 7.319715941259939740, 1435.586172999379869, 204.5315301320030130 ) ) ;
#40243=( BOUNDED_CURVE ( )  B_SPLINE_CURVE ( 3, ( #10124, #19618, #85720, #95236 ),
 .UNSPECIFIED., .F., .T. ) 
 B_SPLINE_CURVE_WITH_KNOTS ( ( 4, 4 ),
 ( 4.150443908561925355, 5.274333949474359962 ),
 .UNSPECIFIED. ) 
 CURVE ( )  GEOMETRIC_REPRESENTATION_ITEM ( )  RATIONAL_B_SPLINE_CURVE ( ( 1.000000000000000000, 0.8974802273446612633, 0.8974802273446612633, 1.000000000000000000 ) ) 
 REPRESENTATION_ITEM ( '' )  );
#40253=CARTESIAN_POINT ( 'NONE',  ( -3.076366055149999834, 1424.853903601579987, 191.3970713258989917 ) ) ;
#40260=CARTESIAN_POINT ( 'NONE',  ( 7.376085248378010384, 1425.097779052370015, 212.5030054048039858 ) ) ;
#40266=CARTESIAN_POINT ( 'NONE',  ( -19.18813880309999931, 1465.797355387890093, 204.3301597990889888 ) ) ;
#40268=CARTESIAN_POINT ( 'NONE',  ( -1.335447573599999993, 1487.231578949990080, 220.0114897263989917 ) ) ;
#40273=FACE_OUTER_BOUND ( 'NONE', #17459, .T. ) ;
#40282=CARTESIAN_POINT ( 'NONE',  ( -4.992349863779999453, 1391.620913471789891, 203.8075142969990168 ) ) ;
#40299=EDGE_CURVE ( 'NONE', #79128, #60672, #83702, .T. ) ;
#40302=CARTESIAN_POINT ( 'NONE',  ( 10.42801528889999929, 1420.646855367029957, 197.8923855931989806 ) ) ;
#40303=CARTESIAN_POINT ( 'NONE',  ( 0.2117397328861620187, 1431.756573977249900, 218.6125798781350227 ) ) ;
#40304=CARTESIAN_POINT ( 'NONE',  ( -10.45765233029969998, 1492.595238526010007, 202.6675476240720002 ) ) ;
#40305=CARTESIAN_POINT ( 'NONE',  ( -5.046753363489999700, 1496.785717051189977, 199.0711811026990006 ) ) ;
#40318=CARTESIAN_POINT ( 'NONE',  ( 10.68268295506589993, 1422.301575183460045, 211.2623176957549731 ) ) ;
#40319=CARTESIAN_POINT ( 'NONE',  ( 11.10553610726389984, 1424.766439379950270, 203.0669930095579900 ) ) ;
#40321=CARTESIAN_POINT ( 'NONE',  ( 2.113384585539999971, 1431.103683422689983, 218.3861821563190233 ) ) ;
#40323=CARTESIAN_POINT ( 'NONE',  ( -7.595251018561734568, 1476.838993603164909, 216.1895794634047832 ) ) ;
#40325=CARTESIAN_POINT ( 'NONE',  ( 9.005216046220072101, 1434.097723414891789, 205.2808641047390665 ) ) ;
#40329=CARTESIAN_POINT ( 'NONE',  ( -9.519812938348620079, 1460.017558366200092, 210.6311618255110147 ) ) ;
#40335=CARTESIAN_POINT ( 'NONE',  ( -7.762930123710000352, 1492.073939571090023, 209.9113589376980258 ) ) ;
#40340=CARTESIAN_POINT ( 'NONE',  ( 11.27339687608339958, 1433.557990205359829, 225.8166789818299947 ) ) ;
#40343=CARTESIAN_POINT ( 'NONE',  ( 5.012117609890212044, 1465.268517957009635, 200.5744003840434857 ) ) ;
#40354=CARTESIAN_POINT ( 'NONE',  ( -10.97842496009999991, 1492.884872791990119, 207.6491268858789851 ) ) ;
#40367=VERTEX_POINT ( 'NONE', #16340 ) ;
#40368=CARTESIAN_POINT ( 'NONE',  ( 3.984158188860000394, 1472.833767862289960, 218.5211933959089947 ) ) ;
#40370=CARTESIAN_POINT ( 'NONE',  ( 9.968391131921531922, 1469.521124705179773, 210.4613160911150089 ) ) ;
#40371=EDGE_CURVE ( 'NONE', #41801, #100706, #69564, .T. ) ;
#40406=EDGE_CURVE ( 'NONE', #44333, #38120, #91836, .T. ) ;
#40410=CARTESIAN_POINT ( 'NONE',  ( -0.3862240863000029889, 1500.063269133189806, 233.1571802061990013 ) ) ;
#40413=ORIENTED_EDGE ( 'NONE', *, *, #9898, .T. ) ;
#40419=CARTESIAN_POINT ( 'NONE',  ( 2.330134126090002145, 1515.499673595019885, 205.0355315948771988 ) ) ;
#40438=CARTESIAN_POINT ( 'NONE',  ( -16.79867715692278907, 1508.454973776049201, 213.5438332828385626 ) ) ;
#40439=CARTESIAN_POINT ( 'NONE',  ( -9.457322321504838314, 1462.148587934049829, 206.2709873367270177 ) ) ;
#40447=CARTESIAN_POINT ( 'NONE',  ( 6.639614474480000084, 1470.122678494290085, 210.8877727176889891 ) ) ;
#40452=CARTESIAN_POINT ( 'NONE',  ( -4.682234856550000046, 1438.893385222290135, 227.1256850459990062 ) ) ;
#40455=CARTESIAN_POINT ( 'NONE',  ( 2.936817763032770312, 1515.374151778960140, 213.3816236606869836 ) ) ;
#40456=CARTESIAN_POINT ( 'NONE',  ( -1.894502717228039979, 1483.831863175760191, 198.6119618997200007 ) ) ;
#40457=CARTESIAN_POINT ( 'NONE',  ( -12.10387469771020008, 1501.702042382700029, 211.4972372465589956 ) ) ;
#40461=CARTESIAN_POINT ( 'NONE',  ( 3.303701760970000123, 1508.421385209789833, 219.9897194252990005 ) ) ;
#40463=CARTESIAN_POINT ( 'NONE',  ( 2.448891952219999890, 1435.321209562490139, 227.4386027112989836 ) ) ;
#40472=CARTESIAN_POINT ( 'NONE',  ( 19.37001854000000023, 1457.793959969789967, 211.0198531007490033 ) ) ;
#40489=CARTESIAN_POINT ( 'NONE',  ( 5.277460848200000498, 1426.742654866309977, 191.8370381630989812 ) ) ;
#40497=DIRECTION ( 'NONE',  ( -0.9980318515193558060, 0.000000000000000000, -0.06270903725019710828 ) ) ;
#40500=CARTESIAN_POINT ( 'NONE',  ( -20.87069991009999725, 1506.658021081189872, 214.5368842940590071 ) ) ;
#40506=ADVANCED_FACE ( 'NONE', ( #55502 ), #89081, .T. ) ;
#40507=CARTESIAN_POINT ( 'NONE',  ( 12.89505231660000106, 1420.989630775359956, 203.4267439564690108 ) ) ;
#40511=CARTESIAN_POINT ( 'NONE',  ( -13.59430914469499996, 1507.912413286850096, 209.4080442005970042 ) ) ;
#40512=CARTESIAN_POINT ( 'NONE',  ( 10.37958006579530057, 1453.090549329029727, 190.0119551464189840 ) ) ;
#40523=CARTESIAN_POINT ( 'NONE',  ( -23.17200737914519948, 1417.287767808789795, 209.8650901584490214 ) ) ;
#40543=CARTESIAN_POINT ( 'NONE',  ( -17.00797328670000397, 1417.537217351680056, 207.7155449971589860 ) ) ;
#40549=ORIENTED_EDGE ( 'NONE', *, *, #54943, .F. ) ;
#40561=CARTESIAN_POINT ( 'NONE',  ( -11.38797607120000066, 1501.230572076990029, 208.0053829869090123 ) ) ;
#40572=FACE_OUTER_BOUND ( 'NONE', #73474, .T. ) ;
#40582=ADVANCED_FACE ( 'NONE', ( #73947 ), #15108, .T. ) ;
#40584=CARTESIAN_POINT ( 'NONE',  ( 3.001614222390000197, 1441.369934486689999, 218.5760139890790299 ) ) ;
#40587=CARTESIAN_POINT ( 'NONE',  ( 9.781792257336670460, 1435.212511321700049, 208.3818996341230161 ) ) ;
#40599=CARTESIAN_POINT ( 'NONE',  ( 12.02413026890000047, 1426.614203559159932, 205.4717539480090238 ) ) ;
#40601=ADVANCED_FACE ( 'NONE', ( #1110 ), #16016, .T. ) ;
#40612=CARTESIAN_POINT ( 'NONE',  ( 10.91793180594200052, 1461.492375007339888, 210.1518181392050053 ) ) ;
#40614=CARTESIAN_POINT ( 'NONE',  ( 4.303723356569999936, 1466.891311542389758, 218.2258331277790262 ) ) ;
#40626=EDGE_CURVE ( 'NONE', #75973, #84881, #86647, .T. ) ;
#40629=CARTESIAN_POINT ( 'NONE',  ( 10.81714288539756730, 1427.819672987908461, 210.7127296406635537 ) ) ;
#40631=AXIS2_PLACEMENT_3D ( 'NONE', #85767, #77384, #109340 ) ;
#40633=CARTESIAN_POINT ( 'NONE',  ( -8.639773871640201719, 1437.117077603399821, 209.3259169240039910 ) ) ;
#40636=CARTESIAN_POINT ( 'NONE',  ( -14.86020447212730033, 1415.677402202029953, 206.8262383623809910 ) ) ;
#40637=CARTESIAN_POINT ( 'NONE',  ( -1.172395513999999869E-13, 1415.677402202029953, 209.1218459616989946 ) ) ;
#40644=ORIENTED_EDGE ( 'NONE', *, *, #11724, .F. ) ;
#40648=CARTESIAN_POINT ( 'NONE',  ( 4.240943730709999748, 1455.710924186590091, 218.4112998676390021 ) ) ;
#40653=CARTESIAN_POINT ( 'NONE',  ( -4.240938128602147472, 1509.032014137962278, 212.8662754392913143 ) ) ;
#40667=CARTESIAN_POINT ( 'NONE',  ( -21.45377186783750290, 1505.623606155929792, 215.8817182770680176 ) ) ;
#40669=CARTESIAN_POINT ( 'NONE',  ( 0.6589060341152864764, 1473.309946152746534, 219.3202346236175231 ) ) ;
#40673=CARTESIAN_POINT ( 'NONE',  ( -7.304960004490000713, 1480.235071529190009, 209.0219926440400116 ) ) ;
#40675=CARTESIAN_POINT ( 'NONE',  ( -3.512275926230000067, 1456.435201441189975, 217.9329361306089936 ) ) ;
#40682=AXIS2_PLACEMENT_3D ( 'NONE', #19106, #10745, #44918 ) ;
#40693=VERTEX_POINT ( 'NONE', #1522 ) ;
#40707=CARTESIAN_POINT ( 'NONE',  ( 4.520890098355639708, 1426.568512013200007, 191.6274461433459919 ) ) ;
#40714=CARTESIAN_POINT ( 'NONE',  ( 5.200694988025460042, 1440.224034440930154, 217.6292548469920121 ) ) ;
#40717=EDGE_LOOP ( 'NONE', ( #19980, #35327, #32805, #67846 ) ) ;
#40719=CARTESIAN_POINT ( 'NONE',  ( -10.13020165310000031, 1472.545330956490034, 208.0133926034690148 ) ) ;
#40728=CARTESIAN_POINT ( 'NONE',  ( 10.72219805821039884, 1490.875092374679980, 211.5234845686590006 ) ) ;
#40729=CARTESIAN_POINT ( 'NONE',  ( 4.798310207610000155, 1486.425997147189946, 199.4446566442690028 ) ) ;
#40740=CARTESIAN_POINT ( 'NONE',  ( -2.609190002560000110, 1475.351101089589974, 219.2386560539989944 ) ) ;
#40742=CARTESIAN_POINT ( 'NONE',  ( -11.40514982007739953, 1470.815891563210016, 208.9000713169049845 ) ) ;
#40743=CARTESIAN_POINT ( 'NONE',  ( -7.069698889257053587, 1508.382370789888455, 219.7441700735184895 ) ) ;
#40745=CARTESIAN_POINT ( 'NONE',  ( 1.779428963082609894, 1456.357349037730046, 198.6855221610310309 ) ) ;
#40746=CARTESIAN_POINT ( 'NONE',  ( -4.086314431204999487, 1515.499673567537911, 210.9648096920523983 ) ) ;
#40756=CARTESIAN_POINT ( 'NONE',  ( -1.464162264810000114, 1442.883873453590013, 200.3486113609690165 ) ) ;
#40757=CARTESIAN_POINT ( 'NONE',  ( 11.76499821370110155, 1501.784643893570092, 211.4691548758199815 ) ) ;
#40761=TOROIDAL_SURFACE ( 'NONE', #1377, 4.250000000000000000, 0.5000000000000000000 ) ;
#40767=CARTESIAN_POINT ( 'NONE',  ( -12.43173911540150023, 1502.554234090240016, 208.9876481361740161 ) ) ;
#40768=CARTESIAN_POINT ( 'NONE',  ( 11.81690186861369973, 1492.270327107419917, 210.4669352574049981 ) ) ;
#40775=CARTESIAN_POINT ( 'NONE',  ( 8.559858904628349308, 1437.030483964089854, 207.9845584131589931 ) ) ;
#40776=ORIENTED_EDGE ( 'NONE', *, *, #9026, .T. ) ;
#40782=CARTESIAN_POINT ( 'NONE',  ( -9.183711187100000117, 1463.569275765890097, 202.8257126108990178 ) ) ;
#40785=CARTESIAN_POINT ( 'NONE',  ( -12.74120642066979947, 1508.551704408389924, 216.7626981741809971 ) ) ;
#40794=ORIENTED_EDGE ( 'NONE', *, *, #13862, .T. ) ;
#40799=CARTESIAN_POINT ( 'NONE',  ( -0.3104492283789259122, 1515.598602702389826, 213.1604326987470017 ) ) ;
#40805=CARTESIAN_POINT ( 'NONE',  ( 2.272601175003300167, 1429.102097603389893, 217.0941385727449813 ) ) ;
#40812=CARTESIAN_POINT ( 'NONE',  ( 7.385549640129020155, 1425.110251876329812, 212.4835268894509852 ) ) ;
#40820=CARTESIAN_POINT ( 'NONE',  ( -4.636806382847598940, 1378.035560348909030, 214.3314208189594297 ) ) ;
#40827=CARTESIAN_POINT ( 'NONE',  ( 11.45308832699999968, 1502.277520793189979, 208.2819378797420029 ) ) ;
#40835=CARTESIAN_POINT ( 'NONE',  ( 20.88002914659999831, 1495.383068942589944, 212.2131686182190151 ) ) ;
#40838=B_SPLINE_CURVE_WITH_KNOTS ( 'NONE', 3,
 ( #40745, #48055, #92250, #64322, #23384, #40195, #82191, #31789, #65423, #98443, #99530, #23923, #66532, #38535, #57574, #81090, #90036, #55917, #47507, #91148, #91699, #39077, #81631, #74377, #6595, #108503, #74921, #39650, #107948, #64877, #109072, #32353, #100636, #14423, #73255, #26693, #85483 ),
 .UNSPECIFIED., .F., .F.,
 ( 4, 3, 3, 3, 3, 3, 3, 3, 3, 3, 3, 3, 4 ),
 ( -13.00030988960000045, -12.70431845186110031, -12.03435738184399995, -11.32254726432860004, -10.57086120063609869, -9.761044970981449964, -8.781608299062758860, -7.853302061585090144, -7.046341670537930035, -6.091992644973400317, -5.300241650221800604, -4.613009676061491149, -3.966463181889999134 ),
 .UNSPECIFIED. ) ;
#40854=CARTESIAN_POINT ( 'NONE',  ( 7.214474816066029028, 1504.316466902849925, 219.6367501992550046 ) ) ;
#40855=CARTESIAN_POINT ( 'NONE',  ( 7.782064256880000030, 1421.606440417200020, 195.8228046871990102 ) ) ;
#40856=CARTESIAN_POINT ( 'NONE',  ( 1.181149777510320131, 1431.413309031290055, 218.5383434680610151 ) ) ;
#40857=CARTESIAN_POINT ( 'NONE',  ( 10.65417391917219980, 1479.073446957750093, 205.9772944084500068 ) ) ;
#40866=FACE_OUTER_BOUND ( 'NONE', #4065, .T. ) ;
#40871=CARTESIAN_POINT ( 'NONE',  ( 9.661937460982130688, 1423.484310766260023, 209.7266508472010003 ) ) ;
#40872=CARTESIAN_POINT ( 'NONE',  ( 10.99916455748379995, 1424.384112525169940, 203.1270655916410135 ) ) ;
#40879=CARTESIAN_POINT ( 'NONE',  ( -16.79355120555579717, 1420.470915846049820, 203.2250788671829866 ) ) ;
#40881=CARTESIAN_POINT ( 'NONE',  ( 7.600171787371139409, 1465.644562267609899, 215.5555306133580018 ) ) ;
#40883=CARTESIAN_POINT ( 'NONE',  ( 5.343927860473110414, 1473.943544974919860, 219.2193853163629740 ) ) ;
#40888=CARTESIAN_POINT ( 'NONE',  ( 1.491420627269999910, 1515.551704408389924, 205.2164164778889983 ) ) ;
#40890=CARTESIAN_POINT ( 'NONE',  ( 1.968601690575629615, 1498.935401749600032, 197.9561509338619771 ) ) ;
#40892=( BOUNDED_CURVE ( )  B_SPLINE_CURVE ( 3, ( #53824, #51592, #34779, #68965 ),
 .UNSPECIFIED., .F., .T. ) 
 B_SPLINE_CURVE_WITH_KNOTS ( ( 4, 4 ),
 ( 4.163468865690415299, 5.261334023187549391 ),
 .UNSPECIFIED. ) 
 CURVE ( )  GEOMETRIC_REPRESENTATION_ITEM ( )  RATIONAL_B_SPLINE_CURVE ( ( 1.000000000000000000, 0.9020546424876372260, 0.9020546424876372260, 1.000000000000000000 ) ) 
 REPRESENTATION_ITEM ( '' )  );
#40902=B_SPLINE_SURFACE_WITH_KNOTS ( 'NONE', 5, 1, ( 
 ( #30966, #100379 ),
 ( #55650, #99810 ),
 ( #23104, #5784 ),
 ( #64603, #15250 ),
 ( #23664, #29863 ),
 ( #5219, #65141 ) ),
 .UNSPECIFIED., .F., .F., .F.,
 ( 6, 6 ),
 ( 2, 2 ),
 ( 0.000000000000000000, 15.53865474348330089 ),
 ( 0.000000000000000000, 14.00001426917759950 ),
 .UNSPECIFIED. ) ;
#40904=CARTESIAN_POINT ( 'NONE',  ( 9.659057376369998948, 1477.882669201989984, 202.4105350377390096 ) ) ;
#40906=DIRECTION ( 'NONE',  ( 0.02091224828123159837, -0.9990482215818557998, 0.03827961371219689574 ) ) ;
#40907=CARTESIAN_POINT ( 'NONE',  ( -5.682011391568829950, 1434.576080618040123, 216.5206222332380150 ) ) ;
#40910=CARTESIAN_POINT ( 'NONE',  ( -15.32670450039999999, 1414.929621208459821, 211.2240752700589894 ) ) ;
#40913=B_SPLINE_SURFACE_WITH_KNOTS ( 'NONE', 5, 1, ( 
 ( #63643, #88815 ),
 ( #36757, #64185 ),
 ( #106704, #70950 ),
 ( #3186, #45736 ),
 ( #37315, #29994 ),
 ( #70391, #71510 ) ),
 .UNSPECIFIED., .F., .F., .F.,
 ( 6, 6 ),
 ( 2, 2 ),
 ( 0.000000000000000000, 3.407694589789999728 ),
 ( 0.000000000000000000, 14.00000000000000000 ),
 .UNSPECIFIED. ) ;
#40916=CARTESIAN_POINT ( 'NONE',  ( 10.39668864703249973, 1424.335650574019837, 206.8537076104200025 ) ) ;
#40923=CARTESIAN_POINT ( 'NONE',  ( 3.438860216040000140, 1473.468534316989917, 218.9084199681889800 ) ) ;
#40925=CARTESIAN_POINT ( 'NONE',  ( 10.10501075033869967, 1471.402064569889944, 212.2221579359460009 ) ) ;
#40935=CARTESIAN_POINT ( 'NONE',  ( 7.257468615629999675, 1448.222523044890295, 203.1720000238289856 ) ) ;
#40943=CARTESIAN_POINT ( 'NONE',  ( -2.664535259099999805E-15, 1424.786834349990158, 209.1218459616989946 ) ) ;
#40950=CARTESIAN_POINT ( 'NONE',  ( 11.90463986800000029, 1500.041165469490124, 206.3230776397589921 ) ) ;
#40956=CARTESIAN_POINT ( 'NONE',  ( -3.829620113550000315, 1515.551704408389924, 211.4519800877889963 ) ) ;
#40957=CARTESIAN_POINT ( 'NONE',  ( 12.62398172905319882, 1500.937524318219857, 210.6201263454209993 ) ) ;
#40961=CARTESIAN_POINT ( 'NONE',  ( -20.36853080839999919, 1464.956632876090225, 210.9458194778790130 ) ) ;
#40973=CARTESIAN_POINT ( 'NONE',  ( 12.65728676410210163, 1420.119835224449844, 200.3472210950669989 ) ) ;
#40983=AXIS2_PLACEMENT_3D ( 'NONE', #84835, #102732, #17057 ) ;
#40987=CARTESIAN_POINT ( 'NONE',  ( 5.994546415740489742, 1429.671868418749909, 216.4766293005329771 ) ) ;
#40988=CARTESIAN_POINT ( 'NONE',  ( -7.823403845102177456, 1435.182002661693332, 212.6572978892697563 ) ) ;
#40989=CARTESIAN_POINT ( 'NONE',  ( -9.771304594386510445, 1462.553183801680007, 206.2411433844070245 ) ) ;
#40991=CARTESIAN_POINT ( 'NONE',  ( 9.905021055853989509, 1468.629943020290057, 207.6432958796129924 ) ) ;
#40992=CARTESIAN_POINT ( 'NONE',  ( -10.54299263360008432, 1469.936041725191217, 213.3752367157486560 ) ) ;
#40996=CARTESIAN_POINT ( 'NONE',  ( 2.487935084889999704, 1508.551704408389924, 214.1089244042930204 ) ) ;
#41006=CARTESIAN_POINT ( 'NONE',  ( 4.138326088227719524, 1515.492270357839971, 211.4517668477679990 ) ) ;
#41010=CARTESIAN_POINT ( 'NONE',  ( -15.51611637578909253, 1415.679618464087071, 209.5978448638990415 ) ) ;
#41011=CARTESIAN_POINT ( 'NONE',  ( -2.182617347539999919, 1508.212127139989889, 220.8438686939989850 ) ) ;
#41016=CARTESIAN_POINT ( 'NONE',  ( 7.923742487380000199, 1501.702996767189916, 206.8471783426489878 ) ) ;
#41017=CARTESIAN_POINT ( 'NONE',  ( 9.201169484990000313, 1472.509397971289900, 190.7635733242989886 ) ) ;
#41021=CIRCLE ( 'NONE', #99998, 11.71219856409999949 ) ;
#41022=ORIENTED_EDGE ( 'NONE', *, *, #34725, .T. ) ;
#41032=CARTESIAN_POINT ( 'NONE',  ( -16.02484169309999729, 1417.968543311129906, 204.0964181816090104 ) ) ;
#41036=CARTESIAN_POINT ( 'NONE',  ( -16.21393388683536330, 1419.735053903993730, 209.9280921983989003 ) ) ;
#41037=CARTESIAN_POINT ( 'NONE',  ( -3.805400412610000060, 1495.647977866990004, 219.6495694401989738 ) ) ;
#41048=CARTESIAN_POINT ( 'NONE',  ( -10.17701364196129887, 1462.839837219120000, 206.1633443696570112 ) ) ;
#41050=B_SPLINE_SURFACE_WITH_KNOTS ( 'NONE', 5, 5, ( 
 ( #52474, #79875, #27253, #69277, #79322, #96674 ),
 ( #95012, #36759, #68727, #3189, #86602, #77658 ),
 ( #102832, #26689, #9353, #53025, #87732, #105068 ),
 ( #2633, #28357, #971, #62555, #11562, #35096 ),
 ( #45738, #87161, #26126, #19382, #2080, #94433 ),
 ( #95560, #18830, #103383, #45181, #60885, #44064 ),
 ( #10450, #78764, #104512, #36209, #70394, #27809 ),
 ( #61991, #65287, #89908, #38943, #63645, #47918 ),
 ( #73694, #37869, #107820, #82053, #3736, #12659 ),
 ( #29996, #4272, #31108, #29448, #13182, #14298 ),
 ( #56324, #91008, #63109, #38402, #13734, #5359 ),
 ( #21587, #4798, #55793, #97760, #107265, #21032 ),
 ( #64187, #98861, #99400, #71512, #37317, #47371 ),
 ( #81496, #97208, #46838, #73123, #106706, #12103 ),
 ( #39518, #89368, #55235, #80967, #90456, #72578 ),
 ( #30560, #64750, #22125, #22679, #56878, #98309 ),
 ( #48487, #54691, #20481, #82627, #105631, #88817 ),
 ( #28918, #46296, #80424, #72054, #106169, #57447 ),
 ( #32760, #14848, #23249, #59636, #99954, #66943 ),
 ( #49039, #75342, #74244, #84805, #100517, #108374 ),
 ( #68051, #59091, #49585, #66397, #25442, #83716 ) ),
 .UNSPECIFIED., .F., .F., .F.,
 ( 6, 3, 3, 3, 3, 3, 6 ),
 ( 6, 6 ),
 ( 2.123077381369999905, 2.437842270119999988, 2.821447585090000043, 3.205052900050000098, 4.739453051259999938, 7.802280429849999699, 10.88241929079999970 ),
 ( 0.000000000000000000, 2.000000000000000000 ),
 .UNSPECIFIED. ) ;
#41057=CARTESIAN_POINT ( 'NONE',  ( 11.35315220146310011, 1478.711703769590031, 206.1320505837120152 ) ) ;
#41062=CARTESIAN_POINT ( 'NONE',  ( 5.093836579314430679, 1436.649832418680035, 228.7462252422310200 ) ) ;
#41064=CARTESIAN_POINT ( 'NONE',  ( -9.771939461242810765, 1448.872234804809978, 190.8346844886999918 ) ) ;
#41068=AXIS2_PLACEMENT_3D ( 'NONE', #34050, #479, #92296 ) ;
#41076=CARTESIAN_POINT ( 'NONE',  ( -16.16601204028820149, 1420.773371822770059, 203.3216470037820045 ) ) ;
#41082=ORIENTED_EDGE ( 'NONE', *, *, #90599, .T. ) ;
#41090=CARTESIAN_POINT ( 'NONE',  ( 3.094100512289999827, 1445.021403822989896, 200.6774107941290026 ) ) ;
#41093=CARTESIAN_POINT ( 'NONE',  ( -4.342662522768870659, 1464.389982461639875, 199.4525629763099914 ) ) ;
#41094=CARTESIAN_POINT ( 'NONE',  ( -17.54273015099310129, 1417.931783278020021, 206.8684746656099946 ) ) ;
#41104=EDGE_CURVE ( 'NONE', #77481, #29796, #99979, .T. ) ;
#41114=ORIENTED_EDGE ( 'NONE', *, *, #24725, .T. ) ;
#41116=VERTEX_POINT ( 'NONE', #55241 ) ;
#41132=CARTESIAN_POINT ( 'NONE',  ( 16.98839455092350192, 1428.323430003820022, 202.7579036764070111 ) ) ;
#41137=CARTESIAN_POINT ( 'NONE',  ( 9.686384332386170470, 1434.926238005200048, 207.6434806796090129 ) ) ;
#41139=FACE_OUTER_BOUND ( 'NONE', #61803, .T. ) ;
#41145=B_SPLINE_SURFACE_WITH_KNOTS ( 'NONE', 5, 5, ( 
 ( #91522, #74734, #83661, #92609, #109979, #57936 ),
 ( #14246, #59040, #92068, #33255, #107767, #56823 ),
 ( #40561, #108319, #58481, #24299, #65781, #48435 ),
 ( #49536, #73637, #15340, #15884, #75289, #82577 ),
 ( #67446, #6957, #6416, #5306, #48987, #108870 ),
 ( #31603, #39465, #99344, #5868, #99899, #13676 ),
 ( #22620, #40010, #32161, #7509, #66894, #41671 ),
 ( #66348, #74190, #23196, #50085, #101002, #14801 ),
 ( #83120, #100465, #23748, #109435, #32712, #84213 ) ),
 .UNSPECIFIED., .F., .F., .F.,
 ( 6, 3, 6 ),
 ( 6, 6 ),
 ( 0.5394538425010000360, 1.941044340399999957, 4.123493948330000158 ),
 ( 0.000000000000000000, 2.000000000000000000 ),
 .UNSPECIFIED. ) ;
#41150=CARTESIAN_POINT ( 'NONE',  ( 0.4193190673965659920, 1494.284500131298500, 220.2488346745992942 ) ) ;
#41158=CARTESIAN_POINT ( 'NONE',  ( -9.288805682565799415, 1448.817640831179915, 209.5382110545150169 ) ) ;
#41166=CARTESIAN_POINT ( 'NONE',  ( 10.81897510151069852, 1461.808313873119914, 210.9528785559000141 ) ) ;
#41170=CARTESIAN_POINT ( 'NONE',  ( 3.775314256393730084, 1507.374707593759922, 220.2027404254530154 ) ) ;
#41178=ADVANCED_FACE ( 'NONE', ( #57175 ), #58969, .T. ) ;
#41180=EDGE_LOOP ( 'NONE', ( #82433, #105863, #42237, #13980 ) ) ;
#41181=CARTESIAN_POINT ( 'NONE',  ( -8.224133852202001549, 1439.811765298699811, 205.6917440491770037 ) ) ;
#41183=EDGE_CURVE ( 'NONE', #51752, #106043, #70263, .T. ) ;
#41191=CARTESIAN_POINT ( 'NONE',  ( 2.807700783748780182, 1495.041702816110046, 220.3586040259340280 ) ) ;
#41192=EDGE_CURVE ( 'NONE', #25016, #57781, #16835, .T. ) ;
#41201=CARTESIAN_POINT ( 'NONE',  ( 1.702416261868870073, 1493.957958506549858, 220.1113518634800243 ) ) ;
#41206=CARTESIAN_POINT ( 'NONE',  ( 2.501002156060000203, 1456.165277925289956, 219.0283583277490038 ) ) ;
#41207=CARTESIAN_POINT ( 'NONE',  ( 1.651430464342579896, 1456.566497830990102, 219.6140531495319976 ) ) ;
#41208=CARTESIAN_POINT ( 'NONE',  ( -3.311233732019999820, 1444.392778043689987, 217.8868263135390180 ) ) ;
#41211=CARTESIAN_POINT ( 'NONE',  ( 9.525081731767038207, 1464.196465044419938, 211.5190840894209998 ) ) ;
#41212=CARTESIAN_POINT ( 'NONE',  ( 7.301745199710000023, 1423.622635854230111, 213.2704416234889777 ) ) ;
#41219=VERTEX_POINT ( 'NONE', #25171 ) ;
#41223=CARTESIAN_POINT ( 'NONE',  ( -13.81174872492939976, 1503.065987535760087, 227.5153026160529919 ) ) ;
#41226=( BOUNDED_CURVE ( )  B_SPLINE_CURVE ( 3, ( #61550, #10017, #53144, #87282 ),
 .UNSPECIFIED., .F., .F. ) 
 B_SPLINE_CURVE_WITH_KNOTS ( ( 4, 4 ),
 ( 2.356485375018650075, 3.926596517583369916 ),
 .UNSPECIFIED. ) 
 CURVE ( )  GEOMETRIC_REPRESENTATION_ITEM ( )  RATIONAL_B_SPLINE_CURVE ( ( 1.000000000000000000, 0.8048993259288232949, 0.8048993259288232949, 1.000000000000000000 ) ) 
 REPRESENTATION_ITEM ( '' )  );
#41231=CARTESIAN_POINT ( 'NONE',  ( 17.85932443592169960, 1430.949825052579854, 205.3160887855020178 ) ) ;
#41237=VERTEX_POINT ( 'NONE', #99423 ) ;
#41252=EDGE_CURVE ( 'NONE', #58610, #80101, #32924, .T. ) ;
#41257=LINE ( 'NONE', #16026, #86510 ) ;
#41262=CARTESIAN_POINT ( 'NONE',  ( 1.125466269979470191, 1425.802411463860153, 191.1258191377030187 ) ) ;
#41268=CARTESIAN_POINT ( 'NONE',  ( -2.455930012020000053, 1497.729421728190118, 200.9736040853090060 ) ) ;
#41269=CARTESIAN_POINT ( 'NONE',  ( 4.943223444412789824, 1441.096092932190004, 216.6493757176620250 ) ) ;
#41285=CARTESIAN_POINT ( 'NONE',  ( 8.809986217320000534, 1488.981908579989977, 201.8653081004390231 ) ) ;
#41293=ORIENTED_EDGE ( 'NONE', *, *, #106335, .F. ) ;
#41298=CARTESIAN_POINT ( 'NONE',  ( -3.439961641710000517, 1475.703222190290035, 218.9903650269789921 ) ) ;
#41301=CARTESIAN_POINT ( 'NONE',  ( -1.247057868944360104, 1423.218537098029856, 191.2427100806079920 ) ) ;
#41302=CARTESIAN_POINT ( 'NONE',  ( -11.25721726106180043, 1471.236964352069890, 207.2321767610409893 ) ) ;
#41303=CARTESIAN_POINT ( 'NONE',  ( -7.460430899790702064, 1508.409396344885863, 219.6019905338215494 ) ) ;
#41308=CARTESIAN_POINT ( 'NONE',  ( -9.699590169216451230, 1472.031374714349795, 212.1565849597349995 ) ) ;
#41309=CARTESIAN_POINT ( 'NONE',  ( 4.328706393743970260, 1515.093143318830244, 207.9156808863739911 ) ) ;
#41311=ORIENTED_EDGE ( 'NONE', *, *, #69228, .T. ) ;
#41317=CARTESIAN_POINT ( 'NONE',  ( -14.17032501240000109, 1507.703614819789891, 209.3618925486269973 ) ) ;
#41318=CARTESIAN_POINT ( 'NONE',  ( 11.60172759230599837, 1502.019123038000089, 211.3760841748210169 ) ) ;
#41322=CARTESIAN_POINT ( 'NONE',  ( 9.555172118568348694, 1422.588896727079828, 212.6615495601689929 ) ) ;
#41324=CARTESIAN_POINT ( 'NONE',  ( -4.282704111109999268, 1515.349907855090123, 208.0217043178890037 ) ) ;
#41330=CARTESIAN_POINT ( 'NONE',  ( 1.295798300469999997, 1456.648087910589993, 219.6777443815990125 ) ) ;
#41334=CARTESIAN_POINT ( 'NONE',  ( 0.2196276506829989983, 1429.899695672290136, 217.4576539075590063 ) ) ;
#41338=CARTESIAN_POINT ( 'NONE',  ( -21.30496379579999910, 1505.027833310889946, 212.2085733242190031 ) ) ;
#41339=CARTESIAN_POINT ( 'NONE',  ( -3.829164872246469731, 1515.551704201149960, 206.7918886383120025 ) ) ;
#41342=CARTESIAN_POINT ( 'NONE',  ( -8.451623981890000081, 1463.123780996790174, 203.2630781829089983 ) ) ;
#41344=CARTESIAN_POINT ( 'NONE',  ( -4.367937192439999450, 1447.898255911189835, 190.6350925615990093 ) ) ;
#41348=CARTESIAN_POINT ( 'NONE',  ( -7.649966233313090669, 1508.551704408389924, 219.0282755267929815 ) ) ;
#41349=CARTESIAN_POINT ( 'NONE',  ( -1.883109339810000060, 1456.914664128490131, 202.5483680118790062 ) ) ;
#41350=B_SPLINE_CURVE_WITH_KNOTS ( 'NONE', 3,
 ( #52759, #70140, #9086, #43252, #79622, #87465, #88026, #104804, #34834, #44362, #69023, #28092, #26426, #35954, #62854, #96966, #80150, #56054, #30284, #56608, #5653, #82352, #64476, #29198, #39801, #54972, #81236, #65011, #20772, #47109, #97503, #106453, #89098, #63922, #12386, #4551, #39235 ),
 .UNSPECIFIED., .F., .F.,
 ( 4, 3, 3, 3, 3, 3, 3, 3, 3, 3, 3, 3, 4 ),
 ( -2.000000000000000000, -1.966354504360819933, -1.792372297947200099, -1.616329574349380183, -1.438982451719919897, -1.251976602293230156, -1.072120690327510006, -0.8919554514786369737, -0.7119274688212668956, -0.5279171072243049601, -0.3502797711574010542, -0.1742312679962050304, 0.000000000000000000 ),
 .UNSPECIFIED. ) ;
#41352=CARTESIAN_POINT ( 'NONE',  ( 0.6499393709957180798, 1486.288793463719912, 197.2259022801050037 ) ) ;
#41353=CARTESIAN_POINT ( 'NONE',  ( 7.374876521353709968, 1435.142022087859914, 204.6561785625810046 ) ) ;
#41364=CARTESIAN_POINT ( 'NONE',  ( 1.847634168259999932, 1478.089546575790109, 198.8590796125990039 ) ) ;
#41371=CARTESIAN_POINT ( 'NONE',  ( 0.7439185208581500230, 1429.698669720969974, 217.4034785395159872 ) ) ;
#41372=CARTESIAN_POINT ( 'NONE',  ( -4.222176722049999498, 1443.314582379889771, 199.9747765569790090 ) ) ;
#41377=CARTESIAN_POINT ( 'NONE',  ( 7.522034444203620218, 1425.444008626959885, 212.2045359387309702 ) ) ;
#41382=CARTESIAN_POINT ( 'NONE',  ( -10.93477970757400008, 1492.771114947679962, 207.3280309501589898 ) ) ;
#41384=CARTESIAN_POINT ( 'NONE',  ( -6.379043878270000079, 1461.120655808090078, 208.1971959041119931 ) ) ;
#41385=CARTESIAN_POINT ( 'NONE',  ( -16.32163182381450284, 1508.551704408389924, 213.4489841974129831 ) ) ;
#41386=CARTESIAN_POINT ( 'NONE',  ( -2.074953700500000053, 1486.986190320790229, 220.1252486097989731 ) ) ;
#41387=EDGE_CURVE ( 'NONE', #3936, #103706, #54023, .T. ) ;
#41403=CARTESIAN_POINT ( 'NONE',  ( 4.832611295398050011, 1508.551704408489968, 211.6097683635340161 ) ) ;
#41412=CARTESIAN_POINT ( 'NONE',  ( 0.4985499550132489466, 1445.062937618880142, 199.0667931780290019 ) ) ;
#41416=EDGE_CURVE ( 'NONE', #33283, #105726, #52992, .T. ) ;
#41418=CARTESIAN_POINT ( 'NONE',  ( -4.449471081727619293, 1508.551704408389924, 213.1599751400310083 ) ) ;
#41421=CARTESIAN_POINT ( 'NONE',  ( 7.986285408849999712, 1421.471180981509860, 195.9504200288989750 ) ) ;
#41423=CARTESIAN_POINT ( 'NONE',  ( 10.06162192388379850, 1480.175689251570020, 205.9450596422540229 ) ) ;
#41426=FACE_OUTER_BOUND ( 'NONE', #70658, .T. ) ;
#41431=ORIENTED_EDGE ( 'NONE', *, *, #88115, .F. ) ;
#41437=CARTESIAN_POINT ( 'NONE',  ( 9.912752747455510161, 1426.220655830240048, 209.0668641679729944 ) ) ;
#41438=CARTESIAN_POINT ( 'NONE',  ( 10.98117345485269958, 1424.286751519139898, 203.1416149009169771 ) ) ;
#41439=CARTESIAN_POINT ( 'NONE',  ( -10.85475431940500002, 1462.808527540379828, 207.0334558119959638 ) ) ;
#41445=CARTESIAN_POINT ( 'NONE',  ( -9.666742485873120572, 1460.834176539050077, 209.6559978844479986 ) ) ;
#41447=CARTESIAN_POINT ( 'NONE',  ( 10.61252713196669895, 1425.442803612520038, 197.7433300990009855 ) ) ;
#41448=CARTESIAN_POINT ( 'NONE',  ( 8.460065138274888596, 1464.559580154269952, 214.4881923900420020 ) ) ;
#41454=CARTESIAN_POINT ( 'NONE',  ( -8.123331533938953797, 1425.256042585743444, 209.1379764726806911 ) ) ;
#41462=CARTESIAN_POINT ( 'NONE',  ( -18.98876737475859855, 1419.092652900649909, 207.4035108679890129 ) ) ;
#41466=ORIENTED_EDGE ( 'NONE', *, *, #87035, .T. ) ;
#41467=B_SPLINE_CURVE_WITH_KNOTS ( 'NONE', 3,
 ( #30088, #98403, #21675, #109029, #84361, #30654, #83809, #100057, #23344, #64840, #82152, #24436, #41262, #7108, #74878, #49128, #48015, #58077, #98948, #92210, #22771, #32312, #40707, #56977, #83261 ),
 .UNSPECIFIED., .F., .F.,
 ( 4, 3, 3, 3, 3, 3, 3, 3, 4 ),
 ( 0.000000000000000000, 0.9101832234901460206, 1.814229467067710155, 2.708290536397560011, 3.291079314230000108, 3.823282037274009948, 4.734358896883110290, 5.649465372364789850, 6.557401248809999750 ),
 .UNSPECIFIED. ) ;
#41474=CARTESIAN_POINT ( 'NONE',  ( -1.954670228789999964, 1485.152615003790061, 198.1756555629989975 ) ) ;
#41475=CARTESIAN_POINT ( 'NONE',  ( 9.605737541349999020, 1478.647301563190013, 203.8155412612589998 ) ) ;
#41476=CARTESIAN_POINT ( 'NONE',  ( -16.55223816414050120, 1420.586707762020069, 203.2624066023280136 ) ) ;
#41477=CARTESIAN_POINT ( 'NONE',  ( 19.45418216399269795, 1498.414413235519987, 218.7471445023780063 ) ) ;
#41478=CARTESIAN_POINT ( 'NONE',  ( 18.99535453092520143, 1472.738766242029897, 202.2605984988649936 ) ) ;
#41484=CARTESIAN_POINT ( 'NONE',  ( 12.38845540937129996, 1427.144650814109809, 206.9724466152189848 ) ) ;
#41487=B_SPLINE_CURVE_WITH_KNOTS ( 'NONE', 3,
 ( #108115, #66158, #29761, #98065, #65034, #21336, #64500, #57201, #89666, #90205, #13489, #90768, #14048, #12952, #46595, #14608, #91325, #80730, #72884, #107022, #47679, #48238, #81808, #108675, #5109, #39824, #39264, #73438, #107573, #82379, #5679, #48797, #82919, #20797, #54999, #89122, #12411, #54048, #4167, #106608, #29892, #20387, #54590, #38845, #36660, #97118, #89810, #22020, #72478 ),
 .UNSPECIFIED., .F., .F.,
 ( 4, 3, 3, 3, 3, 3, 3, 3, 3, 3, 3, 3, 3, 3, 3, 3, 4 ),
 ( -12.57626448940000152, -12.52235396050270033, -12.19521703350000053, -11.85293761877430008, -11.51065820404859963, -11.17664517332659990, -10.83712121993539945, -10.49485907924760042, -10.14901485447220075, -9.802596852533810079, -9.456470061949168837, -9.112590635329999245, -8.869360225144090393, -8.533531448524120933, -8.201658424667050085, -7.872532270376759733, -7.548593288820000247 ),
 .UNSPECIFIED. ) ;
#41491=CARTESIAN_POINT ( 'NONE',  ( 3.195005116169999937, 1472.592485613090048, 218.8132852216689912 ) ) ;
#41494=CARTESIAN_POINT ( 'NONE',  ( -5.202920349680000278, 1495.777356229890074, 199.0561181787990108 ) ) ;
#41499=CARTESIAN_POINT ( 'NONE',  ( 5.037981958419999629, 1447.001160774289929, 201.0441824198890117 ) ) ;
#41502=CARTESIAN_POINT ( 'NONE',  ( -2.039871424690000268, 1455.397043516590202, 199.5224340987989819 ) ) ;
#41510=CARTESIAN_POINT ( 'NONE',  ( -17.54273015099310129, 1417.931783278020021, 206.8684746656099946 ) ) ;
#41520=B_SPLINE_CURVE_WITH_KNOTS ( 'NONE', 3,
 ( #87422, #19079, #53283, #62811, #20194, #27502, #1221, #79039, #103664, #79581, #86860, #26962, #2885, #10718, #2340, #37004, #80112, #86309, #44889, #71196, #104215, #28052, #43763, #88525, #95267, #96368, #36453 ),
 .UNSPECIFIED., .F., .F.,
 ( 4, 2, 2, 1, 1, 1, 2, 2, 2, 2, 1, 1, 2, 2, 2, 4 ),
 ( 0.000000000000000000, 0.1250000000031543101, 0.1875000000047308546, 0.2187500000055191129, 0.2343750000059132421, 0.2421875000061094463, 0.2460937500061190775, 0.2500000000061286531, 0.3750000000060828564, 0.4375000000060604854, 0.4687500000059777738, 0.4843750000059379168, 0.4921875000059188765, 0.5000000000058997252, 0.7500000000029501956, 1.000000000000000000 ),
 .UNSPECIFIED. ) ;
#41525=CARTESIAN_POINT ( 'NONE',  ( 4.976599076821749179, 1508.551704408389924, 211.8383979467219831 ) ) ;
#41528=CARTESIAN_POINT ( 'NONE',  ( -18.65942339678869999, 1468.219813745079819, 201.0822072839200132 ) ) ;
#41533=CARTESIAN_POINT ( 'NONE',  ( 10.54167417284469899, 1452.797503886009963, 210.1255431293710103 ) ) ;
#41535=CARTESIAN_POINT ( 'NONE',  ( -13.59448361969050012, 1507.983769305739997, 209.3963040809830147 ) ) ;
#41537=CARTESIAN_POINT ( 'NONE',  ( 4.328507300020000059, 1515.100746401290053, 210.1973568915390160 ) ) ;
#41540=CARTESIAN_POINT ( 'NONE',  ( -20.06562366400000030, 1485.934169092390221, 214.0282076738189971 ) ) ;
#41541=FACE_OUTER_BOUND ( 'NONE', #53521, .T. ) ;
#41543=CARTESIAN_POINT ( 'NONE',  ( -3.263114576272079827E-31, 1414.677402202029953, 209.1218459616989946 ) ) ;
#41559=CARTESIAN_POINT ( 'NONE',  ( 11.09419342938610065, 1470.256789811390036, 206.9270417508720072 ) ) ;
#41560=CARTESIAN_POINT ( 'NONE',  ( -9.644458973949999958, 1472.935586159989953, 205.1723540604189964 ) ) ;
#41570=EDGE_CURVE ( 'NONE', #38120, #63746, #44388, .T. ) ;
#41575=CARTESIAN_POINT ( 'NONE',  ( -3.984081752359151185, 1515.551704408386286, 211.4519800883278720 ) ) ;
#41576=EDGE_LOOP ( 'NONE', ( #4872, #110779, #20724, #90614 ) ) ;
#41578=CARTESIAN_POINT ( 'NONE',  ( -0.3843944283460010158, 1508.551705141689808, 220.3095046180989698 ) ) ;
#41582=CARTESIAN_POINT ( 'NONE',  ( 2.670692781143860106, 1446.036047624690127, 199.3704865114669929 ) ) ;
#41584=CARTESIAN_POINT ( 'NONE',  ( 8.024292235439999033, 1501.827778037190001, 207.2343894779990023 ) ) ;
#41585=CARTESIAN_POINT ( 'NONE',  ( 6.420990609280000427, 1480.020290046689979, 205.1468653125089929 ) ) ;
#41587=CARTESIAN_POINT ( 'NONE',  ( -16.38166793929999798, 1503.850271706589865, 209.2715074860340110 ) ) ;
#41594=DIRECTION ( 'NONE',  ( 1.224646799147350002E-16, -1.836970198721029688E-16, -1.000000000000000000 ) ) ;
#41595=CARTESIAN_POINT ( 'NONE',  ( 3.261561639834900106, 1454.263685100609791, 217.9259794001679893 ) ) ;
#41599=CARTESIAN_POINT ( 'NONE',  ( -14.75778373319999837, 1417.788090000929969, 203.2704188695489904 ) ) ;
#41606=CARTESIAN_POINT ( 'NONE',  ( 10.48718144549209974, 1482.007409792639919, 210.6586160354689810 ) ) ;
#41607=CARTESIAN_POINT ( 'NONE',  ( -12.16253670259992070, 1419.838831626010915, 197.2883662463995336 ) ) ;
#41616=CARTESIAN_POINT ( 'NONE',  ( 4.290508147089998836, 1515.379315998089851, 209.1218459616989946 ) ) ;
#41621=CARTESIAN_POINT ( 'NONE',  ( 10.23616613091340000, 1480.714510420149963, 206.5818171423960052 ) ) ;
#41623=CARTESIAN_POINT ( 'NONE',  ( 11.87053796280000029, 1436.297149115689990, 225.5644864776990062 ) ) ;
#41625=CARTESIAN_POINT ( 'NONE',  ( 11.69994065948550066, 1435.514598502499894, 225.6365353821880149 ) ) ;
#41630=CARTESIAN_POINT ( 'NONE',  ( 0.000000000000000000, 1391.913060387289988, 209.1218459616989946 ) ) ;
#41631=CARTESIAN_POINT ( 'NONE',  ( 10.29623711278930109, 1451.524458584259946, 207.0169742271000075 ) ) ;
#41634=CARTESIAN_POINT ( 'NONE',  ( -18.89253556303020076, 1486.193265656730091, 200.5306675107350145 ) ) ;
#41646=CARTESIAN_POINT ( 'NONE',  ( -8.796782887879999180, 1468.013265501289879, 190.7844261045989640 ) ) ;
#41648=CARTESIAN_POINT ( 'NONE',  ( -4.678155166858989134, 1508.611350403214146, 211.6097810837688087 ) ) ;
#41649=CARTESIAN_POINT ( 'NONE',  ( -0.5456026930049990842, 1443.714663396890046, 200.0731752116790005 ) ) ;
#41655=CARTESIAN_POINT ( 'NONE',  ( 0.5086982348340010063, 1417.713718843059951, 204.0301964970090012 ) ) ;
#41661=VERTEX_POINT ( 'NONE', #53343 ) ;
#41663=ORIENTED_EDGE ( 'NONE', *, *, #49160, .T. ) ;
#41669=CARTESIAN_POINT ( 'NONE',  ( -19.83859993069999916, 1467.194195006989958, 209.1218459616989946 ) ) ;
#41671=CARTESIAN_POINT ( 'NONE',  ( -13.08802352330000041, 1503.233211745590097, 208.6735908916250253 ) ) ;
#41678=DIRECTION ( 'NONE',  ( -0.02616798426500965835, 0.9993150019883683122, 0.02616798426500950916 ) ) ;
#41686=CARTESIAN_POINT ( 'NONE',  ( 1.779428963082609894, 1456.357349037730046, 198.6855221610310309 ) ) ;
#41697=EDGE_LOOP ( 'NONE', ( #29287, #110791, #76773, #791 ) ) ;
#41701=CARTESIAN_POINT ( 'NONE',  ( 0.9020232525101885557, 1494.156807207756856, 220.2151267746179713 ) ) ;
#41703=CARTESIAN_POINT ( 'NONE',  ( 11.26795897200000063, 1422.300791247489997, 207.0941861644789981 ) ) ;
#41707=CARTESIAN_POINT ( 'NONE',  ( -9.901291130804080964, 1447.905280604810059, 209.8165545639580216 ) ) ;
#41716=CARTESIAN_POINT ( 'NONE',  ( 4.156019621739999614, 1466.560893159090028, 218.5576475902890081 ) ) ;
#41729=CARTESIAN_POINT ( 'NONE',  ( 5.008389395533990651, 1455.723473645530021, 218.4926572036009986 ) ) ;
#41730=B_SPLINE_CURVE_WITH_KNOTS ( 'NONE', 5,
 ( #56570, #13987, #48174, #73923, #57135, #108052 ),
 .UNSPECIFIED., .F., .F.,
 ( 6, 6 ),
 ( 176.6690472260000035, 181.4923368590000052 ),
 .UNSPECIFIED. ) ;
#41731=CARTESIAN_POINT ( 'NONE',  ( 545.1437632904659267, 11220.04953453919370, 2113.080198834563362 ) ) ;
#41735=CARTESIAN_POINT ( 'NONE',  ( -8.803830034714509978, 1437.965405572629834, 209.7008996341119769 ) ) ;
#41736=CARTESIAN_POINT ( 'NONE',  ( -4.329415281104970425, 1515.068899390480283, 212.0799436200479704 ) ) ;
#41739=CARTESIAN_POINT ( 'NONE',  ( 2.330134126090000368, 1515.551704408389924, 212.9514660752490158 ) ) ;
#41741=FACE_OUTER_BOUND ( 'NONE', #52307, .T. ) ;
#41742=ORIENTED_EDGE ( 'NONE', *, *, #62736, .T. ) ;
#41744=CARTESIAN_POINT ( 'NONE',  ( 5.312679136500000787, 1493.059131431590231, 218.8466398904690209 ) ) ;
#41746=ORIENTED_EDGE ( 'NONE', *, *, #79772, .T. ) ;
#41749=CARTESIAN_POINT ( 'NONE',  ( 4.441317194709999860, 1455.879597309289920, 218.7824459606689800 ) ) ;
#41751=CARTESIAN_POINT ( 'NONE',  ( -8.166278650529999794, 1445.984953112289986, 214.8591734898389802 ) ) ;
#41755=CARTESIAN_POINT ( 'NONE',  ( 7.705241972949999685, 1423.949153165739972, 212.4347587744790076 ) ) ;
#41758=CARTESIAN_POINT ( 'NONE',  ( 2.059290213318034191, 1495.373074823845400, 220.5469163244703168 ) ) ;
#41772=EDGE_CURVE ( 'NONE', #777, #8596, #110266, .T. ) ;
#41778=CARTESIAN_POINT ( 'NONE',  ( -8.706652659834380970, 1448.779525635259915, 211.9411403000989935 ) ) ;
#41798=B_SPLINE_CURVE_WITH_KNOTS ( 'NONE', 3,
 ( #26388, #19076, #45976, #17979, #86857, #52174, #45434, #2882, #10149, #86305, #37001, #61149, #71193, #95264, #105315, #9589 ),
 .UNSPECIFIED., .F., .F.,
 ( 4, 3, 3, 3, 3, 4 ),
 ( -48.30090647720000163, -47.55390437728789976, -46.79923191349099909, -45.99756063279310325, -45.16082034306089810, -44.26078367470000074 ),
 .UNSPECIFIED. ) ;
#41801=VERTEX_POINT ( 'NONE', #77423 ) ;
#41819=CARTESIAN_POINT ( 'NONE',  ( -10.84042494649999888, 1471.406554747690052, 207.3881111542589792 ) ) ;
#41822=DIRECTION ( 'NONE',  ( 0.000000000000000000, -1.836970198721029688E-16, -1.000000000000000000 ) ) ;
#41826=CARTESIAN_POINT ( 'NONE',  ( -12.25020723839999981, 1415.706272599410113, 207.6119962243290331 ) ) ;
#41829=CARTESIAN_POINT ( 'NONE',  ( 8.654318022629999163, 1488.600155993789940, 202.1361091811689903 ) ) ;
#41838=B_SPLINE_SURFACE_WITH_KNOTS ( 'NONE', 5, 1, ( 
 ( #104603, #30648 ),
 ( #14926, #92749 ),
 ( #15476, #107352 ),
 ( #73774, #56414 ),
 ( #109020, #64834 ),
 ( #73208, #23336 ),
 ( #98941, #31740 ),
 ( #48007, #58071 ),
 ( #100048, #83803 ) ),
 .UNSPECIFIED., .F., .F., .F.,
 ( 6, 3, 6 ),
 ( 2, 2 ),
 ( 0.000000000000000000, 8.685334524039999948, 17.34448624229999680 ),
 ( 0.000000000000000000, 14.00000434508570102 ),
 .UNSPECIFIED. ) ;
#41839=CARTESIAN_POINT ( 'NONE',  ( -16.95087640679999907, 1420.353012175349932, 203.7180132809789939 ) ) ;
#41840=CARTESIAN_POINT ( 'NONE',  ( -16.32163182381450284, 1508.551704408389924, 213.4489841974129831 ) ) ;
#41842=B_SPLINE_CURVE_WITH_KNOTS ( 'NONE', 5,
 ( #65302, #72592, #40077, #6477, #90473, #99413, #98323, #56341, #46854 ),
 .UNSPECIFIED., .F., .F.,
 ( 6, 3, 6 ),
 ( -3.000000000000000000, -1.500000000000000000, 0.000000000000000000 ),
 .UNSPECIFIED. ) ;
#41843=CARTESIAN_POINT ( 'NONE',  ( 0.5456170147259989944, 1474.667248827789990, 219.7869908219989838 ) ) ;
#41845=CARTESIAN_POINT ( 'NONE',  ( -0.8583877449824180994, 1423.306587861139860, 191.2160083861890030 ) ) ;
#41849=CARTESIAN_POINT ( 'NONE',  ( 12.03449227190490056, 1491.353386486839781, 206.6667661091970274 ) ) ;
#41851=CARTESIAN_POINT ( 'NONE',  ( -7.233408913757819469, 1421.233011291230014, 193.8023897524950030 ) ) ;
#41866=CARTESIAN_POINT ( 'NONE',  ( -4.326992699839999901, 1515.158586648489973, 208.7650084369950036 ) ) ;
#41871=CARTESIAN_POINT ( 'NONE',  ( 11.84335401826939993, 1492.196273574100132, 210.1769102818510078 ) ) ;
#41872=CARTESIAN_POINT ( 'NONE',  ( -1.221315768609999797, 1455.568494079489938, 218.5163151374690074 ) ) ;
#41873=ORIENTED_EDGE ( 'NONE', *, *, #82403, .T. ) ;
#41877=CARTESIAN_POINT ( 'NONE',  ( 4.932890325442090607, 1508.551704408389924, 206.1093674645129852 ) ) ;
#41878=VERTEX_POINT ( 'NONE', #80180 ) ;
#41881=CARTESIAN_POINT ( 'NONE',  ( -21.51339057090000040, 1505.551704408389924, 209.1218459616989946 ) ) ;
#41886=CARTESIAN_POINT ( 'NONE',  ( 11.77194447489770113, 1479.596685624299880, 209.5331444464590049 ) ) ;
#41888=CARTESIAN_POINT ( 'NONE',  ( -2.559284476340000225, 1448.316302177390071, 190.2468044718989972 ) ) ;
#41894=CARTESIAN_POINT ( 'NONE',  ( 1.282357359580419853, 1486.462675952139989, 197.2709641886989971 ) ) ;
#41895=CARTESIAN_POINT ( 'NONE',  ( 2.796706406386159749, 1431.643787548970067, 200.3851250015239884 ) ) ;
#41901=B_SPLINE_SURFACE_WITH_KNOTS ( 'NONE', 5, 5, ( 
 ( #561, #58255, #17301, #77262, #67759, #109210 ),
 ( #102432, #92375, #15647, #66666, #51496, #6725 ),
 ( #58797, #23523, #25163, #25716, #16208, #76145 ),
 ( #93477, #8929, #50412, #91833, #84537, #49853 ),
 ( #83986, #40881, #16748, #85079, #7285, #7826 ),
 ( #32494, #34687, #41448, #57717, #42539, #4 ),
 ( #59367, #101872, #75613, #41996, #109744, #33025 ),
 ( #101311, #34138, #67214, #110290, #33567, #59917 ),
 ( #8370, #85628, #18971, #11167, #87877, #52061 ),
 ( #10040, #36897, #60465, #96821, #78355, #18414 ),
 ( #61572, #61033, #1113, #27391, #45874, #95705 ),
 ( #53166, #62133, #43652, #105215, #69428, #70537 ) ),
 .UNSPECIFIED., .F., .F., .F.,
 ( 6, 3, 3, 6 ),
 ( 6, 6 ),
 ( -7.850178216250999828E-05, 7.062844993700000629, 14.12568998740000126, 17.37861058108219936 ),
 ( 0.000000000000000000, 2.000078501782160068 ),
 .UNSPECIFIED. ) ;
#41902=CARTESIAN_POINT ( 'NONE',  ( -18.31738235171379969, 1464.474234536650101, 217.5285399418669954 ) ) ;
#41907=CARTESIAN_POINT ( 'NONE',  ( -6.848531018220000099, 1473.608249816489888, 207.2687511549490011 ) ) ;
#41910=CARTESIAN_POINT ( 'NONE',  ( -3.829620113550000315, 1515.551704408389924, 211.2083941403789993 ) ) ;
#41913=CARTESIAN_POINT ( 'NONE',  ( -3.151260259420000320, 1476.308151181189942, 199.2625566838590032 ) ) ;
#41918=CARTESIAN_POINT ( 'NONE',  ( 1.316738241441249846, 1429.477911528270170, 217.3230272967620067 ) ) ;
#41919=CARTESIAN_POINT ( 'NONE',  ( -8.016638155169999891, 1425.903768209389909, 207.5828447795889815 ) ) ;
#41925=CARTESIAN_POINT ( 'NONE',  ( 7.535336306764500058, 1425.758512211720017, 212.2082866544780018 ) ) ;
#41933=CARTESIAN_POINT ( 'NONE',  ( -3.018087336003992593, 1475.315668037541400, 198.8202750044643778 ) ) ;
#41936=CARTESIAN_POINT ( 'NONE',  ( 18.03426301339999682, 1429.185447070490000, 206.6153916553589909 ) ) ;
#41941=ORIENTED_EDGE ( 'NONE', *, *, #67477, .F. ) ;
#41958=CARTESIAN_POINT ( 'NONE',  ( 0.1765913036374869849, 1444.932331911239999, 199.0604220796319908 ) ) ;
#41960=ORIENTED_EDGE ( 'NONE', *, *, #82403, .F. ) ;
#41962=CARTESIAN_POINT ( 'NONE',  ( 1.964958540781392982, 1433.107491112560638, 200.8576305902842023 ) ) ;
#41963=DIRECTION ( 'NONE',  ( -1.000000000000000000, 0.000000000000000000, 0.000000000000000000 ) ) ;
#41965=CARTESIAN_POINT ( 'NONE',  ( 7.803888876470000291, 1421.636253146019953, 195.8400330162989746 ) ) ;
#41966=CARTESIAN_POINT ( 'NONE',  ( 0.08322839651420729790, 1431.805008108389984, 218.6146693997570196 ) ) ;
#41968=CARTESIAN_POINT ( 'NONE',  ( -4.522294835890000364, 1496.991527996390232, 198.8128890079989901 ) ) ;
#41975=VECTOR ( 'NONE', #77387, 1000.000000000000000 ) ;
#41977=ORIENTED_EDGE ( 'NONE', *, *, #16871, .F. ) ;
#41981=CARTESIAN_POINT ( 'NONE',  ( -10.61669498371649922, 1508.551704408389924, 207.6874897006059939 ) ) ;
#41985=CARTESIAN_POINT ( 'NONE',  ( 9.216942500360310930, 1427.824353572689915, 211.8045479288090007 ) ) ;
#41986=CARTESIAN_POINT ( 'NONE',  ( 11.11191080231209938, 1422.810623797719927, 203.3290056078989778 ) ) ;
#41987=CARTESIAN_POINT ( 'NONE',  ( -10.90301725406700051, 1462.753400739099789, 207.3092048343249871 ) ) ;
#41992=B_SPLINE_SURFACE_WITH_KNOTS ( 'NONE', 5, 5, ( 
 ( #34000, #16075, #9904, #102297, #84940, #103391 ),
 ( #44073, #68193, #59775, #50278, #85488, #16613 ),
 ( #84407, #76554, #109614, #25582, #7694, #41851 ),
 ( #42401, #93896, #17161, #94441, #69286, #77667 ),
 ( #18289, #42969, #101741, #17720, #77128, #67627 ),
 ( #110710, #51354, #76006, #434, #50810, #32887 ),
 ( #110160, #25029, #34553, #68736, #52482, #59231 ),
 ( #102840, #86610, #26134, #60323, #51922, #67081 ),
 ( #86065, #101184, #980, #35104, #26697, #97767 ) ),
 .UNSPECIFIED., .F., .F., .F.,
 ( 6, 3, 6 ),
 ( 6, 6 ),
 ( 15.02943005950050015, 30.78174686530000059, 37.58808827629950144 ),
 ( -1.629659945966520018E-05, 2.000000000000000000 ),
 .UNSPECIFIED. ) ;
#41993=CARTESIAN_POINT ( 'NONE',  ( -9.670053538248419400, 1461.149818306590078, 208.5229399444750129 ) ) ;
#41996=CARTESIAN_POINT ( 'NONE',  ( 8.997196703874418944, 1463.834352910819916, 214.0592121972250084 ) ) ;
#41997=ADVANCED_FACE ( 'NONE', ( #95055 ), #76047, .F. ) ;
#41998=CARTESIAN_POINT ( 'NONE',  ( 8.800000000000002487, 1413.913060387329779, 209.1218459616989946 ) ) ;
#42005=CARTESIAN_POINT ( 'NONE',  ( -21.26810763296740348, 1485.919194788800041, 201.7808564414550290 ) ) ;
#42007=CARTESIAN_POINT ( 'NONE',  ( -21.07255583944779787, 1418.159754048780087, 208.6257934781920085 ) ) ;
#42020=CARTESIAN_POINT ( 'NONE',  ( 10.10955624819999876, 1478.902419763290027, 204.8960363941690161 ) ) ;
#42024=CARTESIAN_POINT ( 'NONE',  ( -8.694328787849268991, 1436.795955225099988, 213.8530210085260137 ) ) ;
#42030=CARTESIAN_POINT ( 'NONE',  ( 11.54915390828909949, 1427.568721002570101, 209.3630650540049771 ) ) ;
#42035=VERTEX_POINT ( 'NONE', #101772 ) ;
#42036=CARTESIAN_POINT ( 'NONE',  ( 1.396945621630000023, 1473.097535868490013, 219.2356281688989839 ) ) ;
#42039=CARTESIAN_POINT ( 'NONE',  ( -10.84952760220000023, 1492.388833904489957, 203.1614253636989815 ) ) ;
#42040=EDGE_CURVE ( 'NONE', #15017, #37845, #75594, .T. ) ;
#42044=CARTESIAN_POINT ( 'NONE',  ( 8.814478973669999107, 1449.891423584090035, 204.2733476837790079 ) ) ;
#42045=CARTESIAN_POINT ( 'NONE',  ( -21.13674105400000158, 1506.830501455790227, 213.5414170319390053 ) ) ;
#42046=ADVANCED_FACE ( 'NONE', ( #25063 ), #72297, .T. ) ;
#42048=CARTESIAN_POINT ( 'NONE',  ( -2.642610841670000266, 1455.978071948890147, 200.0212207443690033 ) ) ;
#42058=CARTESIAN_POINT ( 'NONE',  ( -17.47050761057940349, 1417.655283096519952, 206.4347063045530035 ) ) ;
#42059=ORIENTED_EDGE ( 'NONE', *, *, #72193, .F. ) ;
#42068=B_SPLINE_SURFACE_WITH_KNOTS ( 'NONE', 5, 5, ( 
 ( #85287, #25928, #51720, #60126, #769, #34898 ),
 ( #69644, #59020, #69086, #103187, #1315, #67429 ),
 ( #8587, #18631, #103767, #26490, #93147, #25374 ),
 ( #16415, #94811, #18087, #102092, #95368, #59566 ),
 ( #52828, #50608, #16959, #51160, #80220, #37661 ),
 ( #44425, #36558, #89165, #11373, #19175, #11912 ),
 ( #21378, #36020, #37109, #71310, #28157, #97570 ),
 ( #3538, #53951, #80772, #12456, #20842, #45544 ),
 ( #71867, #1883, #10249, #88085, #88633, #79684 ) ),
 .UNSPECIFIED., .F., .F., .F.,
 ( 6, 3, 6 ),
 ( 6, 6 ),
 ( 2.894173653929999812, 6.772837685190000734, 11.90357780880000149 ),
 ( 0.000000000000000000, 2.000000000000000000 ),
 .UNSPECIFIED. ) ;
#42073=CARTESIAN_POINT ( 'NONE',  ( 3.425924819994940140, 1508.551704408389924, 213.9259735013179977 ) ) ;
#42082=CARTESIAN_POINT ( 'NONE',  ( 10.17590696771870107, 1453.471716470849969, 212.1423554297430201 ) ) ;
#42084=CARTESIAN_POINT ( 'NONE',  ( -12.00127168876410444, 1417.517758714561751, 199.4623453708297518 ) ) ;
#42086=CARTESIAN_POINT ( 'NONE',  ( 4.138993620949999119, 1515.551749212189861, 209.4962163748910200 ) ) ;
#42087=CARTESIAN_POINT ( 'NONE',  ( -6.445381995435790046, 1454.081129442119845, 202.3077001288629901 ) ) ;
#42103=CARTESIAN_POINT ( 'NONE',  ( -8.341276443498419013, 1436.001163936675994, 211.2993112092940180 ) ) ;
#42105=CARTESIAN_POINT ( 'NONE',  ( -3.505398281758470791, 1488.737999217582001, 219.4357265464652755 ) ) ;
#42108=CARTESIAN_POINT ( 'NONE',  ( -10.52442967350000025, 1471.882653751090174, 205.8053291943989791 ) ) ;
#42113=CARTESIAN_POINT ( 'NONE',  ( 2.487935122070182192, 1508.611350403214601, 213.8000011285579092 ) ) ;
#42123=CARTESIAN_POINT ( 'NONE',  ( -11.38664936716510034, 1500.852607708580081, 211.0998368167220178 ) ) ;
#42126=CARTESIAN_POINT ( 'NONE',  ( -0.9795538395430010148, 1508.551704408389924, 220.0924926876990071 ) ) ;
#42134=CARTESIAN_POINT ( 'NONE',  ( -10.18972684899999948, 1478.941447477790007, 211.7723057433990164 ) ) ;
#42142=VECTOR ( 'NONE', #3531, 1000.000000000000227 ) ;
#42146=CARTESIAN_POINT ( 'NONE',  ( -15.77622222279999953, 1417.628996888570100, 204.9296672929689862 ) ) ;
#42151=CARTESIAN_POINT ( 'NONE',  ( -5.512326787969999309, 1497.963565169690128, 220.3136703888989985 ) ) ;
#42152=CARTESIAN_POINT ( 'NONE',  ( -3.681141709870000334, 1470.728927551090010, 189.4465201588989771 ) ) ;
#42153=CARTESIAN_POINT ( 'NONE',  ( -18.17365796220000007, 1441.208305948289762, 213.5442559039389891 ) ) ;
#42154=CARTESIAN_POINT ( 'NONE',  ( -11.96878399152000050, 1507.593741218769992, 208.5523078654620122 ) ) ;
#42155=FACE_OUTER_BOUND ( 'NONE', #6120, .T. ) ;
#42157=CARTESIAN_POINT ( 'NONE',  ( -18.26023438560000045, 1443.256148476890075, 213.5656046648789754 ) ) ;
#42164=CARTESIAN_POINT ( 'NONE',  ( 5.478408486960455903, 1471.900903316932499, 217.7034505013053547 ) ) ;
#42169=ADVANCED_FACE ( 'NONE', ( #14335 ), #57483, .T. ) ;
#42170=CARTESIAN_POINT ( 'NONE',  ( 4.955221929980000439, 1484.956700206389996, 218.7828209749189909 ) ) ;
#42172=EDGE_CURVE ( 'NONE', #100706, #2433, #67462, .T. ) ;
#42174=CARTESIAN_POINT ( 'NONE',  ( 20.38104524799999950, 1433.225738552389885, 214.6696956538789891 ) ) ;
#42177=LINE ( 'NONE', #18599, #35710 ) ;
#42181=CARTESIAN_POINT ( 'NONE',  ( 9.819515741042740942, 1435.473629839329988, 209.0286173952219997 ) ) ;
#42182=CARTESIAN_POINT ( 'NONE',  ( -14.51552834752570043, 1420.580226155020000, 213.2889873630980162 ) ) ;
#42183=CARTESIAN_POINT ( 'NONE',  ( 3.375977085881459949, 1446.395221913229989, 199.5681764770490076 ) ) ;
#42187=DIRECTION ( 'NONE',  ( 1.000000000000000000, 0.000000000000000000, 0.000000000000000000 ) ) ;
#42198=ORIENTED_EDGE ( 'NONE', *, *, #63062, .T. ) ;
#42201=CARTESIAN_POINT ( 'NONE',  ( 3.582837879391640001, 1515.224507406410112, 205.0446031332039922 ) ) ;
#42216=ORIENTED_EDGE ( 'NONE', *, *, #19715, .F. ) ;
#42221=CARTESIAN_POINT ( 'NONE',  ( -6.915889783819999970, 1473.238612257490104, 208.0311295836789895 ) ) ;
#42223=CARTESIAN_POINT ( 'NONE',  ( 11.84666127166159910, 1421.909629712770084, 209.1686410009280053 ) ) ;
#42229=VERTEX_POINT ( 'NONE', #98353 ) ;
#42236=CARTESIAN_POINT ( 'NONE',  ( -2.472546487080370170, 1422.360492482099744, 192.6709265187130029 ) ) ;
#42237=ORIENTED_EDGE ( 'NONE', *, *, #64081, .F. ) ;
#42244=CARTESIAN_POINT ( 'NONE',  ( -3.812371247207599900, 1428.459941768050157, 200.5740418269730014 ) ) ;
#42251=PLANE ( 'NONE',  #11762 ) ;
#42258=CARTESIAN_POINT ( 'NONE',  ( 10.46737760179999910, 1424.278704277569886, 206.5802270637989864 ) ) ;
#42259=CARTESIAN_POINT ( 'NONE',  ( -0.7183524226490148878, 1444.865767701265895, 218.0773563375222182 ) ) ;
#42260=CARTESIAN_POINT ( 'NONE',  ( -3.152270375085599596, 1474.954422185709745, 198.1306180807430053 ) ) ;
#42262=CARTESIAN_POINT ( 'NONE',  ( -9.161971811502120033, 1449.701013728480120, 209.8667376539109739 ) ) ;
#42271=CARTESIAN_POINT ( 'NONE',  ( 4.363541942640000393, 1466.192484605890058, 218.8344587469289877 ) ) ;
#42279=CARTESIAN_POINT ( 'NONE',  ( -9.901400372228881253, 1447.905338697959905, 209.8163239975949637 ) ) ;
#42281=CARTESIAN_POINT ( 'NONE',  ( -8.937053649178221093, 1440.468819487419978, 205.6155253440409751 ) ) ;
#42287=CARTESIAN_POINT ( 'NONE',  ( 12.13166762299999846, 1501.269883488590040, 211.0250359440489660 ) ) ;
#42289=CARTESIAN_POINT ( 'NONE',  ( 8.185066571180000139, 1426.771507121280138, 211.5403165378289714 ) ) ;
#42293=CARTESIAN_POINT ( 'NONE',  ( -7.542243412319999507, 1483.743633471490057, 200.8664480738789848 ) ) ;
#42301=CARTESIAN_POINT ( 'NONE',  ( 1.026847438530000156, 1494.050500594489904, 217.3813169704690154 ) ) ;
#42302=CARTESIAN_POINT ( 'NONE',  ( -14.79126394052620164, 1416.133454573002609, 204.7564966609269845 ) ) ;
#42305=CARTESIAN_POINT ( 'NONE',  ( -5.467724459860000330, 1444.780760362290039, 217.3521413719989823 ) ) ;
#42309=CARTESIAN_POINT ( 'NONE',  ( 7.578931200799999601, 1423.300307201199985, 213.4057882997690001 ) ) ;
#42323=CARTESIAN_POINT ( 'NONE',  ( 1.081335638410579891, 1415.752565153090018, 209.4296050402819844 ) ) ;
#42328=DIRECTION ( 'NONE',  ( 1.000000000000000000, 0.000000000000000000, 0.000000000000000000 ) ) ;
#42331=CARTESIAN_POINT ( 'NONE',  ( -9.909475446137518517, 1446.884018808590099, 211.9943844666950099 ) ) ;
#42337=ORIENTED_EDGE ( 'NONE', *, *, #69646, .F. ) ;
#42338=VERTEX_POINT ( 'NONE', #73163 ) ;
#42340=CARTESIAN_POINT ( 'NONE',  ( 7.487277797411009850, 1424.824108058459842, 194.2252290839009845 ) ) ;
#42357=CARTESIAN_POINT ( 'NONE',  ( -11.16953914610450127, 1480.956324501380095, 211.2841307982869807 ) ) ;
#42363=CARTESIAN_POINT ( 'NONE',  ( 9.586487508724173878, 1493.457082605286359, 189.9081600023157819 ) ) ;
#42371=CARTESIAN_POINT ( 'NONE',  ( -3.824657326589999684, 1429.713551423189983, 201.7356720059990209 ) ) ;
#42374=CARTESIAN_POINT ( 'NONE',  ( -14.61243671689999957, 1417.122520118429975, 205.5241932702090253 ) ) ;
#42376=CARTESIAN_POINT ( 'NONE',  ( 5.495445188540000636, 1487.154938902290041, 199.6385650399689951 ) ) ;
#42378=CARTESIAN_POINT ( 'NONE',  ( 10.49215161174419997, 1461.076717979740124, 208.4970850488610097 ) ) ;
#42384=ORIENTED_EDGE ( 'NONE', *, *, #17225, .F. ) ;
#42386=CARTESIAN_POINT ( 'NONE',  ( -16.79355118000000147, 1420.470915882059899, 203.2250788364389678 ) ) ;
#42387=ORIENTED_EDGE ( 'NONE', *, *, #90708, .F. ) ;
#42388=CARTESIAN_POINT ( 'NONE',  ( -18.28629418055740175, 1508.551704408389924, 210.6167475138960015 ) ) ;
#42392=CARTESIAN_POINT ( 'NONE',  ( -11.39446592756109844, 1470.674086296440009, 209.5209556861319982 ) ) ;
#42393=CARTESIAN_POINT ( 'NONE',  ( -4.249061451088596009, 1508.172007302874363, 220.6133281201646810 ) ) ;
#42397=CARTESIAN_POINT ( 'NONE',  ( -7.013461631340700997, 1458.033762489906394, 215.6076664431717802 ) ) ;
#42398=CARTESIAN_POINT ( 'NONE',  ( -9289.452348480423097, -2339.359351152911131, 1609.629554519071007 ) ) ;
#42400=EDGE_CURVE ( 'NONE', #18368, #288, #72993, .T. ) ;
#42401=CARTESIAN_POINT ( 'NONE',  ( -8.367456039295358750, 1418.839936894859875, 195.8971482936690052 ) ) ;
#42402=CARTESIAN_POINT ( 'NONE',  ( 4.327091944037150029, 1515.154796665620097, 208.8633048373430086 ) ) ;
#42410=CARTESIAN_POINT ( 'NONE',  ( 9.651066088509999474, 1425.440658930580184, 195.4941615409990163 ) ) ;
#42412=CARTESIAN_POINT ( 'NONE',  ( 10.29338229012589956, 1422.407096038270083, 211.7839187185859942 ) ) ;
#42413=CARTESIAN_POINT ( 'NONE',  ( -4.646147325060000277, 1378.399971913189802, 203.6922293430689876 ) ) ;
#42414=CARTESIAN_POINT ( 'NONE',  ( 18.38166433807079869, 1428.164289305379953, 201.4944191049719961 ) ) ;
#42418=CARTESIAN_POINT ( 'NONE',  ( 10.92074801238010018, 1490.510034778949830, 210.1931246329349960 ) ) ;
#42431=CARTESIAN_POINT ( 'NONE',  ( -9.467901848279998589, 1462.744805377290049, 205.1999451337790106 ) ) ;
#42439=CARTESIAN_POINT ( 'NONE',  ( 2.625463805309249832, 1431.952376572269941, 200.6791034752619964 ) ) ;
#42445=CARTESIAN_POINT ( 'NONE',  ( 5.021805632604219305, 1470.186357947040051, 187.8118227978269772 ) ) ;
#42446=CARTESIAN_POINT ( 'NONE',  ( -11.03352341481849841, 1462.446812322350070, 208.7213867630900097 ) ) ;
#42452=EDGE_CURVE ( 'NONE', #4789, #12462, #55831, .T. ) ;
#42454=CARTESIAN_POINT ( 'NONE',  ( 0.3867091632760010222, 1476.097381945789948, 198.0337097418990027 ) ) ;
#42459=CARTESIAN_POINT ( 'NONE',  ( 3.433134143449350084, 1428.624608639609960, 216.6434505333259892 ) ) ;
#42460=CARTESIAN_POINT ( 'NONE',  ( -2.858448621680000024, 1443.821599769190016, 199.4616741486989895 ) ) ;
#42465=CARTESIAN_POINT ( 'NONE',  ( -6.657935129248458317, 1470.951763472646689, 216.7381263951724293 ) ) ;
#42466=CARTESIAN_POINT ( 'NONE',  ( 7.485501385385199491, 1426.034470239760140, 212.3577792365530286 ) ) ;
#42474=CARTESIAN_POINT ( 'NONE',  ( -3.829620113550000315, 1515.551704408389924, 207.2788837304390199 ) ) ;
#42475=CARTESIAN_POINT ( 'NONE',  ( 17.68711869539999881, 1428.828027849089949, 204.9896315466789929 ) ) ;
#42476=CARTESIAN_POINT ( 'NONE',  ( 3.639548396805570185, 1468.126230336239814, 218.4317111027060037 ) ) ;
#42481=CARTESIAN_POINT ( 'NONE',  ( 2.487935123020000194, 1509.038615934189920, 204.6345961887290059 ) ) ;
#42483=VERTEX_POINT ( 'NONE', #99997 ) ;
#42487=CARTESIAN_POINT ( 'NONE',  ( -11.41709567969999917, 1481.865892882389971, 208.5947888571609781 ) ) ;
#42492=CARTESIAN_POINT ( 'NONE',  ( 3.865553273121640210, 1508.610338516509955, 213.5325911278659987 ) ) ;
#42503=CARTESIAN_POINT ( 'NONE',  ( 2.685817909462222985, 1433.387035614327488, 201.0472282066888283 ) ) ;
#42504=CARTESIAN_POINT ( 'NONE',  ( -2.885329902869700369, 1508.551704408389924, 214.0785756058540130 ) ) ;
#42506=CARTESIAN_POINT ( 'NONE',  ( 7.943378312860001067, 1421.399538177179920, 195.9193817166990073 ) ) ;
#42507=CARTESIAN_POINT ( 'NONE',  ( -3.008413779357860030, 1433.155062154890174, 218.1878497074879988 ) ) ;
#42508=CARTESIAN_POINT ( 'NONE',  ( -3.856935219870000431, 1496.767660296590066, 198.5573707464990036 ) ) ;
#42511=CARTESIAN_POINT ( 'NONE',  ( 4.019837106079773292, 1515.589591810383126, 209.7430514019713428 ) ) ;
#42520=CARTESIAN_POINT ( 'NONE',  ( -10.83363501528680040, 1483.150651703840140, 204.1787077859559929 ) ) ;
#42525=CARTESIAN_POINT ( 'NONE',  ( 10.27889274641360018, 1427.972273100049961, 211.4948331838920126 ) ) ;
#42528=ADVANCED_FACE ( 'NONE', ( #75193 ), #81212, .T. ) ;
#42529=CARTESIAN_POINT ( 'NONE',  ( -11.01785496395880060, 1462.531659345610024, 208.3487688801509989 ) ) ;
#42530=CARTESIAN_POINT ( 'NONE',  ( -1.073363620209200085E-15, 1380.371560387289946, 209.1218459616989946 ) ) ;
#42538=CARTESIAN_POINT ( 'NONE',  ( 11.39828671546239924, 1425.690482886019936, 199.4434797265739974 ) ) ;
#42539=CARTESIAN_POINT ( 'NONE',  ( 8.858323751961959758, 1463.855706633549971, 215.0058157969349679 ) ) ;
#42546=CARTESIAN_POINT ( 'NONE',  ( 0.5707576997041963196, 1477.813279947535420, 198.7217904697586448 ) ) ;
#42548=CARTESIAN_POINT ( 'NONE',  ( -1.471738374290000095, 1515.341568496189893, 204.8474131707589834 ) ) ;
#42550=CARTESIAN_POINT ( 'NONE',  ( -22.19117980480319829, 1483.602007368270051, 216.8115291794120196 ) ) ;
#42553=CARTESIAN_POINT ( 'NONE',  ( -20.54173704900959763, 1418.376418166659960, 208.6868407705159996 ) ) ;
#42556=VERTEX_POINT ( 'NONE', #102174 ) ;
#42563=CARTESIAN_POINT ( 'NONE',  ( -10.55952073400000124, 1471.180150010990019, 209.5617685337520015 ) ) ;
#42565=CARTESIAN_POINT ( 'NONE',  ( 9.959589143500000574, 1478.327753353190019, 203.6760996314889951 ) ) ;
#42567=CARTESIAN_POINT ( 'NONE',  ( 2.979994341136180225, 1507.572973720820073, 217.5187881045870029 ) ) ;
#42568=EDGE_CURVE ( 'NONE', #37624, #37252, #16744, .T. ) ;
#42569=CARTESIAN_POINT ( 'NONE',  ( -9.158906349748429321, 1437.718415169640139, 211.6837391772429839 ) ) ;
#42577=CARTESIAN_POINT ( 'NONE',  ( 11.09274063877570171, 1422.410694574019999, 207.6743043836530092 ) ) ;
#42584=CARTESIAN_POINT ( 'NONE',  ( 1.859895485220000033, 1474.627878747789964, 219.9708147289989881 ) ) ;
#42585=CARTESIAN_POINT ( 'NONE',  ( 1.842962231260000028, 1515.551704408389924, 205.2922258481490303 ) ) ;
#42587=CARTESIAN_POINT ( 'NONE',  ( -9.320710346250001166, 1493.328639440889901, 201.5612320172390071 ) ) ;
#42591=CARTESIAN_POINT ( 'NONE',  ( -1776.370103581280091, 5181.793945261120825, 9288.252068156898531 ) ) ;
#42592=CARTESIAN_POINT ( 'NONE',  ( 5.845238504180000128, 1446.767628288889910, 202.1062060431090117 ) ) ;
#42600=CARTESIAN_POINT ( 'NONE',  ( -0.9164389294989989665, 1497.287211993289930, 197.7316609878989766 ) ) ;
#42602=CARTESIAN_POINT ( 'NONE',  ( 1.265340693600000233, 1494.980160179489758, 220.3616726747989958 ) ) ;
#42617=CARTESIAN_POINT ( 'NONE',  ( 12.70147564075329960, 1500.571916961849865, 209.2764580048830112 ) ) ;
#42619=CARTESIAN_POINT ( 'NONE',  ( -5.146359508130000648, 1391.913486340589998, 214.6520581086589914 ) ) ;
#42623=CARTESIAN_POINT ( 'NONE',  ( 9.387379239281479215, 1461.645186388049979, 206.6211749101620114 ) ) ;
#42625=EDGE_LOOP ( 'NONE', ( #61141, #100371, #47158, #45235, #83306, #87785 ) ) ;
#42627=CARTESIAN_POINT ( 'NONE',  ( -3.076366055149999834, 1424.853903601579987, 191.3970713258989917 ) ) ;
#42629=EDGE_CURVE ( 'NONE', #12135, #35462, #74255, .T. ) ;
#42632=CARTESIAN_POINT ( 'NONE',  ( -15.30723763684610006, 1508.551704406429963, 210.0839430030410142 ) ) ;
#42633=CARTESIAN_POINT ( 'NONE',  ( 4.175275161990000150, 1515.456650324490056, 210.6054913326990174 ) ) ;
#42635=CARTESIAN_POINT ( 'NONE',  ( 12.40160258794860049, 1420.584110727309962, 200.5244627772079866 ) ) ;
#42637=CARTESIAN_POINT ( 'NONE',  ( 9.176106830921559876, 1450.535193219119947, 208.1385774281999943 ) ) ;
#42651=CARTESIAN_POINT ( 'NONE',  ( -10.15064982388159898, 1462.077207233110130, 208.4365470241570222 ) ) ;
#42655=CARTESIAN_POINT ( 'NONE',  ( -9.950505953960002259, 1472.615817291290114, 206.1541412670590034 ) ) ;
#42656=CARTESIAN_POINT ( 'NONE',  ( 6.128601823160000350, 1493.316819573389921, 218.4060617982489987 ) ) ;
#42660=CARTESIAN_POINT ( 'NONE',  ( 3.844278957675350217, 1466.491520180780071, 198.7404678004429854 ) ) ;
#42663=ORIENTED_EDGE ( 'NONE', *, *, #81097, .T. ) ;
#42669=CARTESIAN_POINT ( 'NONE',  ( -1.842963219480119985, 1515.064792700640055, 204.7923971808919816 ) ) ;
#42675=CARTESIAN_POINT ( 'NONE',  ( 19.79299573329999617, 1474.475016451189958, 213.0583662838989767 ) ) ;
#42680=EDGE_CURVE ( 'NONE', #18354, #5861, #78334, .T. ) ;
#42682=CARTESIAN_POINT ( 'NONE',  ( -11.74755037768770016, 1482.417789575780262, 207.1586782760400069 ) ) ;
#42683=CARTESIAN_POINT ( 'NONE',  ( 6.826200034800000260, 1424.874072630889941, 213.4902541782590220 ) ) ;
#42685=ORIENTED_EDGE ( 'NONE', *, *, #31314, .T. ) ;
#42699=CARTESIAN_POINT ( 'NONE',  ( -15.34446697350000122, 1417.328256708470008, 204.9827898744490255 ) ) ;
#42701=CARTESIAN_POINT ( 'NONE',  ( -3.362747762569299859, 1485.356940126880090, 197.7060954189079780 ) ) ;
#42702=CARTESIAN_POINT ( 'NONE',  ( -16.04213126322901672, 1419.787388156080397, 210.3004129104147637 ) ) ;
#42704=EDGE_LOOP ( 'NONE', ( #45839, #29010, #28907, #18380 ) ) ;
#42708=CARTESIAN_POINT ( 'NONE',  ( -11.54256419585919957, 1508.172464970640021, 207.9362749538369997 ) ) ;
#42714=ADVANCED_FACE ( 'NONE', ( #24761 ), #13263, .T. ) ;
#42720=CARTESIAN_POINT ( 'NONE',  ( 9.549000552458089430, 1470.075890067440014, 212.3436661921319910 ) ) ;
#42721=CARTESIAN_POINT ( 'NONE',  ( -2.360319324342201153, 1507.471933479789868, 221.3436898553985941 ) ) ;
#42724=CARTESIAN_POINT ( 'NONE',  ( 3.323702338719999982, 1484.956220939089917, 220.0842284974989695 ) ) ;
#42727=CARTESIAN_POINT ( 'NONE',  ( -19.86559622680790227, 1442.607244639209966, 212.9307904419119950 ) ) ;
#42735=CARTESIAN_POINT ( 'NONE',  ( 9.027641301329820678, 1449.985334637959795, 203.9681922101850091 ) ) ;
#42750=CARTESIAN_POINT ( 'NONE',  ( -10.22594067180810029, 1448.813191590999850, 207.3202860899079951 ) ) ;
#42761=CARTESIAN_POINT ( 'NONE',  ( 11.76014171143800091, 1479.338753478690023, 208.6264959333659874 ) ) ;
#42772=FACE_OUTER_BOUND ( 'NONE', #83203, .T. ) ;
#42773=CARTESIAN_POINT ( 'NONE',  ( -19.27355791249999939, 1467.813399981289876, 204.3088842694490097 ) ) ;
#42785=ORIENTED_EDGE ( 'NONE', *, *, #62736, .F. ) ;
#42788=CARTESIAN_POINT ( 'NONE',  ( 0.7166837575268250049, 1423.109731908320100, 192.5084507060149974 ) ) ;
#42791=CARTESIAN_POINT ( 'NONE',  ( -15.44253390423740058, 1508.551704408389924, 210.3695883813369960 ) ) ;
#42798=CARTESIAN_POINT ( 'NONE',  ( -2.831928916266819751, 1429.014365125550057, 200.1906073963359916 ) ) ;
#42802=CARTESIAN_POINT ( 'NONE',  ( -11.71534935561269819, 1482.452763970830119, 207.0198387685339867 ) ) ;
#42810=CARTESIAN_POINT ( 'NONE',  ( -3.703568358935259930, 1497.311626042180023, 220.9591690318370070 ) ) ;
#42813=CARTESIAN_POINT ( 'NONE',  ( -5.721601866879999498, 1461.879722082089756, 205.5653134029390117 ) ) ;
#42817=CARTESIAN_POINT ( 'NONE',  ( -9.905565548761760652, 1448.662754155020139, 208.1208174031709746 ) ) ;
#42819=ORIENTED_EDGE ( 'NONE', *, *, #110287, .T. ) ;
#42823=TOROIDAL_SURFACE ( 'NONE', #60754, 10.71315034250000053, 1.000000000000000000 ) ;
#42824=EDGE_CURVE ( 'NONE', #96418, #11469, #54183, .T. ) ;
#42827=CARTESIAN_POINT ( 'NONE',  ( -19.83859993069999916, 1467.194195006989958, 209.1218459616989946 ) ) ;
#42828=CARTESIAN_POINT ( 'NONE',  ( 2.093054630779237257, 1468.720840884834388, 218.9195178419581396 ) ) ;
#42832=CARTESIAN_POINT ( 'NONE',  ( -2.127754871950000126, 1429.399568160389890, 199.9814804629589844 ) ) ;
#42834=CARTESIAN_POINT ( 'NONE',  ( 11.26319909285720122, 1480.121028330829859, 210.5495473590729887 ) ) ;
#42849=CARTESIAN_POINT ( 'NONE',  ( 10.41177329615350011, 1460.024665156439823, 205.9063136364349873 ) ) ;
#42852=FACE_BOUND ( 'NONE', #34906, .T. ) ;
#42858=EDGE_CURVE ( 'NONE', #91618, #106043, #63515, .T. ) ;
#42864=CARTESIAN_POINT ( 'NONE',  ( -3.829620113920000346, 1515.551704408389924, 206.7917118429090237 ) ) ;
#42867=CARTESIAN_POINT ( 'NONE',  ( -2.807895857490450009, 1457.864021610489999, 219.4185499695559827 ) ) ;
#42873=CARTESIAN_POINT ( 'NONE',  ( 7.868158389100000427, 1422.937290482379922, 214.1570520181289794 ) ) ;
#42874=CARTESIAN_POINT ( 'NONE',  ( 3.217370068670000194, 1424.184623524309927, 188.9579833761989960 ) ) ;
#42888=CARTESIAN_POINT ( 'NONE',  ( 1.658713306182930225, 1476.135684546660059, 197.7577052247330016 ) ) ;
#42890=DIRECTION ( 'NONE',  ( 0.000000000000000000, 0.000000000000000000, 1.000000000000000000 ) ) ;
#42906=CARTESIAN_POINT ( 'NONE',  ( -9.842849654513400992, 1471.074449186950005, 212.0442494326119913 ) ) ;
#42930=CARTESIAN_POINT ( 'NONE',  ( 8.691106598842869957, 1437.158280762230106, 210.3924950745289948 ) ) ;
#42931=CARTESIAN_POINT ( 'NONE',  ( 17.08121475022219471, 1494.817603994912133, 195.5684645336626204 ) ) ;
#42939=CARTESIAN_POINT ( 'NONE',  ( -3.727996856979999940, 1429.778334239190144, 201.6824411274789952 ) ) ;
#42946=CARTESIAN_POINT ( 'NONE',  ( 10.10905480207389928, 1461.386512538610077, 208.4426341898000032 ) ) ;
#42951=VERTEX_POINT ( 'NONE', #10629 ) ;
#42953=CARTESIAN_POINT ( 'NONE',  ( -16.91136577339999647, 1420.382390858989993, 203.5950266307289951 ) ) ;
#42956=ADVANCED_FACE ( 'NONE', ( #3354 ), #85812, .T. ) ;
#42959=CARTESIAN_POINT ( 'NONE',  ( -1.634820292203019942, 1423.130284601479843, 191.2821113036930001 ) ) ;
#42961=CARTESIAN_POINT ( 'NONE',  ( -3.620610479546780169, 1508.125677570226799, 220.7440378608293656 ) ) ;
#42969=CARTESIAN_POINT ( 'NONE',  ( -11.00755960056369887, 1418.479267630810000, 198.0234245325859774 ) ) ;
#42970=CARTESIAN_POINT ( 'NONE',  ( -2.898761972770000028, 1491.529727365290000, 188.3233188772989877 ) ) ;
#42977=CARTESIAN_POINT ( 'NONE',  ( 8.876786928998038562, 1425.079649666100067, 195.6689664040229957 ) ) ;
#42981=CARTESIAN_POINT ( 'NONE',  ( -9.104784486305129931, 1421.478983581930152, 192.1853070824809890 ) ) ;
#42987=CARTESIAN_POINT ( 'NONE',  ( 10.57168423260889867, 1452.490699057229904, 209.2976520326539855 ) ) ;
#43002=CARTESIAN_POINT ( 'NONE',  ( -3.467940602053699806, 1495.562067921990092, 197.2905559617530002 ) ) ;
#43007=CARTESIAN_POINT ( 'NONE',  ( 1.120510598883349918, 1486.417731889569950, 197.2577259554180102 ) ) ;
#43008=CARTESIAN_POINT ( 'NONE',  ( 11.34653490123289998, 1471.345105477939796, 210.4582031003209863 ) ) ;
#43010=CARTESIAN_POINT ( 'NONE',  ( -8.316672828268760753, 1425.055149638239982, 204.9623390585310005 ) ) ;
#43015=CARTESIAN_POINT ( 'NONE',  ( 22.29462128660000175, 1476.945831074090165, 209.5903111146230060 ) ) ;
#43017=CARTESIAN_POINT ( 'NONE',  ( 0.000000000000000000, 1524.551704408390151, 209.1218459616989946 ) ) ;
#43022=CARTESIAN_POINT ( 'NONE',  ( -2.112511269397119751, 1421.339275277370007, 193.6972829403189849 ) ) ;
#43024=CARTESIAN_POINT ( 'NONE',  ( -0.7908576644959989244, 1476.560707045389790, 198.6323293514989814 ) ) ;
#43029=CARTESIAN_POINT ( 'NONE',  ( 1.077236975575300182, 1429.570469006359872, 217.3610909002520089 ) ) ;
#43031=ORIENTED_EDGE ( 'NONE', *, *, #106120, .T. ) ;
#43035=B_SPLINE_SURFACE_WITH_KNOTS ( 'NONE', 5, 1, ( 
 ( #103864, #33890 ),
 ( #18190, #85387 ),
 ( #329, #7592 ),
 ( #9801, #68086 ),
 ( #8135, #102198 ),
 ( #9261, #1409 ),
 ( #94340, #110058 ),
 ( #86506, #60790 ),
 ( #42301, #35550 ) ),
 .UNSPECIFIED., .F., .F., .F.,
 ( 6, 3, 6 ),
 ( 2, 2 ),
 ( 0.000000000000000000, 4.014896071639999953, 8.012535616930000160 ),
 ( 0.000000000000000000, 14.00000000000000000 ),
 .UNSPECIFIED. ) ;
#43036=CARTESIAN_POINT ( 'NONE',  ( -7.417501983117125164, 1471.160291404393547, 216.0174856262001128 ) ) ;
#43037=CARTESIAN_POINT ( 'NONE',  ( 7.539259600540419548, 1425.677988097199886, 212.1893721227209824 ) ) ;
#43039=VERTEX_POINT ( 'NONE', #21187 ) ;
#43046=CARTESIAN_POINT ( 'NONE',  ( 7.911464481230000345, 1423.187191425399988, 213.2893462354790017 ) ) ;
#43054=ORIENTED_EDGE ( 'NONE', *, *, #25350, .T. ) ;
#43067=CARTESIAN_POINT ( 'NONE',  ( -0.5237593457439969624, 1444.658999873350012, 199.0797042155420229 ) ) ;
#43068=AXIS2_PLACEMENT_3D ( 'NONE', #89554, #12286, #46480 ) ;
#43073=CARTESIAN_POINT ( 'NONE',  ( -3.274413360710510368, 1508.551704408389924, 213.9819696425469715 ) ) ;
#43075=CARTESIAN_POINT ( 'NONE',  ( 8.028494635650000433, 1421.573180670790180, 196.0255996755989827 ) ) ;
#43077=CARTESIAN_POINT ( 'NONE',  ( -3.370191024799999990, 1496.076861593789772, 198.0269959760989877 ) ) ;
#43088=CARTESIAN_POINT ( 'NONE',  ( -13.58041510073769942, 1508.551704408389924, 210.3416170870220014 ) ) ;
#43090=CARTESIAN_POINT ( 'NONE',  ( 9.544470063946011607, 1422.591896480089872, 212.6773163756829774 ) ) ;
#43093=CARTESIAN_POINT ( 'NONE',  ( 0.9870989395629991003, 1430.542139991489876, 217.5404054456389815 ) ) ;
#43094=DIRECTION ( 'NONE',  ( 0.8775825618903763115, 0.000000000000000000, -0.4794255386041963996 ) ) ;
#43098=CARTESIAN_POINT ( 'NONE',  ( -9.681529208496559846, 1461.089882836170091, 208.7501511576820121 ) ) ;
#43099=CIRCLE ( 'NONE', #86010, 0.9999999999999971134 ) ;
#43100=CARTESIAN_POINT ( 'NONE',  ( -17.17366476699999822, 1421.220024669489931, 201.7389906317289956 ) ) ;
#43101=CARTESIAN_POINT ( 'NONE',  ( 11.20832017736389830, 1422.284948798140022, 203.3916373928120152 ) ) ;
#43108=CARTESIAN_POINT ( 'NONE',  ( -8.114887008623513864, 1425.452370286069936, 208.6318797277072861 ) ) ;
#43111=CARTESIAN_POINT ( 'NONE',  ( 3.115880651068799967, 1508.551704408389924, 219.3718644903320012 ) ) ;
#43113=CARTESIAN_POINT ( 'NONE',  ( 19.38664731554619891, 1498.811923964060043, 221.8202412713110050 ) ) ;
#43115=CARTESIAN_POINT ( 'NONE',  ( -17.56945858326109899, 1419.688318994619976, 207.5872967556749984 ) ) ;
#43117=CARTESIAN_POINT ( 'NONE',  ( 3.060041444019999890, 1442.201653547689830, 217.5704310926890059 ) ) ;
#43129=CARTESIAN_POINT ( 'NONE',  ( 4.726708812725099129, 1506.677470858050128, 216.7649860373589945 ) ) ;
#43131=CARTESIAN_POINT ( 'NONE',  ( -8.342137585866080229, 1436.639472651299911, 213.6062562556910223 ) ) ;
#43133=CARTESIAN_POINT ( 'NONE',  ( -17.01518731959999897, 1422.007497235210167, 208.9682088309940013 ) ) ;
#43134=CARTESIAN_POINT ( 'NONE',  ( 10.95098532600490060, 1471.837423856070018, 212.3987399694809994 ) ) ;
#43138=CARTESIAN_POINT ( 'NONE',  ( 10.86984765289039956, 1425.686504684909778, 206.4627855528160012 ) ) ;
#43140=VECTOR ( 'NONE', #78323, 1000.000000000000000 ) ;
#43142=CARTESIAN_POINT ( 'NONE',  ( 3.063543637962659716, 1437.235349907490217, 227.3972379739110181 ) ) ;
#43148=CARTESIAN_POINT ( 'NONE',  ( -11.03587947549999981, 1492.068057612589882, 205.8034202075890278 ) ) ;
#43152=B_SPLINE_CURVE_WITH_KNOTS ( 'NONE', 3,
 ( #24837, #68546, #93162, #50624, #76374, #59583, #788, #86977, #35472, #10266, #110523, #34917, #68001, #76935, #27087, #69663, #16432, #69103, #84758, #103204, #42223, #94261, #26509, #17537, #94829, #60706, #78586, #44442, #33807, #51739, #18105 ),
 .UNSPECIFIED., .F., .F.,
 ( 4, 3, 3, 3, 3, 3, 3, 3, 3, 3, 4 ),
 ( -8.078160033293929843, -8.078122911508929249, -8.000183041957479091, -7.821082747455149864, -7.564042583401359821, -7.049962255293790392, -6.267197145476660403, -5.680236814612510621, -5.048466761624530008, -4.152322103108110340, -3.282032658275399584 ),
 .UNSPECIFIED. ) ;
#43154=CARTESIAN_POINT ( 'NONE',  ( 8.704769445429999308, 1449.383511506689956, 205.9663214812090359 ) ) ;
#43157=CARTESIAN_POINT ( 'NONE',  ( -0.1310594861909990250, 1456.247027522389999, 199.2609668081589973 ) ) ;
#43161=DIRECTION ( 'NONE',  ( 9.158755289808628626E-47, -1.000000000000000000, 1.836970198721029688E-16 ) ) ;
#43162=CARTESIAN_POINT ( 'NONE',  ( -3.040146223219999833, 1497.073695284489986, 198.2723897717989985 ) ) ;
#43163=CARTESIAN_POINT ( 'NONE',  ( 0.1770319947259980098, 1496.149864682889984, 221.4922559367990118 ) ) ;
#43181=CARTESIAN_POINT ( 'NONE',  ( -5.022927203800000129, 1391.808120115790189, 214.6810046976989952 ) ) ;
#43185=CARTESIAN_POINT ( 'NONE',  ( -19.65244154950000066, 1464.918788182289973, 211.1248570675190024 ) ) ;
#43188=EDGE_LOOP ( 'NONE', ( #6670, #59668, #66185, #85848 ) ) ;
#43189=CARTESIAN_POINT ( 'NONE',  ( 9.099844284766479774, 1451.227735247490045, 210.8294423051630133 ) ) ;
#43193=CARTESIAN_POINT ( 'NONE',  ( -10.83335895338246146, 1417.972034830828079, 198.1741477617316036 ) ) ;
#43197=CARTESIAN_POINT ( 'NONE',  ( 9.146213936677568768, 1449.998330935229887, 208.1168021020649803 ) ) ;
#43199=ADVANCED_FACE ( 'NONE', ( #39111 ), #102777, .F. ) ;
#43214=CARTESIAN_POINT ( 'NONE',  ( -10.46250751532009993, 1491.356802638789986, 212.5409670664860187 ) ) ;
#43216=CARTESIAN_POINT ( 'NONE',  ( 10.52707133736559975, 1469.924776803789882, 207.1255290707819938 ) ) ;
#43217=CARTESIAN_POINT ( 'NONE',  ( -10.06450494029999909, 1472.332863763290106, 203.5506889703189870 ) ) ;
#43219=CARTESIAN_POINT ( 'NONE',  ( 6.287037606400000200, 1493.763477428889928, 218.4859723337289950 ) ) ;
#43225=CARTESIAN_POINT ( 'NONE',  ( 12.16734073514860093, 1492.598615756489835, 211.2522116035209763 ) ) ;
#43232=FACE_OUTER_BOUND ( 'NONE', #98246, .T. ) ;
#43233=CARTESIAN_POINT ( 'NONE',  ( -0.8282867551389770933, 1515.122054816080208, 204.7938966422100009 ) ) ;
#43239=CARTESIAN_POINT ( 'NONE',  ( -3.665756889290000320, 1509.038615934189920, 213.6090957346689834 ) ) ;
#43245=CARTESIAN_POINT ( 'NONE',  ( -10.37333465676420019, 1481.132217322410270, 207.0983991584610067 ) ) ;
#43246=CARTESIAN_POINT ( 'NONE',  ( -12.79440631669999995, 1464.855048088789999, 225.0716344319989730 ) ) ;
#43252=CARTESIAN_POINT ( 'NONE',  ( -15.59069434664220211, 1418.231165713569908, 203.0305569057429693 ) ) ;
#43256=CARTESIAN_POINT ( 'NONE',  ( -15.90345171279999903, 1418.061017481300269, 203.7331489593690037 ) ) ;
#43258=CARTESIAN_POINT ( 'NONE',  ( -5.786158641081859955, 1484.802378851279855, 198.7188167466890150 ) ) ;
#43260=CARTESIAN_POINT ( 'NONE',  ( -9.612987031380001213, 1499.623719321889894, 216.9466790759489925 ) ) ;
#43265=CARTESIAN_POINT ( 'NONE',  ( -12.13242141250689876, 1508.441653837850026, 209.3107298190460028 ) ) ;
#43278=CARTESIAN_POINT ( 'NONE',  ( -15.80168118454438542, 1415.804992922690644, 209.5032348057993090 ) ) ;
#43288=CARTESIAN_POINT ( 'NONE',  ( 11.27337545052449919, 1433.557891923710031, 225.8166880305549853 ) ) ;
#43290=CARTESIAN_POINT ( 'NONE',  ( 5.076283890887699712, 1469.790178735639984, 187.8425608536880134 ) ) ;
#43294=CARTESIAN_POINT ( 'NONE',  ( 9.716708914843909639, 1436.182072645820199, 210.6488788081859980 ) ) ;
#43295=CARTESIAN_POINT ( 'NONE',  ( -10.62228157299999864, 1490.415513672490079, 212.3812309668689977 ) ) ;
#43296=CARTESIAN_POINT ( 'NONE',  ( 9.522150312267969596, 1450.466928359630174, 204.8643194434029908 ) ) ;
#43303=CARTESIAN_POINT ( 'NONE',  ( 7.252896346444960507, 1505.517465422420173, 218.2988040474139950 ) ) ;
#43306=VERTEX_POINT ( 'NONE', #28955 ) ;
#43312=EDGE_CURVE ( 'NONE', #86829, #69095, #32835, .T. ) ;
#43313=CARTESIAN_POINT ( 'NONE',  ( -10.36555841800240074, 1448.133745289950184, 208.8105289421490056 ) ) ;
#43323=CARTESIAN_POINT ( 'NONE',  ( 1.875672330807159893, 1456.514202357329850, 219.5762932319839820 ) ) ;
#43330=CARTESIAN_POINT ( 'NONE',  ( -0.1361343663501470291, 1432.257650919470052, 200.6952069693479928 ) ) ;
#43332=ORIENTED_EDGE ( 'NONE', *, *, #10326, .T. ) ;
#43336=CARTESIAN_POINT ( 'NONE',  ( 21.14413832960000050, 1497.093652768289985, 210.1540944253389966 ) ) ;
#43354=CARTESIAN_POINT ( 'NONE',  ( -16.78006084555529753, 1508.551704408389924, 210.3901253742230040 ) ) ;
#43362=CARTESIAN_POINT ( 'NONE',  ( -2.675466344130340346, 1429.100645368589994, 200.1409435021539878 ) ) ;
#43378=CARTESIAN_POINT ( 'NONE',  ( -9.207810800643882132, 1450.012628189060251, 209.2145258953920006 ) ) ;
#43382=CARTESIAN_POINT ( 'NONE',  ( -10.60922226581860173, 1508.438309873620028, 218.5024624024570130 ) ) ;
#43384=CARTESIAN_POINT ( 'NONE',  ( 4.490619219238107362, 1508.909942010395071, 211.6097810847319920 ) ) ;
#43388=CARTESIAN_POINT ( 'NONE',  ( 18.72979941119999836, 1454.437773883689943, 204.5413093961989830 ) ) ;
#43392=CARTESIAN_POINT ( 'NONE',  ( -2.521939269659999816, 1431.047916005589968, 201.1291089318189904 ) ) ;
#43393=CARTESIAN_POINT ( 'NONE',  ( 10.67459791866189889, 1480.672717750939910, 209.7791954089520061 ) ) ;
#43400=CARTESIAN_POINT ( 'NONE',  ( 2.070952440869999744, 1486.243875337790087, 198.1392447632989899 ) ) ;
#43401=DIRECTION ( 'NONE',  ( 0.000000000000000000, -1.836970198721029688E-16, -1.000000000000000000 ) ) ;
#43406=CARTESIAN_POINT ( 'NONE',  ( 6.870966381969999759, 1425.576645473769986, 212.2423038635290027 ) ) ;
#43417=CARTESIAN_POINT ( 'NONE',  ( -1.031112549849209969, 1488.425549442109968, 217.1473076880390067 ) ) ;
#43421=CARTESIAN_POINT ( 'NONE',  ( -15.28485084270191408, 1416.039222364684520, 206.5424821588011923 ) ) ;
#43422=CARTESIAN_POINT ( 'NONE',  ( 1.776583262209999958, 1456.341123502790197, 219.1753798273990128 ) ) ;
#43423=CARTESIAN_POINT ( 'NONE',  ( -3.056112608387090201, 1457.952188555200109, 219.3550834608830087 ) ) ;
#43424=B_SPLINE_CURVE_WITH_KNOTS ( 'NONE', 5,
 ( #76162, #67232, #66683, #34156, #68342, #101328 ),
 .UNSPECIFIED., .F., .F.,
 ( 6, 6 ),
 ( 0.000000000000000000, 1.000000000000000000 ),
 .UNSPECIFIED. ) ;
#43428=CARTESIAN_POINT ( 'NONE',  ( -13.05162051250000133, 1467.538720777590015, 191.8992815354989716 ) ) ;
#43432=CARTESIAN_POINT ( 'NONE',  ( 5.641423425050000162, 1453.485726096290136, 216.6286100207389893 ) ) ;
#43438=CARTESIAN_POINT ( 'NONE',  ( 10.92766316885620093, 1501.618323021010156, 205.6861136770480130 ) ) ;
#43441=EDGE_CURVE ( 'NONE', #60672, #1788, #11338, .T. ) ;
#43455=EDGE_LOOP ( 'NONE', ( #53817, #53392, #79784, #57830 ) ) ;
#43477=CARTESIAN_POINT ( 'NONE',  ( 5.945307986799999611, 1451.422783942589831, 210.3535049228189848 ) ) ;
#43489=ORIENTED_EDGE ( 'NONE', *, *, #94808, .F. ) ;
#43493=ORIENTED_EDGE ( 'NONE', *, *, #83137, .T. ) ;
#43494=CARTESIAN_POINT ( 'NONE',  ( -8.106555885276549134, 1438.741351455190170, 205.9368832915250209 ) ) ;
#43500=CARTESIAN_POINT ( 'NONE',  ( 2.561313721290320089, 1430.951449648099924, 218.2616813023740008 ) ) ;
#43511=( BOUNDED_SURFACE ( )  B_SPLINE_SURFACE ( 1, 2, ( 
 ( #67091, #109084, #91712, #57588, #32895, #49182, #110168 ),
 ( #6608, #32365, #66547, #100649, #92262, #15533, #102849 ) ),
 .UNSPECIFIED., .F., .F., .F. ) 
 B_SPLINE_SURFACE_WITH_KNOTS ( ( 2, 2 ),
 ( 3, 2, 2, 3 ),
 ( -10000.00000000000000, 10000.00000000000000 ),
 ( 5.770213214421419323, 6.283185307179590673, 7.853981633974480125, 8.911805878012049931 ),
 .UNSPECIFIED. ) 
 GEOMETRIC_REPRESENTATION_ITEM ( )  RATIONAL_B_SPLINE_SURFACE ( (
 ( 0.8711730249286460115, 0.9043503954990910199, 1.000000000000000000, 0.7071067811865480168, 1.000000000000000000, 0.8027563838226849935, 0.8711730262222899812),
 ( 0.8711730249286460115, 0.9043503954990910199, 1.000000000000000000, 0.7071067811865480168, 1.000000000000000000, 0.8027563838226849935, 0.8711730262222899812) ) ) 
 REPRESENTATION_ITEM ( '' )  SURFACE ( )  );
#43512=CARTESIAN_POINT ( 'NONE',  ( -21.56904447630000021, 1506.866154825289868, 209.3454515566180021 ) ) ;
#43517=CARTESIAN_POINT ( 'NONE',  ( -3.637603509031002158, 1508.126921005884469, 220.7408464239917407 ) ) ;
#43518=B_SPLINE_CURVE_WITH_KNOTS ( 'NONE', 3,
 ( #87245, #9429, #43593, #2168, #17239, #69923 ),
 .UNSPECIFIED., .F., .F.,
 ( 4, 2, 4 ),
 ( 0.000000000000000000, 0.5000000000000000000, 1.000000000000000000 ),
 .UNSPECIFIED. ) ;
#43521=CARTESIAN_POINT ( 'NONE',  ( -6.785334565741740320, 1457.914568211761662, 215.8412113930604335 ) ) ;
#43524=CARTESIAN_POINT ( 'NONE',  ( -10.16243888589800015, 1472.559490735430018, 209.8188024594959984 ) ) ;
#43526=CARTESIAN_POINT ( 'NONE',  ( -3.250000000000000000, 1524.051704408389924, 209.1218459616989946 ) ) ;
#43528=CARTESIAN_POINT ( 'NONE',  ( -8.356240136749999436, 1508.431981883589970, 219.3528788934989961 ) ) ;
#43531=CARTESIAN_POINT ( 'NONE',  ( 9.651066088509999474, 1425.440658930580184, 195.4941615409990163 ) ) ;
#43532=CARTESIAN_POINT ( 'NONE',  ( 5.145309177750649887, 1422.426130283250131, 194.5914460530619863 ) ) ;
#43533=CARTESIAN_POINT ( 'NONE',  ( -11.39446592756109844, 1470.674086296440009, 209.5209556861319982 ) ) ;
#43535=CARTESIAN_POINT ( 'NONE',  ( 20.33508558929999666, 1432.834457682990205, 214.7556889579689994 ) ) ;
#43541=ORIENTED_EDGE ( 'NONE', *, *, #62860, .T. ) ;
#43552=CARTESIAN_POINT ( 'NONE',  ( 8.626226792742770044, 1436.875340518389976, 208.7668036561229883 ) ) ;
#43554=DIRECTION ( 'NONE',  ( 0.8775825618903700942, 0.000000000000000000, -0.4794255386042075018 ) ) ;
#43555=DIRECTION ( 'NONE',  ( -0.8826905754104281687, -0.3875151742776350439, -0.2658746655591340269 ) ) ;
#43560=CARTESIAN_POINT ( 'NONE',  ( -12.25922289946369936, 1422.754725847070176, 204.0266690164509953 ) ) ;
#43564=CARTESIAN_POINT ( 'NONE',  ( -2.487922401834420594, 1508.551704408489968, 213.9544572570970047 ) ) ;
#43565=CARTESIAN_POINT ( 'NONE',  ( 22.20352485945739929, 1475.168806475580141, 209.9014948442749926 ) ) ;
#43567=DIRECTION ( 'NONE',  ( -1.000000000000000000, 0.000000000000000000, 0.000000000000000000 ) ) ;
#43572=CARTESIAN_POINT ( 'NONE',  ( -19.97968237250000101, 1483.906011188890034, 214.0068283976289933 ) ) ;
#43580=CARTESIAN_POINT ( 'NONE',  ( -8.403628046679999741, 1423.510048004620103, 210.2177463927289978 ) ) ;
#43586=CARTESIAN_POINT ( 'NONE',  ( 7.531010940995349401, 1425.504834242530023, 212.1895840461209843 ) ) ;
#43589=EDGE_CURVE ( 'NONE', #2493, #2466, #70180, .T. ) ;
#43593=CARTESIAN_POINT ( 'NONE',  ( 6.375244903274786878, 1427.171875868285724, 214.3396874122583711 ) ) ;
#43594=CARTESIAN_POINT ( 'NONE',  ( -18.95466419752950316, 1508.523044920219718, 209.9298748376089918 ) ) ;
#43603=VERTEX_POINT ( 'NONE', #47688 ) ;
#43613=B_SPLINE_CURVE_WITH_KNOTS ( 'NONE', 5,
 ( #82714, #88908, #30089, #89460, #4896, #91109 ),
 .UNSPECIFIED., .F., .F.,
 ( 6, 6 ),
 ( 172.3296575809999922, 177.0697656899999970 ),
 .UNSPECIFIED. ) ;
#43615=CARTESIAN_POINT ( 'NONE',  ( -4.734430706410000411, 1428.274085907389917, 201.8092844071990157 ) ) ;
#43625=CARTESIAN_POINT ( 'NONE',  ( -3.704457720420359923, 1508.551704408389924, 213.7941704926340094 ) ) ;
#43627=CARTESIAN_POINT ( 'NONE',  ( 7.472825078389999653, 1423.077329920680086, 195.6326666296990027 ) ) ;
#43630=LINE ( 'NONE', #28480, #67853 ) ;
#43641=CARTESIAN_POINT ( 'NONE',  ( 0.6255730392936860174, 1421.220699880276015, 193.7286507490917415 ) ) ;
#43649=CARTESIAN_POINT ( 'NONE',  ( -17.71128632129999758, 1420.275165550689962, 207.4128878226090080 ) ) ;
#43650=CARTESIAN_POINT ( 'NONE',  ( 11.09566315855570018, 1425.086810962289974, 203.0248004916680031 ) ) ;
#43652=CARTESIAN_POINT ( 'NONE',  ( 9.774680401711808742, 1462.791281439700242, 210.7173239812339887 ) ) ;
#43658=CARTESIAN_POINT ( 'NONE',  ( -0.001293896702980919895, 1473.458796427790048, 216.6124729060890104 ) ) ;
#43661=CARTESIAN_POINT ( 'NONE',  ( -0.03315910861134309384, 1502.038559631680073, 233.2541124739660177 ) ) ;
#43663=CARTESIAN_POINT ( 'NONE',  ( -16.21109120713730078, 1420.416353679290069, 206.3072091156649890 ) ) ;
#43664=CARTESIAN_POINT ( 'NONE',  ( 9.105494218695110220, 1451.204579960250157, 210.7726874829440078 ) ) ;
#43665=CARTESIAN_POINT ( 'NONE',  ( 3.533229526830000022, 1442.898285365590027, 217.2834840181990046 ) ) ;
#43670=CARTESIAN_POINT ( 'NONE',  ( -4.796874865469999527, 1476.201330746690019, 199.9539643786289957 ) ) ;
#43672=CARTESIAN_POINT ( 'NONE',  ( -6.168107933492159134, 1508.551704408389924, 219.3995182160069817 ) ) ;
#43675=CARTESIAN_POINT ( 'NONE',  ( -4.987078426973329925, 1508.551704408389924, 206.6339106789369851 ) ) ;
#43679=CARTESIAN_POINT ( 'NONE',  ( 4.478041536509679510, 1465.868555709299926, 203.7095503217849739 ) ) ;
#43695=CARTESIAN_POINT ( 'NONE',  ( -7.537381089459999295, 1495.227545663890169, 200.7918938288690072 ) ) ;
#43701=CARTESIAN_POINT ( 'NONE',  ( -20.87069991009999725, 1506.658021081189872, 214.5368842940590071 ) ) ;
#43709=CARTESIAN_POINT ( 'NONE',  ( -2.658323007379999936, 1496.524950806489869, 220.4400205060989890 ) ) ;
#43724=CARTESIAN_POINT ( 'NONE',  ( -5.026420246739999875, 1391.797184865090003, 214.5825844794689772 ) ) ;
#43728=CARTESIAN_POINT ( 'NONE',  ( 9.941518348215939938, 1460.939688249500023, 207.2380014999110074 ) ) ;
#43734=CARTESIAN_POINT ( 'NONE',  ( 9.242927444819999394, 1424.975928711410006, 196.2247933120989956 ) ) ;
#43735=VERTEX_POINT ( 'NONE', #82388 ) ;
#43736=CARTESIAN_POINT ( 'NONE',  ( -7.756928808066270165, 1508.430203411700177, 219.4938965895260026 ) ) ;
#43737=CARTESIAN_POINT ( 'NONE',  ( -9.335045448769683674, 1418.488145321254478, 196.8730397695123884 ) ) ;
#43743=CARTESIAN_POINT ( 'NONE',  ( 10.54229472710979998, 1452.173451298499913, 208.4873773006349893 ) ) ;
#43756=CARTESIAN_POINT ( 'NONE',  ( -1.811252493420050014, 1468.887500306539778, 219.1128618160599899 ) ) ;
#43761=CARTESIAN_POINT ( 'NONE',  ( 8.185540730390000519, 1494.061971860590120, 217.8458731800789963 ) ) ;
#43763=CARTESIAN_POINT ( 'NONE',  ( 8.107340703835214768, 1424.171636185274110, 195.7651162605105810 ) ) ;
#43764=CARTESIAN_POINT ( 'NONE',  ( -3.617573937782270210, 1497.333809982809953, 198.4503636364750037 ) ) ;
#43765=CARTESIAN_POINT ( 'NONE',  ( 9.751541468637160648, 1469.019378510909974, 203.4839537346510099 ) ) ;
#43773=CARTESIAN_POINT ( 'NONE',  ( -14.68224678300000008, 1416.181292664740113, 213.8220209240589895 ) ) ;
#43774=AXIS2_PLACEMENT_3D ( 'NONE', #58919, #58369, #48882 ) ;
#43775=CARTESIAN_POINT ( 'NONE',  ( 1.694729585907490010, 1515.066341861380124, 204.7924377471120181 ) ) ;
#43776=VERTEX_POINT ( 'NONE', #101915 ) ;
#43777=CARTESIAN_POINT ( 'NONE',  ( -15.85288220972839035, 1415.900318358362483, 209.7246934675221723 ) ) ;
#43781=CARTESIAN_POINT ( 'NONE',  ( -11.03352341481849841, 1462.446812322350070, 208.7213867630900097 ) ) ;
#43786=CARTESIAN_POINT ( 'NONE',  ( -10.22273176409999884, 1479.690303922389830, 215.0709727714090036 ) ) ;
#43794=EDGE_CURVE ( 'NONE', #87329, #3165, #68764, .T. ) ;
#43801=CARTESIAN_POINT ( 'NONE',  ( -2.487935123034410001, 1509.038615930399828, 213.6090957347729784 ) ) ;
#43802=EDGE_CURVE ( 'NONE', #75670, #78107, #66200, .T. ) ;
#43810=CARTESIAN_POINT ( 'NONE',  ( -12.28097721992999958, 1508.220391055730033, 209.1123848330070132 ) ) ;
#43825=B_SPLINE_CURVE_WITH_KNOTS ( 'NONE', 3,
 ( #100243, #50952, #7283, #82882, #49301, #85077, #99666, #23521, #92934, #83426 ),
 .UNSPECIFIED., .F., .F.,
 ( 4, 2, 2, 2, 4 ),
 ( 2.065250908360339998E-07, 0.03315402003890329657, 0.05105978556791049977, 0.05919766143195339531, 0.06630775015685380636 ),
 .UNSPECIFIED. ) ;
#43828=CARTESIAN_POINT ( 'NONE',  ( 4.070747692530000350, 1486.294283939790148, 219.1124398665789954 ) ) ;
#43829=CARTESIAN_POINT ( 'NONE',  ( 11.24836030156600053, 1479.301895909970199, 207.8159963017580196 ) ) ;
#43832=CARTESIAN_POINT ( 'NONE',  ( 20.79429048353240006, 1456.232304843699922, 207.0687085352159897 ) ) ;
#43834=ADVANCED_FACE ( 'NONE', ( #77846 ), #93826, .T. ) ;
#43835=CARTESIAN_POINT ( 'NONE',  ( -17.55008888293159686, 1487.029577683950038, 194.9701234137779977 ) ) ;
#43838=CARTESIAN_POINT ( 'NONE',  ( -4.992439177819999685, 1391.624324237289784, 203.6930817768189854 ) ) ;
#43840=CARTESIAN_POINT ( 'NONE',  ( -11.71397067460000052, 1489.483176008789997, 212.5377880877490213 ) ) ;
#43841=CARTESIAN_POINT ( 'NONE',  ( 9.833400138500138610, 1450.823812866140088, 205.5646184881250065 ) ) ;
#43847=CARTESIAN_POINT ( 'NONE',  ( 8.147371244622188868, 1505.597128609329957, 217.5190773777700031 ) ) ;
#43848=CARTESIAN_POINT ( 'NONE',  ( -9.821980025724538876, 1422.689482519856483, 210.6756101855388863 ) ) ;
#43850=ORIENTED_EDGE ( 'NONE', *, *, #4155, .T. ) ;
#43869=CARTESIAN_POINT ( 'NONE',  ( -14.92548077329999856, 1420.621803361759930, 210.5949619620589885 ) ) ;
#43873=CARTESIAN_POINT ( 'NONE',  ( 1.248319867352440049, 1432.832940376729994, 200.7627304351539976 ) ) ;
#43880=CARTESIAN_POINT ( 'NONE',  ( 9.831195298860000875, 1461.796653712189936, 208.3421129825899811 ) ) ;
#43894=CARTESIAN_POINT ( 'NONE',  ( 4.144810350071930216, 1423.945503712369828, 193.0065599516869952 ) ) ;
#43895=VERTEX_POINT ( 'NONE', #18455 ) ;
#43900=EDGE_CURVE ( 'NONE', #93500, #10365, #739, .T. ) ;
#43902=CARTESIAN_POINT ( 'NONE',  ( -1.880981557899999990, 1491.684224442789855, 188.2614447320989939 ) ) ;
#43903=EDGE_CURVE ( 'NONE', #14195, #88662, #80853, .T. ) ;
#43905=CARTESIAN_POINT ( 'NONE',  ( -3.259994511801839856, 1428.775419947709906, 200.3424632861539862 ) ) ;
#43913=VERTEX_POINT ( 'NONE', #47555 ) ;
#43915=CARTESIAN_POINT ( 'NONE',  ( 10.88673685277470149, 1490.602448971980039, 210.5186076668310022 ) ) ;
#43916=FACE_OUTER_BOUND ( 'NONE', #61241, .T. ) ;
#43932=CARTESIAN_POINT ( 'NONE',  ( 3.395043742270000386, 1466.412111213989874, 219.6384586637989855 ) ) ;
#43933=CARTESIAN_POINT ( 'NONE',  ( 8.759801967190000482, 1450.891143041990063, 191.6269498783990173 ) ) ;
#43938=CARTESIAN_POINT ( 'NONE',  ( 0.7579935661000010150, 1432.645091882289989, 200.6977994915789907 ) ) ;
#43939=CARTESIAN_POINT ( 'NONE',  ( 10.95552075894139854, 1480.084818102109921, 209.3730989235789934 ) ) ;
#43948=CARTESIAN_POINT ( 'NONE',  ( 3.197956043390000058, 1485.326915628889992, 198.8549714615990069 ) ) ;
#43951=CARTESIAN_POINT ( 'NONE',  ( 11.36432067319999994, 1502.559788237589828, 210.8834125687090193 ) ) ;
#43953=CARTESIAN_POINT ( 'NONE',  ( 8.044556495430001064, 1427.503828071409998, 212.2292562717090050 ) ) ;
#43955=EDGE_CURVE ( 'NONE', #89851, #37990, #44463, .T. ) ;
#43957=CARTESIAN_POINT ( 'NONE',  ( -9.069247167689999500, 1483.910511149589865, 201.2456827287589931 ) ) ;
#43964=ORIENTED_EDGE ( 'NONE', *, *, #6559, .F. ) ;
#43966=FACE_OUTER_BOUND ( 'NONE', #33775, .T. ) ;
#43967=CARTESIAN_POINT ( 'NONE',  ( -14.48519483975229960, 1416.181292564900104, 203.8595933512790168 ) ) ;
#43970=CARTESIAN_POINT ( 'NONE',  ( -1.604553179929740114, 1457.465057722440179, 219.6491839707440192 ) ) ;
#43975=CARTESIAN_POINT ( 'NONE',  ( 7.597901083480000040, 1425.607998949240027, 212.0366610610989824 ) ) ;
#43976=CARTESIAN_POINT ( 'NONE',  ( -20.43379408400000230, 1466.940146741789931, 211.2182734472289951 ) ) ;
#43982=CARTESIAN_POINT ( 'NONE',  ( 4.594279763170000308, 1454.322381208490015, 217.3118965033989980 ) ) ;
#43983=ORIENTED_EDGE ( 'NONE', *, *, #65812, .F. ) ;
#43990=CARTESIAN_POINT ( 'NONE',  ( 7.527142396971010285, 1500.274912714168295, 200.5649840229101812 ) ) ;
#44006=CARTESIAN_POINT ( 'NONE',  ( -4.062020363349999386, 1454.690385904389814, 200.4959040790290032 ) ) ;
#44015=EDGE_CURVE ( 'NONE', #108309, #7222, #65963, .T. ) ;
#44023=CARTESIAN_POINT ( 'NONE',  ( -10.28013528708800095, 1471.607561417190027, 209.6293381314150110 ) ) ;
#44025=ORIENTED_EDGE ( 'NONE', *, *, #66456, .F. ) ;
#44033=CARTESIAN_POINT ( 'NONE',  ( 4.363292141028189519, 1485.773534554989965, 215.9131765237970058 ) ) ;
#44042=ADVANCED_FACE ( 'NONE', ( #25075 ), #94495, .T. ) ;
#44062=CARTESIAN_POINT ( 'NONE',  ( -12.73491051959999965, 1505.539654372990071, 209.0093621724030015 ) ) ;
#44064=CARTESIAN_POINT ( 'NONE',  ( 2.833473913299999758, 1441.452951622389946, 218.6297931320189889 ) ) ;
#44069=EDGE_CURVE ( 'NONE', #26627, #3898, #18884, .T. ) ;
#44070=CARTESIAN_POINT ( 'NONE',  ( -9.361711274563111473, 1459.704131987939718, 211.5409763055165797 ) ) ;
#44073=CARTESIAN_POINT ( 'NONE',  ( -4.153788892804460176, 1419.995762630720037, 194.1221349337969855 ) ) ;
#44078=CARTESIAN_POINT ( 'NONE',  ( -4.987078446123650366, 1508.551704408389924, 211.6097672649169681 ) ) ;
#44084=CARTESIAN_POINT ( 'NONE',  ( -11.38839566446790030, 1470.646819187970095, 209.6436936467169687 ) ) ;
#44086=CARTESIAN_POINT ( 'NONE',  ( -4.636579742356272682, 1378.025655545858172, 203.9278500733525732 ) ) ;
#44093=CARTESIAN_POINT ( 'NONE',  ( 10.35455463498039919, 1451.650344723270109, 207.2882537262890139 ) ) ;
#44103=VECTOR ( 'NONE', #67845, 1000.000000000000227 ) ;
#44107=B_SPLINE_CURVE_WITH_KNOTS ( 'NONE', 5,
 ( #71611, #20578, #105168, #95107, #28458, #54778, #27344, #87261, #79420 ),
 .UNSPECIFIED., .F., .F.,
 ( 6, 3, 6 ),
 ( 0.000000000000000000, 0.6011310882172063996, 1.000000000000000000 ),
 .UNSPECIFIED. ) ;
#44108=CARTESIAN_POINT ( 'NONE',  ( 8.591050007833809232, 1437.123692357109803, 208.1883534641620201 ) ) ;
#44117=CARTESIAN_POINT ( 'NONE',  ( -9.207216801295770026, 1450.122646856020083, 208.9920191583770190 ) ) ;
#44118=CARTESIAN_POINT ( 'NONE',  ( -12.67427553544369800, 1422.533749357050056, 203.9427823080079918 ) ) ;
#44122=CARTESIAN_POINT ( 'NONE',  ( -11.64264026049999856, 1508.093831663089986, 207.6305009244389908 ) ) ;
#44123=CARTESIAN_POINT ( 'NONE',  ( 4.831085042146060715, 1471.573324702249920, 187.7042132603309881 ) ) ;
#44128=CARTESIAN_POINT ( 'NONE',  ( -2.330134118790000208, 1515.551704408389924, 212.9514660756190096 ) ) ;
#44136=LINE ( 'NONE', #10520, #24691 ) ;
#44138=CARTESIAN_POINT ( 'NONE',  ( -9.200421029710000198, 1422.937291652149952, 210.7384574684489849 ) ) ;
#44143=CARTESIAN_POINT ( 'NONE',  ( 7.479962015650619023, 1426.053219697059831, 212.3726218137090029 ) ) ;
#44145=CARTESIAN_POINT ( 'NONE',  ( -2.670576961741749855, 1496.965622226749929, 221.2123459303559798 ) ) ;
#44153=CARTESIAN_POINT ( 'NONE',  ( -8.510946600262379036, 1439.450974936100238, 206.5611942902239946 ) ) ;
#44158=CARTESIAN_POINT ( 'NONE',  ( 8.534077335428490230, 1434.919601520179867, 206.3687546489890110 ) ) ;
#44179=CARTESIAN_POINT ( 'NONE',  ( 2.487924095911270062, 1509.038643251730036, 204.6345969343269928 ) ) ;
#44189=VECTOR ( 'NONE', #10734, 1000.000000000000227 ) ;
#44196=CARTESIAN_POINT ( 'NONE',  ( 0.8903091994049979752, 1462.735716105790061, 228.8847082000989985 ) ) ;
#44200=DIRECTION ( 'NONE',  ( -1.699538841806929935E-33, 1.000000000000000000, -1.698192320643030073E-16 ) ) ;
#44201=CARTESIAN_POINT ( 'NONE',  ( -4.329448776040000446, 1515.064792882589927, 207.3534014088789945 ) ) ;
#44202=EDGE_CURVE ( 'NONE', #27485, #53857, #8635, .T. ) ;
#44204=CARTESIAN_POINT ( 'NONE',  ( -14.42895190569277730, 1415.865101995087116, 203.8800253993052536 ) ) ;
#44209=CARTESIAN_POINT ( 'NONE',  ( -17.22999524109999925, 1421.609273190410022, 201.8193996009690068 ) ) ;
#44216=VECTOR ( 'NONE', #43555, 1000.000000000000227 ) ;
#44218=CARTESIAN_POINT ( 'NONE',  ( -17.47221698915792487, 1419.835909614559569, 206.8863186588654060 ) ) ;
#44221=CARTESIAN_POINT ( 'NONE',  ( -22.15968324266369649, 1485.573346209269857, 217.2083651811669824 ) ) ;
#44223=CARTESIAN_POINT ( 'NONE',  ( 203.9558787908000284, -8382.262153571269664, -1760.903728536709878 ) ) ;
#44226=CARTESIAN_POINT ( 'NONE',  ( 2.999852707240000083, 1441.831684494889942, 217.8331580874990152 ) ) ;
#44233=CARTESIAN_POINT ( 'NONE',  ( 14.43087674896799832, 1426.807405976119981, 195.4949895358049901 ) ) ;
#44234=ORIENTED_EDGE ( 'NONE', *, *, #107818, .T. ) ;
#44239=CARTESIAN_POINT ( 'NONE',  ( 0.1274077701469989998, 1431.278402656690105, 217.8904900432389979 ) ) ;
#44240=CARTESIAN_POINT ( 'NONE',  ( -10.84355950384670209, 1471.555694810890145, 206.8501174806650056 ) ) ;
#44249=CARTESIAN_POINT ( 'NONE',  ( 11.68008220344320058, 1491.335982786950126, 207.1828859132960190 ) ) ;
#44252=CARTESIAN_POINT ( 'NONE',  ( -19.50375265270000114, 1467.690089012490034, 205.2528463378490073 ) ) ;
#44253=ORIENTED_EDGE ( 'NONE', *, *, #14410, .F. ) ;
#44254=ADVANCED_FACE ( 'NONE', ( #45241 ), #35557, .T. ) ;
#44255=CARTESIAN_POINT ( 'NONE',  ( -18.50490982315079691, 1441.562997674779808, 211.9760908666659986 ) ) ;
#44263=CARTESIAN_POINT ( 'NONE',  ( -8.323380306660000727, 1512.192073244490075, 211.6849953306190173 ) ) ;
#44265=CARTESIAN_POINT ( 'NONE',  ( -15.90854778520130175, 1487.107804145120099, 195.7315998840579994 ) ) ;
#44266=CARTESIAN_POINT ( 'NONE',  ( 1.186695575399999925, 1456.165747688890178, 198.6030552828989926 ) ) ;
#44271=CARTESIAN_POINT ( 'NONE',  ( -2.924124371280000023, 1495.932676772589957, 197.5380625559990051 ) ) ;
#44272=CARTESIAN_POINT ( 'NONE',  ( -2.781330248550000217, 1495.730979733589948, 219.9850975371990103 ) ) ;
#44275=VERTEX_POINT ( 'NONE', #90516 ) ;
#44286=CARTESIAN_POINT ( 'NONE',  ( 4.860123680919410383, 1508.551704408389924, 212.3962593222019848 ) ) ;
#44290=CARTESIAN_POINT ( 'NONE',  ( 9.170246928576359480, 1461.406349500210126, 205.9599371887860002 ) ) ;
#44293=ORIENTED_EDGE ( 'NONE', *, *, #41252, .F. ) ;
#44299=B_SPLINE_CURVE_WITH_KNOTS ( 'NONE', 3,
 ( #84400, #83845, #7144, #42959, #41301, #41845, #67619, #67072, #51346, #57570, #85479, #24472, #60315, #19947, #54140, #11010, #1515, #18280, #88269, #35648, #78203, #70953, #69837, #86056, #61435 ),
 .UNSPECIFIED., .F., .F.,
 ( 4, 3, 3, 3, 3, 3, 3, 3, 4 ),
 ( -3.202470023179999625, -2.306874149981480215, -1.412366672554860036, -0.5199827250689450509, -0.01259353077460012571, 0.6689285225653880396, 1.550313525218030453, 2.444820790987910275, 3.202470023179999625 ),
 .UNSPECIFIED. ) ;
#44304=CARTESIAN_POINT ( 'NONE',  ( 9.229093028962669365, 1450.500814747789946, 209.1422214426999915 ) ) ;
#44305=CARTESIAN_POINT ( 'NONE',  ( 19.40352163639999716, 1457.233006875389947, 208.1928089228509862 ) ) ;
#44311=B_SPLINE_CURVE_WITH_KNOTS ( 'NONE', 3,
 ( #46714, #21453, #39939, #23118, #6335, #55664, #22547, #108239, #48915, #14171, #89786, #71938, #98736, #30429, #106050, #14725, #29327, #21996, #13057 ),
 .UNSPECIFIED., .F., .F.,
 ( 4, 3, 3, 3, 3, 3, 4 ),
 ( -7.154418202789190495, -6.862826068025819737, -5.884430753544330095, -5.043863493629519468, -4.380177091811430223, -3.634519997509699785, -2.933308256780000178 ),
 .UNSPECIFIED. ) ;
#44316=CARTESIAN_POINT ( 'NONE',  ( -5.904615859283640411, 1508.524893063339960, 219.7761321644620125 ) ) ;
#44323=CARTESIAN_POINT ( 'NONE',  ( 8.810981746659999558, 1493.003242455989721, 216.1956613704689971 ) ) ;
#44327=DIRECTION ( 'NONE',  ( 0.000000000000000000, 1.000000000000000000, -1.836970198721029688E-16 ) ) ;
#44328=B_SPLINE_CURVE_WITH_KNOTS ( 'NONE', 3,
 ( #26408, #60600, #41010, #32622, #100897, #24194, #7412, #37020, #78484, #44341, #35371, #70119, #96386, #63367, #104783, #11827, #69559, #53298, #28069, #44906, #62829, #62258, #1234, #18546, #43777, #19663, #10168, #103679, #2357, #105897, #52740, #71778, #53867, #87439, #26978, #1798, #37577, #88007 ),
 .UNSPECIFIED., .F., .F.,
 ( 4, 2, 2, 1, 2, 2, 2, 2, 1, 2, 2, 2, 2, 2, 2, 2, 1, 1, 2, 2, 4 ),
 ( 0.000000000000000000, 0.1250000000021257163, 0.1875000000032436553, 0.2187500000037996550, 0.2343750000041891490, 0.2500000000045786153, 0.3750000000091979757, 0.4375000000115244481, 0.4687500000129335986, 0.4843750000136203271, 0.5000000000143071111, 0.6250000000158285607, 0.6406250000158579816, 0.6562500000158874025, 0.6875000000159626756, 0.7187500000160379487, 0.7343750000153863589, 0.7421875000150697232, 0.7460937500149279478, 0.7500000000147862833, 1.000000000000000000 ),
 .UNSPECIFIED. ) ;
#44330=CONICAL_SURFACE ( 'NONE', #13831, 0.9999999999999962252, 0.7853981633970000820 ) ;
#44333=VERTEX_POINT ( 'NONE', #7069 ) ;
#44337=CARTESIAN_POINT ( 'NONE',  ( 3.958201235949999841, 1505.664173997190119, 220.8429677841990042 ) ) ;
#44338=CARTESIAN_POINT ( 'NONE',  ( -14.41799994660000017, 1415.865102022439942, 214.3937196626189916 ) ) ;
#44339=CARTESIAN_POINT ( 'NONE',  ( -1.037000659099919897, 1515.105800736289893, 204.7934710141580013 ) ) ;
#44341=CARTESIAN_POINT ( 'NONE',  ( -15.63150152900681711, 1415.710789684446127, 209.6412575786757486 ) ) ;
#44343=CARTESIAN_POINT ( 'NONE',  ( -16.12211571039999924, 1416.421578853600067, 209.3062130255779891 ) ) ;
#44351=CARTESIAN_POINT ( 'NONE',  ( -10.46078355659999914, 1480.011043621090039, 213.7014894041190018 ) ) ;
#44352=VECTOR ( 'NONE', #12026, 1000.000000000000227 ) ;
#44362=CARTESIAN_POINT ( 'NONE',  ( -15.21142308021189926, 1418.043559783950059, 203.1433581529450123 ) ) ;
#44363=CARTESIAN_POINT ( 'NONE',  ( 11.68596223914080490, 1479.116955846581277, 226.2253689540566484 ) ) ;
#44365=CARTESIAN_POINT ( 'NONE',  ( -3.750000000000000000, 1516.051704408390151, 209.1218459616989946 ) ) ;
#44369=CARTESIAN_POINT ( 'NONE',  ( 18.16492559431619824, 1429.493622211720094, 208.0479421485399882 ) ) ;
#44375=AXIS2_PLACEMENT_3D ( 'NONE', #36098, #63534, #46720 ) ;
#44379=CARTESIAN_POINT ( 'NONE',  ( -11.60766219054749904, 1481.111691938549939, 211.3876766262449962 ) ) ;
#44388=LINE ( 'NONE', #35977, #74992 ) ;
#44389=CARTESIAN_POINT ( 'NONE',  ( 4.038582018749999669, 1515.598601288590089, 208.7452592413320076 ) ) ;
#44394=CARTESIAN_POINT ( 'NONE',  ( 3.577381990939999756, 1484.682277373190118, 220.4174637111989909 ) ) ;
#44395=CARTESIAN_POINT ( 'NONE',  ( 3.844095850890000055, 1423.015328829079863, 194.0309013266989950 ) ) ;
#44397=CARTESIAN_POINT ( 'NONE',  ( 10.19122987350000109, 1454.066670175989884, 189.8474967225990042 ) ) ;
#44399=CARTESIAN_POINT ( 'NONE',  ( -5.221955786979189718, 1489.269541097040019, 185.8916489436120116 ) ) ;
#44400=CARTESIAN_POINT ( 'NONE',  ( -16.63063656698919957, 1417.185604235359961, 208.3711397553730365 ) ) ;
#44402=CARTESIAN_POINT ( 'NONE',  ( -5.249805860389999523, 1391.918259904190109, 203.6797944339089952 ) ) ;
#44403=CARTESIAN_POINT ( 'NONE',  ( 9.682511080499990541, 1436.279831232390052, 210.8541354582289955 ) ) ;
#44404=CARTESIAN_POINT ( 'NONE',  ( -12.16056974390000001, 1489.995349075190006, 210.5160904517290135 ) ) ;
#44405=DIRECTION ( 'NONE',  ( -0.000000000000000000, 1.836970198721029688E-16, 1.000000000000000000 ) ) ;
#44411=CARTESIAN_POINT ( 'NONE',  ( 10.53612673599999994, 1504.170325135620033, 214.0656471538289907 ) ) ;
#44412=CARTESIAN_POINT ( 'NONE',  ( -14.55278341820118904, 1420.461940006850000, 213.8336615198852542 ) ) ;
#44419=CARTESIAN_POINT ( 'NONE',  ( -2.117392871511483143, 1456.721470742955034, 199.8652278568989971 ) ) ;
#44423=CARTESIAN_POINT ( 'NONE',  ( 6.559971419567009576, 1464.740524891430141, 211.2618235806450002 ) ) ;
#44425=CARTESIAN_POINT ( 'NONE',  ( 0.1354934564249989926, 1469.338281066689888, 219.1920829782989983 ) ) ;
#44429=FACE_OUTER_BOUND ( 'NONE', #73061, .T. ) ;
#44433=CARTESIAN_POINT ( 'NONE',  ( 0.5120954883415810288, 1432.537586748190051, 200.6984891597549847 ) ) ;
#44439=CARTESIAN_POINT ( 'NONE',  ( 12.68571948835449881, 1500.401381075140080, 208.6071435724910259 ) ) ;
#44441=CARTESIAN_POINT ( 'NONE',  ( 10.52615244620000112, 1461.364316732390080, 209.2693891041070060 ) ) ;
#44442=CARTESIAN_POINT ( 'NONE',  ( 12.26969082843189973, 1421.718210678810010, 208.0791346696769892 ) ) ;
#44446=CARTESIAN_POINT ( 'NONE',  ( 8.659233064277689351, 1437.759822022720073, 209.5177019368769891 ) ) ;
#44452=VERTEX_POINT ( 'NONE', #75396 ) ;
#44456=CARTESIAN_POINT ( 'NONE',  ( 4.387855888652730130, 1424.007127652020017, 193.0709937674239995 ) ) ;
#44457=CARTESIAN_POINT ( 'NONE',  ( 1.326713953160000070, 1454.806608698389937, 218.4390644836289823 ) ) ;
#44463=CIRCLE ( 'NONE', #105261, 15.09021984820000029 ) ;
#44466=CARTESIAN_POINT ( 'NONE',  ( -3.701520565116230177, 1428.523979340189953, 200.5242126073240172 ) ) ;
#44470=CARTESIAN_POINT ( 'NONE',  ( -11.73826079527449906, 1482.415590711050072, 207.1601296673129866 ) ) ;
#44480=CARTESIAN_POINT ( 'NONE',  ( -12.23489994130180136, 1490.237666497490181, 209.6383001777070092 ) ) ;
#44484=VECTOR ( 'NONE', #20155, 999.9999999999998863 ) ;
#44487=CARTESIAN_POINT ( 'NONE',  ( 8.723134474349999223, 1451.781317889190177, 212.2855316608589931 ) ) ;
#44490=( BOUNDED_CURVE ( )  B_SPLINE_CURVE ( 3, ( #7879, #91890, #33619, #15703 ),
 .UNSPECIFIED., .F., .F. ) 
 B_SPLINE_CURVE_WITH_KNOTS ( ( 4, 4 ),
 ( 4.129383272231839541, 5.295394741052569465 ),
 .UNSPECIFIED. ) 
 CURVE ( )  GEOMETRIC_REPRESENTATION_ITEM ( )  RATIONAL_B_SPLINE_CURVE ( ( 1.000000000000000000, 0.8898744396721667282, 0.8898744396721667282, 1.000000000000000000 ) ) 
 REPRESENTATION_ITEM ( '' )  );
#44492=CARTESIAN_POINT ( 'NONE',  ( 20.65270365140000308, 1496.273551523690003, 204.7144476429189979 ) ) ;
#44497=CARTESIAN_POINT ( 'NONE',  ( 0.3714955681550010103, 1430.530475112889917, 199.6801487385589837 ) ) ;
#44498=CARTESIAN_POINT ( 'NONE',  ( -15.92986207429999901, 1416.139014782290133, 209.7537124246929920 ) ) ;
#44501=ORIENTED_EDGE ( 'NONE', *, *, #31522, .T. ) ;
#44503=CARTESIAN_POINT ( 'NONE',  ( 1.066336734320000090, 1485.534576645189873, 198.2622823792990232 ) ) ;
#44504=CARTESIAN_POINT ( 'NONE',  ( 9.740996373304689371, 1468.658287592850002, 206.6114599079629670 ) ) ;
#44506=CARTESIAN_POINT ( 'NONE',  ( 11.43524938500000054, 1502.933412134090077, 210.4930575720590014 ) ) ;
#44508=CARTESIAN_POINT ( 'NONE',  ( 7.338784656529999673, 1425.472921401149961, 211.8656132916889874 ) ) ;
#44510=B_SPLINE_SURFACE_WITH_KNOTS ( 'NONE', 5, 5, ( 
 ( #46151, #79191, #36615, #28771, #12518, #98164 ),
 ( #96529, #90308, #30410, #106036, #3596, #72443 ),
 ( #37720, #38807, #64599, #4135, #28213, #20897 ),
 ( #62972, #4669, #62402, #89223, #46696, #107120 ),
 ( #71922, #11428, #21978, #13039, #70815, #20350 ),
 ( #55647, #19804, #54554, #80826, #56170, #88688 ),
 ( #21436, #29860, #104928, #64046, #54009, #88140 ),
 ( #29313, #63511, #45597, #97629, #55096, #39368 ),
 ( #75192, #83559, #7415, #23100, #74090, #5779 ) ),
 .UNSPECIFIED., .F., .F., .F.,
 ( 6, 3, 6 ),
 ( 6, 6 ),
 ( 3.966820261850000140, 8.905289209860001165, 13.57492324310000065 ),
 ( 0.000000000000000000, 0.5000000000000000000 ),
 .UNSPECIFIED. ) ;
#44512=CARTESIAN_POINT ( 'NONE',  ( -11.41675737880000163, 1482.775670507890027, 205.7339588576290055 ) ) ;
#44520=CARTESIAN_POINT ( 'NONE',  ( -11.32820085813967381, 1502.497619087743260, 207.1796466604740488 ) ) ;
#44521=CARTESIAN_POINT ( 'NONE',  ( -14.87047397674367488, 1416.119917872056249, 205.0110095938617292 ) ) ;
#44525=CARTESIAN_POINT ( 'NONE',  ( -1.663182004820000115, 1450.571104617790070, 190.0477235955989954 ) ) ;
#44526=CARTESIAN_POINT ( 'NONE',  ( -8.669013948499998179, 1451.120073550389861, 205.1633857913290058 ) ) ;
#44530=CARTESIAN_POINT ( 'NONE',  ( 7.850505384759999039, 1425.611863130590109, 211.6471506695990001 ) ) ;
#44531=CARTESIAN_POINT ( 'NONE',  ( -19.86622903030000131, 1443.388330262490172, 213.1207022696590059 ) ) ;
#44536=CARTESIAN_POINT ( 'NONE',  ( 6.168648949850000562, 1454.757917196489871, 216.8023148204190136 ) ) ;
#44543=CARTESIAN_POINT ( 'NONE',  ( -4.227540919128129460, 1441.218328383909920, 201.3833897788859986 ) ) ;
#44553=EDGE_LOOP ( 'NONE', ( #74743, #94406, #41873, #106948, #63606, #88794, #85208, #67651, #64800, #38541, #41746, #106647 ) ) ;
#44554=CARTESIAN_POINT ( 'NONE',  ( -61.47464146408020014, 1511.504763168490172, 211.0950333733410105 ) ) ;
#44556=ORIENTED_EDGE ( 'NONE', *, *, #63060, .F. ) ;
#44558=CARTESIAN_POINT ( 'NONE',  ( -4.146473569399999448, 1455.609540686289847, 200.6301625394189898 ) ) ;
#44566=EDGE_CURVE ( 'NONE', #10255, #26097, #100848, .T. ) ;
#44570=CARTESIAN_POINT ( 'NONE',  ( -11.71397076299980000, 1489.483175994190105, 212.5377881273170146 ) ) ;
#44580=DIRECTION ( 'NONE',  ( 1.000000000000000000, 0.000000000000000000, 0.000000000000000000 ) ) ;
#44583=CARTESIAN_POINT ( 'NONE',  ( 10.51055398149999931, 1471.685891510089959, 212.2894657440390063 ) ) ;
#44586=CIRCLE ( 'NONE', #87513, 4.250000000000000000 ) ;
#44595=EDGE_CURVE ( 'NONE', #12262, #75688, #55252, .T. ) ;
#44600=CARTESIAN_POINT ( 'NONE',  ( -4.545982226927982595, 1508.783371655784777, 206.6339107757056581 ) ) ;
#44618=EDGE_CURVE ( 'NONE', #64533, #73065, #52687, .T. ) ;
#44624=CARTESIAN_POINT ( 'NONE',  ( -2.472546472639999937, 1422.360492461730018, 192.6709265742990169 ) ) ;
#44632=CARTESIAN_POINT ( 'NONE',  ( 3.830726099870000123, 1487.263094006890014, 197.7783884857990131 ) ) ;
#44639=CARTESIAN_POINT ( 'NONE',  ( -4.165129268920000349, 1485.181570780589936, 197.9537754904989981 ) ) ;
#44640=CIRCLE ( 'NONE', #87571, 8.102416131500007168 ) ;
#44642=B_SPLINE_SURFACE_WITH_KNOTS ( 'NONE', 5, 5, ( 
 ( #17332, #18440, #44799, #79497, #61065, #62159 ),
 ( #46458, #20652, #61599, #54854, #45900, #2260 ),
 ( #28531, #103574, #71686, #78953, #19563, #27975 ),
 ( #80590, #70563, #80035, #52640, #62729, #88977 ),
 ( #11731, #96851, #96286, #105805, #12266, #35271 ),
 ( #10066, #36374, #104681, #2804, #105240, #86777 ),
 ( #29085, #3357, #95182, #44239, #27416, #78384 ),
 ( #53194, #1692, #87905, #26875, #53769, #20119 ),
 ( #35832, #95732, #70016, #63270, #11194, #54312 ) ),
 .UNSPECIFIED., .F., .F., .F.,
 ( 6, 3, 6 ),
 ( 6, 6 ),
 ( 3.809711666910000183, 7.545169656169999683, 12.51705759590000078 ),
 ( 0.000000000000000000, 2.000000000000000000 ),
 .UNSPECIFIED. ) ;
#44644=CARTESIAN_POINT ( 'NONE',  ( -11.21334730859030060, 1470.344185174209997, 211.0928785205099985 ) ) ;
#44645=CARTESIAN_POINT ( 'NONE',  ( -6.943975500687450619, 1487.611661080929935, 219.0757446383669844 ) ) ;
#44646=CARTESIAN_POINT ( 'NONE',  ( -4.290508147279999740, 1515.379315998089851, 209.1218459617929852 ) ) ;
#44649=B_SPLINE_CURVE_WITH_KNOTS ( 'NONE', 3,
 ( #10030, #63233, #2216, #95694, #3866, #27380, #26831, #71077, #69418, #61017, #52602, #96806, #78344 ),
 .UNSPECIFIED., .F., .F.,
 ( 4, 2, 2, 1, 2, 2, 4 ),
 ( 0.000000000000000000, 0.2499999999996690425, 0.3749999999995077271, 0.4374999999994769184, 0.4687499999994652056, 0.4999999999994535482, 1.000000000000000000 ),
 .UNSPECIFIED. ) ;
#44666=CARTESIAN_POINT ( 'NONE',  ( 9.819193384514399270, 1435.740382366890117, 209.6674245052340098 ) ) ;
#44675=CARTESIAN_POINT ( 'NONE',  ( -10.95819916725939969, 1423.467759776100138, 204.3045060729880049 ) ) ;
#44677=CARTESIAN_POINT ( 'NONE',  ( 3.883237672519999517, 1472.390963103490094, 218.5418498176989885 ) ) ;
#44679=CARTESIAN_POINT ( 'NONE',  ( -11.71078717319999996, 1508.002514750790169, 208.1938872918760239 ) ) ;
#44680=CARTESIAN_POINT ( 'NONE',  ( 18.46111193188719923, 1471.786021244009817, 195.2229615556349813 ) ) ;
#44686=EDGE_CURVE ( 'NONE', #16269, #76640, #55273, .T. ) ;
#44687=CARTESIAN_POINT ( 'NONE',  ( 4.329448776040000446, 1515.064792882589927, 210.8902905144720137 ) ) ;
#44691=CARTESIAN_POINT ( 'NONE',  ( -7.806477655520000170, 1459.630680128490212, 215.5618046700689945 ) ) ;
#44695=TOROIDAL_SURFACE ( 'NONE', #16027, 10.10241613150000006, 2.000000000000000000 ) ;
#44696=ORIENTED_EDGE ( 'NONE', *, *, #18739, .F. ) ;
#44697=CARTESIAN_POINT ( 'NONE',  ( -8.223595257310000406, 1424.414600115449957, 208.7481938478530026 ) ) ;
#44703=CARTESIAN_POINT ( 'NONE',  ( -1.555742980830479905, 1496.627161338389897, 221.3873943028199847 ) ) ;
#44709=CARTESIAN_POINT ( 'NONE',  ( 0.07151796957733484728, 1487.750177387291160, 219.9735200923185801 ) ) ;
#44710=CARTESIAN_POINT ( 'NONE',  ( -17.11766752880160070, 1508.551704408389924, 212.4296625737950137 ) ) ;
#44712=CARTESIAN_POINT ( 'NONE',  ( 8.351583721560000839, 1472.370645083189856, 215.7586204441390123 ) ) ;
#44713=CARTESIAN_POINT ( 'NONE',  ( -8.986849192036190814, 1439.553571704909928, 207.2559198570870080 ) ) ;
#44718=CARTESIAN_POINT ( 'NONE',  ( 8.457168192900248016, 1436.776849429390040, 207.4172901971049896 ) ) ;
#44720=EDGE_LOOP ( 'NONE', ( #46513, #64327, #44234, #73720, #105437, #5629 ) ) ;
#44725=CARTESIAN_POINT ( 'NONE',  ( -20.30830883940000220, 1486.101309849389736, 213.0663049186690046 ) ) ;
#44728=B_SPLINE_CURVE_WITH_KNOTS ( 'NONE', 3,
 ( #3434, #106962, #96930, #3985, #20197, #30247, #38654, #71199, #80115, #64441, #105882, #29705, #71765, #63889, #21275, #89609, #53853, #47079, #98557, #87990, #87425, #104771, #62245, #73929, #49282, #82318, #91269, #5054, #64982, #39199, #99646, #22376, #75593, #66647, #109188, #108059, #32473, #91810, #31908, #47622, #48736, #48180, #99098, #82862, #83411, #49834, #56025, #21826, #74492, #90150, #108620, #66096, #13432, #24034, #56576, #107514, #73376, #100748, #31355, #5616, #65539, #100223, #22936, #67188, #6706, #33001, #109724, #75037, #6153, #14547, #81748, #13993, #57141, #30804, #90707, #92356 ),
 .UNSPECIFIED., .F., .F.,
 ( 4, 3, 3, 3, 3, 3, 3, 3, 3, 3, 3, 3, 3, 3, 3, 3, 3, 3, 3, 3, 3, 3, 3, 3, 3, 4 ),
 ( -2.999999896493359852, -2.911009666304300136, -2.785025217194290192, -2.657589902942280258, -2.529356606326549795, -2.400046307149580116, -2.270317747582839996, -2.140430810404549966, -2.010654507406799851, -1.881600297076270190, -1.753346563294839955, -1.626095977948739835, -1.500000865187030019, -1.500000000000000000, -1.410945979647750148, -1.284708769301650122, -1.157056726448419948, -1.028638210627399907, -0.8992145056076812359, -0.7694284976191689829, -0.6395434986963102197, -0.5098282392343080893, -0.3809216422371468624, -0.2528616211501977240, -0.1258403872535915902, 4.440892098500626162E-16 ),
 .UNSPECIFIED. ) ;
#44730=CARTESIAN_POINT ( 'NONE',  ( 1.968601690575629615, 1498.935401749600032, 197.9561509338619771 ) ) ;
#44744=CARTESIAN_POINT ( 'NONE',  ( 7.489828918510000655, 1422.964606643100069, 195.6540423083989992 ) ) ;
#44750=EDGE_CURVE ( 'NONE', #65500, #97980, #46815, .T. ) ;
#44754=EDGE_CURVE ( 'NONE', #18368, #59235, #56649, .T. ) ;
#44757=CARTESIAN_POINT ( 'NONE',  ( -17.11904635710000022, 1417.409719763429848, 207.3632845816489976 ) ) ;
#44761=CARTESIAN_POINT ( 'NONE',  ( 1.711055448681089940E-31, 1424.874073124720098, 209.1218459616989946 ) ) ;
#44762=CARTESIAN_POINT ( 'NONE',  ( 19.41157449629999832, 1457.417846740989944, 209.1218459616989946 ) ) ;
#44764=CIRCLE ( 'NONE', #35875, 0.9999999999999971134 ) ;
#44768=B_SPLINE_SURFACE_WITH_KNOTS ( 'NONE', 5, 1, ( 
 ( #66162, #21339 ),
 ( #22434, #74547 ),
 ( #4042, #14052 ),
 ( #90771, #65596 ),
 ( #89669, #73443 ),
 ( #21882, #12955 ),
 ( #47137, #30314 ),
 ( #20804, #13493 ),
 ( #14614, #63955 ) ),
 .UNSPECIFIED., .F., .F., .F.,
 ( 6, 3, 6 ),
 ( 2, 2 ),
 ( 0.000000000000000000, 4.040465094930000056, 8.068209695480000221 ),
 ( 0.000000000000000000, 14.00000000000000000 ),
 .UNSPECIFIED. ) ;
#44770=CARTESIAN_POINT ( 'NONE',  ( -17.20183000400000140, 1421.414648929949863, 201.7791951163490012 ) ) ;
#44779=CARTESIAN_POINT ( 'NONE',  ( -15.90172418499818541, 1420.263238377089237, 209.8660166653201600 ) ) ;
#44786=CARTESIAN_POINT ( 'NONE',  ( 4.077869218320000044, 1442.578371693189865, 217.0097321978689990 ) ) ;
#44790=CARTESIAN_POINT ( 'NONE',  ( -4.878146142590000345, 1474.403035727189945, 198.7818668649990173 ) ) ;
#44793=CARTESIAN_POINT ( 'NONE',  ( -9.573057217335119162, 1423.428048935199740, 192.3355792750039939 ) ) ;
#44796=CARTESIAN_POINT ( 'NONE',  ( 0.1548802053370030019, 1489.973220511089949, 188.2279286174990034 ) ) ;
#44799=CARTESIAN_POINT ( 'NONE',  ( -3.163732031489999930, 1432.489031102390072, 217.0770860277189911 ) ) ;
#44801=CARTESIAN_POINT ( 'NONE',  ( -10.96092256686609900, 1471.477682962149856, 206.8110093702159986 ) ) ;
#44806=CARTESIAN_POINT ( 'NONE',  ( 9.931488721813659382, 1423.381267080859971, 209.2494160290190166 ) ) ;
#44808=CARTESIAN_POINT ( 'NONE',  ( 10.98780082597929919, 1490.670427006609998, 209.0313451347890066 ) ) ;
#44810=ORIENTED_EDGE ( 'NONE', *, *, #20207, .T. ) ;
#44832=CARTESIAN_POINT ( 'NONE',  ( -3.685264706689999947, 1496.073670527689728, 219.7127572917990221 ) ) ;
#44845=CARTESIAN_POINT ( 'NONE',  ( -1.121951540329999775, 1488.104705274990010, 219.9473760328990011 ) ) ;
#44847=ADVANCED_FACE ( 'NONE', ( #107191 ), #59072, .F. ) ;
#44848=CARTESIAN_POINT ( 'NONE',  ( -4.992349863779999453, 1391.620913471789891, 214.4361776263990009 ) ) ;
#44852=CARTESIAN_POINT ( 'NONE',  ( 10.90988536168999978, 1460.796490171650021, 208.2422925045810018 ) ) ;
#44857=CARTESIAN_POINT ( 'NONE',  ( 9.047070330427949614, 1452.614645995950013, 211.8941571659140095 ) ) ;
#44858=CARTESIAN_POINT ( 'NONE',  ( 8.855603127469999336, 1423.529354507180187, 196.4827216600990027 ) ) ;
#44859=EDGE_CURVE ( 'NONE', #69308, #11716, #34345, .T. ) ;
#44861=CARTESIAN_POINT ( 'NONE',  ( -3.364077551112700348, 1507.415397232589839, 221.5352637752980058 ) ) ;
#44862=CARTESIAN_POINT ( 'NONE',  ( -9.843249962089998917, 1461.614812224390107, 208.6141224610979918 ) ) ;
#44868=CARTESIAN_POINT ( 'NONE',  ( 9.172898573127410415, 1450.102442297790049, 208.3180252651680178 ) ) ;
#44869=CARTESIAN_POINT ( 'NONE',  ( 1.702379247829999942, 1501.792222158089999, 230.4488007676989980 ) ) ;
#44875=B_SPLINE_CURVE_WITH_KNOTS ( 'NONE', 3,
 ( #49274, #83403, #22927, #108611, #73921, #6699, #40854, #31900, #100741, #57132, #84509, #75585, #75029, #31346, #57687, #65530, #99637, #91801, #91259, #49827, #109180, #24025, #14539, #48728, #82854, #58225, #92349, #16181, #15621, #73367, #83957, #107506, #24577, #7257, #109717, #101282, #30796, #17273, #18944, #7798, #9461, #59882, #18388 ),
 .UNSPECIFIED., .F., .F.,
 ( 4, 3, 3, 3, 3, 3, 3, 3, 3, 3, 3, 3, 3, 3, 4 ),
 ( 2.099667498829999878E-15, 1.406846277637760156, 2.814198252419170210, 4.220686603073059651, 5.623444216349149372, 7.022781117988579958, 8.415638966051240288, 8.942376872057339554, 10.31946110557949936, 11.69383206961379962, 13.06413089926859961, 14.42602073298239773, 15.78206364908349890, 17.12804210909719771, 17.88475318529999925 ),
 .UNSPECIFIED. ) ;
#44879=CARTESIAN_POINT ( 'NONE',  ( -6.528218896545719296, 1508.485824417290132, 219.7230302621430269 ) ) ;
#44882=CARTESIAN_POINT ( 'NONE',  ( -9.541786836099248603, 1471.456755149039736, 212.5898191071979966 ) ) ;
#44885=CARTESIAN_POINT ( 'NONE',  ( 9.157303188274740435, 1450.042022675190083, 208.2002544115800049 ) ) ;
#44886=CARTESIAN_POINT ( 'NONE',  ( -6.694418385159999652, 1473.791160286789818, 199.7891180969089930 ) ) ;
#44887=CARTESIAN_POINT ( 'NONE',  ( -2.434348319423109697, 1422.283838751350004, 192.8362627702539953 ) ) ;
#44889=CARTESIAN_POINT ( 'NONE',  ( 8.360704762653028865, 1424.462288153377131, 195.7412347175665559 ) ) ;
#44891=CARTESIAN_POINT ( 'NONE',  ( 10.78499426627680080, 1469.831216462720022, 205.6638516619669872 ) ) ;
#44893=CARTESIAN_POINT ( 'NONE',  ( -9.937510298460209057, 1439.652175453890095, 208.0161710764309930 ) ) ;
#44902=EDGE_CURVE ( 'NONE', #2433, #15049, #25872, .T. ) ;
#44904=CARTESIAN_POINT ( 'NONE',  ( -1.251490820319690167, 1515.089511802750167, 204.7930444736340121 ) ) ;
#44906=CARTESIAN_POINT ( 'NONE',  ( -15.79765598458050491, 1415.826759071379229, 209.7038822556229434 ) ) ;
#44909=FACE_OUTER_BOUND ( 'NONE', #63732, .T. ) ;
#44910=CARTESIAN_POINT ( 'NONE',  ( 1.302631559684990004, 1430.876257361340095, 199.7563870752120181 ) ) ;
#44917=CARTESIAN_POINT ( 'NONE',  ( -6.769446762680000340, 1477.849490981190229, 218.6333586432590153 ) ) ;
#44918=DIRECTION ( 'NONE',  ( -0.9991331916196766194, 0.04162763470901477414, -7.370489309664139796E-05 ) ) ;
#44930=CARTESIAN_POINT ( 'NONE',  ( -16.32386383359999726, 1416.417362032049823, 209.4515642215840217 ) ) ;
#44933=CARTESIAN_POINT ( 'NONE',  ( 18.09194291044959613, 1429.328450707060028, 207.2811966920800160 ) ) ;
#44934=SPHERICAL_SURFACE ( 'NONE', #22825, 0.5000000000000000000 ) ;
#44938=CARTESIAN_POINT ( 'NONE',  ( -13.59512978074699951, 1507.703334056939866, 209.3532892538999874 ) ) ;
#44949=CARTESIAN_POINT ( 'NONE',  ( -8.752495015159368563, 1495.068115196657800, 202.1315847339255356 ) ) ;
#44953=CLOSED_SHELL ( 'NONE', ( #103341, #78275, #55892, #1415, #16716, #10437, #32090, #50326, #44254, #16482, #41997, #79005, #78874, #42169, #98700, #62851, #93080, #65449, #76023, #9780, #72017, #104540, #26349, #109046, #67933, #107495, #73044, #102068, #7710, #71322, #34310, #66560, #96671, #26719, #65819, #90864, #23607, #49818, #8524, #58177, #33307, #98730, #62666, #15249, #6259, #39925, #54222, #52080, #34469, #7156, #39788, #63269, #99538, #34241, #79549, #69861, #51042, #81663, #30586, #21260, #87158, #38895, #72296, #71565, #14568, #46560, #63066, #108048, #78824, #109570, #105768, #87674, #22284, #14445, #7917, #70803, #101106, #61960, #93467, #8880, #46613, #67888, #6171, #22019, #64830, #936, #25551, #101428, #30937, #91062, #66719, #88224, #3156, #103527, #3180, #7808, #86372, #83616, #26121, #61105, #67076, #29038, #46112, #106288, #63904, #40601, #93830, #81053, #98166, #21933, #109181, #84349, #97414, #98823, #90455, #42528, #59753, #91216, #106119, #70427, #18804, #25706, #57398, #74655, #59902, #78353, #33620, #81721, #77480, #106389, #84506, #80856, #35749, #106422, #85255, #4854, #45357, #108819, #110353, #51383, #60360, #77118, #100094, #35789, #46161, #63953, #87145, #91196, #78153, #20599, #71454, #36952, #21212, #100317, #31335, #75696, #72132, #55852, #65773, #13364, #76069, #73407, #76783, #24468, #38627, #99489, #8501, #89722, #91472, #47477, #7635, #53561, #37189, #54240, #5756, #28265, #17083, #65225, #102374, #50678, #106079, #31556, #62458, #1496, #16007, #92554, #16012, #58976, #10568, #63353, #81234, #67946, #50845, #99541, #29821, #88740, #63827, #13714, #102769, #67831, #22071, #42046, #20916, #79752, #96818, #104851, #42956, #104094, #1885, #39092, #99996, #97378, #45971, #101913, #77069, #76203, #47500, #4994, #68081, #4885, #64650, #40142, #106121, #68396, #54516, #37224, #83564, #84510, #43834, #19569, #70679, #65972, #61743, #101920, #97684, #29926, #42714, #25722, #109038, #58973, #80848, #50636, #73673, #39990, #59716, #8248, #49327, #108937, #102058, #83028, #97309, #90694, #89365, #9654, #80213, #70797, #39216, #6567, #65893, #22178, #102240, #29619, #49374, #103572, #37146, #36620, #23411, #84337, #40582, #14319, #2516, #46915, #36367, #54155, #44847, #65469, #88505, #19893, #67226, #89674, #71554, #105269, #9935, #64873, #94566, #5913, #33815, #40506, #43199, #9166, #41178, #87077, #86537, #10469, #94593, #104089, #66897, #17211, #30364, #44042, #51024, #31620, #75204, #70923, #33826, #36515, #26215, #37024, #95122, #107523, #6413, #88543 ) ) ;
#44956=CARTESIAN_POINT ( 'NONE',  ( 3.242267180889999878, 1423.555505585929950, 193.2269609960989953 ) ) ;
#44959=CARTESIAN_POINT ( 'NONE',  ( 18.74597378714840090, 1457.928134532490049, 220.6238524344490202 ) ) ;
#44965=CARTESIAN_POINT ( 'NONE',  ( -10.90539778630000001, 1489.991646564889834, 212.3805117938089779 ) ) ;
#44972=CARTESIAN_POINT ( 'NONE',  ( 7.656493703591820577, 1504.159369564410099, 219.4142504822630144 ) ) ;
#44973=CARTESIAN_POINT ( 'NONE',  ( -13.77489446762966097, 1421.087469475355419, 210.6290704798021522 ) ) ;
#44976=ORIENTED_EDGE ( 'NONE', *, *, #27798, .T. ) ;
#44984=CARTESIAN_POINT ( 'NONE',  ( 5.258395203887199720, 1466.657720361110023, 214.1037399434610222 ) ) ;
#44992=CARTESIAN_POINT ( 'NONE',  ( -3.365241614647759949, 1429.250033114370126, 207.0884890221589956 ) ) ;
#44994=( BOUNDED_CURVE ( )  B_SPLINE_CURVE ( 3, ( #94277, #16446, #101562, #103220 ),
 .UNSPECIFIED., .F., .T. ) 
 B_SPLINE_CURVE_WITH_KNOTS ( ( 4, 4 ),
 ( 1.003383811351443944, 2.138208849194395356 ),
 .UNSPECIFIED. ) 
 CURVE ( )  GEOMETRIC_REPRESENTATION_ITEM ( )  RATIONAL_B_SPLINE_CURVE ( ( 1.000000000000000000, 0.8955296286887992618, 0.8955296286887992618, 1.000000000000000000 ) ) 
 REPRESENTATION_ITEM ( '' )  );
#44998=CARTESIAN_POINT ( 'NONE',  ( 0.2579780539924840244, 1432.430230534230077, 200.6906244575169751 ) ) ;
#45001=ORIENTED_EDGE ( 'NONE', *, *, #79567, .T. ) ;
#45004=CARTESIAN_POINT ( 'NONE',  ( 12.68026019944470129, 1500.377008822790231, 208.5091319790680018 ) ) ;
#45006=CARTESIAN_POINT ( 'NONE',  ( 9.694557698469999707, 1462.254025601890135, 208.2085395626110085 ) ) ;
#45010=CARTESIAN_POINT ( 'NONE',  ( 3.168476225200000052, 1465.480445073689907, 199.6310402015890020 ) ) ;
#45020=EDGE_CURVE ( 'NONE', #19394, #92807, #96172, .T. ) ;
#45025=CARTESIAN_POINT ( 'NONE',  ( 4.647513230146739893, 1424.072963496759940, 193.1398315391210190 ) ) ;
#45031=CARTESIAN_POINT ( 'NONE',  ( 0.1473420581360029846, 1491.995248389390099, 188.1393154328989965 ) ) ;
#45038=CARTESIAN_POINT ( 'NONE',  ( -11.59678483583009978, 1482.606145766309965, 206.4252640944189920 ) ) ;
#45049=AXIS2_PLACEMENT_3D ( 'NONE', #97672, #37223, #96580 ) ;
#45068=CARTESIAN_POINT ( 'NONE',  ( -1.351834365089999990, 1508.907723353190022, 220.8330489178990206 ) ) ;
#45070=ORIENTED_EDGE ( 'NONE', *, *, #27023, .T. ) ;
#45071=DIRECTION ( 'NONE',  ( -1.000000000000000000, 0.000000000000000000, 0.000000000000000000 ) ) ;
#45073=CARTESIAN_POINT ( 'NONE',  ( 8.227317073306119610, 1467.971793790919946, 202.5226687861409971 ) ) ;
#45076=CARTESIAN_POINT ( 'NONE',  ( 9.573136282580000156, 1493.454997221290114, 189.9048530042990137 ) ) ;
#45082=CARTESIAN_POINT ( 'NONE',  ( -10.56986559679999971, 1482.340628544289984, 205.9074541195790005 ) ) ;
#45091=CARTESIAN_POINT ( 'NONE',  ( -3.380779445240819747, 1436.568323192200069, 227.3158197219400165 ) ) ;
#45095=CARTESIAN_POINT ( 'NONE',  ( -9.783936650027678539, 1438.409968310599879, 210.7790528106160082 ) ) ;
#45097=B_SPLINE_CURVE_WITH_KNOTS ( 'NONE', 3,
 ( #100581, #75414, #84875, #49656, #101668, #24958, #25515, #26064, #109004, #84340, #59708, #51290, #50213, #68669, #8171, #92191, #83791, #109553, #42340, #32825, #7086, #110644, #59167, #68127, #16550, #67014, #6535, #101122, #24419, #50740, #7628 ),
 .UNSPECIFIED., .F., .F.,
 ( 4, 3, 3, 3, 3, 3, 3, 3, 3, 3, 4 ),
 ( -31.85201398510000104, -31.81690162971739966, -31.29106762226110305, -30.73012125942219797, -29.75465476144709953, -29.12069379509160072, -28.57063748067939812, -28.09167849124629868, -27.34815097616279900, -26.12566447164610040, -25.28925868605369942 ),
 .UNSPECIFIED. ) ;
#45100=CARTESIAN_POINT ( 'NONE',  ( 7.898683012529999381, 1423.849047743189885, 212.3277966039590012 ) ) ;
#45101=CARTESIAN_POINT ( 'NONE',  ( -19.58884347349999899, 1465.811382978989968, 204.1485388398990040 ) ) ;
#45106=CARTESIAN_POINT ( 'NONE',  ( 7.122515158009999681, 1452.871264857790266, 215.2372064891289654 ) ) ;
#45110=DIRECTION ( 'NONE',  ( -1.000000000000000000, 0.000000000000000000, 0.000000000000000000 ) ) ;
#45115=CARTESIAN_POINT ( 'NONE',  ( -2.054137843158699628, 1464.087208514039958, 199.3848561270889945 ) ) ;
#45121=CARTESIAN_POINT ( 'NONE',  ( -11.87328627558470018, 1482.014094172719979, 208.6022272904490080 ) ) ;
#45132=CARTESIAN_POINT ( 'NONE',  ( 4.966881216750000050, 1424.596682289360160, 209.0258764897109813 ) ) ;
#45140=CARTESIAN_POINT ( 'NONE',  ( 9.565724157538609163, 1462.394397289459903, 207.2652911505539919 ) ) ;
#45151=CIRCLE ( 'NONE', #77345, 8.102416131500007168 ) ;
#45154=CARTESIAN_POINT ( 'NONE',  ( 5.811960035336429797, 1424.824675250879864, 192.0933432259219842 ) ) ;
#45158=ORIENTED_EDGE ( 'NONE', *, *, #80934, .F. ) ;
#45163=CARTESIAN_POINT ( 'NONE',  ( -2.810337449649999986, 1429.891394031290019, 201.1534787522990086 ) ) ;
#45173=CARTESIAN_POINT ( 'NONE',  ( 11.16829484163620023, 1470.316420363600173, 207.0405923250029900 ) ) ;
#45181=CARTESIAN_POINT ( 'NONE',  ( 2.774825831029999801, 1441.953158150089848, 217.9119417670190160 ) ) ;
#45187=CARTESIAN_POINT ( 'NONE',  ( -3.363422329630640029, 1464.767212871569882, 198.6335063457190131 ) ) ;
#45196=CARTESIAN_POINT ( 'NONE',  ( -4.114244456749999834, 1483.278371519489838, 199.2835753141889938 ) ) ;
#45201=CARTESIAN_POINT ( 'NONE',  ( -11.04302901312609997, 1470.202560320620023, 211.8432240382399812 ) ) ;
#45202=CARTESIAN_POINT ( 'NONE',  ( -10.72577289612640072, 1489.848996007629921, 212.9502564920910004 ) ) ;
#45203=CARTESIAN_POINT ( 'NONE',  ( -11.77905477449999871, 1483.168199375790209, 228.2502073304989949 ) ) ;
#45216=VERTEX_POINT ( 'NONE', #106180 ) ;
#45219=CARTESIAN_POINT ( 'NONE',  ( -20.64559663309999848, 1487.101925495689784, 207.0915929621590124 ) ) ;
#45224=CARTESIAN_POINT ( 'NONE',  ( 8.725481330957579829, 1436.236045380599990, 208.5030100741789738 ) ) ;
#45232=CARTESIAN_POINT ( 'NONE',  ( -16.20918397789189669, 1420.752430442280001, 203.3157397894999860 ) ) ;
#45233=CARTESIAN_POINT ( 'NONE',  ( -11.40503443455700072, 1490.739836633030109, 209.6941760169060274 ) ) ;
#45234=CARTESIAN_POINT ( 'NONE',  ( 4.551482758439999721, 1472.189735705889916, 218.2242021444390048 ) ) ;
#45235=ORIENTED_EDGE ( 'NONE', *, *, #53238, .F. ) ;
#45238=CARTESIAN_POINT ( 'NONE',  ( -17.55007421918869781, 1487.029478167789875, 194.9701128493070144 ) ) ;
#45241=FACE_OUTER_BOUND ( 'NONE', #21405, .T. ) ;
#45243=CARTESIAN_POINT ( 'NONE',  ( -4.623067421070000016, 1470.601194648889987, 189.6761541078989808 ) ) ;
#45249=CARTESIAN_POINT ( 'NONE',  ( -9.336750167439999970, 1459.654649201290113, 211.6846149272190303 ) ) ;
#45252=B_SPLINE_CURVE_WITH_KNOTS ( 'NONE', 3,
 ( #10770, #18579, #44379, #72341, #95864, #105378, #20791, #46039, #28107, #20247, #88584, #54992, #54448, #78522, #53333, #80168, #46589, #106470, #29755, #79088, #2396, #104820, #57612, #23954, #15003 ),
 .UNSPECIFIED., .F., .F.,
 ( 4, 3, 3, 3, 3, 3, 3, 3, 4 ),
 ( -7.627880006969999904, -7.586449332979929849, -6.861103662591740537, -6.094327318213479394, -5.380600910333019904, -5.288135639796470500, -4.615464934644060158, -3.827473140728220091, -3.133321433589999927 ),
 .UNSPECIFIED. ) ;
#45255=CARTESIAN_POINT ( 'NONE',  ( -8.440966142320000642, 1423.593311052290119, 209.8619391807339980 ) ) ;
#45257=VERTEX_POINT ( 'NONE', #90469 ) ;
#45259=CARTESIAN_POINT ( 'NONE',  ( 7.589792638401371860, 1507.508085020990166, 200.2016081335497972 ) ) ;
#45266=CARTESIAN_POINT ( 'NONE',  ( -18.08355418696270078, 1508.551704408389924, 210.9733555596099848 ) ) ;
#45268=CARTESIAN_POINT ( 'NONE',  ( 8.068531700010000307, 1471.978696959290119, 215.6387874036589949 ) ) ;
#45269=CARTESIAN_POINT ( 'NONE',  ( 4.962911793259999982, 1424.817228554909889, 209.2445736825380038 ) ) ;
#45270=ORIENTED_EDGE ( 'NONE', *, *, #46868, .T. ) ;
#45274=CARTESIAN_POINT ( 'NONE',  ( 9.769960542006101534, 1435.154130655169865, 208.2355606574099909 ) ) ;
#45279=CARTESIAN_POINT ( 'NONE',  ( 0.4200850585664279713, 1467.359727432810132, 220.1963459426220027 ) ) ;
#45292=CARTESIAN_POINT ( 'NONE',  ( 4.246466822330620339, 1508.879013277289914, 205.3739042749660086 ) ) ;
#45310=VERTEX_POINT ( 'NONE', #77028 ) ;
#45314=CARTESIAN_POINT ( 'NONE',  ( -8.473114352260500581, 1484.074700721370164, 200.7533846890079872 ) ) ;
#45317=CARTESIAN_POINT ( 'NONE',  ( -4.327096512618029855, 1515.154622198479956, 208.8658927233350084 ) ) ;
#45324=DIRECTION ( 'NONE',  ( 1.000000000000000000, 1.810374147724000060E-32, 1.224646799147351975E-16 ) ) ;
#45325=CARTESIAN_POINT ( 'NONE',  ( 14.32856980210140030, 1427.588994036270151, 195.3328737750769903 ) ) ;
#45331=CARTESIAN_POINT ( 'NONE',  ( 12.12948552422830062, 1501.448489250790089, 211.6227393280869933 ) ) ;
#45334=CARTESIAN_POINT ( 'NONE',  ( -15.64806741621447017, 1420.335678436578291, 210.4039352086240626 ) ) ;
#45340=CARTESIAN_POINT ( 'NONE',  ( -1766.069695707609526, -8382.262153571264207, -1964.859607327509593 ) ) ;
#45341=CARTESIAN_POINT ( 'NONE',  ( 9.155703581353909826, 1451.066167471900144, 210.4353983151760019 ) ) ;
#45343=CARTESIAN_POINT ( 'NONE',  ( 3.212280145430000289, 1441.426961928390028, 218.1016817799990122 ) ) ;
#45350=CARTESIAN_POINT ( 'NONE',  ( -4.379874935479580955, 1508.551704408389924, 219.7958719070109908 ) ) ;
#45357=ADVANCED_FACE ( 'NONE', ( #62459 ), #11460, .T. ) ;
#45359=CARTESIAN_POINT ( 'NONE',  ( -17.88808968309999869, 1422.733202112150138, 207.9839376467890020 ) ) ;
#45361=CARTESIAN_POINT ( 'NONE',  ( 18.79226589730000185, 1456.307606824690083, 213.7887498653890077 ) ) ;
#45366=CARTESIAN_POINT ( 'NONE',  ( 11.00095395210620097, 1490.665236598310003, 207.4715718885979925 ) ) ;
#45373=CARTESIAN_POINT ( 'NONE',  ( 12.22507006113399974, 1427.248780726589985, 207.5705273738180097 ) ) ;
#45385=CARTESIAN_POINT ( 'NONE',  ( 1.402559146139999990, 1498.352971756790112, 197.8773470515990027 ) ) ;
#45389=ORIENTED_EDGE ( 'NONE', *, *, #40030, .T. ) ;
#45397=CARTESIAN_POINT ( 'NONE',  ( 2.459010662519999890, 1485.097423333889992, 220.7348024981990307 ) ) ;
#45406=EDGE_LOOP ( 'NONE', ( #15874, #6324, #18185, #20750, #1404, #25662, #55842, #28598, #95637, #100478, #81017, #77171 ) ) ;
#45407=CARTESIAN_POINT ( 'NONE',  ( 9.072576645759729885, 1451.848759158979874, 211.1174303628249902 ) ) ;
#45411=CARTESIAN_POINT ( 'NONE',  ( -11.03352341481849841, 1462.446812322350070, 208.7213867630900097 ) ) ;
#45418=CARTESIAN_POINT ( 'NONE',  ( -0.3613963699280030029, 1502.117394456789953, 230.5447891057989978 ) ) ;
#45419=EDGE_CURVE ( 'NONE', #60672, #51752, #100639, .T. ) ;
#45421=VERTEX_POINT ( 'NONE', #33216 ) ;
#45426=ORIENTED_EDGE ( 'NONE', *, *, #20166, .T. ) ;
#45430=CARTESIAN_POINT ( 'NONE',  ( -9.535170673477109560, 1471.930435161360037, 212.6674250506980002 ) ) ;
#45434=CARTESIAN_POINT ( 'NONE',  ( -12.66657887843499886, 1502.203781315570041, 210.6663731483399999 ) ) ;
#45435=CARTESIAN_POINT ( 'NONE',  ( 9.796230887720000169, 1493.843361169789887, 216.7872332751290116 ) ) ;
#45439=CARTESIAN_POINT ( 'NONE',  ( -14.95480896039999941, 1503.828903730489856, 208.7757359552959997 ) ) ;
#45453=CARTESIAN_POINT ( 'NONE',  ( -14.45258097049999968, 1415.677402202029953, 212.7925583659589677 ) ) ;
#45454=CARTESIAN_POINT ( 'NONE',  ( 12.82765434203870036, 1421.015154487590053, 203.4288627072589861 ) ) ;
#45456=CARTESIAN_POINT ( 'NONE',  ( -16.98474706396019940, 1418.194805350959768, 204.1434201589789836 ) ) ;
#45460=CARTESIAN_POINT ( 'NONE',  ( 0.8227887822411580343, 1430.698630372429989, 199.7159915099159946 ) ) ;
#45468=CARTESIAN_POINT ( 'NONE',  ( -6.409121316630000287, 1477.410212878089851, 217.9096042521290144 ) ) ;
#45475=B_SPLINE_CURVE_WITH_KNOTS ( 'NONE', 5,
 ( #99960, #108933, #107269, #106710, #98865, #82631 ),
 .UNSPECIFIED., .F., .F.,
 ( 6, 6 ),
 ( 367.7284095229999821, 372.8603425570000240 ),
 .UNSPECIFIED. ) ;
#45488=ORIENTED_EDGE ( 'NONE', *, *, #9842, .T. ) ;
#45494=EDGE_CURVE ( 'NONE', #8084, #3002, #94384, .T. ) ;
#45496=B_SPLINE_CURVE_WITH_KNOTS ( 'NONE', 3,
 ( #84118, #30964, #108221, #48899, #58935, #24200 ),
 .UNSPECIFIED., .F., .F.,
 ( 4, 2, 4 ),
 ( 0.000000000000000000, 0.2372834985116590023, 0.4746949337468490127 ),
 .UNSPECIFIED. ) ;
#45507=DIRECTION ( 'NONE',  ( -0.8962072375315806028, 8.149454628506528759E-17, 0.4436356471204868090 ) ) ;
#45513=CARTESIAN_POINT ( 'NONE',  ( -0.6756013102099980294, 1422.780067699609845, 192.4727110829989840 ) ) ;
#45515=CARTESIAN_POINT ( 'NONE',  ( -8.401877990506491756, 1449.017984408099892, 191.5381300880989954 ) ) ;
#45516=CARTESIAN_POINT ( 'NONE',  ( 19.02097995950469667, 1454.195557636890044, 200.7033899366429921 ) ) ;
#45522=CARTESIAN_POINT ( 'NONE',  ( -11.12919673650000085, 1490.198289314490012, 211.5851026735989819 ) ) ;
#45525=CARTESIAN_POINT ( 'NONE',  ( 9.717824533310780666, 1463.678478211699939, 210.3770741684630252 ) ) ;
#45529=EDGE_CURVE ( 'NONE', #100109, #82048, #11894, .T. ) ;
#45530=CARTESIAN_POINT ( 'NONE',  ( -4.237077472001714362, 1454.676950755804683, 200.7191022525509823 ) ) ;
#45531=CARTESIAN_POINT ( 'NONE',  ( -10.65952630784540389, 1422.351730238593291, 210.6396139690640439 ) ) ;
#45532=CONICAL_SURFACE ( 'NONE', #38291, 7.500000000000000000, 0.02617993877989872875 ) ;
#45538=CARTESIAN_POINT ( 'NONE',  ( -7.649966146998510297, 1507.551694032670184, 219.0282776340299904 ) ) ;
#45542=CARTESIAN_POINT ( 'NONE',  ( 15.76562750197309981, 1459.955010096749902, 221.8162589312199771 ) ) ;
#45544=CARTESIAN_POINT ( 'NONE',  ( -1.511034998550000008, 1467.833985848489874, 220.1514606783989905 ) ) ;
#45549=CARTESIAN_POINT ( 'NONE',  ( -3.986282491261569305, 1428.493128888279898, 206.6345495674519839 ) ) ;
#45552=CARTESIAN_POINT ( 'NONE',  ( -8.229011145687781692, 1439.448126226759996, 228.6152129487579998 ) ) ;
#45553=CARTESIAN_POINT ( 'NONE',  ( -10.80389986116539980, 1440.331015950379879, 224.4356702096399943 ) ) ;
#45555=VERTEX_POINT ( 'NONE', #96451 ) ;
#45561=FACE_OUTER_BOUND ( 'NONE', #100148, .T. ) ;
#45565=CARTESIAN_POINT ( 'NONE',  ( 8.660201460965680553, 1437.683719626410038, 209.3645222499649776 ) ) ;
#45576=CARTESIAN_POINT ( 'NONE',  ( -2.086548178679999754, 1515.551704408389924, 205.2922258481490303 ) ) ;
#45577=CARTESIAN_POINT ( 'NONE',  ( -4.391745902125429701, 1433.897785981300103, 217.6620401040709964 ) ) ;
#45581=CARTESIAN_POINT ( 'NONE',  ( -6.454495265129999382, 1508.590068290189947, 219.7017392546990209 ) ) ;
#45583=CARTESIAN_POINT ( 'NONE',  ( 0.8344953249080009350, 1498.972540960489823, 200.5991869134590218 ) ) ;
#45590=CARTESIAN_POINT ( 'NONE',  ( -11.63852489204760055, 1482.558018235800091, 206.6148454379789996 ) ) ;
#45597=CARTESIAN_POINT ( 'NONE',  ( -15.53829606909999939, 1415.702944931670118, 208.9765912623510076 ) ) ;
#45604=CARTESIAN_POINT ( 'NONE',  ( -9.103468112560660686, 1449.499701819690017, 210.3008494512589834 ) ) ;
#45610=CARTESIAN_POINT ( 'NONE',  ( -0.7322251554670010654, 1515.253704548090127, 213.4463482420090088 ) ) ;
#45616=EDGE_CURVE ( 'NONE', #101374, #31336, #33817, .T. ) ;
#45623=CARTESIAN_POINT ( 'NONE',  ( 0.9035508022849989551, 1507.847498519289957, 220.8498822601989957 ) ) ;
#45627=CARTESIAN_POINT ( 'NONE',  ( -574.7977070613925434, -8383.748406600810995, -1686.503645000492497 ) ) ;
#45628=APPLICATION_CONTEXT ( 'automotive_design' ) ;
#45629=CARTESIAN_POINT ( 'NONE',  ( 9.905302590843319877, 1468.559873349059899, 207.6662433566980042 ) ) ;
#45644=ORIENTED_EDGE ( 'NONE', *, *, #9346, .F. ) ;
#45645=CARTESIAN_POINT ( 'NONE',  ( -11.33909794091723278, 1503.312387898769657, 207.0376778566603377 ) ) ;
#45646=CARTESIAN_POINT ( 'NONE',  ( -13.58309651533389939, 1508.536267668799837, 210.1614309259379922 ) ) ;
#45647=CARTESIAN_POINT ( 'NONE',  ( -13.81390074910000010, 1504.365568754290052, 226.5328680220989952 ) ) ;
#45652=CARTESIAN_POINT ( 'NONE',  ( -9.135474993299999014, 1450.134483540889960, 207.9596447350990047 ) ) ;
#45654=CARTESIAN_POINT ( 'NONE',  ( 7.579106951069999987, 1425.391851912110042, 212.0588301213689988 ) ) ;
#45655=CARTESIAN_POINT ( 'NONE',  ( 9.992001554820001630, 1491.422527302990147, 188.4943246008990059 ) ) ;
#45670=EDGE_CURVE ( 'NONE', #54763, #21797, #99251, .T. ) ;
#45689=CARTESIAN_POINT ( 'NONE',  ( 8.136848112800000976, 1426.803698133580156, 211.7678967111889961 ) ) ;
#45700=EDGE_LOOP ( 'NONE', ( #92827, #42819, #52650, #72251 ) ) ;
#45701=FACE_OUTER_BOUND ( 'NONE', #30553, .T. ) ;
#45714=DIRECTION ( 'NONE',  ( 0.000000000000000000, 1.000000000000000000, -1.836970198721029688E-16 ) ) ;
#45719=CARTESIAN_POINT ( 'NONE',  ( -2.669930443950000232, 1429.978190405989835, 201.1023880675990085 ) ) ;
#45736=CARTESIAN_POINT ( 'NONE',  ( 18.16442922799999948, 1430.105938726390150, 210.9087875679190063 ) ) ;
#45738=CARTESIAN_POINT ( 'NONE',  ( 3.187857858790000165, 1443.094984070389955, 217.4314004907489846 ) ) ;
#45748=CARTESIAN_POINT ( 'NONE',  ( 4.329415431088969868, 1515.066066275059939, 207.4128929697799890 ) ) ;
#45751=CARTESIAN_POINT ( 'NONE',  ( 12.32716646574370145, 1492.190914138330072, 209.5898718627249764 ) ) ;
#45754=CARTESIAN_POINT ( 'NONE',  ( -4.927726023229999974, 1485.007261019890166, 198.2757096449989831 ) ) ;
#45760=CARTESIAN_POINT ( 'NONE',  ( -5.169211785684260541, 1487.151124505699954, 220.0115435702170146 ) ) ;
#45761=CARTESIAN_POINT ( 'NONE',  ( 8.129467950829999623, 1461.711574958590063, 228.8738014342989970 ) ) ;
#45767=CARTESIAN_POINT ( 'NONE',  ( 4.085147076609999317, 1428.826406437490050, 216.3215770461389980 ) ) ;
#45768=CARTESIAN_POINT ( 'NONE',  ( -18.80814933326179883, 1444.056498683949940, 209.9870952034320055 ) ) ;
#45773=EDGE_LOOP ( 'NONE', ( #18809, #18476, #93726, #60878 ) ) ;
#45786=CARTESIAN_POINT ( 'NONE',  ( 1.700207153268540106, 1515.066230056300128, 213.4512571039940099 ) ) ;
#45788=CARTESIAN_POINT ( 'NONE',  ( -9.818988496689140533, 1479.475980022059730, 215.4970472198330071 ) ) ;
#45790=DIRECTION ( 'NONE',  ( -0.9824080081115912355, 0.000000000000000000, -0.1867471702549089174 ) ) ;
#45793=CARTESIAN_POINT ( 'NONE',  ( -2.487923763832169843, 1508.731372606449895, 213.6767948502499905 ) ) ;
#45795=CARTESIAN_POINT ( 'NONE',  ( -5.549738551720860613, 1491.048330316449892, 185.8720954308039950 ) ) ;
#45800=CARTESIAN_POINT ( 'NONE',  ( 4.328818125147670060, 1515.088876468540093, 210.3869497035339862 ) ) ;
#45803=CARTESIAN_POINT ( 'NONE',  ( -6.609057684309999736, 1459.054199521789997, 216.6505361422790088 ) ) ;
#45813=CARTESIAN_POINT ( 'NONE',  ( 1.039074886133859899, 1495.944500751950045, 221.4190036890230147 ) ) ;
#45815=CARTESIAN_POINT ( 'NONE',  ( 4.253676957470000630, 1505.389161788490128, 221.1607250897990014 ) ) ;
#45818=CARTESIAN_POINT ( 'NONE',  ( 9.315703281059999341, 1470.272773095790171, 213.0620134152990204 ) ) ;
#45819=CARTESIAN_POINT ( 'NONE',  ( -9.170040964561099628, 1440.195484865749904, 206.3355864816410019 ) ) ;
#45824=CARTESIAN_POINT ( 'NONE',  ( 9.045129543558639185, 1434.758633656339953, 206.7452360523249979 ) ) ;
#45829=CARTESIAN_POINT ( 'NONE',  ( 11.24295886237570130, 1471.530148615479902, 211.1614490031909952 ) ) ;
#45839=ORIENTED_EDGE ( 'NONE', *, *, #30760, .F. ) ;
#45840=CARTESIAN_POINT ( 'NONE',  ( -0.2232815667140019833, 1437.935022234890084, 227.7359842298990031 ) ) ;
#45852=CARTESIAN_POINT ( 'NONE',  ( 10.50688481900000149, 1490.055410347190218, 204.4952978197489983 ) ) ;
#45868=CARTESIAN_POINT ( 'NONE',  ( -2.664535259099999805E-15, 1424.786834349990158, 209.1218459616989946 ) ) ;
#45871=CARTESIAN_POINT ( 'NONE',  ( 10.93422485186690096, 1501.146248672419915, 205.7757054978180236 ) ) ;
#45874=CARTESIAN_POINT ( 'NONE',  ( 10.30255471828350089, 1462.241748833459951, 211.4138787017499794 ) ) ;
#45882=CARTESIAN_POINT ( 'NONE',  ( -3.747768927200330058, 1508.879014986009906, 204.8753727076559983 ) ) ;
#45887=ORIENTED_EDGE ( 'NONE', *, *, #63092, .F. ) ;
#45893=EDGE_LOOP ( 'NONE', ( #92882, #87724, #67823, #71810 ) ) ;
#45894=CARTESIAN_POINT ( 'NONE',  ( 20.10526951509790194, 1430.877901956239839, 215.1856887477609916 ) ) ;
#45897=CARTESIAN_POINT ( 'NONE',  ( 2.802893083669999896, 1485.536432262990047, 201.6817273870490226 ) ) ;
#45900=CARTESIAN_POINT ( 'NONE',  ( -2.787468846669999945, 1432.903039033290042, 217.8476003497590057 ) ) ;
#45907=CARTESIAN_POINT ( 'NONE',  ( 11.46755315091940020, 1491.645850675550037, 209.2229514265190176 ) ) ;
#45908=ORIENTED_EDGE ( 'NONE', *, *, #10728, .T. ) ;
#45911=CARTESIAN_POINT ( 'NONE',  ( 1.395568240770729940, 1496.886843748869978, 196.8164150919409963 ) ) ;
#45913=CARTESIAN_POINT ( 'NONE',  ( 12.16878324720730120, 1427.280607052069854, 207.7518075308990149 ) ) ;
#45919=EDGE_CURVE ( 'NONE', #15049, #91119, #72643, .T. ) ;
#45925=CARTESIAN_POINT ( 'NONE',  ( 0.01496364964870140063, 1498.468111206090043, 197.7767147553989844 ) ) ;
#45935=CARTESIAN_POINT ( 'NONE',  ( 2.423876137830000221, 1485.612096921090142, 220.0019078347989989 ) ) ;
#45942=ORIENTED_EDGE ( 'NONE', *, *, #23098, .T. ) ;
#45944=CARTESIAN_POINT ( 'NONE',  ( 9.359234811488938988, 1452.034566024799915, 210.3500916188470171 ) ) ;
#45945=CARTESIAN_POINT ( 'NONE',  ( 5.046789308220000159, 1422.880134120949833, 194.5523403762989858 ) ) ;
#45947=CARTESIAN_POINT ( 'NONE',  ( -3.954134211063599746, 1507.541399951509902, 221.3757475976190108 ) ) ;
#45948=CARTESIAN_POINT ( 'NONE',  ( -9.311098898702477200, 1418.495954698334117, 196.8548415329698003 ) ) ;
#45953=EDGE_CURVE ( 'NONE', #34173, #60549, #27287, .T. ) ;
#45954=DIRECTION ( 'NONE',  ( 0.9064253123279890634, 0.3026617302209020366, -0.2945997797534770091 ) ) ;
#45958=ORIENTED_EDGE ( 'NONE', *, *, #81537, .F. ) ;
#45965=ORIENTED_EDGE ( 'NONE', *, *, #62581, .F. ) ;
#45966=CARTESIAN_POINT ( 'NONE',  ( -11.01596213409299985, 1481.419441981669934, 209.0719341547870158 ) ) ;
#45968=CARTESIAN_POINT ( 'NONE',  ( -3.763579503338020160, 1508.126400519680146, 220.7366911303400059 ) ) ;
#45969=CARTESIAN_POINT ( 'NONE',  ( 6.500069621292889899, 1497.924601430119992, 198.3228313574259971 ) ) ;
#45971=ADVANCED_FACE ( 'NONE', ( #33359 ), #75133, .T. ) ;
#45972=CARTESIAN_POINT ( 'NONE',  ( -4.157642293380810372, 1469.875985805179880, 218.3513889513289996 ) ) ;
#45975=CARTESIAN_POINT ( 'NONE',  ( 9.176034321767531310, 1450.127176980830200, 208.3686583938580270 ) ) ;
#45976=CARTESIAN_POINT ( 'NONE',  ( -12.55806607928250074, 1501.992048856159954, 211.3070401664170106 ) ) ;
#45977=CARTESIAN_POINT ( 'NONE',  ( 11.59635154200000251, 1493.084219504590010, 213.4865999382489861 ) ) ;
#45979=CARTESIAN_POINT ( 'NONE',  ( 3.552713678799999608E-15, 1507.551704408389924, 209.1218459616989946 ) ) ;
#45981=CARTESIAN_POINT ( 'NONE',  ( -16.38073507929999906, 1503.849976525089915, 209.2714441331769990 ) ) ;
#45992=CARTESIAN_POINT ( 'NONE',  ( 4.212150227310000439, 1506.735180723689837, 220.0177425982989803 ) ) ;
#45993=CARTESIAN_POINT ( 'NONE',  ( -15.15570824359999946, 1415.677402261749876, 210.8787115431290147 ) ) ;
#45995=CARTESIAN_POINT ( 'NONE',  ( -16.50063655363959825, 1419.653847773739926, 209.2961467218439964 ) ) ;
#45997=LINE ( 'NONE', #61168, #44189 ) ;
#46003=EDGE_CURVE ( 'NONE', #328, #86968, #14949, .T. ) ;
#46007=EDGE_CURVE ( 'NONE', #31217, #95667, #78128, .T. ) ;
#46022=CARTESIAN_POINT ( 'NONE',  ( 12.48513440536379981, 1427.066873444910016, 206.5219089466239950 ) ) ;
#46025=CARTESIAN_POINT ( 'NONE',  ( -16.32615623849999764, 1416.524502645009989, 209.0932030950310150 ) ) ;
#46032=CARTESIAN_POINT ( 'NONE',  ( 7.190299821260000002, 1478.329013068389941, 201.1569836108390064 ) ) ;
#46035=CARTESIAN_POINT ( 'NONE',  ( -4.675540975309999681, 1462.620895424390028, 200.5633310686890241 ) ) ;
#46039=CARTESIAN_POINT ( 'NONE',  ( -11.72765336777909972, 1481.328017084940029, 210.7793835027030127 ) ) ;
#46047=EDGE_CURVE ( 'NONE', #100464, #87329, #11496, .T. ) ;
#46054=CARTESIAN_POINT ( 'NONE',  ( -10.10084594930000002, 1498.671139517090069, 214.6853310067990037 ) ) ;
#46056=CARTESIAN_POINT ( 'NONE',  ( -2.140910185329999660, 1421.480997455049874, 193.7252687417990273 ) ) ;
#46059=CARTESIAN_POINT ( 'NONE',  ( 18.68388892448549754, 1457.534866238390123, 220.6832095082359899 ) ) ;
#46061=CARTESIAN_POINT ( 'NONE',  ( 3.281831451650000009, 1466.303209849290170, 198.5678428638989885 ) ) ;
#46063=CARTESIAN_POINT ( 'NONE',  ( -5.263803380099999707, 1391.914765747090087, 203.7221189175089933 ) ) ;
#46065=DIRECTION ( 'NONE',  ( 1.000000000000000000, 0.000000000000000000, 0.000000000000000000 ) ) ;
#46066=CARTESIAN_POINT ( 'NONE',  ( 13.63294200170024162, 1492.115741768783209, 192.2627525536992152 ) ) ;
#46073=CARTESIAN_POINT ( 'NONE',  ( 11.80625193467720102, 1501.815294225020125, 212.7003682637139832 ) ) ;
#46074=CARTESIAN_POINT ( 'NONE',  ( -11.98171406608951628, 1421.814709082018453, 210.6443979596248539 ) ) ;
#46077=VERTEX_POINT ( 'NONE', #97692 ) ;
#46078=ORIENTED_EDGE ( 'NONE', *, *, #60523, .F. ) ;
#46090=CARTESIAN_POINT ( 'NONE',  ( 12.51041186362150093, 1501.167594044880161, 211.3998864982009991 ) ) ;
#46094=CARTESIAN_POINT ( 'NONE',  ( -20.44228942490000023, 1485.240733021890037, 206.1051096756690129 ) ) ;
#46096=CARTESIAN_POINT ( 'NONE',  ( 20.81805214273520122, 1457.016357340710101, 206.8941968723059972 ) ) ;
#46104=CARTESIAN_POINT ( 'NONE',  ( 4.492546581380000958, 1453.878649273890005, 217.3453973181289882 ) ) ;
#46106=AXIS2_PLACEMENT_3D ( 'NONE', #74659, #6876, #75208 ) ;
#46108=CARTESIAN_POINT ( 'NONE',  ( 9.751945027609998817, 1462.536696320589954, 208.9120314007480204 ) ) ;
#46112=ADVANCED_FACE ( 'NONE', ( #79810 ), #69552, .T. ) ;
#46119=CARTESIAN_POINT ( 'NONE',  ( 11.39627603927229949, 1478.751622603650048, 206.3037616009159763 ) ) ;
#46124=CARTESIAN_POINT ( 'NONE',  ( -18.00826777305211124, 1508.456934164587210, 211.8767047476162020 ) ) ;
#46125=CARTESIAN_POINT ( 'NONE',  ( 21.13734888319999783, 1496.938803861589804, 209.1218459616989946 ) ) ;
#46127=CARTESIAN_POINT ( 'NONE',  ( -9.390527344411388810, 1437.694362696060125, 212.1689238372079842 ) ) ;
#46131=CARTESIAN_POINT ( 'NONE',  ( -7.482302563030000186, 1508.669737789789906, 219.1818476679989942 ) ) ;
#46145=CARTESIAN_POINT ( 'NONE',  ( -3.002568591853699953, 1483.560948544299890, 198.8865183318360152 ) ) ;
#46147=VERTEX_POINT ( 'NONE', #94243 ) ;
#46148=DIRECTION ( 'NONE',  ( -1.000000000000000000, 0.000000000000000000, 0.000000000000000000 ) ) ;
#46151=CARTESIAN_POINT ( 'NONE',  ( -14.01525947340000045, 1415.677402202029953, 204.0303135798690164 ) ) ;
#46161=ADVANCED_FACE ( 'NONE', ( #17518 ), #42068, .T. ) ;
#46162=CARTESIAN_POINT ( 'NONE',  ( 1.114108910750000181, 1515.531799303389789, 213.2143613245789879 ) ) ;
#46168=CARTESIAN_POINT ( 'NONE',  ( 2.330134122034449806, 1515.551704408389924, 205.2922258479440245 ) ) ;
#46173=CARTESIAN_POINT ( 'NONE',  ( 3.775315583779999873, 1507.374707175490130, 220.2027399556990019 ) ) ;
#46177=CARTESIAN_POINT ( 'NONE',  ( 5.487466536400559924, 1465.925728487379956, 200.7492532196600052 ) ) ;
#46193=CARTESIAN_POINT ( 'NONE',  ( -3.175620192230000249, 1509.758513049789826, 217.6845658033289794 ) ) ;
#46200=CARTESIAN_POINT ( 'NONE',  ( 7.663837900699999928, 1425.530251840890060, 211.9032649451089867 ) ) ;
#46206=CARTESIAN_POINT ( 'NONE',  ( 8.784742016200000947, 1452.237884818490102, 212.1741301903489898 ) ) ;
#46233=CARTESIAN_POINT ( 'NONE',  ( -3.954567845990000219, 1455.724191770290190, 200.5335190476789933 ) ) ;
#46240=ORIENTED_EDGE ( 'NONE', *, *, #13923, .F. ) ;
#46247=CARTESIAN_POINT ( 'NONE',  ( -12.00397982357779902, 1489.758001204110087, 211.4229914170240079 ) ) ;
#46266=CARTESIAN_POINT ( 'NONE',  ( 14.30096130324469961, 1427.140377532109824, 198.0371785924010055 ) ) ;
#46271=B_SPLINE_CURVE_WITH_KNOTS ( 'NONE', 5,
 ( #51124, #84699, #59528, #26451, #43278, #8000 ),
 .UNSPECIFIED., .F., .F.,
 ( 6, 6 ),
 ( 0.000000000000000000, 1.000000000000000000 ),
 .UNSPECIFIED. ) ;
#46277=CARTESIAN_POINT ( 'NONE',  ( -2.734206733259999744, 1429.237800606489827, 200.5523466973589848 ) ) ;
#46285=CARTESIAN_POINT ( 'NONE',  ( 10.41177329615350011, 1460.024665156439823, 205.9063136364349873 ) ) ;
#46286=FACE_OUTER_BOUND ( 'NONE', #83204, .T. ) ;
#46292=DIRECTION ( 'NONE',  ( 0.000000000000000000, 1.000000000000000000, 0.000000000000000000 ) ) ;
#46296=CARTESIAN_POINT ( 'NONE',  ( -0.2334700972460009849, 1444.212002848689963, 218.0769002143289867 ) ) ;
#46302=DIRECTION ( 'NONE',  ( -1.000000000000000000, 0.000000000000000000, 0.000000000000000000 ) ) ;
#46307=CARTESIAN_POINT ( 'NONE',  ( -11.48415382500000170, 1508.440752798089989, 218.1712173149890077 ) ) ;
#46310=CARTESIAN_POINT ( 'NONE',  ( -2.001528378510000206, 1483.806447908390055, 198.6272630702989943 ) ) ;
#46312=CARTESIAN_POINT ( 'NONE',  ( -16.02483746670864662, 1417.968541902725747, 204.0964192873620959 ) ) ;
#46316=CARTESIAN_POINT ( 'NONE',  ( 4.641807258861630814, 1493.238112264180018, 219.2220438651660004 ) ) ;
#46318=CARTESIAN_POINT ( 'NONE',  ( -4.969322309076429356, 1487.355502429559920, 219.6549086668990185 ) ) ;
#46319=CARTESIAN_POINT ( 'NONE',  ( -18.29179384260000063, 1466.060301038189891, 217.7541513960790098 ) ) ;
#46336=CARTESIAN_POINT ( 'NONE',  ( 11.48709584101343140, 1502.831951580399164, 210.2032813508793083 ) ) ;
#46339=CARTESIAN_POINT ( 'NONE',  ( -5.723713397950000115, 1444.578274639889969, 217.6728780112489972 ) ) ;
#46341=CARTESIAN_POINT ( 'NONE',  ( 1.379638663375890140, 1515.081065330719866, 213.4508686280049972 ) ) ;
#46349=CARTESIAN_POINT ( 'NONE',  ( -22.15023429329999871, 1486.164746652490066, 217.3274157383089857 ) ) ;
#46356=CARTESIAN_POINT ( 'NONE',  ( -9.519812933809998157, 1460.017558320190119, 210.6311618102489831 ) ) ;
#46368=CARTESIAN_POINT ( 'NONE',  ( 1.210523399180029935, 1495.904440378810023, 221.4016620453209896 ) ) ;
#46371=CARTESIAN_POINT ( 'NONE',  ( 4.664268937930000192, 1505.247554523090002, 221.0077437511990013 ) ) ;
#46376=CARTESIAN_POINT ( 'NONE',  ( 4.972072924729999954, 1472.535148281390093, 218.0116174414390002 ) ) ;
#46377=CARTESIAN_POINT ( 'NONE',  ( -9.463103648650079691, 1439.631690924059740, 207.7258123655099951 ) ) ;
#46381=CARTESIAN_POINT ( 'NONE',  ( 8.280067823819621253, 1436.009449604699967, 206.8167673534310325 ) ) ;
#46386=CARTESIAN_POINT ( 'NONE',  ( 1.311009928872819863, 1467.109053032259908, 220.1154688705190097 ) ) ;
#46389=TOROIDAL_SURFACE ( 'NONE', #12381, 10.10241613150000006, 2.000000000000000000 ) ;
#46391=CARTESIAN_POINT ( 'NONE',  ( 8.401749989260000717, 1454.595346029489974, 215.7321778818789824 ) ) ;
#46392=EDGE_CURVE ( 'NONE', #94689, #90525, #48519, .T. ) ;
#46399=CARTESIAN_POINT ( 'NONE',  ( -8.316672828268760753, 1425.055149638239982, 204.9623390585310005 ) ) ;
#46404=EDGE_CURVE ( 'NONE', #86968, #98016, #99746, .T. ) ;
#46405=CARTESIAN_POINT ( 'NONE',  ( -14.22126295610000213, 1417.509116686749849, 204.1625520109990077 ) ) ;
#46410=CARTESIAN_POINT ( 'NONE',  ( -1.289560617741849935, 1504.157614064680047, 209.3656258553460248 ) ) ;
#46415=VERTEX_POINT ( 'NONE', #41385 ) ;
#46416=CARTESIAN_POINT ( 'NONE',  ( -17.33425267040000151, 1417.532075291570209, 206.8248474228290092 ) ) ;
#46426=CARTESIAN_POINT ( 'NONE',  ( -10.07183425689889944, 1461.550206846259925, 210.3700608705820230 ) ) ;
#46430=B_SPLINE_CURVE_WITH_KNOTS ( 'NONE', 5,
 ( #5399, #101501, #69061, #73732, #107855, #65332 ),
 .UNSPECIFIED., .F., .F.,
 ( 6, 6 ),
 ( -13.21653623010000089, -9.791999830326519216 ),
 .UNSPECIFIED. ) ;
#46433=CARTESIAN_POINT ( 'NONE',  ( -1.282176200179999892, 1442.957053292389901, 200.3169478525390161 ) ) ;
#46441=CARTESIAN_POINT ( 'NONE',  ( 3.829620113550000315, 1515.551704408389924, 206.7917118356089929 ) ) ;
#46448=CARTESIAN_POINT ( 'NONE',  ( -3.640869362099999673, 1474.974412159089979, 198.7036061503989970 ) ) ;
#46450=ORIENTED_EDGE ( 'NONE', *, *, #50827, .F. ) ;
#46451=CARTESIAN_POINT ( 'NONE',  ( -11.77904337550669922, 1483.168283496399908, 228.2502193403299771 ) ) ;
#46458=CARTESIAN_POINT ( 'NONE',  ( -3.100192419969999946, 1431.506313241990028, 216.9304414810590060 ) ) ;
#46459=CARTESIAN_POINT ( 'NONE',  ( 7.703785732380000084, 1490.746146274789908, 209.8379679705590206 ) ) ;
#46466=CARTESIAN_POINT ( 'NONE',  ( 10.96071825005859957, 1490.321551646910166, 209.5423776189929868 ) ) ;
#46470=CARTESIAN_POINT ( 'NONE',  ( -13.84742034927290000, 1420.584111001069914, 215.1188189259799799 ) ) ;
#46472=CARTESIAN_POINT ( 'NONE',  ( 0.6919511451386070044, 1496.727473275949933, 196.7667901871089953 ) ) ;
#46480=DIRECTION ( 'NONE',  ( -1.000000000000000000, 0.000000000000000000, 0.000000000000000000 ) ) ;
#46482=AXIS2_PLACEMENT_3D ( 'NONE', #34307, #58423, #76876 ) ;
#46494=DIRECTION ( 'NONE',  ( 0.000000000000000000, -0.02617694830808806397, -0.9996573249755517088 ) ) ;
#46510=CARTESIAN_POINT ( 'NONE',  ( -7.198880892473511928, 1419.144553764449938, 195.5038830598559798 ) ) ;
#46513=ORIENTED_EDGE ( 'NONE', *, *, #60243, .T. ) ;
#46522=CARTESIAN_POINT ( 'NONE',  ( 2.789312393583509131, 1478.277622718212115, 199.0202689340788140 ) ) ;
#46525=CARTESIAN_POINT ( 'NONE',  ( -10.68970859486899805, 1481.192556119350229, 208.4617474437989983 ) ) ;
#46527=CARTESIAN_POINT ( 'NONE',  ( 6.042363554874039977, 1498.446830258970067, 198.9500472058119840 ) ) ;
#46528=CARTESIAN_POINT ( 'NONE',  ( -5.667442515161419614, 1470.223707235179972, 217.5701957336380019 ) ) ;
#46531=CARTESIAN_POINT ( 'NONE',  ( 9.197260543180000525, 1420.703589484819986, 196.7538032495989739 ) ) ;
#46533=CARTESIAN_POINT ( 'NONE',  ( -5.938382366523570433, 1494.685032631710101, 198.3270043733569992 ) ) ;
#46536=CARTESIAN_POINT ( 'NONE',  ( -13.53999783040000082, 1502.986154819089961, 208.9317388931999915 ) ) ;
#46546=CARTESIAN_POINT ( 'NONE',  ( 4.337831292979999809, 1507.165484465889904, 219.9878051107990302 ) ) ;
#46547=CARTESIAN_POINT ( 'NONE',  ( -11.71397119449999913, 1489.483175832489906, 212.5377882278690151 ) ) ;
#46548=CARTESIAN_POINT ( 'NONE',  ( 3.535327672168380175, 1487.160996015089950, 197.6951163816430039 ) ) ;
#46550=CARTESIAN_POINT ( 'NONE',  ( 4.506137960680000276, 1429.623679839590068, 216.5655692257590204 ) ) ;
#46552=CARTESIAN_POINT ( 'NONE',  ( -15.94166470599999919, 1416.020783510179854, 209.6543286340279906 ) ) ;
#46553=CARTESIAN_POINT ( 'NONE',  ( -2.076036472240859965, 1429.421786079320100, 199.9751262666950140 ) ) ;
#46557=CARTESIAN_POINT ( 'NONE',  ( 8.508615264710758908, 1460.260753410110055, 204.1139426562619690 ) ) ;
#46560=ADVANCED_FACE ( 'NONE', ( #59850 ), #105329, .F. ) ;
#46561=CARTESIAN_POINT ( 'NONE',  ( -3.657996696819999727, 1474.872005729190050, 218.7367884669989735 ) ) ;
#46579=CARTESIAN_POINT ( 'NONE',  ( 3.222662844351010136, 1456.191203615270069, 219.2431310769710251 ) ) ;
#46581=FACE_OUTER_BOUND ( 'NONE', #53820, .T. ) ;
#46586=CARTESIAN_POINT ( 'NONE',  ( -5.534100668969379910, 1464.371862158079921, 199.5915835189479992 ) ) ;
#46589=CARTESIAN_POINT ( 'NONE',  ( -11.84446372125409930, 1481.644281931980004, 209.8205016465489621 ) ) ;
#46594=CARTESIAN_POINT ( 'NONE',  ( -12.05523474180890098, 1491.092627158069945, 206.8423379236589881 ) ) ;
#46595=CARTESIAN_POINT ( 'NONE',  ( -4.788487179430729768, 1508.551704408389924, 205.6544253393599888 ) ) ;
#46602=DIRECTION ( 'NONE',  ( -9.500914144214121536E-47, 1.000000000000000000, -1.836970198721029688E-16 ) ) ;
#46608=CARTESIAN_POINT ( 'NONE',  ( 0.2270307469910020082, 1422.992384322039925, 192.4621272340990004 ) ) ;
#46613=ADVANCED_FACE ( 'NONE', ( #82000 ), #41145, .F. ) ;
#46614=CARTESIAN_POINT ( 'NONE',  ( -16.51469981520000019, 1466.007824952989949, 220.7976724296989914 ) ) ;
#46625=CARTESIAN_POINT ( 'NONE',  ( -11.39483696856016692, 1422.053277916610568, 210.6383599177140695 ) ) ;
#46636=EDGE_CURVE ( 'NONE', #22353, #93538, #43152, .T. ) ;
#46640=CARTESIAN_POINT ( 'NONE',  ( 7.396059631071099538, 1483.223942348629862, 217.9804716342530071 ) ) ;
#46645=CARTESIAN_POINT ( 'NONE',  ( 12.24108702360000045, 1428.408480395390143, 194.9166229853989876 ) ) ;
#46655=AXIS2_PLACEMENT_3D ( 'NONE', #18450, #69466, #36930 ) ;
#46660=CARTESIAN_POINT ( 'NONE',  ( -0.1571152812289989820, 1465.182248420690030, 198.5055488938989754 ) ) ;
#46673=CARTESIAN_POINT ( 'NONE',  ( -19.09790268268400126, 1508.458003811930212, 210.0050661408479868 ) ) ;
#46676=CARTESIAN_POINT ( 'NONE',  ( -9.215400547745700166, 1437.452820398420045, 212.6238575580420047 ) ) ;
#46680=LINE ( 'NONE', #20334, #110751 ) ;
#46684=CARTESIAN_POINT ( 'NONE',  ( -3.865992865399999978, 1463.465618750590011, 228.4375626785990221 ) ) ;
#46692=EDGE_LOOP ( 'NONE', ( #59214, #79818, #35014, #88851, #37493 ) ) ;
#46696=CARTESIAN_POINT ( 'NONE',  ( -15.01736473799999949, 1415.953171031319926, 205.5614245712289971 ) ) ;
#46702=CARTESIAN_POINT ( 'NONE',  ( 19.41157449629999832, 1457.417846740989944, 209.1218459616989946 ) ) ;
#46707=EDGE_CURVE ( 'NONE', #92866, #41219, #108581, .T. ) ;
#46709=CARTESIAN_POINT ( 'NONE',  ( -1.842962231260000028, 1515.492058413689847, 213.2603893528589936 ) ) ;
#46711=CARTESIAN_POINT ( 'NONE',  ( -2.735359696209999747, 1470.857183403589943, 189.2159460739989925 ) ) ;
#46714=CARTESIAN_POINT ( 'NONE',  ( -10.33299300126450149, 1447.717326489380184, 209.8084994042759774 ) ) ;
#46716=CARTESIAN_POINT ( 'NONE',  ( -4.468118146560000170, 1458.475370017489922, 218.8772509106790096 ) ) ;
#46720=DIRECTION ( 'NONE',  ( -1.000000000000000000, 0.000000000000000000, 0.000000000000000000 ) ) ;
#46721=ORIENTED_EDGE ( 'NONE', *, *, #89828, .T. ) ;
#46723=CARTESIAN_POINT ( 'NONE',  ( 5.586270675034979760, 1465.491174728670103, 200.8384121407760006 ) ) ;
#46726=CARTESIAN_POINT ( 'NONE',  ( 20.49831092009999978, 1496.178973653789853, 204.1013708937389879 ) ) ;
#46730=CARTESIAN_POINT ( 'NONE',  ( 1.174755966547918140, 1431.055736453459531, 217.8297097953777666 ) ) ;
#46731=CARTESIAN_POINT ( 'NONE',  ( -10.83907793900000094, 1482.736899269390051, 205.3800505913289953 ) ) ;
#46741=FACE_OUTER_BOUND ( 'NONE', #69469, .T. ) ;
#46744=CIRCLE ( 'NONE', #75352, 7.799999999999999822 ) ;
#46751=CARTESIAN_POINT ( 'NONE',  ( 8.377020731070000892, 1427.910351821989934, 212.6460221678989910 ) ) ;
#46752=CARTESIAN_POINT ( 'NONE',  ( 20.56230369369999877, 1477.111288992490017, 217.7195332328089989 ) ) ;
#46760=EDGE_LOOP ( 'NONE', ( #63366, #37454, #58206, #84205 ) ) ;
#46769=CARTESIAN_POINT ( 'NONE',  ( -2.170363546252639608, 1464.474365425050109, 199.1286919944959948 ) ) ;
#46792=VECTOR ( 'NONE', #91116, 1000.000000000000000 ) ;
#46795=CARTESIAN_POINT ( 'NONE',  ( 10.69530615799999929, 1492.057806673789855, 212.3894089256490076 ) ) ;
#46804=VECTOR ( 'NONE', #68908, 1000.000000000000000 ) ;
#46810=CARTESIAN_POINT ( 'NONE',  ( 16.53404221824990117, 1428.071160471989970, 201.6834493251120080 ) ) ;
#46815=( BOUNDED_CURVE ( )  B_SPLINE_CURVE ( 3, ( #14223, #107743, #91500, #81415 ),
 .UNSPECIFIED., .F., .F. ) 
 B_SPLINE_CURVE_WITH_KNOTS ( ( 4, 4 ),
 ( 4.673418987722709694, 4.822346547659980054 ),
 .UNSPECIFIED. ) 
 CURVE ( )  GEOMETRIC_REPRESENTATION_ITEM ( )  RATIONAL_B_SPLINE_CURVE ( ( 1.000000000000000000, 0.9981525690389736472, 0.9981525690389736472, 1.000000000000000000 ) ) 
 REPRESENTATION_ITEM ( '' )  );
#46823=CARTESIAN_POINT ( 'NONE',  ( 10.75070237740000145, 1423.976811909279832, 204.9811967931990182 ) ) ;
#46827=CARTESIAN_POINT ( 'NONE',  ( -4.212124233566025389, 1455.571073703328693, 200.6608987289929757 ) ) ;
#46829=CARTESIAN_POINT ( 'NONE',  ( 10.06738412557950113, 1469.597899895000182, 209.1389479632179871 ) ) ;
#46837=CARTESIAN_POINT ( 'NONE',  ( 7.930811094041184006, 1423.727541757261861, 195.8483739583643342 ) ) ;
#46838=CARTESIAN_POINT ( 'NONE',  ( 1.657211920199999966, 1442.925229136189955, 217.9916902927889737 ) ) ;
#46844=CARTESIAN_POINT ( 'NONE',  ( -2.569508516276699961, 1464.905644613789718, 198.4146467863039902 ) ) ;
#46852=CARTESIAN_POINT ( 'NONE',  ( -9.386420905929998781, 1508.551704408389924, 218.5291032798490107 ) ) ;
#46854=CARTESIAN_POINT ( 'NONE',  ( 11.41287573240554032, 1427.618782186570115, 209.6357587079445182 ) ) ;
#46860=CARTESIAN_POINT ( 'NONE',  ( 3.902834784268570001, 1495.323243761410140, 220.8767705547660114 ) ) ;
#46861=CARTESIAN_POINT ( 'NONE',  ( -2.775543834090889561, 1468.867531313959944, 187.4507025151330026 ) ) ;
#46862=CARTESIAN_POINT ( 'NONE',  ( -15.36839037194300062, 1415.677402202079975, 209.1379692602760088 ) ) ;
#46868=EDGE_CURVE ( 'NONE', #71088, #64216, #7046, .T. ) ;
#46874=CARTESIAN_POINT ( 'NONE',  ( 7.561666052370960678, 1423.087019363542595, 213.9609131946497200 ) ) ;
#46884=CARTESIAN_POINT ( 'NONE',  ( 8.237294568284330154, 1465.649939967559931, 214.5915065964550195 ) ) ;
#46886=CARTESIAN_POINT ( 'NONE',  ( -0.7087989430410059910, 1515.130721759790049, 213.4495683292759907 ) ) ;
#46888=CARTESIAN_POINT ( 'NONE',  ( -3.795278851281820298, 1476.619100922419875, 219.9733720370720107 ) ) ;
#46893=ORIENTED_EDGE ( 'NONE', *, *, #107727, .T. ) ;
#46894=ORIENTED_EDGE ( 'NONE', *, *, #104242, .T. ) ;
#46896=CARTESIAN_POINT ( 'NONE',  ( -5.731845798429999306, 1492.036577540089866, 185.8612320274989997 ) ) ;
#46901=B_SPLINE_CURVE_WITH_KNOTS ( 'NONE', 5,
 ( #63610, #106134, #96637, #89329, #88786, #27767 ),
 .UNSPECIFIED., .F., .F.,
 ( 6, 6 ),
 ( 0.000000000000000000, 1.000000000000000000 ),
 .UNSPECIFIED. ) ;
#46915=ADVANCED_FACE ( 'NONE', ( #9184 ), #17545, .T. ) ;
#46923=CARTESIAN_POINT ( 'NONE',  ( 7.885640402109999059, 1473.211498812089985, 217.4524272520789907 ) ) ;
#46931=ORIENTED_EDGE ( 'NONE', *, *, #88751, .T. ) ;
#46932=EDGE_LOOP ( 'NONE', ( #17656, #26218, #27949, #19006, #84082 ) ) ;
#46934=CARTESIAN_POINT ( 'NONE',  ( 11.15425147308119946, 1471.646069826549819, 211.6152046850310171 ) ) ;
#46951=CARTESIAN_POINT ( 'NONE',  ( -11.61983319979999862, 1416.674354222800048, 204.7879751430089925 ) ) ;
#46960=ORIENTED_EDGE ( 'NONE', *, *, #54478, .F. ) ;
#46978=CARTESIAN_POINT ( 'NONE',  ( 12.30852457429709901, 1501.337141734960142, 211.6826237522950009 ) ) ;
#46979=B_SPLINE_CURVE_WITH_KNOTS ( 'NONE', 3,
 ( #105142, #37386, #96187, #37945, #19463, #96751, #29527, #87807, #106241, #54216, #71587, #97827, #21105, #12733, #1589, #69915, #39590, #13257, #98384, #56952, #91081, #5432, #4347, #72653, #22202, #73194, #31725, #58055, #89983, #4874, #91638, #73761, #5983, #21655 ),
 .UNSPECIFIED., .F., .F.,
 ( 4, 3, 3, 3, 3, 3, 3, 3, 3, 3, 3, 4 ),
 ( -2.000000000000000000, -1.894376539578449981, -1.708008357126509891, -1.519432768888129948, -1.329646548225599911, -1.138371395304140110, -0.9466417899035080019, -0.7549279318903319158, -0.5636971425523138457, -0.3741224486121028647, -0.1861321647941660551, 0.000000000000000000 ),
 .UNSPECIFIED. ) ;
#46980=CARTESIAN_POINT ( 'NONE',  ( -10.46900974659999939, 1491.361946609490133, 212.5217932129490066 ) ) ;
#46983=CARTESIAN_POINT ( 'NONE',  ( -4.058118992948309689, 1508.551704408389924, 204.4428593323469840 ) ) ;
#46991=EDGE_CURVE ( 'NONE', #53764, #78921, #9610, .T. ) ;
#46992=CARTESIAN_POINT ( 'NONE',  ( -3.349195415509999663, 1474.892783691989962, 198.1874921133990028 ) ) ;
#46995=CARTESIAN_POINT ( 'NONE',  ( 18.68388055094409950, 1457.534813197310086, 220.6832175138739842 ) ) ;
#46999=LINE ( 'NONE', #82782, #20803 ) ;
#47000=CARTESIAN_POINT ( 'NONE',  ( 11.22296312822500752, 1503.420383748715722, 211.9371915619264541 ) ) ;
#47035=CARTESIAN_POINT ( 'NONE',  ( -2.521622038060000293, 1415.707855076169835, 204.8799433334789910 ) ) ;
#47042=CARTESIAN_POINT ( 'NONE',  ( -5.030623778630000764, 1391.799617351889992, 214.4844137014689807 ) ) ;
#47048=ORIENTED_EDGE ( 'NONE', *, *, #45020, .T. ) ;
#47049=ORIENTED_EDGE ( 'NONE', *, *, #109695, .F. ) ;
#47053=CARTESIAN_POINT ( 'NONE',  ( -4.626185416090139668, 1439.746126037229942, 205.5536779009150052 ) ) ;
#47056=CARTESIAN_POINT ( 'NONE',  ( -0.2549717317763739999, 1442.897952001810154, 200.2186391711400120 ) ) ;
#47070=CARTESIAN_POINT ( 'NONE',  ( -9.891642072088888682, 1470.030674514850034, 213.7492784014550011 ) ) ;
#47072=CARTESIAN_POINT ( 'NONE',  ( 9.223040078240002160, 1420.831005969599801, 196.7861790798990000 ) ) ;
#47073=CARTESIAN_POINT ( 'NONE',  ( -2.229670771031690091, 1476.033530122819911, 220.3577958911180019 ) ) ;
#47074=CARTESIAN_POINT ( 'NONE',  ( -3.263114576272079827E-31, 1414.677402202029953, 209.1218459616989946 ) ) ;
#47079=CARTESIAN_POINT ( 'NONE',  ( 11.23478826778469930, 1422.543918281529841, 207.0476803316210237 ) ) ;
#47081=CARTESIAN_POINT ( 'NONE',  ( -9.788108383745552032, 1440.056842154589958, 207.0031482218739995 ) ) ;
#47088=CARTESIAN_POINT ( 'NONE',  ( 10.47511427260239891, 1482.040461736080033, 210.7458695605469927 ) ) ;
#47089=CARTESIAN_POINT ( 'NONE',  ( -10.28857233090000101, 1463.185141274090256, 204.9217573806190273 ) ) ;
#47091=CARTESIAN_POINT ( 'NONE',  ( -16.70830179842720042, 1417.149226859160080, 207.3570905742490140 ) ) ;
#47093=CARTESIAN_POINT ( 'NONE',  ( -8.102530104066362426, 1477.152887553389974, 215.6207631052049294 ) ) ;
#47094=CARTESIAN_POINT ( 'NONE',  ( 9.682511080499990541, 1436.279831232390052, 210.8541354582289955 ) ) ;
#47097=CARTESIAN_POINT ( 'NONE',  ( 3.313918604249419975, 1458.909887735149823, 200.0205288476430212 ) ) ;
#47109=CARTESIAN_POINT ( 'NONE',  ( -14.30580887908100074, 1416.879264667930101, 203.2316167391460056 ) ) ;
#47110=( BOUNDED_CURVE ( )  B_SPLINE_CURVE ( 3, ( #51505, #19403, #68333, #102440 ),
 .UNSPECIFIED., .F., .F. ) 
 B_SPLINE_CURVE_WITH_KNOTS ( ( 4, 4 ),
 ( 0.9971162661778150138, 2.144476395621194964 ),
 .UNSPECIFIED. ) 
 CURVE ( )  GEOMETRIC_REPRESENTATION_ITEM ( )  RATIONAL_B_SPLINE_CURVE ( ( 1.000000000000000000, 0.8932729319369855370, 0.8932729319369855370, 1.000000000000000000 ) ) 
 REPRESENTATION_ITEM ( '' )  );
#47116=CARTESIAN_POINT ( 'NONE',  ( 0.6485169668797152731, 1484.502209508327951, 198.4327370695805257 ) ) ;
#47123=CARTESIAN_POINT ( 'NONE',  ( -12.25106032620000107, 1490.322274117190091, 209.3376309630089622 ) ) ;
#47124=CARTESIAN_POINT ( 'NONE',  ( -8.992287217462708426, 1437.995524108949894, 210.4996962295319918 ) ) ;
#47127=CARTESIAN_POINT ( 'NONE',  ( 9.345710454894810226, 1422.635914553260136, 212.8840094578699791 ) ) ;
#47137=CARTESIAN_POINT ( 'NONE',  ( -0.3888774176050009967, 1508.936806585589920, 218.1328934611190107 ) ) ;
#47141=CARTESIAN_POINT ( 'NONE',  ( -7.465188678339999662, 1497.180420109090164, 217.7707592773190015 ) ) ;
#47143=CARTESIAN_POINT ( 'NONE',  ( 1.833868989029999952, 1422.484255930740119, 193.6377413423990106 ) ) ;
#47147=CARTESIAN_POINT ( 'NONE',  ( -16.61337859989249921, 1463.629512765479831, 220.4655032150840270 ) ) ;
#47158=ORIENTED_EDGE ( 'NONE', *, *, #26171, .F. ) ;
#47159=CARTESIAN_POINT ( 'NONE',  ( 11.20410962351969886, 1503.462441903569925, 212.0609900696560146 ) ) ;
#47167=CARTESIAN_POINT ( 'NONE',  ( 11.35976097320000022, 1500.240390108989914, 205.8138550405789999 ) ) ;
#47174=CARTESIAN_POINT ( 'NONE',  ( 9.690694291389919002, 1481.940033707770226, 215.3400710034819951 ) ) ;
#47175=SHAPE_DEFINITION_REPRESENTATION ( #57247, #22211 ) ;
#47178=CARTESIAN_POINT ( 'NONE',  ( -14.38097578403179888, 1422.143783148600050, 196.2925640312170117 ) ) ;
#47187=CARTESIAN_POINT ( 'NONE',  ( -16.88275388290000123, 1507.705444072489854, 209.4032267757409898 ) ) ;
#47192=CARTESIAN_POINT ( 'NONE',  ( 0.9125060962980010570, 1465.149707686289730, 198.8904297983990261 ) ) ;
#47203=CARTESIAN_POINT ( 'NONE',  ( -7.500000000000000000, 1391.913060387289988, 209.1218459616989946 ) ) ;
#47204=CARTESIAN_POINT ( 'NONE',  ( -17.85077614882369090, 1508.456763636446112, 212.1147255241837115 ) ) ;
#47205=CARTESIAN_POINT ( 'NONE',  ( 8.206329918199999796, 1502.256773578390039, 208.4091422247220180 ) ) ;
#47206=CARTESIAN_POINT ( 'NONE',  ( -8.906178969139920909, 1437.089246318600090, 213.2884079821210150 ) ) ;
#47221=CARTESIAN_POINT ( 'NONE',  ( -5.102340803919999779, 1483.010473641589897, 199.7820758705289848 ) ) ;
#47227=CARTESIAN_POINT ( 'NONE',  ( -1.637258856660000150, 1483.893433971690001, 198.5669146070989939 ) ) ;
#47230=CARTESIAN_POINT ( 'NONE',  ( 8.247379814629999473, 1421.181889050119935, 196.1087402428989890 ) ) ;
#47231=CARTESIAN_POINT ( 'NONE',  ( -8.809238219330000064, 1438.685537000089880, 208.2566061143539855 ) ) ;
#47235=ORIENTED_EDGE ( 'NONE', *, *, #85004, .T. ) ;
#47243=B_SPLINE_CURVE_WITH_KNOTS ( 'NONE', 3,
 ( #84922, #66520, #6028, #102281, #8215, #92782 ),
 .UNSPECIFIED., .F., .F.,
 ( 4, 2, 4 ),
 ( 0.000000000000000000, 0.5000000000000000000, 1.000000000000000000 ),
 .UNSPECIFIED. ) ;
#47248=CARTESIAN_POINT ( 'NONE',  ( -3.984081798389999651, 1515.551704150889918, 210.9648099238589793 ) ) ;
#47256=CARTESIAN_POINT ( 'NONE',  ( 9.296941329909470753, 1453.078838434450063, 212.1081459014599773 ) ) ;
#47262=CARTESIAN_POINT ( 'NONE',  ( 12.24165105991550107, 1491.712733692510028, 207.8385283740699947 ) ) ;
#47268=EDGE_LOOP ( 'NONE', ( #63588, #64151, #60264, #97121, #94131 ) ) ;
#47271=CARTESIAN_POINT ( 'NONE',  ( -13.58498611669640077, 1508.504310626469987, 210.0344663469770126 ) ) ;
#47272=FACE_OUTER_BOUND ( 'NONE', #56509, .T. ) ;
#47276=CARTESIAN_POINT ( 'NONE',  ( -5.101062890589999732, 1453.677351314490124, 200.8020249629389866 ) ) ;
#47278=CARTESIAN_POINT ( 'NONE',  ( 7.360599658199999062, 1427.547306193929899, 213.0878178632989943 ) ) ;
#47289=CARTESIAN_POINT ( 'NONE',  ( 10.13545654959800046, 1453.511789294690061, 212.2748785446170245 ) ) ;
#47294=CARTESIAN_POINT ( 'NONE',  ( -21.50985349126370139, 1505.528545743399945, 209.4501121847560228 ) ) ;
#47305=ORIENTED_EDGE ( 'NONE', *, *, #34725, .F. ) ;
#47315=CARTESIAN_POINT ( 'NONE',  ( -18.30672310084519694, 1508.551704408389924, 210.5933980790459827 ) ) ;
#47337=CARTESIAN_POINT ( 'NONE',  ( 6.900299337267749245, 1425.082553785249956, 192.4924159130339945 ) ) ;
#47348=EDGE_CURVE ( 'NONE', #67457, #26746, #89746, .T. ) ;
#47354=CARTESIAN_POINT ( 'NONE',  ( 11.15518508559999944, 1425.266589066719916, 204.1085830429390171 ) ) ;
#47355=CARTESIAN_POINT ( 'NONE',  ( 0.6019981773732412389, 1498.612803264159538, 197.8140259511527006 ) ) ;
#47360=CARTESIAN_POINT ( 'NONE',  ( 11.21992499831749868, 1470.403109959280073, 207.2954163329770267 ) ) ;
#47361=ORIENTED_EDGE ( 'NONE', *, *, #27023, .F. ) ;
#47368=CARTESIAN_POINT ( 'NONE',  ( 10.95486373408519931, 1461.099043641600019, 209.0941366827430272 ) ) ;
#47371=CARTESIAN_POINT ( 'NONE',  ( 2.032300221149999864, 1441.827160225690022, 218.8459470114090379 ) ) ;
#47373=CARTESIAN_POINT ( 'NONE',  ( 4.967684365510000255, 1469.890599266690060, 189.7939106698990201 ) ) ;
#47382=CARTESIAN_POINT ( 'NONE',  ( -10.16240527536719895, 1472.558926193989919, 209.8189312950259762 ) ) ;
#47383=B_SPLINE_CURVE_WITH_KNOTS ( 'NONE', 3,
 ( #54325, #35849, #36934, #105819, #21203, #106349, #36389, #29635, #20666, #45911, #20131, #12278, #53783, #46472, #87920, #105252, #2815, #63822, #70034, #88455, #27431, #70578, #63282, #3369, #61614, #97935, #80603, #80047, #88990, #27990, #10082, #11742, #54867, #29097, #97396, #62744, #3919 ),
 .UNSPECIFIED., .F., .F.,
 ( 4, 3, 3, 3, 3, 3, 3, 3, 3, 3, 3, 3, 4 ),
 ( -13.59025040360000069, -13.39461751845870019, -12.66963757110119992, -11.90222376896450029, -11.09384317622529892, -10.22895211640910063, -9.214965427742340509, -8.224269270894209782, -7.395227323644159689, -6.444494315334388546, -5.598046305014300117, -4.859242130686430627, -4.164915011539999767 ),
 .UNSPECIFIED. ) ;
#47386=CARTESIAN_POINT ( 'NONE',  ( -13.11794498660000130, 1508.551704418990084, 216.7314840583389923 ) ) ;
#47389=CARTESIAN_POINT ( 'NONE',  ( 11.25715570474750038, 1470.474397315270153, 207.5113747759559999 ) ) ;
#47391=CARTESIAN_POINT ( 'NONE',  ( -10.46250751532009993, 1491.356802638789986, 212.5409670664860187 ) ) ;
#47394=B_SPLINE_SURFACE_WITH_KNOTS ( 'NONE', 4, 5, ( 
 ( #82763, #22269, #75489, #109622, #107958, #90603 ),
 ( #64888, #74389, #32894, #16083, #48067, #92811 ),
 ( #30702, #31252, #65435, #31804, #23397, #57586 ),
 ( #91711, #86617, #93903, #34562, #42977, #76563 ),
 ( #9911, #69295, #33439, #43531, #35664, #42410 ) ),
 .UNSPECIFIED., .F., .F., .F.,
 ( 5, 5 ),
 ( 6, 6 ),
 ( 0.000000000000000000, 4.166045933440000404 ),
 ( 0.000000000000000000, 0.5000005421829999408 ),
 .UNSPECIFIED. ) ;
#47401=CARTESIAN_POINT ( 'NONE',  ( 7.393822440330000134, 1429.049734447289893, 215.1950306291689969 ) ) ;
#47402=CARTESIAN_POINT ( 'NONE',  ( 17.01540922059999872, 1497.106364323189837, 222.9636020297990058 ) ) ;
#47406=EDGE_LOOP ( 'NONE', ( #44293, #75179, #96745, #58092, #78475 ) ) ;
#47407=EDGE_LOOP ( 'NONE', ( #2775, #27127, #15231, #34080, #93689 ) ) ;
#47420=CARTESIAN_POINT ( 'NONE',  ( -0.04897144331352380753, 1515.158513834189989, 213.4488405682529617 ) ) ;
#47422=CARTESIAN_POINT ( 'NONE',  ( -5.368410399077579775, 1477.261207538329927, 219.3405594986899985 ) ) ;
#47429=CARTESIAN_POINT ( 'NONE',  ( -11.74583512589999934, 1503.658496363889981, 208.1214728489190122 ) ) ;
#47430=CARTESIAN_POINT ( 'NONE',  ( -18.85104330493919633, 1504.529957806199945, 222.4016543459620152 ) ) ;
#47435=CARTESIAN_POINT ( 'NONE',  ( 4.326992699981060397, 1515.158586643130093, 209.1431034449670108 ) ) ;
#47436=CARTESIAN_POINT ( 'NONE',  ( 4.908653116315950804, 1484.161144941180055, 219.8999275612819986 ) ) ;
#47438=CARTESIAN_POINT ( 'NONE',  ( -6.120030076239999950, 1458.493692400089913, 216.6798046192089942 ) ) ;
#47443=EDGE_LOOP ( 'NONE', ( #53269, #11021, #70234, #36505 ) ) ;
#47449=CARTESIAN_POINT ( 'NONE',  ( -17.63102292954804895, 1419.721208921065681, 206.9322081005539360 ) ) ;
#47469=CARTESIAN_POINT ( 'NONE',  ( 2.740633910414560059, 1466.650861077639775, 219.8322804162909847 ) ) ;
#47475=CARTESIAN_POINT ( 'NONE',  ( 6.666983987850649385, 1439.588742573630043, 215.5177180616709904 ) ) ;
#47477=ADVANCED_FACE ( 'NONE', ( #101275 ), #25049, .T. ) ;
#47491=CARTESIAN_POINT ( 'NONE',  ( 10.68762204729999965, 1490.102721893990065, 205.8926831195890088 ) ) ;
#47494=EDGE_CURVE ( 'NONE', #49356, #76758, #30822, .T. ) ;
#47500=ADVANCED_FACE ( 'NONE', ( #811 ), #12356, .T. ) ;
#47507=CARTESIAN_POINT ( 'NONE',  ( -0.6415093019302169353, 1455.478019572560015, 198.6153582363290013 ) ) ;
#47508=LINE ( 'NONE', #81632, #86282 ) ;
#47509=B_SPLINE_SURFACE_WITH_KNOTS ( 'NONE', 5, 5, ( 
 ( #9782, #87043, #34981, #70843, #26574, #79767 ),
 ( #43948, #88164, #56066, #27693, #62432, #103846 ),
 ( #94895, #52367, #64488, #27146, #21867, #19829 ),
 ( #3074, #79215, #2523, #43400, #87612, #18715 ),
 ( #98603, #11452, #44503, #38696, #90193, #77551 ),
 ( #86487, #61331, #78650, #1965, #36102, #104398 ),
 ( #61879, #66688, #56620, #6199, #67237, #109771 ),
 ( #33049, #24085, #109233, #81795, #100795, #48226 ),
 ( #90755, #7308, #73972, #41474, #82908, #75083 ) ),
 .UNSPECIFIED., .F., .F., .F.,
 ( 6, 3, 6 ),
 ( 6, 6 ),
 ( 4.119224442280000176, 8.124444112980000909, 13.43342673250000097 ),
 ( 0.000000000000000000, 2.000000000000000000 ),
 .UNSPECIFIED. ) ;
#47511=CARTESIAN_POINT ( 'NONE',  ( -11.14782975800259912, 1470.277812220770102, 211.4323380035779962 ) ) ;
#47512=CARTESIAN_POINT ( 'NONE',  ( 8.761752346032359640, 1498.445853823050129, 199.9005563031199983 ) ) ;
#47513=ORIENTED_EDGE ( 'NONE', *, *, #41570, .F. ) ;
#47518=CARTESIAN_POINT ( 'NONE',  ( -1.326067526109999895, 1442.466427602190151, 200.3461943362390230 ) ) ;
#47519=CARTESIAN_POINT ( 'NONE',  ( -5.036242141850692633, 1491.189339853503043, 188.8516911269720993 ) ) ;
#47520=EDGE_CURVE ( 'NONE', #37990, #73491, #37708, .T. ) ;
#47522=CARTESIAN_POINT ( 'NONE',  ( 1.840021611441419846, 1508.551704408389924, 219.7092512643660029 ) ) ;
#47524=CIRCLE ( 'NONE', #63469, 11.71219856409999949 ) ;
#47527=CARTESIAN_POINT ( 'NONE',  ( -12.62836648000669904, 1502.649130299180115, 209.0071212651150176 ) ) ;
#47533=CARTESIAN_POINT ( 'NONE',  ( 4.449471081249349425, 1508.551704408389924, 205.0837167827569942 ) ) ;
#47535=ORIENTED_EDGE ( 'NONE', *, *, #63062, .F. ) ;
#47536=CARTESIAN_POINT ( 'NONE',  ( 8.129483923442441196, 1461.711659188759995, 228.8737998629739820 ) ) ;
#47545=CARTESIAN_POINT ( 'NONE',  ( -10.07264118456989976, 1472.874378509069857, 207.3195388941770148 ) ) ;
#47548=CARTESIAN_POINT ( 'NONE',  ( 7.724188899110816742, 1461.608062285011329, 227.4089472320192442 ) ) ;
#47555=CARTESIAN_POINT ( 'NONE',  ( -20.02799630220000182, 1485.574563381989947, 204.1280247810589970 ) ) ;
#47559=CARTESIAN_POINT ( 'NONE',  ( -15.08663666819999882, 1420.078856858149948, 212.5885907255689915 ) ) ;
#47563=DIRECTION ( 'NONE',  ( 8.727810504445229884E-47, -1.000000000000000000, 1.836970198721029688E-16 ) ) ;
#47571=CARTESIAN_POINT ( 'NONE',  ( 7.312941311139250722, 1425.031074977940079, 212.6307961945279885 ) ) ;
#47587=CARTESIAN_POINT ( 'NONE',  ( -3.958338145845619049, 1515.551704408390151, 206.7917118413306241 ) ) ;
#47592=ORIENTED_EDGE ( 'NONE', *, *, #3551, .T. ) ;
#47594=CARTESIAN_POINT ( 'NONE',  ( -4.329448776040000446, 1515.064792882589927, 211.4519800877889963 ) ) ;
#47601=FACE_OUTER_BOUND ( 'NONE', #77897, .T. ) ;
#47603=ORIENTED_EDGE ( 'NONE', *, *, #33184, .F. ) ;
#47604=CARTESIAN_POINT ( 'NONE',  ( -3.077634474923088170, 1432.970815717276764, 217.4382276955035991 ) ) ;
#47611=CARTESIAN_POINT ( 'NONE',  ( -2.181792844398890097, 1508.008799467449990, 220.9520129855879986 ) ) ;
#47615=CARTESIAN_POINT ( 'NONE',  ( 11.77327517880000052, 1420.353493371139848, 199.1939701564990060 ) ) ;
#47616=CARTESIAN_POINT ( 'NONE',  ( -3.523962699983150149, 1476.511731499819916, 220.0526012347959863 ) ) ;
#47622=CARTESIAN_POINT ( 'NONE',  ( 10.66776494291289978, 1424.286286161430098, 206.6302605353940010 ) ) ;
#47631=CARTESIAN_POINT ( 'NONE',  ( 9.591773081235949405, 1427.106394943569967, 210.3977398271019865 ) ) ;
#47632=CARTESIAN_POINT ( 'NONE',  ( -16.52130536630199842, 1419.782083806110222, 209.2901812870670142 ) ) ;
#47634=CARTESIAN_POINT ( 'NONE',  ( 4.760952894889999065, 1429.902475422190037, 216.8416751273590251 ) ) ;
#47637=CARTESIAN_POINT ( 'NONE',  ( -16.98382738839999817, 1417.304179998030122, 207.5927328966690197 ) ) ;
#47645=CARTESIAN_POINT ( 'NONE',  ( 2.871115274837119813, 1474.577308913379966, 220.1770025878000183 ) ) ;
#47651=CARTESIAN_POINT ( 'NONE',  ( 0.4463512193210009693, 1458.283482050889916, 202.2977778409189966 ) ) ;
#47653=CARTESIAN_POINT ( 'NONE',  ( 0.7620301704480010319, 1515.588179473189939, 205.1071895219889996 ) ) ;
#47654=CARTESIAN_POINT ( 'NONE',  ( 12.47025950862620114, 1427.078089640870076, 206.5892868991739988 ) ) ;
#47662=CARTESIAN_POINT ( 'NONE',  ( -0.3238248822707833208, 1484.229047029399453, 198.4309250370245934 ) ) ;
#47668=CARTESIAN_POINT ( 'NONE',  ( 8.703395638689999103, 1478.819332251489868, 202.9087528450090190 ) ) ;
#47670=CARTESIAN_POINT ( 'NONE',  ( -11.41602169729999972, 1491.175948940390072, 208.3010286188369946 ) ) ;
#47671=CARTESIAN_POINT ( 'NONE',  ( -8.480431295684640602, 1436.263860089859918, 210.8443010970399882 ) ) ;
#47678=CARTESIAN_POINT ( 'NONE',  ( -7.980167497413499511, 1424.314663469349398, 210.5240444418427899 ) ) ;
#47679=CARTESIAN_POINT ( 'NONE',  ( -4.530454247226269437, 1508.551704408389924, 205.1921026621450324 ) ) ;
#47685=ORIENTED_EDGE ( 'NONE', *, *, #102194, .F. ) ;
#47687=CARTESIAN_POINT ( 'NONE',  ( 9.858506243812300340, 1469.740707437229958, 211.1772101207760102 ) ) ;
#47688=CARTESIAN_POINT ( 'NONE',  ( 12.44780704128189974, 1501.268281525590055, 211.7240718234590133 ) ) ;
#47694=CARTESIAN_POINT ( 'NONE',  ( -13.10665367552279825, 1467.935415218449862, 191.9179395855259997 ) ) ;
#47713=CARTESIAN_POINT ( 'NONE',  ( 1.478581789801439950, 1485.417738077120021, 220.8958599741850151 ) ) ;
#47721=CARTESIAN_POINT ( 'NONE',  ( 8.403712088333849195, 1482.711991784579823, 217.0153515255709920 ) ) ;
#47726=CARTESIAN_POINT ( 'NONE',  ( 20.10528729609999843, 1430.878053336090034, 215.1856554784289983 ) ) ;
#47727=CARTESIAN_POINT ( 'NONE',  ( -3.696289592874629548, 1429.417634134486434, 201.6803503126470218 ) ) ;
#47729=VERTEX_POINT ( 'NONE', #12506 ) ;
#47732=CARTESIAN_POINT ( 'NONE',  ( 12.49505606288779980, 1500.014223150440102, 206.9771888552629662 ) ) ;
#47733=CARTESIAN_POINT ( 'NONE',  ( -16.86744945587559741, 1508.551704408389924, 210.3912200788219877 ) ) ;
#47737=DIRECTION ( 'NONE',  ( 0.6480245870892008542, 0.000000000000000000, -0.7616194158028475325 ) ) ;
#47742=CARTESIAN_POINT ( 'NONE',  ( 9.387051760214630391, 1462.123984385330004, 206.5521735341949920 ) ) ;
#47759=CIRCLE ( 'NONE', #40631, 2.458500000000000352 ) ;
#47768=CARTESIAN_POINT ( 'NONE',  ( -3.837713176184200048, 1483.349439374189842, 199.1769404390510090 ) ) ;
#47769=CARTESIAN_POINT ( 'NONE',  ( -10.93667282414601694, 1508.551702216402191, 207.6442590326176401 ) ) ;
#47776=CARTESIAN_POINT ( 'NONE',  ( -7.618671585723859607, 1439.752128060139967, 204.7697547506639921 ) ) ;
#47778=CARTESIAN_POINT ( 'NONE',  ( 8.135441375949998388, 1421.256651981180084, 196.0379973919989709 ) ) ;
#47781=CARTESIAN_POINT ( 'NONE',  ( -18.26050052379999755, 1504.444625823090064, 209.3988868026209786 ) ) ;
#47787=CARTESIAN_POINT ( 'NONE',  ( 0.7050289746089989373, 1515.139588934790027, 213.4493361341789921 ) ) ;
#47791=CARTESIAN_POINT ( 'NONE',  ( -0.4918821362568480682, 1463.495325596601333, 199.3433850722970817 ) ) ;
#47793=CARTESIAN_POINT ( 'NONE',  ( -6.570337678066239917, 1439.978317356713887, 203.3223113697309259 ) ) ;
#47797=CARTESIAN_POINT ( 'NONE',  ( -2.367088349510000356, 1507.435255637589989, 221.3405631526989907 ) ) ;
#47798=CARTESIAN_POINT ( 'NONE',  ( -10.26603356420000068, 1498.779766624589911, 214.4369877271390123 ) ) ;
#47808=CARTESIAN_POINT ( 'NONE',  ( -9.234134023826198856, 1461.205490114660051, 206.1827678865119822 ) ) ;
#47811=CARTESIAN_POINT ( 'NONE',  ( 12.26176529699089990, 1491.759805890980033, 208.0003969321799957 ) ) ;
#47820=CARTESIAN_POINT ( 'NONE',  ( 18.28862923867550094, 1430.119187293129926, 201.0315415175020064 ) ) ;
#47824=CARTESIAN_POINT ( 'NONE',  ( -7.099928628730000746, 1453.632733172990129, 202.8366510152990259 ) ) ;
#47827=CARTESIAN_POINT ( 'NONE',  ( 7.531671725839999887, 1426.336758191899889, 212.2880588734690264 ) ) ;
#47829=CARTESIAN_POINT ( 'NONE',  ( 24.04367183769999983, 1494.655699983489967, 207.1743773500889745 ) ) ;
#47842=CARTESIAN_POINT ( 'NONE',  ( 2.329906352153470195, 1515.372228416580128, 204.8601837675520017 ) ) ;
#47846=CARTESIAN_POINT ( 'NONE',  ( -3.783954225830480134, 1462.812684261019967, 200.1151939703100027 ) ) ;
#47857=CARTESIAN_POINT ( 'NONE',  ( 11.86874272849999912, 1492.043035549590059, 209.5970695671510100 ) ) ;
#47859=CIRCLE ( 'NONE', #89001, 0.4999999999999449329 ) ;
#47881=CARTESIAN_POINT ( 'NONE',  ( 21.04904418909999819, 1494.916427559390058, 209.1218459616989946 ) ) ;
#47885=VECTOR ( 'NONE', #70181, 1000.000000000000000 ) ;
#47888=CARTESIAN_POINT ( 'NONE',  ( 11.99250861867660056, 1492.789266563229830, 212.0938347205880063 ) ) ;
#47903=CARTESIAN_POINT ( 'NONE',  ( 10.95509605640000039, 1422.839500331020190, 206.5757350954289961 ) ) ;
#47904=CARTESIAN_POINT ( 'NONE',  ( 0.7581006759604393963, 1498.651877382277689, 197.8214185162987917 ) ) ;
#47906=CARTESIAN_POINT ( 'NONE',  ( -15.85591190879999779, 1415.880081504350073, 209.4912631162540038 ) ) ;
#47917=CARTESIAN_POINT ( 'NONE',  ( 9.625916079488465726, 1425.428719264066558, 195.5010095755044119 ) ) ;
#47918=CARTESIAN_POINT ( 'NONE',  ( 2.713660715419999647, 1441.511099666689915, 218.6663635638090000 ) ) ;
#47930=CARTESIAN_POINT ( 'NONE',  ( -15.46794562779999893, 1508.541555192090073, 214.7748198980189898 ) ) ;
#47932=EDGE_CURVE ( 'NONE', #97755, #74404, #12183, .T. ) ;
#47939=CARTESIAN_POINT ( 'NONE',  ( -9.139715296915689180, 1438.756510518619962, 209.0162231784520088 ) ) ;
#47942=CARTESIAN_POINT ( 'NONE',  ( -14.87973836575140041, 1415.677402202029953, 206.9056846400189897 ) ) ;
#47943=DIRECTION ( 'NONE',  ( -1.000000000000000000, 0.000000000000000000, 0.000000000000000000 ) ) ;
#47944=CARTESIAN_POINT ( 'NONE',  ( 7.987221624930000985, 1428.707470559690137, 214.3354289489490156 ) ) ;
#47946=ORIENTED_EDGE ( 'NONE', *, *, #107050, .F. ) ;
#47950=ORIENTED_EDGE ( 'NONE', *, *, #60374, .F. ) ;
#47951=CARTESIAN_POINT ( 'NONE',  ( -12.75386558790000002, 1502.395049388389907, 210.0740108765389778 ) ) ;
#47952=CARTESIAN_POINT ( 'NONE',  ( -8.589426147275000645, 1436.798469860880004, 209.9038450004319998 ) ) ;
#47961=CARTESIAN_POINT ( 'NONE',  ( 0.9669097429690169943, 1515.111355597249940, 213.4500754500990070 ) ) ;
#47962=CARTESIAN_POINT ( 'NONE',  ( -19.97968237250000101, 1483.906011188890034, 214.0068283976289933 ) ) ;
#47968=ORIENTED_EDGE ( 'NONE', *, *, #70625, .F. ) ;
#47973=CARTESIAN_POINT ( 'NONE',  ( 13.58730094343779982, 1498.318843676340066, 227.8486215837370139 ) ) ;
#47984=CARTESIAN_POINT ( 'NONE',  ( -3.440623305239999929, 1458.093607836889760, 219.2469823057990084 ) ) ;
#48001=B_SPLINE_CURVE_WITH_KNOTS ( 'NONE', 5,
 ( #62223, #53828, #70082, #44869, #45418, #71177, #104195, #53264, #85729 ),
 .UNSPECIFIED., .F., .F.,
 ( 6, 3, 6 ),
 ( 463.1457853109999974, 468.8934854820000169, 473.5625621899999942 ),
 .UNSPECIFIED. ) ;
#48007=CARTESIAN_POINT ( 'NONE',  ( -6.682617376610000548, 1481.590913066989970, 205.7929905812889899 ) ) ;
#48015=CARTESIAN_POINT ( 'NONE',  ( 2.199364402880799929, 1426.043163797689886, 191.2103802779980128 ) ) ;
#48033=CARTESIAN_POINT ( 'NONE',  ( -2.480175256589999933, 1429.207669907389800, 200.0830570456390092 ) ) ;
#48035=CARTESIAN_POINT ( 'NONE',  ( -7.982037141949999359, 1424.874072662569915, 210.5243721551090061 ) ) ;
#48045=CARTESIAN_POINT ( 'NONE',  ( -4.692099526989998992, 1474.463958302690116, 198.6947328130989945 ) ) ;
#48053=B_SPLINE_CURVE_WITH_KNOTS ( 'NONE', 5,
 ( #39654, #62842, #96955, #20221, #54422, #11838 ),
 .UNSPECIFIED., .F., .F.,
 ( 6, 6 ),
 ( 0.9643540072699122723, 1.000000000000000000 ),
 .UNSPECIFIED. ) ;
#48055=CARTESIAN_POINT ( 'NONE',  ( 1.722617949397659887, 1456.338984862310099, 198.6776180596440042 ) ) ;
#48063=B_SPLINE_CURVE_WITH_KNOTS ( 'NONE', 5,
 ( #76581, #41334, #75504, #74951, #109638, #25051, #91724, #33453, #8809 ),
 .UNSPECIFIED., .F., .F.,
 ( 6, 3, 6 ),
 ( -12.51705759590000078, -7.545169656169999683, -3.809711666909999295 ),
 .UNSPECIFIED. ) ;
#48066=CARTESIAN_POINT ( 'NONE',  ( -4.304668157050000055, 1442.652147467789973, 200.8964050455090273 ) ) ;
#48067=CARTESIAN_POINT ( 'NONE',  ( 7.815357466500000072, 1423.735213141060058, 195.8220613176989957 ) ) ;
#48071=DIRECTION ( 'NONE',  ( 0.8775825618903763115, 0.000000000000000000, -0.4794255386041963996 ) ) ;
#48079=CARTESIAN_POINT ( 'NONE',  ( 3.196970390959999797, 1490.438169550290013, 188.4165637325990303 ) ) ;
#48082=EDGE_CURVE ( 'NONE', #288, #1510, #71270, .T. ) ;
#48084=CARTESIAN_POINT ( 'NONE',  ( 2.968682044221400140, 1508.551704408389924, 204.1814749987780147 ) ) ;
#48086=EDGE_LOOP ( 'NONE', ( #26933, #35284, #75407, #72256 ) ) ;
#48087=CARTESIAN_POINT ( 'NONE',  ( 22.24401761576379855, 1475.958701603000009, 209.7631723292300023 ) ) ;
#48092=FACE_OUTER_BOUND ( 'NONE', #20357, .T. ) ;
#48094=CARTESIAN_POINT ( 'NONE',  ( 3.958338146192914131, 1515.551704408294881, 211.4519800820672799 ) ) ;
#48095=CARTESIAN_POINT ( 'NONE',  ( 7.729166927079999638, 1490.261404644089907, 208.7262156379529756 ) ) ;
#48098=CARTESIAN_POINT ( 'NONE',  ( -2.016889697369080192, 1485.643995215409859, 197.3940317714459809 ) ) ;
#48122=CARTESIAN_POINT ( 'NONE',  ( -8.891021255688182023, 1447.878015951419911, 211.6948139168939917 ) ) ;
#48127=CARTESIAN_POINT ( 'NONE',  ( 4.329341231296368164, 1515.068899845852911, 206.1636068449589629 ) ) ;
#48128=CARTESIAN_POINT ( 'NONE',  ( 6.826200034800000260, 1424.874072630889941, 213.4902541782590220 ) ) ;
#48131=AXIS2_PLACEMENT_3D ( 'NONE', #98899, #30602, #82099 ) ;
#48138=CARTESIAN_POINT ( 'NONE',  ( -2.194060776939999791, 1486.670284103789982, 220.4458495409990064 ) ) ;
#48145=CARTESIAN_POINT ( 'NONE',  ( 10.93416347059999794, 1501.622886110689933, 205.7061242847990172 ) ) ;
#48146=ORIENTED_EDGE ( 'NONE', *, *, #87461, .F. ) ;
#48158=FACE_OUTER_BOUND ( 'NONE', #39528, .T. ) ;
#48165=CARTESIAN_POINT ( 'NONE',  ( -3.154911953494088372, 1432.397052738174352, 216.9484949157356652 ) ) ;
#48173=CARTESIAN_POINT ( 'NONE',  ( 11.61220494760000044, 1420.579219889470096, 199.3493800206389892 ) ) ;
#48174=CARTESIAN_POINT ( 'NONE',  ( 19.28172097450000066, 1455.754227538689975, 211.0042463156089809 ) ) ;
#48176=CARTESIAN_POINT ( 'NONE',  ( 10.04874238532330111, 1480.247552555629909, 205.9343909418280134 ) ) ;
#48180=CARTESIAN_POINT ( 'NONE',  ( 10.67027879645779898, 1424.424156321159899, 206.6093414022110153 ) ) ;
#48181=CARTESIAN_POINT ( 'NONE',  ( -9.702105246842089414, 1440.203813892860126, 206.6216695874250036 ) ) ;
#48186=CARTESIAN_POINT ( 'NONE',  ( 4.163336342339999869E-15, 1416.181292664740113, 209.1218459616989946 ) ) ;
#48190=CARTESIAN_POINT ( 'NONE',  ( 20.17014401999999862, 1476.180243796189870, 211.1081103605989995 ) ) ;
#48191=CARTESIAN_POINT ( 'NONE',  ( 11.30832794868720015, 1425.224311524470068, 202.9888470784990204 ) ) ;
#48193=CARTESIAN_POINT ( 'NONE',  ( 4.198346516710000031, 1429.752558846089869, 216.7561471261590214 ) ) ;
#48196=DIRECTION ( 'NONE',  ( 2.041467857569999829E-16, -1.000000000000000000, 5.573852046271030309E-16 ) ) ;
#48208=CARTESIAN_POINT ( 'NONE',  ( -7.898270967410000232, 1498.870872765589866, 219.0971900149289979 ) ) ;
#48211=CARTESIAN_POINT ( 'NONE',  ( 3.406070268200000140, 1459.762959874990202, 203.0322602957690208 ) ) ;
#48213=CARTESIAN_POINT ( 'NONE',  ( -0.7244299514709989785, 1515.369718807090067, 204.8338105401389839 ) ) ;
#48221=CARTESIAN_POINT ( 'NONE',  ( -0.3977757332677263613, 1484.209072442955403, 198.4342325285878985 ) ) ;
#48226=CARTESIAN_POINT ( 'NONE',  ( -1.516559207410000054, 1485.748721136590120, 197.3030500067990261 ) ) ;
#48227=CARTESIAN_POINT ( 'NONE',  ( 8.518975719829999349, 1479.750272970590004, 202.8267940536090066 ) ) ;
#48229=CARTESIAN_POINT ( 'NONE',  ( -12.12815397179999977, 1490.956868768189906, 207.2466138458389935 ) ) ;
#48237=CARTESIAN_POINT ( 'NONE',  ( -12.15078451844060048, 1490.894239016419988, 207.4451287176520111 ) ) ;
#48238=CARTESIAN_POINT ( 'NONE',  ( -4.476507717933579933, 1508.551704408389924, 205.1212419221770062 ) ) ;
#48242=ORIENTED_EDGE ( 'NONE', *, *, #99362, .T. ) ;
#48244=CARTESIAN_POINT ( 'NONE',  ( 9.673908127945217927, 1470.479523918640098, 212.0206101308270092 ) ) ;
#48253=CARTESIAN_POINT ( 'NONE',  ( -20.39463414511109818, 1465.749978440089990, 211.0547928264969926 ) ) ;
#48259=CYLINDRICAL_SURFACE ( 'NONE', #109839, 0.5000000000000022204 ) ;
#48266=CARTESIAN_POINT ( 'NONE',  ( 3.350944662710000355, 1464.628126271390101, 199.8699733667390035 ) ) ;
#48275=CARTESIAN_POINT ( 'NONE',  ( 11.44311714350000031, 1501.817457610490237, 208.4257029495360030 ) ) ;
#48280=CARTESIAN_POINT ( 'NONE',  ( -3.208637253543818346, 1515.551704408389696, 212.9514661164405709 ) ) ;
#48281=CARTESIAN_POINT ( 'NONE',  ( 8.197264105214189911, 1483.021012307500087, 216.7088607698530041 ) ) ;
#48286=CARTESIAN_POINT ( 'NONE',  ( 10.59813991459999905, 1477.524080022390081, 229.9254213492990004 ) ) ;
#48293=CARTESIAN_POINT ( 'NONE',  ( 12.42784828245430084, 1499.940815291620083, 206.6466454406019864 ) ) ;
#48297=TOROIDAL_SURFACE ( 'NONE', #8, 14.91144628110000170, 0.5000000000000000000 ) ;
#48299=CARTESIAN_POINT ( 'NONE',  ( 12.54251639656375161, 1420.481606446594924, 200.4267854580531889 ) ) ;
#48300=CARTESIAN_POINT ( 'NONE',  ( 0.8889729592620010390, 1465.607921463989896, 198.1135291515989820 ) ) ;
#48308=ORIENTED_EDGE ( 'NONE', *, *, #92582, .F. ) ;
#48311=ORIENTED_EDGE ( 'NONE', *, *, #89334, .F. ) ;
#48313=CARTESIAN_POINT ( 'NONE',  ( 3.885417831612716366, 1424.874073124720098, 216.2340555961886821 ) ) ;
#48316=CARTESIAN_POINT ( 'NONE',  ( -10.98772071141650031, 1462.627874614629945, 207.9149163331969987 ) ) ;
#48332=CARTESIAN_POINT ( 'NONE',  ( 3.829222805974359822, 1515.551704203360032, 211.9228896269929976 ) ) ;
#48335=ORIENTED_EDGE ( 'NONE', *, *, #58223, .F. ) ;
#48341=CARTESIAN_POINT ( 'NONE',  ( -8.922484925833558123, 1440.999120902360119, 204.4963729060849857 ) ) ;
#48346=CARTESIAN_POINT ( 'NONE',  ( -10.22049849524720067, 1480.811388884020062, 206.5019967615200187 ) ) ;
#48347=CARTESIAN_POINT ( 'NONE',  ( 6.596949724929999981, 1463.298537539390054, 209.1528258517670054 ) ) ;
#48356=CARTESIAN_POINT ( 'NONE',  ( -7.948879223625117341, 1438.924303876842714, 205.5137112676434299 ) ) ;
#48361=CARTESIAN_POINT ( 'NONE',  ( -4.325405444010000267, 1515.219201233190006, 210.9648094371690092 ) ) ;
#48376=CARTESIAN_POINT ( 'NONE',  ( 12.09325773686249939, 1491.439490036820189, 206.9352952286269840 ) ) ;
#48386=CARTESIAN_POINT ( 'NONE',  ( 18.68390456912029762, 1457.534965337250014, 220.6831945509709954 ) ) ;
#48387=CARTESIAN_POINT ( 'NONE',  ( -15.98290998149800046, 1416.244087889359889, 209.6359233886850006 ) ) ;
#48391=CARTESIAN_POINT ( 'NONE',  ( -8.170885357179999531, 1451.453810839889911, 203.6936318906290069 ) ) ;
#48394=CARTESIAN_POINT ( 'NONE',  ( 7.363774774100000364, 1426.339825040939786, 212.6604317995690110 ) ) ;
#48401=EDGE_LOOP ( 'NONE', ( #13952, #82778, #109245, #16248 ) ) ;
#48406=DIRECTION ( 'NONE',  ( 0.9386936612375377242, 0.3031620644484189775, 0.1641553320237859603 ) ) ;
#48410=CARTESIAN_POINT ( 'NONE',  ( 2.551450060280000098, 1445.555848560289860, 200.0930493208989844 ) ) ;
#48411=CARTESIAN_POINT ( 'NONE',  ( -21.52452246478599918, 1505.819333768819888, 209.2233725332250174 ) ) ;
#48416=CARTESIAN_POINT ( 'NONE',  ( 4.647212535750000484, 1424.553094292009973, 191.7362356993989749 ) ) ;
#48435=CARTESIAN_POINT ( 'NONE',  ( -12.78956172709999883, 1502.763085786289821, 208.8827437375920226 ) ) ;
#48441=ORIENTED_EDGE ( 'NONE', *, *, #32448, .T. ) ;
#48444=CARTESIAN_POINT ( 'NONE',  ( -7.446870712126620440, 1453.253929861869892, 203.4788461265429760 ) ) ;
#48445=B_SPLINE_SURFACE_WITH_KNOTS ( 'NONE', 5, 1, ( 
 ( #101361, #43701 ),
 ( #44263, #42045 ),
 ( #77854, #35293 ),
 ( #17354, #24651 ),
 ( #8421, #50462 ),
 ( #95203, #76197 ) ),
 .UNSPECIFIED., .F., .F., .F.,
 ( 6, 6 ),
 ( 2, 2 ),
 ( 0.000000000000000000, 4.008920757899999465 ),
 ( 0.000000000000000000, 14.00000000000000000 ),
 .UNSPECIFIED. ) ;
#48459=CARTESIAN_POINT ( 'NONE',  ( 12.24972954961170046, 1492.464136767450100, 210.6849265718639970 ) ) ;
#48473=CARTESIAN_POINT ( 'NONE',  ( 11.62117845040000041, 1421.988945507780045, 205.3376110126490062 ) ) ;
#48485=CARTESIAN_POINT ( 'NONE',  ( 10.95263331896989811, 1461.248509904520006, 209.5029505453279910 ) ) ;
#48486=CARTESIAN_POINT ( 'NONE',  ( 8.956968256945643247, 1424.994159167145881, 195.6940687255158480 ) ) ;
#48487=CARTESIAN_POINT ( 'NONE',  ( 0.5411951686119990113, 1444.367775260089957, 218.0750552485089884 ) ) ;
#48500=B_SPLINE_CURVE_WITH_KNOTS ( 'NONE', 3,
 ( #104211, #44885, #10148, #45975, #62238, #11806, #17978, #61685, #60582, #26958, #96923, #2336, #34798, #52173, #79035, #35915 ),
 .UNSPECIFIED., .F., .F.,
 ( 4, 3, 3, 3, 3, 4 ),
 ( -7.293777645795730180, -6.759547601150760698, -5.814523359711800232, -4.874165951496349791, -3.935888733346409651, -3.000356897310000548 ),
 .UNSPECIFIED. ) ;
#48501=CARTESIAN_POINT ( 'NONE',  ( 11.20607753534230078, 1470.380238220569936, 207.2284536391540257 ) ) ;
#48509=CARTESIAN_POINT ( 'NONE',  ( -15.01193293222859815, 1415.677402202029953, 207.4711775341719999 ) ) ;
#48519=B_SPLINE_CURVE_WITH_KNOTS ( 'NONE', 5,
 ( #42474, #33501, #76631, #93422, #9430, #74997 ),
 .UNSPECIFIED., .F., .F.,
 ( 6, 6 ),
 ( 0.000000000000000000, 1.000000000000000000 ),
 .UNSPECIFIED. ) ;
#48521=CARTESIAN_POINT ( 'NONE',  ( 4.758389699129999428, 1454.760432536389999, 217.3925755712789964 ) ) ;
#48537=CARTESIAN_POINT ( 'NONE',  ( -13.43029793530000049, 1505.160453439490084, 208.9607663354669853 ) ) ;
#48538=CARTESIAN_POINT ( 'NONE',  ( 24.07100108422400098, 1495.446790078319964, 207.0356552236710002 ) ) ;
#48547=CARTESIAN_POINT ( 'NONE',  ( 10.03041208372980009, 1469.257739677249901, 209.6369766770589820 ) ) ;
#48548=CARTESIAN_POINT ( 'NONE',  ( -6.124734198089999637, 1458.063336725389945, 216.4789210408089843 ) ) ;
#48567=CARTESIAN_POINT ( 'NONE',  ( -17.29525745463784503, 1505.122270163578605, 223.1329967567506856 ) ) ;
#48569=( BOUNDED_CURVE ( )  B_SPLINE_CURVE ( 3, ( #803, #68017, #34932, #59598 ),
 .UNSPECIFIED., .F., .F. ) 
 B_SPLINE_CURVE_WITH_KNOTS ( ( 4, 4 ),
 ( 1.018872757951490016, 2.122719868645289942 ),
 .UNSPECIFIED. ) 
 CURVE ( )  GEOMETRIC_REPRESENTATION_ITEM ( )  RATIONAL_B_SPLINE_CURVE ( ( 1.000000000000000000, 0.9010116851119320813, 0.9010116851119320813, 1.000000000000000000 ) ) 
 REPRESENTATION_ITEM ( '' )  );
#48575=ORIENTED_EDGE ( 'NONE', *, *, #38800, .T. ) ;
#48578=CARTESIAN_POINT ( 'NONE',  ( 10.92857032808210072, 1460.888924644350027, 208.5047758900509791 ) ) ;
#48583=CARTESIAN_POINT ( 'NONE',  ( 8.447516053086825849, 1461.289618066398816, 204.2828433158165069 ) ) ;
#48585=CARTESIAN_POINT ( 'NONE',  ( 7.752047435854870550, 1438.685045526630120, 214.1104276491739711 ) ) ;
#48586=CARTESIAN_POINT ( 'NONE',  ( 4.760896992130000172, 1449.971761959190189, 190.6385172635989704 ) ) ;
#48589=ORIENTED_EDGE ( 'NONE', *, *, #94752, .F. ) ;
#48591=CARTESIAN_POINT ( 'NONE',  ( -10.50362050230000044, 1471.648827043890151, 207.7636308339789650 ) ) ;
#48600=CARTESIAN_POINT ( 'NONE',  ( 6.636923444789999849, 1488.278828811890207, 199.0403411110989964 ) ) ;
#48601=DIRECTION ( 'NONE',  ( -9.439841191556039654E-47, 1.000000000000000000, -1.836970198721029688E-16 ) ) ;
#48603=CARTESIAN_POINT ( 'NONE',  ( -18.16080229929628231, 1445.425848083091978, 203.8898520025014705 ) ) ;
#48611=CARTESIAN_POINT ( 'NONE',  ( -15.38373915201839992, 1508.451228047400036, 215.1348082370930115 ) ) ;
#48614=CARTESIAN_POINT ( 'NONE',  ( -3.009012269849999921, 1476.164698171590089, 219.7802673373990103 ) ) ;
#48624=CARTESIAN_POINT ( 'NONE',  ( -9.774084277346261729, 1471.600999675089952, 211.8492761500930328 ) ) ;
#48625=CARTESIAN_POINT ( 'NONE',  ( 9.999026927027419021, 1469.414161099939975, 210.1225948180470198 ) ) ;
#48629=CARTESIAN_POINT ( 'NONE',  ( 10.53896813186729986, 1480.812051149729996, 208.6340423618050011 ) ) ;
#48631=CIRCLE ( 'NONE', #82592, 0.4999999999999995559 ) ;
#48632=CARTESIAN_POINT ( 'NONE',  ( -4.077180901879999375, 1442.282981986689947, 201.0855821934289906 ) ) ;
#48635=CARTESIAN_POINT ( 'NONE',  ( 10.90534049613379963, 1422.234868131600251, 210.9169051273459843 ) ) ;
#48643=CARTESIAN_POINT ( 'NONE',  ( 11.50050621948940055, 1492.682587485599925, 212.1934388399340037 ) ) ;
#48644=CARTESIAN_POINT ( 'NONE',  ( -0.9025875204510009908, 1457.243920652990028, 219.7495316366990039 ) ) ;
#48645=ORIENTED_EDGE ( 'NONE', *, *, #35240, .F. ) ;
#48649=CARTESIAN_POINT ( 'NONE',  ( 4.333038849890169963, 1508.551704408389924, 204.9468833496109994 ) ) ;
#48651=ORIENTED_EDGE ( 'NONE', *, *, #67252, .F. ) ;
#48654=CARTESIAN_POINT ( 'NONE',  ( -3.582801916544020138, 1515.224507089990084, 205.0446044820039901 ) ) ;
#48657=CARTESIAN_POINT ( 'NONE',  ( -4.675540975309999681, 1462.620895424390028, 200.5633310686890241 ) ) ;
#48660=CARTESIAN_POINT ( 'NONE',  ( -15.94676957688830043, 1508.551704408389924, 213.8922084002869894 ) ) ;
#48664=CARTESIAN_POINT ( 'NONE',  ( 8.009065970051258532, 1433.461148587649859, 203.5451095248959916 ) ) ;
#48676=CARTESIAN_POINT ( 'NONE',  ( -15.59398630749999981, 1420.072677430659951, 211.3401063871789916 ) ) ;
#48687=CARTESIAN_POINT ( 'NONE',  ( 7.476667830162710082, 1425.276938917010057, 212.2943805765499690 ) ) ;
#48695=CARTESIAN_POINT ( 'NONE',  ( -1.450932694090000252, 1486.832070779689957, 220.2329197926989934 ) ) ;
#48702=CARTESIAN_POINT ( 'NONE',  ( 11.45577226660000036, 1502.286415424589904, 208.3140783707030153 ) ) ;
#48710=PLANE ( 'NONE',  #72446 ) ;
#48711=EDGE_CURVE ( 'NONE', #59235, #43039, #67804, .T. ) ;
#48717=CARTESIAN_POINT ( 'NONE',  ( -6.545266366469999930, 1426.912378977409844, 203.3789669689390109 ) ) ;
#48726=CARTESIAN_POINT ( 'NONE',  ( -2.176449243140819778, 1508.203772142160233, 220.8519538129899900 ) ) ;
#48728=CARTESIAN_POINT ( 'NONE',  ( 10.41399337298259908, 1502.882161159430098, 216.4575550115480098 ) ) ;
#48729=CARTESIAN_POINT ( 'NONE',  ( 10.46140733719999893, 1420.326681975860083, 197.7779852210990157 ) ) ;
#48730=CARTESIAN_POINT ( 'NONE',  ( 0.9509688288689980284, 1431.491297202929900, 218.5646205313049961 ) ) ;
#48732=CARTESIAN_POINT ( 'NONE',  ( 10.19285232582329925, 1479.751836143369928, 205.9895992793150015 ) ) ;
#48736=CARTESIAN_POINT ( 'NONE',  ( 10.66784415300089961, 1424.355176726809987, 206.6195069038519989 ) ) ;
#48738=EDGE_CURVE ( 'NONE', #103217, #84181, #4083, .T. ) ;
#48747=CARTESIAN_POINT ( 'NONE',  ( 9.891757830708639787, 1427.006033834340087, 209.9233085989019969 ) ) ;
#48748=CARTESIAN_POINT ( 'NONE',  ( 11.05020669801949929, 1423.000693000939918, 203.3085683099579910 ) ) ;
#48751=CARTESIAN_POINT ( 'NONE',  ( 4.271857500090000315, 1429.250640823790036, 216.3852677031590019 ) ) ;
#48758=CARTESIAN_POINT ( 'NONE',  ( -6.148099858600874157, 1457.597472786487742, 216.4201080312880379 ) ) ;
#48761=EDGE_CURVE ( 'NONE', #60549, #62781, #66768, .T. ) ;
#48764=FACE_OUTER_BOUND ( 'NONE', #99084, .T. ) ;
#48766=CARTESIAN_POINT ( 'NONE',  ( -2.823272442860000009, 1474.899276188389877, 216.0777664757990237 ) ) ;
#48772=EDGE_CURVE ( 'NONE', #38113, #73081, #24589, .T. ) ;
#48784=B_SPLINE_CURVE_WITH_KNOTS ( 'NONE', 3,
 ( #108658, #90188, #13472, #31946, #98044, #82361, #48221, #5659, #47662, #49318, #21318, #55522, #89649, #47116, #81243, #38691, #107002, #65017, #30290, #81789, #5092 ),
 .UNSPECIFIED., .F., .F.,
 ( 4, 2, 1, 1, 1, 2, 2, 2, 1, 1, 2, 2, 4 ),
 ( 0.000000000000000000, 0.1250000000001823541, 0.1875000000002875200, 0.2187500000003548828, 0.2343750000003742007, 0.2421875000003838596, 0.2500000000003935186, 0.3750000000002933764, 0.4375000000002595146, 0.4687500000002259304, 0.4843750000002263745, 0.5000000000002269296, 1.000000000000000000 ),
 .UNSPECIFIED. ) ;
#48787=CARTESIAN_POINT ( 'NONE',  ( -11.10863372729999909, 1491.777316212490177, 207.8912015286890096 ) ) ;
#48790=CARTESIAN_POINT ( 'NONE',  ( -4.992349872352332518, 1391.620913799028131, 214.5306134754782761 ) ) ;
#48792=CARTESIAN_POINT ( 'NONE',  ( -17.71563513420000291, 1420.335625605900077, 207.4269338723890144 ) ) ;
#48797=CARTESIAN_POINT ( 'NONE',  ( -3.816599468434689779, 1508.551704408389924, 204.5159469375300034 ) ) ;
#48803=CARTESIAN_POINT ( 'NONE',  ( -9.234134023826198856, 1461.205490114660051, 206.1827678865119822 ) ) ;
#48804=CARTESIAN_POINT ( 'NONE',  ( 11.10467535518500171, 1471.705490391439980, 211.8499711634750042 ) ) ;
#48810=LINE ( 'NONE', #4588, #83899 ) ;
#48812=CARTESIAN_POINT ( 'NONE',  ( 11.78380890789823354, 1499.475951658889471, 204.3830416974864193 ) ) ;
#48816=DIRECTION ( 'NONE',  ( 1.224646799147350002E-16, -1.836970198721029688E-16, -1.000000000000000000 ) ) ;
#48825=EDGE_LOOP ( 'NONE', ( #80250, #100873, #81455, #9522, #102802 ) ) ;
#48830=CARTESIAN_POINT ( 'NONE',  ( 2.229471592959419990, 1485.171155440719758, 220.7696600089880121 ) ) ;
#48831=CARTESIAN_POINT ( 'NONE',  ( 11.83904535559999971, 1500.842106766089955, 208.3226773703530057 ) ) ;
#48835=EDGE_CURVE ( 'NONE', #2195, #26364, #18709, .T. ) ;
#48845=CARTESIAN_POINT ( 'NONE',  ( 19.38665381416110023, 1498.811973477250149, 221.8202357131370093 ) ) ;
#48847=ORIENTED_EDGE ( 'NONE', *, *, #31167, .T. ) ;
#48848=ORIENTED_EDGE ( 'NONE', *, *, #93114, .T. ) ;
#48855=CARTESIAN_POINT ( 'NONE',  ( 4.327507137520000491, 1515.138941066290045, 209.8355549535610010 ) ) ;
#48858=CARTESIAN_POINT ( 'NONE',  ( 1.153790625369999878, 1463.908919862690027, 199.3495073382590022 ) ) ;
#48865=ORIENTED_EDGE ( 'NONE', *, *, #108900, .T. ) ;
#48871=CARTESIAN_POINT ( 'NONE',  ( 7.801033191672110512, 1428.789703093460048, 214.5172910005400126 ) ) ;
#48873=CARTESIAN_POINT ( 'NONE',  ( -10.61991956690710026, 1462.990895942619773, 206.0507601276690082 ) ) ;
#48882=DIRECTION ( 'NONE',  ( 0.8775825618903700942, 0.000000000000000000, -0.4794255386042075018 ) ) ;
#48889=CARTESIAN_POINT ( 'NONE',  ( 4.136749811987169956, 1515.492902828930028, 212.0199439695689989 ) ) ;
#48894=CARTESIAN_POINT ( 'NONE',  ( 3.406451235749999640, 1507.508084657790050, 220.3277233380989912 ) ) ;
#48898=CARTESIAN_POINT ( 'NONE',  ( -5.466351949607379801, 1442.136625457690116, 201.6172741276789964 ) ) ;
#48899=CARTESIAN_POINT ( 'NONE',  ( -18.62956325327520091, 1444.934402157219893, 206.0431600358409980 ) ) ;
#48900=CARTESIAN_POINT ( 'NONE',  ( -7.866319717195060512, 1425.555983808420024, 204.1407689886210051 ) ) ;
#48902=EDGE_CURVE ( 'NONE', #24522, #77826, #11989, .T. ) ;
#48904=CARTESIAN_POINT ( 'NONE',  ( -17.70278889250000276, 1504.268309054989913, 209.3612281098589847 ) ) ;
#48906=ORIENTED_EDGE ( 'NONE', *, *, #1457, .T. ) ;
#48915=CARTESIAN_POINT ( 'NONE',  ( -10.19077500720859852, 1447.300597530319919, 210.8667737859159956 ) ) ;
#48927=CARTESIAN_POINT ( 'NONE',  ( -15.15772398740000071, 1439.441663529990137, 221.0618115286989962 ) ) ;
#48940=CARTESIAN_POINT ( 'NONE',  ( -19.83859993069999916, 1467.194195006989958, 209.1218459616989946 ) ) ;
#48942=CARTESIAN_POINT ( 'NONE',  ( -3.005262499256480258, 1450.300071509800091, 188.5532295967200014 ) ) ;
#48950=CARTESIAN_POINT ( 'NONE',  ( 7.231061069169999911, 1427.019244165460123, 212.9903255762889955 ) ) ;
#48962=EDGE_LOOP ( 'NONE', ( #84356, #41022, #97297, #23740 ) ) ;
#48966=CARTESIAN_POINT ( 'NONE',  ( 1.234729273729999965, 1445.364456438190018, 199.0923708265989944 ) ) ;
#48970=CARTESIAN_POINT ( 'NONE',  ( -1.139751506879999932, 1423.243574032600009, 191.2093741592990170 ) ) ;
#48987=CARTESIAN_POINT ( 'NONE',  ( -12.40467953689999980, 1502.876200019789849, 208.6411846686590081 ) ) ;
#48990=ORIENTED_EDGE ( 'NONE', *, *, #63669, .T. ) ;
#49000=DIRECTION ( 'NONE',  ( 9.261055619630009070E-47, -1.000000000000000000, 1.836970198721029688E-16 ) ) ;
#49008=CARTESIAN_POINT ( 'NONE',  ( 2.975355613810000133, 1441.383001986190038, 218.5845790346389776 ) ) ;
#49023=CARTESIAN_POINT ( 'NONE',  ( 12.66524796160000044, 1426.904560545630147, 205.5255884876389985 ) ) ;
#49024=CARTESIAN_POINT ( 'NONE',  ( -0.4036693690347583630, 1498.351677242009828, 197.8065570372807827 ) ) ;
#49034=CIRCLE ( 'NONE', #16754, 2.458500000000000352 ) ;
#49037=CARTESIAN_POINT ( 'NONE',  ( 10.78159844869479933, 1461.896569297480028, 211.1674770051990038 ) ) ;
#49038=CARTESIAN_POINT ( 'NONE',  ( 8.375776142020290749, 1424.393421303552714, 195.8297818163817112 ) ) ;
#49039=CARTESIAN_POINT ( 'NONE',  ( -0.7466494764550010155, 1444.875944096290141, 218.0743976162490014 ) ) ;
#49050=B_SPLINE_CURVE_WITH_KNOTS ( 'NONE', 3,
 ( #41510, #32556, #100835, #58314, #50472, #82416, #92436, #15712, #84048, #42058, #7347, #39855 ),
 .UNSPECIFIED., .F., .F.,
 ( 4, 2, 2, 2, 2, 4 ),
 ( -0.09623281651891979482, -0.08712861168082250418, -0.07809605755948040295, -0.05948248759999250068, -0.03461062426328559427, -2.460911216473071761E-08 ),
 .UNSPECIFIED. ) ;
#49052=CARTESIAN_POINT ( 'NONE',  ( 11.16354646297939901, 1470.309690817349747, 207.0219044217840008 ) ) ;
#49053=CARTESIAN_POINT ( 'NONE',  ( 11.41287573240554032, 1427.618782186570115, 209.6357587079445182 ) ) ;
#49057=CARTESIAN_POINT ( 'NONE',  ( -8.833352578285419199, 1438.178637326770058, 209.2923841634130042 ) ) ;
#49058=CARTESIAN_POINT ( 'NONE',  ( -4.138326087764060190, 1515.492270357739926, 211.4517668545689730 ) ) ;
#49072=CARTESIAN_POINT ( 'NONE',  ( 4.199771657899999511, 1453.975215170089996, 217.5101452743190009 ) ) ;
#49080=CARTESIAN_POINT ( 'NONE',  ( -4.187288789294350444, 1453.810560376779904, 199.5230725183479876 ) ) ;
#49087=CARTESIAN_POINT ( 'NONE',  ( -2.161027938733468545, 1508.551740403373060, 220.4424620650312363 ) ) ;
#49088=CARTESIAN_POINT ( 'NONE',  ( -21.44083287200000143, 1507.004319579390085, 216.1313484145690040 ) ) ;
#49091=( BOUNDED_CURVE ( )  B_SPLINE_CURVE ( 3, ( #16631, #15539, #49738, #76025 ),
 .UNSPECIFIED., .F., .T. ) 
 B_SPLINE_CURVE_WITH_KNOTS ( ( 4, 4 ),
 ( 1.008471431651680073, 2.133121240772390070 ),
 .UNSPECIFIED. ) 
 CURVE ( )  GEOMETRIC_REPRESENTATION_ITEM ( )  RATIONAL_B_SPLINE_CURVE ( ( 1.000000000000000000, 0.8973452434195507976, 0.8973452434195507976, 1.000000000000000000 ) ) 
 REPRESENTATION_ITEM ( '' )  );
#49095=CARTESIAN_POINT ( 'NONE',  ( -20.60448988230000111, 1484.737042837089803, 209.1218459616989946 ) ) ;
#49097=CARTESIAN_POINT ( 'NONE',  ( -3.550708236880000257, 1457.374719892490020, 218.1022976105089981 ) ) ;
#49101=CARTESIAN_POINT ( 'NONE',  ( -4.329448781177520189, 1515.064792686469900, 210.9648092169189795 ) ) ;
#49113=B_SPLINE_SURFACE_WITH_KNOTS ( 'NONE', 5, 1, ( 
 ( #66049, #5006 ),
 ( #22884, #57094 ),
 ( #12854, #91219 ),
 ( #47035, #72784 ),
 ( #107462, #55981 ),
 ( #39153, #62574 ) ),
 .UNSPECIFIED., .F., .F., .F.,
 ( 6, 6 ),
 ( 2, 2 ),
 ( 0.000000000000000000, 14.21110430600000107 ),
 ( 0.000000000000000000, 14.00000000000000000 ),
 .UNSPECIFIED. ) ;
#49125=ORIENTED_EDGE ( 'NONE', *, *, #39902, .T. ) ;
#49128=CARTESIAN_POINT ( 'NONE',  ( 1.809416385432540242, 1425.955702030009888, 191.1749219456789888 ) ) ;
#49135=CARTESIAN_POINT ( 'NONE',  ( 8.306907985085359769, 1439.017606053439977, 211.8916603637549940 ) ) ;
#49141=CIRCLE ( 'NONE', #70839, 0.4999999999999995559 ) ;
#49143=ORIENTED_EDGE ( 'NONE', *, *, #37884, .F. ) ;
#49149=CARTESIAN_POINT ( 'NONE',  ( 10.83224975562239933, 1490.714117854160122, 210.9222104128400019 ) ) ;
#49150=CARTESIAN_POINT ( 'NONE',  ( 9.061725897470001456, 1489.261074100890028, 201.5581573919090204 ) ) ;
#49158=CARTESIAN_POINT ( 'NONE',  ( -3.349195415509999663, 1474.892783691989962, 198.1874921133990028 ) ) ;
#49160=EDGE_CURVE ( 'NONE', #86968, #642, #89525, .T. ) ;
#49161=CARTESIAN_POINT ( 'NONE',  ( -13.82287742442830059, 1508.446990094839748, 216.5222845503169822 ) ) ;
#49162=CARTESIAN_POINT ( 'NONE',  ( -2.127304298620000367, 1475.553256189390140, 219.6136142033990097 ) ) ;
#49165=CARTESIAN_POINT ( 'NONE',  ( -7.077403913657799528, 1508.382900477385647, 219.7413862116793268 ) ) ;
#49171=CARTESIAN_POINT ( 'NONE',  ( -9.842598580781601214, 1471.074680866249992, 212.0444714742759800 ) ) ;
#49172=CARTESIAN_POINT ( 'NONE',  ( 4.327871496238250515, 1515.125026768150065, 208.3313100357229928 ) ) ;
#49173=LINE ( 'NONE', #83305, #97564 ) ;
#49177=CIRCLE ( 'NONE', #38363, 15.09021984820000029 ) ;
#49178=CARTESIAN_POINT ( 'NONE',  ( 10.53150541081210001, 1481.128416490849986, 211.0448888799710119 ) ) ;
#49180=CARTESIAN_POINT ( 'NONE',  ( -3.258755850400000043, 1441.659648558289973, 200.8802078077489739 ) ) ;
#49181=CARTESIAN_POINT ( 'NONE',  ( 11.38148961198079867, 1502.618718762939807, 211.1685771008779966 ) ) ;
#49182=CARTESIAN_POINT ( 'NONE',  ( -1829.302631503789826, 11216.44053380569858, -1188.015784187918598 ) ) ;
#49183=AXIS2_PLACEMENT_3D ( 'NONE', #71784, #62837, #106439 ) ;
#49185=CARTESIAN_POINT ( 'NONE',  ( -0.8041292380773119586, 1508.551704408389924, 220.0687458904899927 ) ) ;
#49191=CARTESIAN_POINT ( 'NONE',  ( 10.69502106051730017, 1492.057597410500193, 212.3896476547330110 ) ) ;
#49195=B_SPLINE_SURFACE_WITH_KNOTS ( 'NONE', 5, 1, ( 
 ( #14154, #82479 ),
 ( #30962, #84116 ),
 ( #92510, #66800 ),
 ( #65137, #108773 ),
 ( #39921, #57843 ),
 ( #49979, #6852 ),
 ( #99805, #40463 ),
 ( #15777, #24198 ),
 ( #100375, #99250 ) ),
 .UNSPECIFIED., .F., .F., .F.,
 ( 6, 3, 6 ),
 ( 2, 2 ),
 ( 0.000000000000000000, 3.461179286750000195, 6.897024932289999910 ),
 ( 0.000000000000000000, 14.00000000000000000 ),
 .UNSPECIFIED. ) ;
#49203=CARTESIAN_POINT ( 'NONE',  ( 3.584503077415259753, 1486.500511906220027, 219.3043361390229791 ) ) ;
#49204=CARTESIAN_POINT ( 'NONE',  ( -9.806574738260000146, 1463.377913006889912, 203.8363535297289957 ) ) ;
#49211=CARTESIAN_POINT ( 'NONE',  ( -1.956232596697950132, 1468.321003611494234, 219.3647435431511781 ) ) ;
#49220=CARTESIAN_POINT ( 'NONE',  ( 12.88439093021430004, 1420.965050148459795, 203.2552933692489887 ) ) ;
#49221=CARTESIAN_POINT ( 'NONE',  ( -1.550651194838236657, 1515.551704408390606, 213.0145024707716175 ) ) ;
#49222=CARTESIAN_POINT ( 'NONE',  ( -15.57808732350000014, 1420.358151750999923, 210.5578191881789678 ) ) ;
#49229=CARTESIAN_POINT ( 'NONE',  ( -1.637338503800000122, 1444.255706267190135, 199.2007328904890073 ) ) ;
#49236=CARTESIAN_POINT ( 'NONE',  ( 7.201669765347830321, 1424.954475730090053, 212.8464732492809901 ) ) ;
#49237=ORIENTED_EDGE ( 'NONE', *, *, #29171, .F. ) ;
#49244=CARTESIAN_POINT ( 'NONE',  ( -1.952464535469999873, 1487.388627956889877, 219.9077361037989817 ) ) ;
#49250=CARTESIAN_POINT ( 'NONE',  ( 10.82976971369999930, 1461.788039422589918, 210.9060527513990166 ) ) ;
#49253=B_SPLINE_CURVE_WITH_KNOTS ( 'NONE', 3,
 ( #8340, #26811, #25687, #52031, #17272, #101281 ),
 .UNSPECIFIED., .F., .F.,
 ( 4, 2, 4 ),
 ( 0.000000000000000000, 0.5000000000000000000, 1.000000000000000000 ),
 .UNSPECIFIED. ) ;
#49258=FACE_OUTER_BOUND ( 'NONE', #47407, .T. ) ;
#49267=CARTESIAN_POINT ( 'NONE',  ( 10.51881725948639890, 1481.320945440649893, 214.4817285840509840 ) ) ;
#49269=CARTESIAN_POINT ( 'NONE',  ( 1.852152499140000019, 1428.774755345290032, 214.2804808353390058 ) ) ;
#49274=CARTESIAN_POINT ( 'NONE',  ( 5.662343758720000508, 1504.894618425089902, 220.5557215505990314 ) ) ;
#49275=CARTESIAN_POINT ( 'NONE',  ( 7.840123310800001022, 1421.694352030239997, 195.8842445130989915 ) ) ;
#49276=CARTESIAN_POINT ( 'NONE',  ( 1.338019250827790163, 1431.361302059610125, 218.5179660117710227 ) ) ;
#49277=CARTESIAN_POINT ( 'NONE',  ( -11.14995156302100021, 1492.106312947269998, 203.9618532963989992 ) ) ;
#49278=CARTESIAN_POINT ( 'NONE',  ( -5.387808366170000696, 1496.648306349289896, 199.2595289264190228 ) ) ;
#49282=CARTESIAN_POINT ( 'NONE',  ( 10.89583921004300038, 1423.141224889920068, 206.8676328055360045 ) ) ;
#49291=CARTESIAN_POINT ( 'NONE',  ( 20.21728935790000037, 1475.862786327189951, 209.1218459616989946 ) ) ;
#49292=CARTESIAN_POINT ( 'NONE',  ( 11.94906839412739963, 1421.563497253679998, 203.4275386238590215 ) ) ;
#49293=CARTESIAN_POINT ( 'NONE',  ( -11.02848016370420048, 1462.482799370420025, 208.5648133604260011 ) ) ;
#49295=CARTESIAN_POINT ( 'NONE',  ( -8.101358069183218547, 1477.152134414194506, 215.6221709765751484 ) ) ;
#49299=DIRECTION ( 'NONE',  ( 0.000000000000000000, 4.493040424372315268E-15, -1.000000000000000000 ) ) ;
#49301=CARTESIAN_POINT ( 'NONE',  ( -16.85895935491750208, 1420.422674679470219, 203.4210585105750226 ) ) ;
#49308=CARTESIAN_POINT ( 'NONE',  ( -2.175315985799999741, 1479.578773637490031, 229.4213946198989902 ) ) ;
#49311=CARTESIAN_POINT ( 'NONE',  ( -5.027589337301257899, 1391.774060041337634, 203.8075142969989884 ) ) ;
#49315=CARTESIAN_POINT ( 'NONE',  ( 4.203127346707122847, 1464.947251126380934, 200.1638074967223986 ) ) ;
#49318=CARTESIAN_POINT ( 'NONE',  ( -0.3078888690928980321, 1484.233364050224282, 198.4302670740845542 ) ) ;
#49322=ORIENTED_EDGE ( 'NONE', *, *, #37123, .T. ) ;
#49324=CARTESIAN_POINT ( 'NONE',  ( 0.000000000000000000, 1398.755125754900064, 209.1218459616989946 ) ) ;
#49327=ADVANCED_FACE ( 'NONE', ( #34538 ), #106246, .F. ) ;
#49328=CARTESIAN_POINT ( 'NONE',  ( -5.047164175452439672, 1434.247983095549898, 217.4094108637509919 ) ) ;
#49330=CARTESIAN_POINT ( 'NONE',  ( -17.62923792119999788, 1419.134474756159989, 207.1478831079190002 ) ) ;
#49335=CARTESIAN_POINT ( 'NONE',  ( 10.72891033486649981, 1425.799916289779958, 207.0245073530009847 ) ) ;
#49341=CARTESIAN_POINT ( 'NONE',  ( 5.102416067990000137, 1474.008965365689846, 219.3522235086990122 ) ) ;
#49343=CARTESIAN_POINT ( 'NONE',  ( 10.00447882353569895, 1469.985636142700059, 210.3446379253909981 ) ) ;
#49350=CARTESIAN_POINT ( 'NONE',  ( 2.475018581880529922, 1497.111080376900190, 196.9667223532030107 ) ) ;
#49351=CARTESIAN_POINT ( 'NONE',  ( 5.024380392590000355, 1446.652863129090065, 201.3514328607089965 ) ) ;
#49353=CARTESIAN_POINT ( 'NONE',  ( -2.824235741780000364, 1454.999275414490057, 199.7442147925889913 ) ) ;
#49356=VERTEX_POINT ( 'NONE', #76541 ) ;
#49373=CARTESIAN_POINT ( 'NONE',  ( 5.898235284490000119, 1476.924971998690125, 199.0552711020989705 ) ) ;
#49374=ADVANCED_FACE ( 'NONE', ( #59761 ), #28909, .F. ) ;
#49375=CARTESIAN_POINT ( 'NONE',  ( 12.70216927250840122, 1500.518191181640077, 209.0698827285919776 ) ) ;
#49380=CARTESIAN_POINT ( 'NONE',  ( -19.73707911742420151, 1467.795398142200156, 204.3773320539029896 ) ) ;
#49384=EDGE_CURVE ( 'NONE', #108726, #74706, #87726, .T. ) ;
#49387=CARTESIAN_POINT ( 'NONE',  ( 12.34885615716000018, 1499.864449722190102, 206.2962984148029761 ) ) ;
#49388=FACE_OUTER_BOUND ( 'NONE', #86522, .T. ) ;
#49399=ORIENTED_EDGE ( 'NONE', *, *, #56340, .T. ) ;
#49404=B_SPLINE_CURVE_WITH_KNOTS ( 'NONE', 5,
 ( #9410, #9958, #86117, #67683, #50865, #59828, #7747, #60945, #33481 ),
 .UNSPECIFIED., .F., .F.,
 ( 6, 3, 6 ),
 ( 0.000000000000000000, 0.6063230996941525452, 1.000000000000000000 ),
 .UNSPECIFIED. ) ;
#49411=CARTESIAN_POINT ( 'NONE',  ( -9.524909850325949279, 1462.104426478840196, 206.5005804455079783 ) ) ;
#49420=CARTESIAN_POINT ( 'NONE',  ( 20.12874795999999833, 1473.837606016890049, 209.1218459616989946 ) ) ;
#49433=VERTEX_POINT ( 'NONE', #18825 ) ;
#49435=CARTESIAN_POINT ( 'NONE',  ( 2.910278962130000480, 1507.875172689290139, 220.4768199434989810 ) ) ;
#49440=CARTESIAN_POINT ( 'NONE',  ( -5.068030367662819557, 1427.701625857500176, 201.2694279692279906 ) ) ;
#49444=CARTESIAN_POINT ( 'NONE',  ( -6.569077907430000529, 1472.000453839789998, 211.3893757832889833 ) ) ;
#49455=CARTESIAN_POINT ( 'NONE',  ( -10.93162295028230169, 1470.132889486390013, 212.2376398131100075 ) ) ;
#49457=FACE_OUTER_BOUND ( 'NONE', #21134, .T. ) ;
#49460=CARTESIAN_POINT ( 'NONE',  ( -8.606197445582770555, 1437.745991313129934, 208.0916336407960046 ) ) ;
#49461=CARTESIAN_POINT ( 'NONE',  ( -4.091781189539999808, 1515.531881637889910, 210.2416342621790193 ) ) ;
#49462=CARTESIAN_POINT ( 'NONE',  ( -18.74729292449999818, 1442.199705176290081, 209.1218459616989946 ) ) ;
#49479=CARTESIAN_POINT ( 'NONE',  ( 12.58642104890130042, 1421.533884203790194, 206.9918965626969793 ) ) ;
#49481=FACE_OUTER_BOUND ( 'NONE', #20088, .T. ) ;
#49485=CARTESIAN_POINT ( 'NONE',  ( -9.299413003310359471, 1446.922194731980198, 190.6945041834079859 ) ) ;
#49487=CARTESIAN_POINT ( 'NONE',  ( -20.43379628966849637, 1466.940213777560075, 211.2182826552119934 ) ) ;
#49491=CARTESIAN_POINT ( 'NONE',  ( -15.92986207429999901, 1416.139014782290133, 209.7537124246929920 ) ) ;
#49492=EDGE_CURVE ( 'NONE', #3178, #67457, #93473, .T. ) ;
#49493=CARTESIAN_POINT ( 'NONE',  ( -4.523944061129999916, 1455.378620928990131, 200.8408218435490085 ) ) ;
#49498=CARTESIAN_POINT ( 'NONE',  ( -18.79896864135620049, 1419.283855142989978, 205.9425027332000013 ) ) ;
#49513=CARTESIAN_POINT ( 'NONE',  ( -0.1531850412299990138, 1444.288508142990167, 199.7853600647590042 ) ) ;
#49517=CARTESIAN_POINT ( 'NONE',  ( -3.357869919927010116, 1463.835494135860017, 199.7544149164289990 ) ) ;
#49533=CARTESIAN_POINT ( 'NONE',  ( -6.961461350099999557, 1472.923786193189926, 208.7096068999990166 ) ) ;
#49536=CARTESIAN_POINT ( 'NONE',  ( -11.37049282409999940, 1501.435198116990023, 207.7796432001189828 ) ) ;
#49539=ORIENTED_EDGE ( 'NONE', *, *, #8655, .F. ) ;
#49543=CARTESIAN_POINT ( 'NONE',  ( -9.173749095941850840, 1450.559996438570124, 208.1432995907519796 ) ) ;
#49549=CARTESIAN_POINT ( 'NONE',  ( -14.38287540707779932, 1508.551704408389924, 210.3535996512349868 ) ) ;
#49560=CARTESIAN_POINT ( 'NONE',  ( 9.627346003815750564, 1434.811529568090009, 207.3365483151889919 ) ) ;
#49569=CARTESIAN_POINT ( 'NONE',  ( -1.565589935376011876, 1494.863348305362479, 220.1740265712254541 ) ) ;
#49570=CARTESIAN_POINT ( 'NONE',  ( 6.284801111650899941, 1485.306667862180120, 217.9298748690059995 ) ) ;
#49583=CARTESIAN_POINT ( 'NONE',  ( 10.94239808399780145, 1461.353457147069776, 209.7851273180980058 ) ) ;
#49584=DIRECTION ( 'NONE',  ( -1.305148739725796033E-31, 1.000000000000000000, -1.836970198721029688E-16 ) ) ;
#49585=CARTESIAN_POINT ( 'NONE',  ( -1.329471185999999916, 1444.143595228889808, 218.0942866151389978 ) ) ;
#49596=CARTESIAN_POINT ( 'NONE',  ( -8.744120078331269141, 1440.655636409200042, 205.1339896302730210 ) ) ;
#49604=CARTESIAN_POINT ( 'NONE',  ( -9.126921779760198916, 1438.547899077590046, 209.4465929603159964 ) ) ;
#49605=CARTESIAN_POINT ( 'NONE',  ( -4.136749821589599918, 1515.492902831140100, 212.0199450294899748 ) ) ;
#49608=CARTESIAN_POINT ( 'NONE',  ( -9.519812938348620079, 1460.017558366200092, 210.6311618255110147 ) ) ;
#49619=CARTESIAN_POINT ( 'NONE',  ( 2.857814868949999809, 1456.075906465790013, 218.9302595098089910 ) ) ;
#49620=CARTESIAN_POINT ( 'NONE',  ( 1.813411856763470054, 1456.528622295709965, 219.5870533402340072 ) ) ;
#49621=CARTESIAN_POINT ( 'NONE',  ( -2.363918620589999797, 1443.448698872290151, 218.8950620034389942 ) ) ;
#49625=CARTESIAN_POINT ( 'NONE',  ( 9.699117481028789456, 1463.751773247410028, 210.5389327360290110 ) ) ;
#49629=CARTESIAN_POINT ( 'NONE',  ( 2.236830499208590339, 1495.676457082710158, 221.2569898128769807 ) ) ;
#49633=ORIENTED_EDGE ( 'NONE', *, *, #77581, .T. ) ;
#49634=EDGE_LOOP ( 'NONE', ( #77319, #106944, #58315, #40022 ) ) ;
#49636=CARTESIAN_POINT ( 'NONE',  ( 0.1433731509459970077, 1503.026203598089978, 233.3025785448990064 ) ) ;
#49638=CARTESIAN_POINT ( 'NONE',  ( -1.397588342842136067, 1473.980173416578509, 219.2767284909027978 ) ) ;
#49643=CARTESIAN_POINT ( 'NONE',  ( -20.40422799699999956, 1484.238920065389721, 212.0834907045089892 ) ) ;
#49644=CARTESIAN_POINT ( 'NONE',  ( 18.17843454563659833, 1431.368984425399731, 207.2510453969530033 ) ) ;
#49649=EDGE_LOOP ( 'NONE', ( #26377, #20702, #24704, #32719 ) ) ;
#49653=ORIENTED_EDGE ( 'NONE', *, *, #52310, .T. ) ;
#49656=CARTESIAN_POINT ( 'NONE',  ( 5.186873127341490530, 1424.212018954599898, 193.3034105768099948 ) ) ;
#49657=B_SPLINE_CURVE_WITH_KNOTS ( 'NONE', 5,
 ( #63630, #29980, #98293, #55778, #81479, #73675 ),
 .UNSPECIFIED., .F., .F.,
 ( 6, 6 ),
 ( 0.000000000000000000, 1.000000000000000000 ),
 .UNSPECIFIED. ) ;
#49661=TOROIDAL_SURFACE ( 'NONE', #24590, 11.23850026409999892, 0.5000000000000000000 ) ;
#49671=LINE ( 'NONE', #74871, #105339 ) ;
#49673=ORIENTED_EDGE ( 'NONE', *, *, #70951, .T. ) ;
#49674=ORIENTED_EDGE ( 'NONE', *, *, #25313, .T. ) ;
#49675=CARTESIAN_POINT ( 'NONE',  ( 19.01216659339999993, 1456.124166689789945, 212.8700632932389851 ) ) ;
#49677=B_SPLINE_CURVE_WITH_KNOTS ( 'NONE', 3,
 ( #7817, #8360, #92927, #49293, #77253, #51487, #84529, #42529, #91824, #6717, #50401, #102424, #25705, #75605, #85618, #16738, #109201, #24050, #15639, #59907, #49845, #94028, #8917, #41987, #58244, #83975, #7275, #41439, #33015, #35232, #53158, #26834, #69420, #87298, #2766, #79456, #28493 ),
 .UNSPECIFIED., .F., .F.,
 ( 4, 3, 3, 3, 3, 3, 3, 3, 3, 3, 3, 3, 4 ),
 ( -7.354143352820449842, -7.102020254820109457, -6.848251370393399817, -6.567365280386119331, -6.254732362112719990, -5.795795420936189934, -5.472496633131050281, -5.187277023006039656, -5.019032731589150309, -4.627402102584190047, -4.173454028035540553, -3.481905268385339536, -3.020409492390000672 ),
 .UNSPECIFIED. ) ;
#49685=CARTESIAN_POINT ( 'NONE',  ( 4.253771920025769759, 1442.472176597800171, 216.9083527837719885 ) ) ;
#49691=CARTESIAN_POINT ( 'NONE',  ( -10.21277674610000119, 1472.144828979990052, 207.6413912857090054 ) ) ;
#49694=CARTESIAN_POINT ( 'NONE',  ( 7.334060111060000331, 1482.070333873989966, 210.1443983621290101 ) ) ;
#49699=CARTESIAN_POINT ( 'NONE',  ( 8.613733814799999777, 1488.162647577689995, 202.3373066378090073 ) ) ;
#49711=CARTESIAN_POINT ( 'NONE',  ( 0.4394944473979990329, 1474.293113249590078, 219.5254300097989812 ) ) ;
#49714=CARTESIAN_POINT ( 'NONE',  ( -11.33492574265600084, 1471.089256498150007, 207.7878841706139781 ) ) ;
#49721=CARTESIAN_POINT ( 'NONE',  ( 4.328283507529889995, 1515.109292691759947, 208.1261415868569884 ) ) ;
#49730=DIRECTION ( 'NONE',  ( -0.9824080081115912355, 0.000000000000000000, -0.1867471702549089174 ) ) ;
#49733=CARTESIAN_POINT ( 'NONE',  ( -1.947517617149490121, 1508.551704408389924, 220.0725308712329991 ) ) ;
#49738=CARTESIAN_POINT ( 'NONE',  ( 4.546874241639798697, 1466.877133849231996, 217.9623086141598662 ) ) ;
#49740=CARTESIAN_POINT ( 'NONE',  ( 10.67479214083029859, 1490.933195892699814, 211.7486846328050092 ) ) ;
#49741=CARTESIAN_POINT ( 'NONE',  ( 1.003916534810000094, 1455.812332551789950, 218.6660764286289691 ) ) ;
#49745=CARTESIAN_POINT ( 'NONE',  ( 8.224891776136750821, 1436.419357605579989, 206.5810456655080145 ) ) ;
#49747=ORIENTED_EDGE ( 'NONE', *, *, #81481, .T. ) ;
#49748=LINE ( 'NONE', #16103, #58209 ) ;
#49752=CARTESIAN_POINT ( 'NONE',  ( -6.533716117800000056, 1463.955653170889946, 200.7628773010889915 ) ) ;
#49754=CARTESIAN_POINT ( 'NONE',  ( 2.508384027800000027, 1444.574164590290138, 203.3639928317590204 ) ) ;
#49756=CARTESIAN_POINT ( 'NONE',  ( -9.371448800484090569, 1508.551704408389924, 218.5138698305420064 ) ) ;
#49758=DIRECTION ( 'NONE',  ( -0.2781944220536289869, 0.3718881641442650099, -0.8856111205871658454 ) ) ;
#49761=CARTESIAN_POINT ( 'NONE',  ( 4.934384483489999695, 1432.131467662490195, 200.8226675911659811 ) ) ;
#49771=CARTESIAN_POINT ( 'NONE',  ( 1.063863508520000112, 1476.023003326389926, 197.6717150904989921 ) ) ;
#49777=CARTESIAN_POINT ( 'NONE',  ( -8.952944454599998991, 1424.162919053179849, 206.7489373822789673 ) ) ;
#49782=CARTESIAN_POINT ( 'NONE',  ( 7.401232516239121040, 1425.131641740689929, 212.4511809372470168 ) ) ;
#49787=CARTESIAN_POINT ( 'NONE',  ( -11.93165340550180176, 1491.195427457339974, 206.6891418979790274 ) ) ;
#49791=CARTESIAN_POINT ( 'NONE',  ( -4.644345245587025772, 1378.331153274604731, 214.5506328342511893 ) ) ;
#49800=B_SPLINE_CURVE_WITH_KNOTS ( 'NONE', 3,
 ( #6666, #49791, #57099, #66054, #55986, #5575, #81704, #22337, #91225, #40820, #108017, #100178, #39725, #109686 ),
 .UNSPECIFIED., .F., .F.,
 ( 4, 2, 2, 1, 1, 2, 2, 4 ),
 ( 0.000000000000000000, 0.2500000000026890712, 0.3750000000040576986, 0.4375000000044669823, 0.4687500000046716520, 0.4843750000049625859, 0.5000000000052535754, 1.000000000000000000 ),
 .UNSPECIFIED. ) ;
#49809=AXIS2_PLACEMENT_3D ( 'NONE', #20692, #12303, #46494 ) ;
#49811=CARTESIAN_POINT ( 'NONE',  ( 4.678144193461809763, 1508.611354624159958, 211.6097691212250140 ) ) ;
#49813=AXIS2_PLACEMENT_3D ( 'NONE', #77495, #41678, #795 ) ;
#49816=CARTESIAN_POINT ( 'NONE',  ( -7.703846517339999700, 1425.539117803740055, 205.4402351432489979 ) ) ;
#49818=ADVANCED_FACE ( 'NONE', ( #5073 ), #8086, .T. ) ;
#49824=CARTESIAN_POINT ( 'NONE',  ( -10.52288318266220024, 1480.315364330569992, 209.5795690133369931 ) ) ;
#49827=CARTESIAN_POINT ( 'NONE',  ( 9.921621853607028640, 1503.139275714190262, 217.1109786641990240 ) ) ;
#49828=CARTESIAN_POINT ( 'NONE',  ( 7.616185062369999592, 1421.938201076239693, 195.7452753503989697 ) ) ;
#49830=CARTESIAN_POINT ( 'NONE',  ( 10.41266471604430066, 1479.358872247189993, 205.9982438997039935 ) ) ;
#49834=CARTESIAN_POINT ( 'NONE',  ( 10.70954747716070088, 1424.785111699970230, 206.5629283040009909 ) ) ;
#49840=CARTESIAN_POINT ( 'NONE',  ( -17.30770383199540419, 1417.598457286296025, 206.4021992971377699 ) ) ;
#49844=CARTESIAN_POINT ( 'NONE',  ( 11.87355315023980040, 1421.630887076790032, 203.4247053331970108 ) ) ;
#49845=CARTESIAN_POINT ( 'NONE',  ( -10.92292198257390012, 1462.727308076620147, 207.4371260179439957 ) ) ;
#49849=CARTESIAN_POINT ( 'NONE',  ( 4.934393719438509684, 1432.131471246516185, 200.8226737949341612 ) ) ;
#49850=CARTESIAN_POINT ( 'NONE',  ( -9.684192816560390327, 1460.964679204169897, 209.2041052100069862 ) ) ;
#49853=CARTESIAN_POINT ( 'NONE',  ( 6.937455853977830600, 1464.940067841279870, 217.7536605638889853 ) ) ;
#49855=CARTESIAN_POINT ( 'NONE',  ( 4.090209565960320148, 1474.271260243390088, 219.7854241566030282 ) ) ;
#49857=CARTESIAN_POINT ( 'NONE',  ( -8.124763164904772239, 1425.330096299151137, 208.9405766535813314 ) ) ;
#49858=CARTESIAN_POINT ( 'NONE',  ( -0.3742911815734584757, 1477.585138614035486, 198.7218481745984775 ) ) ;
#49860=CARTESIAN_POINT ( 'NONE',  ( 1.842962231260000028, 1515.064792882589927, 204.7923971856590128 ) ) ;
#49862=CARTESIAN_POINT ( 'NONE',  ( -16.83568187507700031, 1418.884533216219779, 201.2565367485750016 ) ) ;
#49864=CARTESIAN_POINT ( 'NONE',  ( -19.43345977031810179, 1418.906471912719780, 207.3470523668889882 ) ) ;
#49869=CARTESIAN_POINT ( 'NONE',  ( 2.175409717514719593E-31, 1397.551704408390151, 209.1218459616989946 ) ) ;
#49874=B_SPLINE_SURFACE_WITH_KNOTS ( 'NONE', 5, 5, ( 
 ( #48657, #81662, #106872, #82231, #81123, #73293 ),
 ( #91184, #14463, #82783, #107427, #40229, #74412 ),
 ( #108537, #20650, #4441, #54853, #30723, #3904 ),
 ( #30165, #92282, #67111, #17193, #49752, #93380 ),
 ( #24509, #83882, #101769, #84973, #50843, #15006 ),
 ( #32387, #6628, #91732, #41342, #83332, #40782 ),
 ( #15552, #50312, #32921, #7187, #84441, #49204 ),
 ( #34033, #109108, #101213, #42431, #23422, #67662 ),
 ( #66014, #58700, #66570, #33460, #25060, #59262 ) ),
 .UNSPECIFIED., .F., .F., .F.,
 ( 6, 3, 6 ),
 ( 6, 6 ),
 ( 11.38875369420000006, 15.52868752870000080, 24.98742667679999840 ),
 ( 0.000000000000000000, 2.000000000000000000 ),
 .UNSPECIFIED. ) ;
#49876=CARTESIAN_POINT ( 'NONE',  ( 10.35181298299999852, 1478.133428305090092, 203.4857779180190107 ) ) ;
#49877=CARTESIAN_POINT ( 'NONE',  ( -16.67289555338749807, 1420.528706056600186, 203.2438192415110052 ) ) ;
#49879=CARTESIAN_POINT ( 'NONE',  ( -5.540266061381259988, 1433.565922541270083, 215.6367219123060011 ) ) ;
#49883=CARTESIAN_POINT ( 'NONE',  ( 4.325405441727872002, 1515.219201590508419, 210.9648081759952163 ) ) ;
#49887=CARTESIAN_POINT ( 'NONE',  ( 10.60756267625500016, 1423.066441122550032, 207.7293007016729973 ) ) ;
#49894=CARTESIAN_POINT ( 'NONE',  ( 2.125574643609999814, 1472.895346367389948, 219.1091941688290206 ) ) ;
#49896=CARTESIAN_POINT ( 'NONE',  ( 18.19723846073130247, 1429.891490729359930, 209.9056605128800186 ) ) ;
#49902=CARTESIAN_POINT ( 'NONE',  ( 7.374335209140000735, 1448.578211398790017, 202.8746320373990102 ) ) ;
#49911=CARTESIAN_POINT ( 'NONE',  ( -20.86254339170000094, 1504.682062816289999, 214.2159060785090219 ) ) ;
#49917=CARTESIAN_POINT ( 'NONE',  ( 12.24365554470000106, 1500.600794515889902, 208.6479362693279711 ) ) ;
#49928=CARTESIAN_POINT ( 'NONE',  ( -11.77904797301389905, 1483.168249568389911, 228.2502144964559818 ) ) ;
#49932=FACE_OUTER_BOUND ( 'NONE', #20515, .T. ) ;
#49935=CARTESIAN_POINT ( 'NONE',  ( -14.74403395979999942, 1507.703932417990245, 209.3705301297690085 ) ) ;
#49936=CARTESIAN_POINT ( 'NONE',  ( 4.325805487360000257, 1515.203924463989779, 210.5850643037490215 ) ) ;
#49941=DIRECTION ( 'NONE',  ( -1.224227143275518948E-16, 0.02617694830788859853, 0.9996573249755569268 ) ) ;
#49947=ORIENTED_EDGE ( 'NONE', *, *, #57059, .T. ) ;
#49951=VERTEX_POINT ( 'NONE', #25162 ) ;
#49955=CARTESIAN_POINT ( 'NONE',  ( -10.46614408832069998, 1462.592476666500033, 207.4320058997580247 ) ) ;
#49958=CARTESIAN_POINT ( 'NONE',  ( -10.18040284890000002, 1472.197773114690108, 205.9807533724089978 ) ) ;
#49963=CARTESIAN_POINT ( 'NONE',  ( 5.811772643825870333, 1467.189857448589919, 199.6405403245489936 ) ) ;
#49964=CARTESIAN_POINT ( 'NONE',  ( 19.96781675539999767, 1474.314029133290205, 212.0813829049089918 ) ) ;
#49972=CARTESIAN_POINT ( 'NONE',  ( 2.849563100782139813, 1515.551843419129909, 213.1048050505769993 ) ) ;
#49977=CARTESIAN_POINT ( 'NONE',  ( -0.3510182098590010069, 1508.319869606589918, 220.7744203783990145 ) ) ;
#49979=CARTESIAN_POINT ( 'NONE',  ( -0.7666883967970010705, 1430.262722078590059, 214.7518399592089793 ) ) ;
#49980=CARTESIAN_POINT ( 'NONE',  ( -6.384336360429650803, 1441.163446422609923, 202.7784055348689947 ) ) ;
#49982=CARTESIAN_POINT ( 'NONE',  ( 8.206329918199999796, 1502.256773578390039, 208.4091422247220180 ) ) ;
#49985=CARTESIAN_POINT ( 'NONE',  ( -10.39513868812339936, 1481.808198652379815, 206.4190733064540098 ) ) ;
#49993=EDGE_CURVE ( 'NONE', #7587, #107938, #21263, .T. ) ;
#49996=CARTESIAN_POINT ( 'NONE',  ( 1.663997124576299891, 1454.715882351969867, 218.3807490822640034 ) ) ;
#49999=CARTESIAN_POINT ( 'NONE',  ( -15.17668577640000116, 1418.088921015730193, 203.1694998214689747 ) ) ;
#50004=EDGE_CURVE ( 'NONE', #1876, #87891, #37690, .T. ) ;
#50005=CARTESIAN_POINT ( 'NONE',  ( -5.387811863060000483, 1496.648312753189884, 199.2595355468089906 ) ) ;
#50007=CARTESIAN_POINT ( 'NONE',  ( 0.7498365066470009666, 1478.145630918389998, 201.5100879341690074 ) ) ;
#50010=CARTESIAN_POINT ( 'NONE',  ( 10.47511427260239891, 1482.040461736080033, 210.7458695605469927 ) ) ;
#50022=LINE ( 'NONE', #25333, #25008 ) ;
#50028=CARTESIAN_POINT ( 'NONE',  ( 10.99410683563099767, 1478.963161965750032, 206.4867629818700152 ) ) ;
#50029=B_SPLINE_SURFACE_WITH_KNOTS ( 'NONE', 5, 1, ( 
 ( #102994, #87890 ),
 ( #19549, #1126 ),
 ( #94050, #34700 ),
 ( #70000, #26291 ),
 ( #27963, #96272 ),
 ( #94599, #59933 ) ),
 .UNSPECIFIED., .F., .F., .F.,
 ( 6, 6 ),
 ( 2, 2 ),
 ( 0.000000000000000000, 3.242714680140000194 ),
 ( 0.000000000000000000, 14.00000000000000000 ),
 .UNSPECIFIED. ) ;
#50031=CARTESIAN_POINT ( 'NONE',  ( -8.627774960320888198, 1437.492597821660183, 228.3379533698820012 ) ) ;
#50034=CARTESIAN_POINT ( 'NONE',  ( -9.299436816696520225, 1446.922293005960000, 190.6945112479180011 ) ) ;
#50035=CARTESIAN_POINT ( 'NONE',  ( -16.09548523901650086, 1416.444417915309941, 209.3983194699009971 ) ) ;
#50037=FACE_OUTER_BOUND ( 'NONE', #86715, .T. ) ;
#50040=FACE_OUTER_BOUND ( 'NONE', #4451, .T. ) ;
#50042=CARTESIAN_POINT ( 'NONE',  ( 7.718983249339360420, 1448.959774226909985, 202.2765896645470036 ) ) ;
#50053=ORIENTED_EDGE ( 'NONE', *, *, #33017, .F. ) ;
#50058=CARTESIAN_POINT ( 'NONE',  ( -4.602356253840000022, 1468.583955076089978, 189.7619545879989857 ) ) ;
#50062=CARTESIAN_POINT ( 'NONE',  ( 2.375134825399999539, 1444.621758423489837, 200.4616579052089946 ) ) ;
#50085=CARTESIAN_POINT ( 'NONE',  ( -12.14270316730000054, 1503.406043248689912, 208.4356947272389959 ) ) ;
#50090=ORIENTED_EDGE ( 'NONE', *, *, #4346, .F. ) ;
#50108=CARTESIAN_POINT ( 'NONE',  ( 2.594761893819999887, 1441.567844146989955, 218.7008844616090073 ) ) ;
#50112=PLANE ( 'NONE',  #17986 ) ;
#50115=ORIENTED_EDGE ( 'NONE', *, *, #41192, .F. ) ;
#50122=CARTESIAN_POINT ( 'NONE',  ( -2.948785487947506390, 1495.323990659472429, 219.9171465939708980 ) ) ;
#50128=CARTESIAN_POINT ( 'NONE',  ( -9.181507157277641440, 1449.803788077400213, 209.6493162511999913 ) ) ;
#50130=ORIENTED_EDGE ( 'NONE', *, *, #19897, .T. ) ;
#50138=CARTESIAN_POINT ( 'NONE',  ( -2.157536728407480009, 1378.013060387289897, 210.3005136483574518 ) ) ;
#50139=CARTESIAN_POINT ( 'NONE',  ( 4.378631935749999649, 1467.806944014989995, 218.0906305500190001 ) ) ;
#50153=EDGE_CURVE ( 'NONE', #27470, #60953, #76037, .T. ) ;
#50154=CARTESIAN_POINT ( 'NONE',  ( -765.6063658702573775, -8383.748406600814633, -1617.797774209815316 ) ) ;
#50161=CARTESIAN_POINT ( 'NONE',  ( -4.324121584285179232, 1515.222544093250008, 212.0786738497689896 ) ) ;
#50168=ORIENTED_EDGE ( 'NONE', *, *, #1619, .F. ) ;
#50172=VERTEX_POINT ( 'NONE', #36713 ) ;
#50173=VERTEX_POINT ( 'NONE', #88227 ) ;
#50175=CARTESIAN_POINT ( 'NONE',  ( 3.561219592449999638, 1455.895344195389953, 218.7021084924690228 ) ) ;
#50177=CARTESIAN_POINT ( 'NONE',  ( -1.194279839290000034, 1444.571198474990069, 218.0071126885590047 ) ) ;
#50182=CARTESIAN_POINT ( 'NONE',  ( 7.541206810410000294, 1424.198099201060131, 212.4425681308690059 ) ) ;
#50190=CARTESIAN_POINT ( 'NONE',  ( 4.987078435459999071, 1508.551704408389924, 209.1218459616989946 ) ) ;
#50202=CARTESIAN_POINT ( 'NONE',  ( 3.552713678799999608E-15, 1413.913060387330006, 209.1218459616989946 ) ) ;
#50205=CARTESIAN_POINT ( 'NONE',  ( -9.499875067660077832, 1448.112547453520165, 210.0994082806479923 ) ) ;
#50213=CARTESIAN_POINT ( 'NONE',  ( 6.664268339219599824, 1424.601171630709814, 193.8494905227429967 ) ) ;
#50215=DIRECTION ( 'NONE',  ( -1.156023075842281927E-31, 1.000000000000000000, -1.698192320643030073E-16 ) ) ;
#50226=CARTESIAN_POINT ( 'NONE',  ( -8.106555885276549134, 1438.741351455190170, 205.9368832915250209 ) ) ;
#50232=CARTESIAN_POINT ( 'NONE',  ( 10.92202464131200124, 1460.857965367780025, 208.4167310687169845 ) ) ;
#50233=EDGE_CURVE ( 'NONE', #18362, #44275, #66744, .T. ) ;
#50239=CARTESIAN_POINT ( 'NONE',  ( -2.064501014040000193, 1497.911843841890004, 200.8390656523289977 ) ) ;
#50246=CARTESIAN_POINT ( 'NONE',  ( -11.16643432470000086, 1471.372555798990106, 206.7508257807689915 ) ) ;
#50248=ORIENTED_EDGE ( 'NONE', *, *, #48772, .T. ) ;
#50249=DIRECTION ( 'NONE',  ( 0.000000000000000000, 1.000000000000000000, -1.836970198721029688E-16 ) ) ;
#50254=CARTESIAN_POINT ( 'NONE',  ( -9.608263814349999876, 1414.782003256130110, 207.8393504740089952 ) ) ;
#50257=CARTESIAN_POINT ( 'NONE',  ( 4.151488833330000183, 1485.695544300589972, 199.1893064789089749 ) ) ;
#50258=CARTESIAN_POINT ( 'NONE',  ( 3.791557891630739974, 1430.522366444419958, 217.8194754324450173 ) ) ;
#50266=CARTESIAN_POINT ( 'NONE',  ( -16.72115780329999879, 1420.505589990380031, 203.2363230761090165 ) ) ;
#50268=CARTESIAN_POINT ( 'NONE',  ( -1.281400930710000052, 1474.396637362589900, 219.3408303083989779 ) ) ;
#50271=CARTESIAN_POINT ( 'NONE',  ( -11.40295414052340028, 1470.727202249070160, 209.2846016133759974 ) ) ;
#50272=CARTESIAN_POINT ( 'NONE',  ( -4.849196095585594612, 1508.218303878354391, 220.4640527089468662 ) ) ;
#50278=CARTESIAN_POINT ( 'NONE',  ( -4.558402699344750175, 1421.324977942919986, 193.7899644519529829 ) ) ;
#50286=CARTESIAN_POINT ( 'NONE',  ( -5.243297302279999350, 1438.659032880589848, 207.2722467018089958 ) ) ;
#50292=EDGE_CURVE ( 'NONE', #53580, #3936, #100018, .T. ) ;
#50293=CARTESIAN_POINT ( 'NONE',  ( -3.736170183908800180, 1487.848895934140046, 219.5114665497349904 ) ) ;
#50294=CARTESIAN_POINT ( 'NONE',  ( -4.287909922120000772, 1515.369373403189911, 208.3886085559139758 ) ) ;
#50297=CARTESIAN_POINT ( 'NONE',  ( 10.21500163810000039, 1470.289493831289747, 209.7507578853689836 ) ) ;
#50298=CARTESIAN_POINT ( 'NONE',  ( 11.22342845537009914, 1492.268138787170074, 211.5860973086979868 ) ) ;
#50300=CARTESIAN_POINT ( 'NONE',  ( 1.217071433320000118, 1456.474392760389946, 219.2743944847990178 ) ) ;
#50312=CARTESIAN_POINT ( 'NONE',  ( -8.550067366969999583, 1462.070379093089969, 204.3084576837289887 ) ) ;
#50314=CARTESIAN_POINT ( 'NONE',  ( 2.237652899700000031, 1444.342138342490216, 203.2451014604889963 ) ) ;
#50320=CARTESIAN_POINT ( 'NONE',  ( 2.335054519268260353, 1486.771262222820042, 197.4158623816819897 ) ) ;
#50322=CARTESIAN_POINT ( 'NONE',  ( 3.373264501941120042, 1432.691143165750191, 201.1530439168859914 ) ) ;
#50326=ADVANCED_FACE ( 'NONE', ( #33975 ), #100261, .T. ) ;
#50327=CARTESIAN_POINT ( 'NONE',  ( -19.78154490129999843, 1468.390536983390120, 204.4459624408089837 ) ) ;
#50333=CARTESIAN_POINT ( 'NONE',  ( 9.146299198640271300, 1461.861878385089767, 205.8341600298289791 ) ) ;
#50335=CARTESIAN_POINT ( 'NONE',  ( 0.1511760582950009979, 1477.260385247390104, 198.7062178346990038 ) ) ;
#50342=CARTESIAN_POINT ( 'NONE',  ( -7.968780129149999780, 1425.481181651620091, 207.4285999761289929 ) ) ;
#50346=CARTESIAN_POINT ( 'NONE',  ( 7.263451787643480095, 1426.472202734280017, 212.8712549859859848 ) ) ;
#50354=CARTESIAN_POINT ( 'NONE',  ( -16.45840115875039800, 1508.541818857670023, 213.5626919147919978 ) ) ;
#50361=CARTESIAN_POINT ( 'NONE',  ( 8.090998277665431004, 1435.786064241179929, 206.2615718783590069 ) ) ;
#50383=CARTESIAN_POINT ( 'NONE',  ( 7.516769032520000060, 1422.170349638209927, 195.6959265412990021 ) ) ;
#50385=CARTESIAN_POINT ( 'NONE',  ( 11.05853588759599937, 1478.760309791250165, 205.9079366425139881 ) ) ;
#50388=CARTESIAN_POINT ( 'NONE',  ( 4.038582018629999659, 1515.598601288590089, 209.1218459616989946 ) ) ;
#50396=CARTESIAN_POINT ( 'NONE',  ( -10.71760456835239950, 1483.213272081000014, 203.9247400436699991 ) ) ;
#50398=CARTESIAN_POINT ( 'NONE',  ( 8.482184659042799169, 1423.325493229070162, 211.9867658860320034 ) ) ;
#50400=CARTESIAN_POINT ( 'NONE',  ( 11.52796152851120048, 1425.560458258250264, 202.9256552550970127 ) ) ;
#50401=CARTESIAN_POINT ( 'NONE',  ( -11.00543052331669891, 1462.571841119889996, 208.1677703206260048 ) ) ;
#50410=CARTESIAN_POINT ( 'NONE',  ( -17.51543113656909867, 1417.552258021759826, 206.7803033077899784 ) ) ;
#50411=CARTESIAN_POINT ( 'NONE',  ( 9.043577616344240511, 1419.744760940520109, 194.5516119844990044 ) ) ;
#50412=CARTESIAN_POINT ( 'NONE',  ( 6.494921822917000043, 1465.840553322820142, 216.8173835122059927 ) ) ;
#50417=CARTESIAN_POINT ( 'NONE',  ( -8.110034436179123674, 1425.494577458902768, 208.5273439571141409 ) ) ;
#50421=CARTESIAN_POINT ( 'NONE',  ( 12.71867950848070095, 1426.806024775080004, 204.8922107218619999 ) ) ;
#50423=B_SPLINE_CURVE_WITH_KNOTS ( 'NONE', 3,
 ( #37915, #12700, #77301, #1704, #1152, #98355, #69468, #599, #72096, #103019, #26315, #94630, #106211, #17905, #35844, #103586, #26888, #55282, #61078, #46884, #38445, #70029, #106751, #19007, #104142, #27427, #61610, #30039, #98901, #74283, #107856, #101091, #89954, #56369, #82102, #22718, #56919, #41211, #38989, #99441, #92160, #32796, #57484, #91050, #65878, #109520, #49625, #14336, #24390 ),
 .UNSPECIFIED., .F., .F.,
 ( 4, 3, 3, 3, 3, 3, 3, 3, 3, 3, 3, 3, 3, 3, 3, 3, 4 ),
 ( 0.000000000000000000, 1.367534301173350064, 2.791361796389739691, 4.169044824514560155, 5.615944553276730034, 7.062844282038899912, 8.459574530849598872, 9.876103170593360403, 11.24898385078170016, 12.61392778173159890, 13.96829556498239988, 14.12568908982460059, 14.94249011817409922, 15.71017679274670087, 16.35253358467650031, 16.91884759190949694, 17.37853207929999755 ),
 .UNSPECIFIED. ) ;
#50424=CARTESIAN_POINT ( 'NONE',  ( -17.63599094636219888, 1419.790072980149944, 206.1021312808440200 ) ) ;
#50431=DIRECTION ( 'NONE',  ( 0.000000000000000000, -1.000000000000000000, 0.000000000000000000 ) ) ;
#50438=CARTESIAN_POINT ( 'NONE',  ( 17.12499568933700189, 1499.118982824430077, 222.9618237066810025 ) ) ;
#50439=CARTESIAN_POINT ( 'NONE',  ( -8.200787980966151025, 1436.145857994200242, 211.9570384925519875 ) ) ;
#50447=CARTESIAN_POINT ( 'NONE',  ( 11.63682296995209953, 1421.992969092299973, 209.6317927274760109 ) ) ;
#50452=CARTESIAN_POINT ( 'NONE',  ( 2.227690093140000105, 1473.333206620189912, 219.1070348612290104 ) ) ;
#50456=CARTESIAN_POINT ( 'NONE',  ( -10.20231950299999824, 1492.893084484690235, 203.6441250547690061 ) ) ;
#50462=CARTESIAN_POINT ( 'NONE',  ( -21.57334207099999901, 1507.349712068389863, 210.4840098404890227 ) ) ;
#50464=CARTESIAN_POINT ( 'NONE',  ( -3.021161635200000362, 1455.772982809590076, 200.1537592901690061 ) ) ;
#50471=VERTEX_POINT ( 'NONE', #106155 ) ;
#50472=CARTESIAN_POINT ( 'NONE',  ( -17.53307272543440121, 1417.831573838860095, 206.8262974944190091 ) ) ;
#50473=ORIENTED_EDGE ( 'NONE', *, *, #3285, .F. ) ;
#50481=DIRECTION ( 'NONE',  ( 0.4436356471204865315, 1.250495761681361773E-32, 0.8962072375315807138 ) ) ;
#50484=CARTESIAN_POINT ( 'NONE',  ( 12.60056023386209922, 1500.993407397960027, 210.8144105449839856 ) ) ;
#50488=ORIENTED_EDGE ( 'NONE', *, *, #23300, .F. ) ;
#50491=ORIENTED_EDGE ( 'NONE', *, *, #7663, .F. ) ;
#50492=VERTEX_POINT ( 'NONE', #11548 ) ;
#50493=CARTESIAN_POINT ( 'NONE',  ( -1.413982343730000091, 1425.233086417520099, 191.1415897097990069 ) ) ;
#50496=CARTESIAN_POINT ( 'NONE',  ( -13.02765491641741846, 1417.056304985424049, 200.8910991843737008 ) ) ;
#50498=CARTESIAN_POINT ( 'NONE',  ( 4.287909922120000772, 1515.369373403189911, 209.8550833674839851 ) ) ;
#50499=CARTESIAN_POINT ( 'NONE',  ( -6.272372246000269769, 1454.211692497139893, 202.1362065909700050 ) ) ;
#50501=CARTESIAN_POINT ( 'NONE',  ( -19.71644462915288187, 1485.715905243316456, 215.2741460507342310 ) ) ;
#50514=CARTESIAN_POINT ( 'NONE',  ( -4.170038484254391165, 1432.161950885697252, 216.4833537471189402 ) ) ;
#50515=CARTESIAN_POINT ( 'NONE',  ( -10.57410958284499891, 1462.298602691789938, 208.7181287738039828 ) ) ;
#50517=CARTESIAN_POINT ( 'NONE',  ( 10.12605604320560104, 1469.432876218259935, 207.3487825585040127 ) ) ;
#50518=CARTESIAN_POINT ( 'NONE',  ( -9.237108298879999069, 1474.172111518589873, 204.4935998512690105 ) ) ;
#50522=CARTESIAN_POINT ( 'NONE',  ( -20.64498752849999974, 1505.794066315190094, 209.1536330714720009 ) ) ;
#50523=CARTESIAN_POINT ( 'NONE',  ( 8.543286749999769114, 1468.346214803730163, 201.8597651585060078 ) ) ;
#50524=DIRECTION ( 'NONE',  ( 0.1677289028140550031, 0.3720281548064550137, -0.9129414368907229349 ) ) ;
#50527=DIRECTION ( 'NONE',  ( 9.156846217086110244E-47, -1.000000000000000000, 1.836970198721029688E-16 ) ) ;
#50531=CARTESIAN_POINT ( 'NONE',  ( -1.766059939614330165, 1483.862676877220110, 198.5882530496979825 ) ) ;
#50532=CARTESIAN_POINT ( 'NONE',  ( -11.55143878132009938, 1501.163903211799834, 211.2289541138460152 ) ) ;
#50535=CARTESIAN_POINT ( 'NONE',  ( -0.4021349000140009844, 1508.551704408389924, 220.0610460832990043 ) ) ;
#50539=CARTESIAN_POINT ( 'NONE',  ( 4.760896992130000172, 1449.971761959190189, 190.6385172635989704 ) ) ;
#50540=CARTESIAN_POINT ( 'NONE',  ( 20.49831092009999978, 1496.178973653789853, 204.1013708937389879 ) ) ;
#50541=CARTESIAN_POINT ( 'NONE',  ( 1.113400974650000208, 1478.239378551490063, 201.5788049939389737 ) ) ;
#50543=CARTESIAN_POINT ( 'NONE',  ( -10.68990730692100044, 1481.192710571149973, 208.4620442137509997 ) ) ;
#50544=CARTESIAN_POINT ( 'NONE',  ( -8.929044350759999915, 1464.245425498190116, 227.2010804325990136 ) ) ;
#50555=CARTESIAN_POINT ( 'NONE',  ( -15.84994825389999740, 1416.551565560330118, 207.9043296938389744 ) ) ;
#50559=CARTESIAN_POINT ( 'NONE',  ( -16.63648012991517433, 1419.612236357899292, 209.0575818519019720 ) ) ;
#50560=CARTESIAN_POINT ( 'NONE',  ( -4.795131425830000182, 1497.578645253790000, 220.1696405719989968 ) ) ;
#50561=CARTESIAN_POINT ( 'NONE',  ( 0.1832230673610020233, 1471.246529402990063, 189.0482111049990124 ) ) ;
#50562=CARTESIAN_POINT ( 'NONE',  ( -18.39258007780000170, 1441.405133176690015, 212.6808529323389791 ) ) ;
#50563=CARTESIAN_POINT ( 'NONE',  ( -11.65979349303169954, 1507.853111589269929, 207.9005118103889913 ) ) ;
#50564=CARTESIAN_POINT ( 'NONE',  ( -4.882950377119058771, 1421.798896365259225, 193.0164691839993907 ) ) ;
#50577=CARTESIAN_POINT ( 'NONE',  ( 4.722118042039999963, 1485.526134326590181, 218.7852782599590000 ) ) ;
#50578=CARTESIAN_POINT ( 'NONE',  ( 10.17866008307600012, 1479.588344398260006, 206.0280708825729903 ) ) ;
#50579=CARTESIAN_POINT ( 'NONE',  ( -18.31485190103290250, 1445.278724020879963, 204.5307765124340165 ) ) ;
#50580=CARTESIAN_POINT ( 'NONE',  ( -19.31924249874780131, 1445.911422301539915, 199.9640984727790283 ) ) ;
#50582=CARTESIAN_POINT ( 'NONE',  ( -16.76045707751869784, 1417.322363310820037, 208.1402530697109796 ) ) ;
#50589=CARTESIAN_POINT ( 'NONE',  ( -11.73357813035489983, 1488.009932409569956, 191.9067504558449855 ) ) ;
#50602=CARTESIAN_POINT ( 'NONE',  ( -10.34253148339749906, 1448.363770563499884, 208.2854772084710078 ) ) ;
#50603=CARTESIAN_POINT ( 'NONE',  ( 4.324121584285009590, 1515.222544093250008, 206.1650180736299944 ) ) ;
#50608=CARTESIAN_POINT ( 'NONE',  ( 1.047166550769999871, 1468.609441862589847, 219.1136373509289967 ) ) ;
#50609=CARTESIAN_POINT ( 'NONE',  ( -0.3062940834119980416, 1423.431708106900032, 191.1679817776989694 ) ) ;
#50610=SURFACE_STYLE_USAGE ( .BOTH. , #59022 ) ;
#50621=CARTESIAN_POINT ( 'NONE',  ( -8.690454074780983973, 1474.493355088299722, 203.6172070775714928 ) ) ;
#50624=CARTESIAN_POINT ( 'NONE',  ( 11.19148775935109974, 1422.145533233709784, 210.4506149377330075 ) ) ;
#50636=ADVANCED_FACE ( 'NONE', ( #52459 ), #79399, .T. ) ;
#50641=CARTESIAN_POINT ( 'NONE',  ( 17.78284146230000218, 1432.724246433989947, 213.5810953123289835 ) ) ;
#50645=CARTESIAN_POINT ( 'NONE',  ( -1.541850711665649963E-13, 1515.064792882589927, 213.4512947377390049 ) ) ;
#50647=CARTESIAN_POINT ( 'NONE',  ( -3.215255062656879659, 1428.800608840759878, 200.3254522118909904 ) ) ;
#50651=CARTESIAN_POINT ( 'NONE',  ( 9.574980784980720472, 1434.721929005479979, 207.0935444517720043 ) ) ;
#50671=CARTESIAN_POINT ( 'NONE',  ( -7.515458858486791627, 1461.908370352513202, 202.9557135729516517 ) ) ;
#50677=CARTESIAN_POINT ( 'NONE',  ( -2.670661672390000074, 1430.456431923590117, 201.2104187199990122 ) ) ;
#50678=ADVANCED_FACE ( 'NONE', ( #6995 ), #35540, .T. ) ;
#50683=CARTESIAN_POINT ( 'NONE',  ( 9.717824533310780666, 1463.678478211699939, 210.3770741684630252 ) ) ;
#50689=CARTESIAN_POINT ( 'NONE',  ( 11.47508409600000157, 1501.971768102289843, 208.9761436802440073 ) ) ;
#50691=CARTESIAN_POINT ( 'NONE',  ( 8.191473432960000522, 1428.034249043490036, 212.8209790924290132 ) ) ;
#50692=CARTESIAN_POINT ( 'NONE',  ( -4.259777698987590178, 1515.374151778960140, 212.0586637247320141 ) ) ;
#50695=CARTESIAN_POINT ( 'NONE',  ( -5.345845988899998957, 1483.903125241190082, 199.7205319149290119 ) ) ;
#50699=ORIENTED_EDGE ( 'NONE', *, *, #88465, .F. ) ;
#50704=FACE_OUTER_BOUND ( 'NONE', #57493, .T. ) ;
#50708=CARTESIAN_POINT ( 'NONE',  ( -1.693092261709999935, 1443.235800066189995, 218.9922124666489935 ) ) ;
#50715=CARTESIAN_POINT ( 'NONE',  ( -3.644092503733519894, 1454.098320749749973, 199.2979021310670191 ) ) ;
#50722=CARTESIAN_POINT ( 'NONE',  ( -2.188078410709979771, 1508.020976590390092, 220.9453026643990086 ) ) ;
#50728=CARTESIAN_POINT ( 'NONE',  ( 2.096969080950850106, 1476.217590029780013, 197.8222115087120017 ) ) ;
#50731=CARTESIAN_POINT ( 'NONE',  ( -10.04889086637309958, 1447.057712588790082, 211.5131067902999860 ) ) ;
#50735=CARTESIAN_POINT ( 'NONE',  ( -4.328283507529860685, 1515.109292691759947, 210.1175503365320196 ) ) ;
#50740=CARTESIAN_POINT ( 'NONE',  ( 9.475492894836309077, 1425.388351994820141, 195.3726508077949688 ) ) ;
#50747=EDGE_CURVE ( 'NONE', #60042, #23187, #26551, .T. ) ;
#50748=EDGE_CURVE ( 'NONE', #78107, #97433, #85476, .T. ) ;
#50758=ORIENTED_EDGE ( 'NONE', *, *, #83572, .F. ) ;
#50763=EDGE_CURVE ( 'NONE', #80101, #23359, #62528, .T. ) ;
#50764=CARTESIAN_POINT ( 'NONE',  ( 10.73980232230699983, 1460.418891470940025, 207.1303042227569904 ) ) ;
#50769=CARTESIAN_POINT ( 'NONE',  ( -18.53032035940000100, 1445.072917693090176, 205.4274489127490142 ) ) ;
#50780=B_SPLINE_SURFACE_WITH_KNOTS ( 'NONE', 5, 1, ( 
 ( #105065, #51341 ),
 ( #85475, #8774 ),
 ( #77116, #9349 ),
 ( #34540, #97756 ),
 ( #80420, #13176 ),
 ( #55231, #3733 ) ),
 .UNSPECIFIED., .F., .F., .F.,
 ( 6, 6 ),
 ( 2, 2 ),
 ( -2.070056070795430156E-05, 17.51321923676070114 ),
 ( 0.000000000000000000, 14.00002070056070025 ),
 .UNSPECIFIED. ) ;
#50783=CARTESIAN_POINT ( 'NONE',  ( -12.32280451139999933, 1415.506406008910062, 208.1838605997770060 ) ) ;
#50785=CARTESIAN_POINT ( 'NONE',  ( 5.547280765580000050, 1487.873461314389942, 198.4571336758990014 ) ) ;
#50790=CARTESIAN_POINT ( 'NONE',  ( -7.777329619812174855, 1449.162765272808201, 191.3840481915840144 ) ) ;
#50796=CARTESIAN_POINT ( 'NONE',  ( -17.01683863309999722, 1420.343045529830079, 203.4497032551290090 ) ) ;
#50800=B_SPLINE_CURVE_WITH_KNOTS ( 'NONE', 5,
 ( #55446, #11240, #89573, #79003, #29124, #30209, #70609, #28575, #2306 ),
 .UNSPECIFIED., .F., .F.,
 ( 6, 3, 6 ),
 ( -14.37983903770000005, -7.189919518870000026, -1.776356839400250465E-15 ),
 .UNSPECIFIED. ) ;
#50803=CARTESIAN_POINT ( 'NONE',  ( -11.16643434163729864, 1471.372555858320084, 206.7508257846899937 ) ) ;
#50804=CARTESIAN_POINT ( 'NONE',  ( -4.309330992969162999, 1508.176589348497373, 220.5992834243717766 ) ) ;
#50807=CARTESIAN_POINT ( 'NONE',  ( 9.146295267174979315, 1461.861888617270097, 205.8341477717290218 ) ) ;
#50810=CARTESIAN_POINT ( 'NONE',  ( -13.79952627106220042, 1418.844960651139900, 200.3911282168379842 ) ) ;
#50814=ORIENTED_EDGE ( 'NONE', *, *, #75300, .T. ) ;
#50815=CARTESIAN_POINT ( 'NONE',  ( -12.48995958582669985, 1501.883328869510024, 211.6213070116990025 ) ) ;
#50820=B_SPLINE_SURFACE_WITH_KNOTS ( 'NONE', 5, 1, ( 
 ( #45132, #42475 ),
 ( #50890, #110228 ),
 ( #104457, #79274 ),
 ( #85020, #61943 ),
 ( #19330, #16152 ),
 ( #8314, #93423 ),
 ( #33502, #67703 ),
 ( #25105, #76632 ),
 ( #25659, #70900 ) ),
 .UNSPECIFIED., .F., .F., .F.,
 ( 6, 3, 6 ),
 ( 2, 2 ),
 ( 0.000000000000000000, 7.208900216690000029, 14.43479085090000069 ),
 ( 0.000000000000000000, 14.00000000000000000 ),
 .UNSPECIFIED. ) ;
#50821=CARTESIAN_POINT ( 'NONE',  ( 9.379603162543640238, 1422.628403586280001, 212.8485163645989928 ) ) ;
#50823=CARTESIAN_POINT ( 'NONE',  ( -4.635897072777390271, 1377.991090176196622, 203.9911396117953188 ) ) ;
#50824=CARTESIAN_POINT ( 'NONE',  ( 10.75633390746000018, 1451.138030594549946, 190.3409186702180023 ) ) ;
#50827=EDGE_CURVE ( 'NONE', #8084, #29796, #8506, .T. ) ;
#50828=CARTESIAN_POINT ( 'NONE',  ( -5.219699508016872436, 1391.908825959211299, 214.5074746467423950 ) ) ;
#50830=CARTESIAN_POINT ( 'NONE',  ( -1.107012941800000094, 1455.995237770089943, 218.5495680003989776 ) ) ;
#50834=CARTESIAN_POINT ( 'NONE',  ( 4.865329319716050094, 1508.551704408389924, 205.8589166638820132 ) ) ;
#50843=CARTESIAN_POINT ( 'NONE',  ( -7.773290426329999114, 1463.683257113590116, 201.8013873513490068 ) ) ;
#50845=ADVANCED_FACE ( 'NONE', ( #7418 ), #71402, .T. ) ;
#50848=CARTESIAN_POINT ( 'NONE',  ( -11.08276793864819965, 1508.551704408389924, 217.7591383316709823 ) ) ;
#50851=CARTESIAN_POINT ( 'NONE',  ( -1.772523594583782724, 1468.998700552058153, 218.9957837055941638 ) ) ;
#50857=CARTESIAN_POINT ( 'NONE',  ( 11.14734945969999913, 1480.282866945889964, 229.7914729789989963 ) ) ;
#50861=CARTESIAN_POINT ( 'NONE',  ( -14.20118038929999926, 1469.193620957790017, 194.7233937116990035 ) ) ;
#50865=CARTESIAN_POINT ( 'NONE',  ( -12.38301933081382877, 1507.638490212013721, 208.9814132965477427 ) ) ;
#50867=CARTESIAN_POINT ( 'NONE',  ( -2.199814249270000133, 1475.434091217589867, 198.2859427615989887 ) ) ;
#50874=CARTESIAN_POINT ( 'NONE',  ( -8.089559954360000305, 1425.642170091349954, 208.1666042629669846 ) ) ;
#50875=ORIENTED_EDGE ( 'NONE', *, *, #90513, .F. ) ;
#50878=CARTESIAN_POINT ( 'NONE',  ( -8.938145041388430911, 1471.651254853389446, 214.0140567895946901 ) ) ;
#50879=CARTESIAN_POINT ( 'NONE',  ( 7.311343960930040353, 1426.407259653950177, 212.7706406922160056 ) ) ;
#50881=ORIENTED_EDGE ( 'NONE', *, *, #11868, .T. ) ;
#50883=CARTESIAN_POINT ( 'NONE',  ( -10.93326214739339974, 1492.840634310439782, 207.3500978010279994 ) ) ;
#50885=EDGE_CURVE ( 'NONE', #76758, #28705, #17233, .T. ) ;
#50888=B_SPLINE_CURVE_WITH_KNOTS ( 'NONE', 3,
 ( #71195, #30243, #62810, #3982, #50385, #5612, #15624, #100219, #25139, #23499, #67184, #40857, #91806, #73925, #83960, #108054, #49830, #32996, #57137, #66092, #75033, #76121, #48732, #91265, #101285, #24580, #84513, #7260, #41423, #48176, #92352, #57691, #109184, #99641 ),
 .UNSPECIFIED., .F., .F.,
 ( 4, 3, 3, 3, 3, 3, 3, 3, 3, 3, 3, 4 ),
 ( -2.000000000000000000, -1.859445973531549834, -1.676484109249690047, -1.491267025722599948, -1.304875122534860044, -1.117035657520179859, -0.9287884496328548956, -0.7405969126087090793, -0.5529186171893840651, -0.3669390813415169816, -0.1825462010525040757, 0.000000000000000000 ),
 .UNSPECIFIED. ) ;
#50890=CARTESIAN_POINT ( 'NONE',  ( 4.975825873569999835, 1424.099705961009931, 208.5330668394979909 ) ) ;
#50897=CARTESIAN_POINT ( 'NONE',  ( 8.980818830724000890, 1434.681779501059964, 206.5340080207419931 ) ) ;
#50899=ORIENTED_EDGE ( 'NONE', *, *, #10863, .F. ) ;
#50915=CARTESIAN_POINT ( 'NONE',  ( 8.036006549726169013, 1434.089066884029990, 225.8500050052630002 ) ) ;
#50917=CARTESIAN_POINT ( 'NONE',  ( 4.987078446123650366, 1508.551704408389924, 206.6339246584809928 ) ) ;
#50919=CARTESIAN_POINT ( 'NONE',  ( -4.913312227335970839, 1508.551704408389924, 212.2183601949549825 ) ) ;
#50921=CARTESIAN_POINT ( 'NONE',  ( 7.439417113980000273, 1422.547532122410075, 195.6475770543989938 ) ) ;
#50923=CARTESIAN_POINT ( 'NONE',  ( -2.787430966700440216, 1433.043516581739823, 218.2512527028169984 ) ) ;
#50925=CARTESIAN_POINT ( 'NONE',  ( -4.075622605530000442, 1495.353897722689908, 197.4859375650989932 ) ) ;
#50941=B_SPLINE_SURFACE_WITH_KNOTS ( 'NONE', 5, 1, ( 
 ( #110172, #68207 ),
 ( #9372, #95032 ),
 ( #26712, #17175 ),
 ( #42981, #35119 ),
 ( #77140, #16627 ),
 ( #60906, #102310 ),
 ( #42414, #69301 ),
 ( #1537, #43535 ),
 ( #77680, #26149 ),
 ( #60338, #93362 ),
 ( #35671, #992 ),
 ( #103977, #51366 ),
 ( #84954, #68751 ),
 ( #102854, #27272 ),
 ( #61456, #95582 ),
 ( #18850, #53047 ),
 ( #50824, #33444 ),
 ( #8246, #67644 ),
 ( #101753, #3761 ),
 ( #62012, #96132 ),
 ( #19410, #45761 ),
 ( #12681, #55260 ),
 ( #89392, #37895 ),
 ( #104535, #105658 ),
 ( #80448, #46319 ),
 ( #37340, #106191 ),
 ( #70415, #27831 ),
 ( #72077, #11585 ),
 ( #20505, #97233 ),
 ( #46861, #38424 ),
 ( #53612, #71537 ),
 ( #2656, #11036 ),
 ( #79344, #63665 ),
 ( #28943, #29473 ),
 ( #97779, #105091 ),
 ( #72599, #12126 ),
 ( #54714, #45203 ),
 ( #55814, #62583 ),
 ( #106728, #30018 ),
 ( #88841, #89931 ),
 ( #21055, #21609 ),
 ( #13208, #80991 ),
 ( #19971, #4297 ),
 ( #64209, #87754 ),
 ( #98332, #78788 ),
 ( #2102, #63132 ),
 ( #36230, #36783 ),
 ( #70976, #28381 ),
 ( #96700, #54165 ),
 ( #88290, #79898 ),
 ( #3211, #22700 ) ),
 .UNSPECIFIED., .F., .F., .F.,
 ( 6, 3, 3, 3, 3, 3, 3, 3, 3, 3, 3, 3, 3, 3, 3, 3, 6 ),
 ( 2, 2 ),
 ( 0.000000000000000000, 28.69702819429999963, 61.04778752440000034, 93.62768910810000023, 123.7336603250000024, 156.1762685979999787, 187.3272846180000215, 220.4669312460000015, 237.3878297990000021, 254.2938300590000154, 289.2398204710000300, 325.3030936050000150, 360.8626869010000178, 395.8828220460000011, 432.6128460950000090, 468.8934854820000169, 502.1482307969999965 ),
 ( -8.108887887879349314E-05, 2.001700839520000219 ),
 .UNSPECIFIED. ) ;
#50944=CARTESIAN_POINT ( 'NONE',  ( 1.632599499710808422, 1421.481676329297898, 193.8011752862853712 ) ) ;
#50951=CARTESIAN_POINT ( 'NONE',  ( -11.04008170774799957, 1462.385341758290224, 208.9869242049449838 ) ) ;
#50952=CARTESIAN_POINT ( 'NONE',  ( -16.95945306273139863, 1420.347400483130059, 203.7374467786609955 ) ) ;
#50953=CARTESIAN_POINT ( 'NONE',  ( 12.67647370521179973, 1426.478948021449924, 202.7078733498550207 ) ) ;
#50959=CARTESIAN_POINT ( 'NONE',  ( -0.7008159675984454440, 1477.501393641809045, 198.7433666631080769 ) ) ;
#50961=CARTESIAN_POINT ( 'NONE',  ( 3.353036578218081321, 1508.146033441647660, 220.1520117934527150 ) ) ;
#50963=CARTESIAN_POINT ( 'NONE',  ( -4.354856832958300394, 1481.954697149059939, 231.1149924593809999 ) ) ;
#50965=CARTESIAN_POINT ( 'NONE',  ( -14.57368822342009906, 1420.954711568789889, 207.9848542621210186 ) ) ;
#50974=ORIENTED_EDGE ( 'NONE', *, *, #76076, .T. ) ;
#50981=CARTESIAN_POINT ( 'NONE',  ( -4.782325726783580144, 1433.817978782009959, 216.6757878527850210 ) ) ;
#50983=CARTESIAN_POINT ( 'NONE',  ( -15.64027221210000107, 1419.286982173109891, 210.8948112567390183 ) ) ;
#50988=CARTESIAN_POINT ( 'NONE',  ( 10.78765558695330107, 1422.957222186570107, 207.1808645241220290 ) ) ;
#50994=CARTESIAN_POINT ( 'NONE',  ( 1.742415919699999982, 1474.343050966390138, 219.6228429884990305 ) ) ;
#50997=CARTESIAN_POINT ( 'NONE',  ( -7.648516765129999229, 1495.666136353089996, 200.8684719025990262 ) ) ;
#51002=CARTESIAN_POINT ( 'NONE',  ( 8.347715551000000289, 1448.434209623990000, 205.2198596814789937 ) ) ;
#51005=CARTESIAN_POINT ( 'NONE',  ( -3.201474586160000246, 1454.788669850390079, 199.8827619061390237 ) ) ;
#51009=CARTESIAN_POINT ( 'NONE',  ( -1.966612674429999652, 1496.552542902290043, 197.6618318493989932 ) ) ;
#51010=FACE_OUTER_BOUND ( 'NONE', #40717, .T. ) ;
#51024=ADVANCED_FACE ( 'NONE', ( #692 ), #1980, .F. ) ;
#51025=CARTESIAN_POINT ( 'NONE',  ( 4.174962612117290028, 1508.551704408389924, 213.4548848115649946 ) ) ;
#51029=CARTESIAN_POINT ( 'NONE',  ( 9.778911541403340735, 1461.615419081409982, 207.8750183380009844 ) ) ;
#51039=CARTESIAN_POINT ( 'NONE',  ( -10.84387077669929589, 1417.968182827059536, 198.1845410755198600 ) ) ;
#51040=CARTESIAN_POINT ( 'NONE',  ( 2.330134122034449806, 1515.551704408389924, 205.2922258479440245 ) ) ;
#51041=CARTESIAN_POINT ( 'NONE',  ( -6.092591263813240232, 1454.342283619849923, 201.9713694523269965 ) ) ;
#51042=ADVANCED_FACE ( 'NONE', ( #1805 ), #105717, .F. ) ;
#51045=AXIS2_PLACEMENT_3D ( 'NONE', #43526, #95021, #94443 ) ;
#51048=VERTEX_POINT ( 'NONE', #35377 ) ;
#51054=B_SPLINE_CURVE_WITH_KNOTS ( 'NONE', 3,
 ( #1544, #44093, #9922, #51939, #85508, #52499, #77146, #86083, #53617, #93914, #61461, #9377, #8805, #53052, #18856, #77685, #60911, #78231, #87190, #450, #70422, #42987, #68756, #998, #95039, #25602, #59794, #2109 ),
 .UNSPECIFIED., .F., .F.,
 ( 4, 3, 3, 3, 3, 3, 3, 3, 3, 4 ),
 ( -7.293785117949999730, -7.169388331878350229, -6.566796097046200487, -5.839807076142389697, -5.147073161146510145, -4.739076892086050208, -4.240156153919569348, -3.759358294541570000, -3.363905596364519912, -3.000356897310000548 ),
 .UNSPECIFIED. ) ;
#51058=CARTESIAN_POINT ( 'NONE',  ( 5.009886284249999377, 1430.069699660889910, 217.1776678749689893 ) ) ;
#51059=CARTESIAN_POINT ( 'NONE',  ( -18.74729292449999818, 1442.199705176290081, 209.1218459616989946 ) ) ;
#51061=CARTESIAN_POINT ( 'NONE',  ( -3.701332510601603953, 1488.791807424273657, 219.3688952161021746 ) ) ;
#51068=CARTESIAN_POINT ( 'NONE',  ( -3.644795242719999884, 1497.323677685689972, 198.4600586451990125 ) ) ;
#51069=CARTESIAN_POINT ( 'NONE',  ( 8.358086347145718520, 1468.256939908329969, 201.6625126024160295 ) ) ;
#51071=B_SPLINE_SURFACE_WITH_KNOTS ( 'NONE', 5, 1, ( 
 ( #4077, #103764 ),
 ( #44423, #27066 ),
 ( #61251, #45542 ),
 ( #44984, #78565 ),
 ( #1881, #62917 ),
 ( #53379, #28153 ) ),
 .UNSPECIFIED., .F., .F., .F.,
 ( 6, 6 ),
 ( 2, 2 ),
 ( -1.032047596522180116E-05, 16.54785843137600310 ),
 ( 0.000000000000000000, 14.00001032047599914 ),
 .UNSPECIFIED. ) ;
#51074=CARTESIAN_POINT ( 'NONE',  ( -7.910413875049510324, 1499.455618961650089, 212.0002310091700224 ) ) ;
#51080=CARTESIAN_POINT ( 'NONE',  ( -14.30113686340000179, 1415.739699861750069, 214.3509892272290074 ) ) ;
#51090=CARTESIAN_POINT ( 'NONE',  ( 21.13068363900000080, 1496.786787671390130, 208.1084808827089887 ) ) ;
#51093=CARTESIAN_POINT ( 'NONE',  ( -9.366078551730000257, 1478.880934751289942, 214.2941079828090096 ) ) ;
#51102=CARTESIAN_POINT ( 'NONE',  ( 1.439473459159019919, 1454.776503338229986, 218.4216800315260230 ) ) ;
#51105=CARTESIAN_POINT ( 'NONE',  ( -14.50510915870000161, 1416.687742578199959, 203.9073860009089856 ) ) ;
#51107=CARTESIAN_POINT ( 'NONE',  ( -4.159019969402780070, 1485.181217399250045, 197.9706610134819869 ) ) ;
#51108=B_SPLINE_SURFACE_WITH_KNOTS ( 'NONE', 5, 1, ( 
 ( #29110, #36947 ),
 ( #71145, #63296 ),
 ( #21776, #81157 ),
 ( #29652, #88471 ),
 ( #30195, #79525 ),
 ( #98508, #63839 ),
 ( #97951, #54881 ),
 ( #3935, #11755 ),
 ( #80061, #96875 ) ),
 .UNSPECIFIED., .F., .F., .F.,
 ( 6, 3, 6 ),
 ( 2, 2 ),
 ( -3.570158630500980045E-05, 8.847362025080000691, 17.72538832238630135 ),
 ( 0.000000000000000000, 14.00003570158630062 ),
 .UNSPECIFIED. ) ;
#51109=CARTESIAN_POINT ( 'NONE',  ( -16.09212348995429664, 1419.771771290114657, 210.1905430961424486 ) ) ;
#51110=CARTESIAN_POINT ( 'NONE',  ( -9.930122423809999432, 1499.782504084789934, 217.2571562510489969 ) ) ;
#51114=CARTESIAN_POINT ( 'NONE',  ( 10.56762249884929972, 1481.680206704629882, 209.7477003755120109 ) ) ;
#51124=CARTESIAN_POINT ( 'NONE',  ( -15.46337563405010052, 1415.677402202039957, 209.5778891453549875 ) ) ;
#51128=CARTESIAN_POINT ( 'NONE',  ( 4.957343604469999221, 1484.564563689889837, 219.0507238675290012 ) ) ;
#51129=CARTESIAN_POINT ( 'NONE',  ( 3.855903970259999980, 1423.712488786839913, 193.3614856424989910 ) ) ;
#51131=CARTESIAN_POINT ( 'NONE',  ( -19.86496342331569664, 1441.826159015929989, 212.7408786141659789 ) ) ;
#51134=CARTESIAN_POINT ( 'NONE',  ( -18.92738905877370215, 1503.346139544750031, 222.1981867165029882 ) ) ;
#51135=CARTESIAN_POINT ( 'NONE',  ( -16.60706435110729728, 1417.159713941199925, 208.4134677303929948 ) ) ;
#51139=CARTESIAN_POINT ( 'NONE',  ( -19.15298488520000220, 1464.559837765089924, 213.8319524061190009 ) ) ;
#51140=CARTESIAN_POINT ( 'NONE',  ( 4.850088428599620194, 1447.195166418000099, 200.1568079554039912 ) ) ;
#51146=CARTESIAN_POINT ( 'NONE',  ( 10.51435689538379847, 1503.261304779379998, 214.3454426394149834 ) ) ;
#51154=CARTESIAN_POINT ( 'NONE',  ( -10.25711658408749827, 1448.721523702089826, 207.5095412171060332 ) ) ;
#51155=CARTESIAN_POINT ( 'NONE',  ( 2.936816566051839938, 1515.374151772610048, 204.8620682733370018 ) ) ;
#51156=CARTESIAN_POINT ( 'NONE',  ( -0.9161538208349989665, 1443.103178644890022, 200.2678594588790020 ) ) ;
#51160=CARTESIAN_POINT ( 'NONE',  ( 0.8760155196429990632, 1467.778340247989945, 219.4697915747989896 ) ) ;
#51165=CARTESIAN_POINT ( 'NONE',  ( 5.277460848200000498, 1426.742654866309977, 191.8370381630989812 ) ) ;
#51190=CARTESIAN_POINT ( 'NONE',  ( -16.61699100185279931, 1508.551704408389924, 210.3875922597520116 ) ) ;
#51191=CARTESIAN_POINT ( 'NONE',  ( -4.038582018629999659, 1515.598601288590089, 209.1218459616989946 ) ) ;
#51195=CARTESIAN_POINT ( 'NONE',  ( -3.162210773369679817, 1428.830388020579903, 200.3057258517670220 ) ) ;
#51200=CARTESIAN_POINT ( 'NONE',  ( -11.72713760778269965, 1482.434255557160213, 207.0899337349270013 ) ) ;
#51204=ORIENTED_EDGE ( 'NONE', *, *, #23577, .F. ) ;
#51207=CARTESIAN_POINT ( 'NONE',  ( 10.85948193710989962, 1490.658306709410226, 210.7204932393690058 ) ) ;
#51210=CARTESIAN_POINT ( 'NONE',  ( 10.86975233959999976, 1425.686310118649772, 206.4629375099989943 ) ) ;
#51218=CARTESIAN_POINT ( 'NONE',  ( -11.57853339036000051, 1508.440951728300206, 218.0096696868039885 ) ) ;
#51222=CARTESIAN_POINT ( 'NONE',  ( 4.025649270539999769, 1466.171376325889923, 219.4115622680990043 ) ) ;
#51223=CARTESIAN_POINT ( 'NONE',  ( -0.3665735836847974771, 1469.467114346855169, 219.1664881883607165 ) ) ;
#51229=CARTESIAN_POINT ( 'NONE',  ( 11.75435543447689923, 1479.754058704430008, 210.0662386466290172 ) ) ;
#51241=CARTESIAN_POINT ( 'NONE',  ( 9.217029512000001645, 1427.824332272489983, 211.8044453694090237 ) ) ;
#51242=CARTESIAN_POINT ( 'NONE',  ( -2.956826570601670312, 1515.222544082249897, 213.4459675328979813 ) ) ;
#51254=CARTESIAN_POINT ( 'NONE',  ( -11.48424209289999887, 1501.246870413989882, 210.7154051127189973 ) ) ;
#51255=CARTESIAN_POINT ( 'NONE',  ( -15.30458060377867646, 1416.034819603857841, 206.6266340747784227 ) ) ;
#51257=CARTESIAN_POINT ( 'NONE',  ( -9.966727850805121136, 1439.480327375449860, 208.4309914983489875 ) ) ;
#51262=CARTESIAN_POINT ( 'NONE',  ( 7.004917722090000076, 1424.454089082370047, 213.1672744739490213 ) ) ;
#51263=CARTESIAN_POINT ( 'NONE',  ( -18.29179384260000063, 1466.060301038189891, 217.7541513960790098 ) ) ;
#51269=CARTESIAN_POINT ( 'NONE',  ( 19.32263322520000060, 1455.378559704889767, 209.1218459616989946 ) ) ;
#51281=CARTESIAN_POINT ( 'NONE',  ( -9.735300322427688613, 1447.426970202749999, 210.9824412164790317 ) ) ;
#51284=EDGE_LOOP ( 'NONE', ( #88743, #93353, #92131, #107090 ) ) ;
#51287=ORIENTED_EDGE ( 'NONE', *, *, #35739, .F. ) ;
#51290=CARTESIAN_POINT ( 'NONE',  ( 6.435621394989889943, 1424.539923079149958, 193.7524916796629952 ) ) ;
#51295=CARTESIAN_POINT ( 'NONE',  ( -8.881784197000000993E-16, 1391.913060387289988, 209.1218459616989946 ) ) ;
#51303=VERTEX_POINT ( 'NONE', #69566 ) ;
#51313=CARTESIAN_POINT ( 'NONE',  ( 8.594280337688530835, 1437.591337424159974, 210.1983079730889870 ) ) ;
#51320=ORIENTED_EDGE ( 'NONE', *, *, #40299, .T. ) ;
#51322=CARTESIAN_POINT ( 'NONE',  ( -10.60846321666980074, 1492.499096768809977, 202.9143931177430034 ) ) ;
#51339=CARTESIAN_POINT ( 'NONE',  ( -16.64876402000000155, 1420.540327547920015, 203.2475213236290017 ) ) ;
#51340=ORIENTED_EDGE ( 'NONE', *, *, #45919, .F. ) ;
#51341=CARTESIAN_POINT ( 'NONE',  ( 20.41260875014629761, 1494.156740513740033, 204.1224910194729887 ) ) ;
#51342=( BOUNDED_CURVE ( )  B_SPLINE_CURVE ( 3, ( #1532, #25593, #34563, #43532 ),
 .UNSPECIFIED., .F., .F. ) 
 B_SPLINE_CURVE_WITH_KNOTS ( ( 4, 4 ),
 ( 0.9863028871718200197, 2.155290151626870099 ),
 .UNSPECIFIED. ) 
 CURVE ( )  GEOMETRIC_REPRESENTATION_ITEM ( )  RATIONAL_B_SPLINE_CURVE ( ( 1.000000000000000000, 0.8893277299739500430, 0.8893277299739500430, 1.000000000000000000 ) ) 
 REPRESENTATION_ITEM ( '' )  );
#51343=CARTESIAN_POINT ( 'NONE',  ( -12.96940454689999989, 1511.061367290189992, 209.8579693186340194 ) ) ;
#51346=CARTESIAN_POINT ( 'NONE',  ( 0.3061100630284139812, 1423.569528417510128, 191.1866024191019733 ) ) ;
#51347=CARTESIAN_POINT ( 'NONE',  ( -11.34294724864570014, 1471.070521140359915, 207.8607066046959915 ) ) ;
#51348=CARTESIAN_POINT ( 'NONE',  ( -6.379498533362892410, 1508.334156579840510, 219.9884138064801959 ) ) ;
#51351=CARTESIAN_POINT ( 'NONE',  ( 8.782444512891389721, 1461.515893433170049, 204.8665823944039914 ) ) ;
#51354=CARTESIAN_POINT ( 'NONE',  ( -12.91642173549690042, 1417.638397378020045, 200.6455995762629811 ) ) ;
#51357=ORIENTED_EDGE ( 'NONE', *, *, #96051, .F. ) ;
#51358=CARTESIAN_POINT ( 'NONE',  ( -11.17096468969999812, 1500.478073591689963, 215.5530715242690007 ) ) ;
#51361=CARTESIAN_POINT ( 'NONE',  ( -4.633397089669999858, 1377.913060387289988, 209.1218459563329759 ) ) ;
#51363=CARTESIAN_POINT ( 'NONE',  ( -10.51130365114040011, 1479.967629185039868, 209.1301374756710061 ) ) ;
#51366=CARTESIAN_POINT ( 'NONE',  ( -17.51440555739999994, 1442.103933559090137, 219.2287671671990097 ) ) ;
#51369=EDGE_CURVE ( 'NONE', #36236, #15891, #37314, .T. ) ;
#51380=CARTESIAN_POINT ( 'NONE',  ( 4.973792553537950134, 1508.551704408389924, 206.3628108551109790 ) ) ;
#51383=ADVANCED_FACE ( 'NONE', ( #21297 ), #101033, .T. ) ;
#51389=B_SPLINE_CURVE_WITH_KNOTS ( 'NONE', 5,
 ( #43572, #77721, #1034, #35157, #69900, #104016 ),
 .UNSPECIFIED., .F., .F.,
 ( 6, 6 ),
 ( 362.7063815370000270, 367.7284095229999821 ),
 .UNSPECIFIED. ) ;
#51390=CARTESIAN_POINT ( 'NONE',  ( 11.75160532048070117, 1479.729357405969949, 209.9771243583440139 ) ) ;
#51397=CARTESIAN_POINT ( 'NONE',  ( 8.062593549087260669, 1436.235959150659937, 206.1283030154239952 ) ) ;
#51403=CARTESIAN_POINT ( 'NONE',  ( 4.749348430879999583, 1472.167733319789932, 187.6580953298989982 ) ) ;
#51409=CARTESIAN_POINT ( 'NONE',  ( 2.330134126628495839, 1515.551704408385831, 213.1059277140580548 ) ) ;
#51410=CARTESIAN_POINT ( 'NONE',  ( 9.170465408922220618, 1461.406018709129967, 205.9602291374590095 ) ) ;
#51413=CARTESIAN_POINT ( 'NONE',  ( -2.245641459690000286, 1475.226982416989813, 197.8915804961989693 ) ) ;
#51420=CARTESIAN_POINT ( 'NONE',  ( -7.973575425169999953, 1425.245987008030170, 205.1887793146490253 ) ) ;
#51427=CARTESIAN_POINT ( 'NONE',  ( 7.527129073409500215, 1425.476184744899911, 212.1957883662609845 ) ) ;
#51429=ORIENTED_EDGE ( 'NONE', *, *, #80934, .T. ) ;
#51431=CARTESIAN_POINT ( 'NONE',  ( -10.96112826740149870, 1492.491747564250090, 207.2364351939560265 ) ) ;
#51435=CARTESIAN_POINT ( 'NONE',  ( 7.892648486029999688, 1424.312437875390060, 211.9575832887890101 ) ) ;
#51454=CARTESIAN_POINT ( 'NONE',  ( -3.824657317049999783, 1429.713551374290091, 201.7356719887889938 ) ) ;
#51460=EDGE_LOOP ( 'NONE', ( #43541, #102918, #8612, #67544 ) ) ;
#51463=CARTESIAN_POINT ( 'NONE',  ( -2.640559407880699982, 1508.551704408389924, 214.1054286845740080 ) ) ;
#51465=CARTESIAN_POINT ( 'NONE',  ( 7.481687810619999546, 1422.866741622099880, 195.6598841224989940 ) ) ;
#51476=EDGE_CURVE ( 'NONE', #94471, #50492, #29367, .T. ) ;
#51482=CARTESIAN_POINT ( 'NONE',  ( -10.22150738884329968, 1483.444541873599974, 203.0139270434760022 ) ) ;
#51485=CARTESIAN_POINT ( 'NONE',  ( 9.270085536629588674, 1427.204361394170064, 210.8459614755520022 ) ) ;
#51486=CARTESIAN_POINT ( 'NONE',  ( 1.547169282253892053, 1421.459440452008039, 193.7923915457423902 ) ) ;
#51487=CARTESIAN_POINT ( 'NONE',  ( -11.02391225866199953, 1462.506727572930004, 208.4595876642919734 ) ) ;
#51490=CARTESIAN_POINT ( 'NONE',  ( -10.24091433091644809, 1479.068389395743679, 211.4585749931201235 ) ) ;
#51493=CARTESIAN_POINT ( 'NONE',  ( -9.686238329417539816, 1461.028144820860007, 208.9774245188330042 ) ) ;
#51494=CARTESIAN_POINT ( 'NONE',  ( 2.645368138919999890, 1426.526422906339803, 188.7496620777990017 ) ) ;
#51495=CARTESIAN_POINT ( 'NONE',  ( 11.32501011340429997, 1425.466614524120132, 201.3329890293439917 ) ) ;
#51496=CARTESIAN_POINT ( 'NONE',  ( 5.378706850333720091, 1465.763327832039977, 218.3327295566870134 ) ) ;
#51502=CARTESIAN_POINT ( 'NONE',  ( 0.6427929286027795897, 1477.829905493179695, 198.7252071007316090 ) ) ;
#51504=CARTESIAN_POINT ( 'NONE',  ( -1.485593186740000071, 1515.527915486090023, 205.0761616848290032 ) ) ;
#51505=CARTESIAN_POINT ( 'NONE',  ( 5.826428076080000906, 1473.811884028689974, 218.9454251420289950 ) ) ;
#51507=CARTESIAN_POINT ( 'NONE',  ( -19.73707540517630221, 1467.795348456740157, 204.3773263242620146 ) ) ;
#51509=CARTESIAN_POINT ( 'NONE',  ( -11.35287584023299878, 1423.238978238550089, 204.2096404009320167 ) ) ;
#51512=CARTESIAN_POINT ( 'NONE',  ( 4.010802518989999399, 1440.993092037090037, 217.7599617541789883 ) ) ;
#51516=CARTESIAN_POINT ( 'NONE',  ( 3.250000000000000000, 1524.051704408389924, 209.1218459616989946 ) ) ;
#51520=CARTESIAN_POINT ( 'NONE',  ( -10.96582334520000046, 1470.988105993590125, 208.9883436308459750 ) ) ;
#51524=CARTESIAN_POINT ( 'NONE',  ( -9.198895294782719390, 1437.332964060710310, 212.8805274561509862 ) ) ;
#51525=EDGE_CURVE ( 'NONE', #10141, #77824, #94828, .T. ) ;
#51528=CARTESIAN_POINT ( 'NONE',  ( -10.35182684444420076, 1472.068470821749997, 207.0629838042650022 ) ) ;
#51533=CARTESIAN_POINT ( 'NONE',  ( 10.91486453896849973, 1422.290287042430009, 209.5939553138669851 ) ) ;
#51535=EDGE_CURVE ( 'NONE', #52413, #43913, #45475, .T. ) ;
#51538=ORIENTED_EDGE ( 'NONE', *, *, #76021, .F. ) ;
#51539=CARTESIAN_POINT ( 'NONE',  ( 4.650852508730000778, 1472.634552772589814, 218.1962482253990174 ) ) ;
#51541=CARTESIAN_POINT ( 'NONE',  ( 18.72979941119999836, 1454.437773883689943, 204.5413093961989830 ) ) ;
#51548=CARTESIAN_POINT ( 'NONE',  ( 5.134328406469999884, 1447.265806521789955, 200.6829430861090202 ) ) ;
#51550=B_SPLINE_CURVE_WITH_KNOTS ( 'NONE', 5,
 ( #25450, #93754, #17031, #51794, #8657, #36640, #3617, #61872, #54574, #97647, #19823, #20917 ),
 .UNSPECIFIED., .F., .F.,
 ( 6, 3, 3, 6 ),
 ( 0.000000000000000000, 0.4064120419304899090, 0.8128240838611042740, 1.000000000000000000 ),
 .UNSPECIFIED. ) ;
#51553=CARTESIAN_POINT ( 'NONE',  ( -2.455032153949999962, 1454.699340087689961, 198.9067334848990072 ) ) ;
#51559=CARTESIAN_POINT ( 'NONE',  ( -3.394304438509999855, 1495.766742855890016, 197.6817022580989942 ) ) ;
#51567=CARTESIAN_POINT ( 'NONE',  ( -8.881784197000000993E-16, 1391.913060387289988, 209.1218459616989946 ) ) ;
#51573=VECTOR ( 'NONE', #12176, 1000.000000000000227 ) ;
#51579=CARTESIAN_POINT ( 'NONE',  ( 4.850704082057680111, 1508.551704408389924, 212.4235637436360093 ) ) ;
#51583=CARTESIAN_POINT ( 'NONE',  ( 9.669214496953919991, 1462.615592212159982, 207.8321519686910221 ) ) ;
#51587=CARTESIAN_POINT ( 'NONE',  ( 9.837801962708470072, 1453.205870278119846, 211.6882699933420042 ) ) ;
#51591=CARTESIAN_POINT ( 'NONE',  ( -14.16402923184379858, 1508.451126306549895, 209.7829216516819884 ) ) ;
#51592=CARTESIAN_POINT ( 'NONE',  ( -1.260434061590582910, 1444.023716841911892, 199.8554606798724365 ) ) ;
#51593=CARTESIAN_POINT ( 'NONE',  ( 12.51045652733512981, 1414.677402202029953, 211.4999743317719663 ) ) ;
#51595=CARTESIAN_POINT ( 'NONE',  ( 9.224564342578489118, 1450.690345550029861, 209.5619459605489965 ) ) ;
#51603=B_SPLINE_CURVE_WITH_KNOTS ( 'NONE', 5,
 ( #14702, #41575, #33699, #83554, #84656, #75186 ),
 .UNSPECIFIED., .F., .F.,
 ( 6, 6 ),
 ( 0.000000000000000000, 1.000000000000000000 ),
 .UNSPECIFIED. ) ;
#51609=CARTESIAN_POINT ( 'NONE',  ( -7.318182648980661398, 1489.884714771882273, 217.2580560210730027 ) ) ;
#51612=LINE ( 'NONE', #83539, #13752 ) ;
#51614=CARTESIAN_POINT ( 'NONE',  ( 5.400236726889999339, 1493.509547987889846, 218.8212158057690147 ) ) ;
#51618=CARTESIAN_POINT ( 'NONE',  ( 8.892135936816799813, 1468.525511668620084, 202.2742229671289920 ) ) ;
#51627=CARTESIAN_POINT ( 'NONE',  ( 0.04897144338186310009, 1515.158513834189989, 204.7948513551449992 ) ) ;
#51640=CARTESIAN_POINT ( 'NONE',  ( 10.52837420263239920, 1481.199010226290284, 208.2608686310830137 ) ) ;
#51653=CARTESIAN_POINT ( 'NONE',  ( -15.06253099230000103, 1415.635739491490085, 205.8115256829090072 ) ) ;
#51656=CARTESIAN_POINT ( 'NONE',  ( -5.167079976729559654, 1484.950571581749955, 198.3957337195609796 ) ) ;
#51657=CARTESIAN_POINT ( 'NONE',  ( -15.94781981578667995, 1419.817486795263449, 210.5094882503032352 ) ) ;
#51665=CARTESIAN_POINT ( 'NONE',  ( -14.75797208140014938, 1418.752374206816057, 201.0754936769993151 ) ) ;
#51676=CARTESIAN_POINT ( 'NONE',  ( -8.194496425724276278, 1495.378119627901697, 201.4616218148407256 ) ) ;
#51682=CARTESIAN_POINT ( 'NONE',  ( 11.16961893628350033, 1479.160307786130033, 207.2818337165830087 ) ) ;
#51683=CARTESIAN_POINT ( 'NONE',  ( -4.046039468759740743, 1455.103744561050235, 203.6879517955759979 ) ) ;
#51684=CARTESIAN_POINT ( 'NONE',  ( 4.955072371518870256, 1436.062886099170100, 228.7521548814630137 ) ) ;
#51686=CARTESIAN_POINT ( 'NONE',  ( -0.03314732912356650046, 1502.038625534309858, 233.2541157079660081 ) ) ;
#51691=CARTESIAN_POINT ( 'NONE',  ( -11.38785606999999978, 1490.657837854590070, 209.9657568313180036 ) ) ;
#51692=CARTESIAN_POINT ( 'NONE',  ( 7.361562866177969511, 1448.713196798179979, 201.9147366591519983 ) ) ;
#51702=CARTESIAN_POINT ( 'NONE',  ( -9.927720267860891568, 1422.647037618466356, 210.6683186352579185 ) ) ;
#51709=CARTESIAN_POINT ( 'NONE',  ( -3.641325192198154870, 1462.848003559786548, 199.9870330951486324 ) ) ;
#51712=CARTESIAN_POINT ( 'NONE',  ( -1.333619433810000254, 1444.154719577489914, 199.5606630350989974 ) ) ;
#51714=EDGE_CURVE ( 'NONE', #74194, #75452, #52903, .T. ) ;
#51720=CARTESIAN_POINT ( 'NONE',  ( 3.172882057879999884, 1467.373998898590116, 218.6974008828489673 ) ) ;
#51723=B_SPLINE_SURFACE_WITH_KNOTS ( 'NONE', 5, 5, ( 
 ( #97992, #12334, #46525, #73363, #5042, #106408 ),
 ( #80659, #82307, #81734, #22364, #30235, #30792 ),
 ( #5605, #107500, #64971, #45966, #106949, #21259 ),
 ( #64426, #56565, #39756, #108046, #65527, #75025 ),
 ( #100208, #49824, #109176, #16177, #110255, #76115 ),
 ( #83953, #57684, #31897, #101277, #24574, #58765 ),
 ( #67731, #59336, #92345, #93446, #82850, #110810 ),
 ( #15617, #58220, #66082, #23492, #15075, #6140 ),
 ( #14536, #7254, #91798, #92903, #8338, #33529 ) ),
 .UNSPECIFIED., .F., .F., .F.,
 ( 6, 3, 6 ),
 ( 6, 6 ),
 ( 3.132904301029519889, 5.380600720280000360, 7.628289045712770111 ),
 ( -0.0004171348989584099847, 2.000000000000000000 ),
 .UNSPECIFIED. ) ;
#51728=ORIENTED_EDGE ( 'NONE', *, *, #13834, .T. ) ;
#51730=ORIENTED_EDGE ( 'NONE', *, *, #1511, .T. ) ;
#51734=CARTESIAN_POINT ( 'NONE',  ( -8.305592643558565413, 1474.704246973548607, 203.0641412134559403 ) ) ;
#51739=CARTESIAN_POINT ( 'NONE',  ( 12.39400990049870011, 1421.652661456120086, 207.6978078727499906 ) ) ;
#51748=ORIENTED_EDGE ( 'NONE', *, *, #24232, .T. ) ;
#51752=VERTEX_POINT ( 'NONE', #54572 ) ;
#51754=CARTESIAN_POINT ( 'NONE',  ( -16.17659802858249662, 1508.551704408389924, 210.3807973950520136 ) ) ;
#51756=CARTESIAN_POINT ( 'NONE',  ( 8.225616979109998894, 1452.226705206789802, 213.5360760307489727 ) ) ;
#51761=CARTESIAN_POINT ( 'NONE',  ( 1.946290797379999882, 1468.809136692889979, 216.1326187760289770 ) ) ;
#51765=CARTESIAN_POINT ( 'NONE',  ( -11.79975722151939976, 1482.296391875749805, 207.6022922335340297 ) ) ;
#51774=B_SPLINE_CURVE_WITH_KNOTS ( 'NONE', 3,
 ( #39416, #48387, #108823, #50035, #7464, #109933, #33211, #98765, #22027, #82530, #5826, #108272, #31558, #93116, #51135, #44400, #26461, #50582, #86931, #67400, #16386, #16933 ),
 .UNSPECIFIED., .F., .F.,
 ( 4, 3, 3, 3, 3, 3, 3, 4 ),
 ( 10.65476131940000037, 12.10693589158530159, 12.77474861870000034, 14.28402943510999989, 15.71731362297010115, 16.21876727693750198, 17.58349865633480036, 18.78936860560000000 ),
 .UNSPECIFIED. ) ;
#51775=CARTESIAN_POINT ( 'NONE',  ( -18.15654714260000091, 1466.352650648189865, 200.0994765531190183 ) ) ;
#51782=CARTESIAN_POINT ( 'NONE',  ( -10.71865670083870192, 1508.438609848949909, 218.4505424401079949 ) ) ;
#51786=CARTESIAN_POINT ( 'NONE',  ( -9.234134023826198856, 1461.205490114660051, 206.1827678865119822 ) ) ;
#51787=CARTESIAN_POINT ( 'NONE',  ( 3.313200396079999610, 1466.616402805890175, 219.2512007924990201 ) ) ;
#51792=CARTESIAN_POINT ( 'NONE',  ( -2.348673686699999763, 1430.656302287590051, 201.0926571014589967 ) ) ;
#51794=CARTESIAN_POINT ( 'NONE',  ( 6.937425782160731025, 1464.940099892885883, 217.7535805317997131 ) ) ;
#51795=CARTESIAN_POINT ( 'NONE',  ( -9.244895511235538876, 1448.612347789799969, 209.9869602076240085 ) ) ;
#51799=CARTESIAN_POINT ( 'NONE',  ( 1.953870304974810068, 1456.496003654670176, 219.5623012099979690 ) ) ;
#51801=PLANE ( 'NONE',  #16676 ) ;
#51803=CARTESIAN_POINT ( 'NONE',  ( 11.45577218270000053, 1502.286415152389964, 208.3140800519860250 ) ) ;
#51806=CARTESIAN_POINT ( 'NONE',  ( 7.919198134229999297, 1428.084552926790138, 213.0326556074190307 ) ) ;
#51818=CARTESIAN_POINT ( 'NONE',  ( -13.40902085879850070, 1483.658216990520032, 225.6646531694549935 ) ) ;
#51823=CARTESIAN_POINT ( 'NONE',  ( -14.82486707557663586, 1416.127778529439411, 204.8631623252366580 ) ) ;
#51825=CARTESIAN_POINT ( 'NONE',  ( -2.676030461421510243, 1457.817666378469767, 219.4510933441680152 ) ) ;
#51831=CARTESIAN_POINT ( 'NONE',  ( -20.36853080839999919, 1464.956632876090225, 210.9458194778790130 ) ) ;
#51835=CARTESIAN_POINT ( 'NONE',  ( 5.183480683570000025, 1454.129157349589832, 216.9717332163589845 ) ) ;
#51839=CARTESIAN_POINT ( 'NONE',  ( -21.61356760059999971, 1507.917715158790088, 209.5243360325540039 ) ) ;
#51843=EDGE_CURVE ( 'NONE', #60672, #91618, #52680, .T. ) ;
#51845=CARTESIAN_POINT ( 'NONE',  ( 1.953691794509409663, 1476.191320038690037, 197.7993456081649981 ) ) ;
#51857=ORIENTED_EDGE ( 'NONE', *, *, #98653, .F. ) ;
#51867=CIRCLE ( 'NONE', #12536, 1.999999999999994227 ) ;
#51894=CARTESIAN_POINT ( 'NONE',  ( -9.023097092110859307, 1493.387773720369978, 200.7584573620279969 ) ) ;
#51913=DIRECTION ( 'NONE',  ( -0.2360473468807729458, 0.3679196751255739417, -0.8993980001567938309 ) ) ;
#51918=CARTESIAN_POINT ( 'NONE',  ( 1.959285284397550120, 1474.800623515119923, 220.3715842348549927 ) ) ;
#51920=CARTESIAN_POINT ( 'NONE',  ( 8821.345249565620179, 5182.654794667094393, -2585.374449305243161 ) ) ;
#51922=CARTESIAN_POINT ( 'NONE',  ( -14.79231131374850072, 1418.341681852919919, 202.2100798908639945 ) ) ;
#51923=CARTESIAN_POINT ( 'NONE',  ( 4.329294185584050325, 1515.070696454110021, 207.5527501733459985 ) ) ;
#51926=CARTESIAN_POINT ( 'NONE',  ( -7.672264733570000494, 1508.551704439589912, 219.1253561400989724 ) ) ;
#51930=CARTESIAN_POINT ( 'NONE',  ( -10.48474110849999974, 1480.275079708390194, 208.2232256045050178 ) ) ;
#51933=CARTESIAN_POINT ( 'NONE',  ( -4.636604420221742906, 1378.026799461571272, 203.9259778311827063 ) ) ;
#51939=CARTESIAN_POINT ( 'NONE',  ( 10.36440324736019925, 1451.671856551549809, 207.3348124021030117 ) ) ;
#51946=VERTEX_POINT ( 'NONE', #79208 ) ;
#51949=CARTESIAN_POINT ( 'NONE',  ( -3.737543590866930110, 1457.196795654610014, 214.7727701001950038 ) ) ;
#51954=CARTESIAN_POINT ( 'NONE',  ( 8.750084289021121009, 1436.836525569339756, 209.7700227241190021 ) ) ;
#51959=CARTESIAN_POINT ( 'NONE',  ( 3.116401324629539893, 1487.019696768639960, 197.5841379987910216 ) ) ;
#51961=CARTESIAN_POINT ( 'NONE',  ( -9.198164182857258453, 1450.369964096400054, 208.5037453834269741 ) ) ;
#51962=CARTESIAN_POINT ( 'NONE',  ( -8.535066471915349950, 1424.913453952659893, 204.9008513312109869 ) ) ;
#51967=CARTESIAN_POINT ( 'NONE',  ( -12.35793136629999900, 1506.116535470989902, 208.8889582108720049 ) ) ;
#51968=CARTESIAN_POINT ( 'NONE',  ( 22.27437808960000254, 1476.550945564490121, 209.6594615055550150 ) ) ;
#51972=CARTESIAN_POINT ( 'NONE',  ( -3.227261282950000254, 1476.559864218489793, 202.2993187396990038 ) ) ;
#51973=CARTESIAN_POINT ( 'NONE',  ( 2.330134126090000368, 1515.064792882589927, 213.4512947377390049 ) ) ;
#51975=CARTESIAN_POINT ( 'NONE',  ( -2.039114686836970058, 1421.064113876339889, 193.7872318451859712 ) ) ;
#51983=CARTESIAN_POINT ( 'NONE',  ( -8.110586521360000134, 1425.115383700800066, 209.5285450949000108 ) ) ;
#51989=CARTESIAN_POINT ( 'NONE',  ( 7.499492845059839929, 1425.981480573469753, 212.3193081490009888 ) ) ;
#51998=CARTESIAN_POINT ( 'NONE',  ( -0.07708582513870239350, 1460.859163483989960, 228.7412678487989979 ) ) ;
#52004=DIRECTION ( 'NONE',  ( -0.02616798426450828510, 0.9993150019883944024, 0.02616798426450818449 ) ) ;
#52017=CARTESIAN_POINT ( 'NONE',  ( -4.820692999790000322, 1427.981916302389891, 201.4689414325489736 ) ) ;
#52024=EDGE_LOOP ( 'NONE', ( #49322, #54683, #14513, #73488 ) ) ;
#52025=CARTESIAN_POINT ( 'NONE',  ( 4.240940644616750355, 1509.032041130069956, 205.3774179143429990 ) ) ;
#52026=B_SPLINE_CURVE_WITH_KNOTS ( 'NONE', 3,
 ( #64177, #96663, #46827, #54680 ),
 .UNSPECIFIED., .F., .F.,
 ( 4, 4 ),
 ( 0.000000000000000000, 1.000000000000000000 ),
 .UNSPECIFIED. ) ;
#52031=CARTESIAN_POINT ( 'NONE',  ( 2.487935123032368967, 1508.603735228351297, 204.3914617891122703 ) ) ;
#52033=CARTESIAN_POINT ( 'NONE',  ( 7.535268056249999624, 1422.940929649649888, 195.7043803497990098 ) ) ;
#52043=ORIENTED_EDGE ( 'NONE', *, *, #1905, .F. ) ;
#52047=CARTESIAN_POINT ( 'NONE',  ( -7.853014526819640295, 1484.259593461030136, 200.1697423039280181 ) ) ;
#52049=CARTESIAN_POINT ( 'NONE',  ( -1.599049516947889105, 1420.649782495757108, 193.7985443746896124 ) ) ;
#52051=CARTESIAN_POINT ( 'NONE',  ( -4.328404850859190134, 1515.104658776890119, 208.0669027827329955 ) ) ;
#52057=EDGE_CURVE ( 'NONE', #108598, #44333, #70662, .T. ) ;
#52059=CARTESIAN_POINT ( 'NONE',  ( -13.97983274584369973, 1420.196076808720136, 195.9955686830610091 ) ) ;
#52060=CARTESIAN_POINT ( 'NONE',  ( 11.64982809710589962, 1421.677256869899793, 203.4368870229210131 ) ) ;
#52061=CARTESIAN_POINT ( 'NONE',  ( 10.52578744093320040, 1462.363382362089851, 212.2902631912189975 ) ) ;
#52066=CARTESIAN_POINT ( 'NONE',  ( -8.116894974276100072, 1425.431424825695331, 208.6843198518954523 ) ) ;
#52070=CARTESIAN_POINT ( 'NONE',  ( 4.803837556235689199, 1471.771475080379787, 187.6888395172460093 ) ) ;
#52072=CARTESIAN_POINT ( 'NONE',  ( -13.75591821840509965, 1421.742616532689908, 205.2219009381699948 ) ) ;
#52073=CARTESIAN_POINT ( 'NONE',  ( 9.181100887863649973, 1450.964097471789955, 210.1935140534000084 ) ) ;
#52074=CARTESIAN_POINT ( 'NONE',  ( 3.899014136759999971, 1442.684943332589910, 217.1061286285590199 ) ) ;
#52075=ORIENTED_EDGE ( 'NONE', *, *, #42568, .F. ) ;
#52080=ADVANCED_FACE ( 'NONE', ( #49457 ), #20382, .T. ) ;
#52082=CARTESIAN_POINT ( 'NONE',  ( -17.11734631873629908, 1420.830859248140086, 201.6585988287660030 ) ) ;
#52083=ORIENTED_EDGE ( 'NONE', *, *, #80068, .F. ) ;
#52084=CARTESIAN_POINT ( 'NONE',  ( -10.14857146029999946, 1472.086425142190137, 209.7191475309859925 ) ) ;
#52096=CARTESIAN_POINT ( 'NONE',  ( 9.490563787272430218, 1424.812203410370103, 209.0803129943540171 ) ) ;
#52102=CARTESIAN_POINT ( 'NONE',  ( -19.67625207089999861, 1467.566588935489790, 206.2108820087490244 ) ) ;
#52110=CARTESIAN_POINT ( 'NONE',  ( -7302.760118613915438, 5181.793945261120825, -10646.37847981480263 ) ) ;
#52114=CARTESIAN_POINT ( 'NONE',  ( 1.102161665280000147, 1456.373626168390047, 198.9794195941990154 ) ) ;
#52120=CARTESIAN_POINT ( 'NONE',  ( -3.617573937850000032, 1497.333809982789944, 198.4503636364990200 ) ) ;
#52121=CARTESIAN_POINT ( 'NONE',  ( -3.619841760469999947, 1497.142537370389846, 220.5541520919989864 ) ) ;
#52136=CARTESIAN_POINT ( 'NONE',  ( -4.992622102040000343, 1391.631309831290082, 214.6079342942889809 ) ) ;
#52140=CARTESIAN_POINT ( 'NONE',  ( 9.597484669293001147, 1461.985966042660266, 207.5232997255220084 ) ) ;
#52143=VERTEX_POINT ( 'NONE', #44365 ) ;
#52144=FACE_OUTER_BOUND ( 'NONE', #87665, .T. ) ;
#52148=CARTESIAN_POINT ( 'NONE',  ( -9.534864884007895114, 1418.422607348942392, 197.0272821719209730 ) ) ;
#52154=CARTESIAN_POINT ( 'NONE',  ( 10.12302436080650025, 1452.223079970169920, 209.0282544715680046 ) ) ;
#52163=VECTOR ( 'NONE', #82608, 1000.000000000000227 ) ;
#52170=CARTESIAN_POINT ( 'NONE',  ( -1.748905610829809998, 1488.269106374019884, 219.8524659745219765 ) ) ;
#52173=CARTESIAN_POINT ( 'NONE',  ( 9.207192151108898770, 1450.833480228639928, 209.8877954179420158 ) ) ;
#52174=CARTESIAN_POINT ( 'NONE',  ( -12.64341534048310045, 1502.151632001139888, 210.8278707494170021 ) ) ;
#52175=CARTESIAN_POINT ( 'NONE',  ( 7.220783133089999417, 1493.964658354389940, 218.1716920474590040 ) ) ;
#52179=CARTESIAN_POINT ( 'NONE',  ( -3.699130484579999933, 1497.303414919790157, 198.4797053902989887 ) ) ;
#52183=FACE_OUTER_BOUND ( 'NONE', #72739, .T. ) ;
#52189=CARTESIAN_POINT ( 'NONE',  ( -14.80222597220000047, 1415.865102022439942, 213.2039056074190171 ) ) ;
#52190=EDGE_CURVE ( 'NONE', #46077, #73174, #7736, .T. ) ;
#52191=CARTESIAN_POINT ( 'NONE',  ( 1.130521170281699961, 1515.098624608320051, 204.7932831006150138 ) ) ;
#52192=ORIENTED_EDGE ( 'NONE', *, *, #35830, .T. ) ;
#52197=CARTESIAN_POINT ( 'NONE',  ( -10.95020795142180070, 1462.043827289809997, 210.3303817636600002 ) ) ;
#52203=CARTESIAN_POINT ( 'NONE',  ( 16.35241204879999799, 1473.763677363790066, 196.1841466627989803 ) ) ;
#52204=CARTESIAN_POINT ( 'NONE',  ( -9.562019153030000496, 1479.258837048789928, 214.5473981509090038 ) ) ;
#52215=CARTESIAN_POINT ( 'NONE',  ( 6.674324621289978055, 1480.055983087696859, 228.4398896743051068 ) ) ;
#52219=CARTESIAN_POINT ( 'NONE',  ( -2.519506328514930171, 1485.538153147889943, 197.4903980647760022 ) ) ;
#52221=CARTESIAN_POINT ( 'NONE',  ( -4.922266137120000273, 1497.746000166390104, 220.5680551797990177 ) ) ;
#52228=B_SPLINE_CURVE_WITH_KNOTS ( 'NONE', 5,
 ( #9626, #36498, #52760, #86896, #44363, #78508, #52215, #77947, #1818 ),
 .UNSPECIFIED., .F., .F.,
 ( 6, 3, 6 ),
 ( 0.000000000000000000, 0.7707393916760963970, 1.000000000000000000 ),
 .UNSPECIFIED. ) ;
#52245=CARTESIAN_POINT ( 'NONE',  ( 3.842540062219999886, 1485.442838166189858, 219.2998310712989962 ) ) ;
#52246=CARTESIAN_POINT ( 'NONE',  ( 5.057113137720000040, 1424.030137378339987, 193.7146021066990045 ) ) ;
#52249=CARTESIAN_POINT ( 'NONE',  ( 18.90935262129999828, 1456.544091939490045, 200.1670491895490045 ) ) ;
#52250=CARTESIAN_POINT ( 'NONE',  ( -3.892696961574322323, 1515.551704300027950, 210.6723164294263029 ) ) ;
#52255=CARTESIAN_POINT ( 'NONE',  ( 9.691987769041398693, 1436.253413666279812, 210.7989517529429975 ) ) ;
#52256=CARTESIAN_POINT ( 'NONE',  ( -10.95999825190000010, 1490.767389346189930, 211.0929827415589841 ) ) ;
#52257=CARTESIAN_POINT ( 'NONE',  ( 3.728847569731689848, 1446.583145393379937, 199.6841023494010017 ) ) ;
#52263=CARTESIAN_POINT ( 'NONE',  ( 14.02295695628119887, 1432.459693560080041, 221.0332480332689897 ) ) ;
#52266=CARTESIAN_POINT ( 'NONE',  ( 5.662322984621799726, 1504.894625891569831, 220.5557319434630017 ) ) ;
#52275=CARTESIAN_POINT ( 'NONE',  ( -10.34166276688940123, 1447.760272548699959, 209.7025959161350102 ) ) ;
#52286=CARTESIAN_POINT ( 'NONE',  ( -4.761835946750000659, 1382.817942133689940, 214.6047291967390152 ) ) ;
#52291=CARTESIAN_POINT ( 'NONE',  ( -1.005805788909989840, 1431.851947266499792, 200.7719531180060244 ) ) ;
#52296=CARTESIAN_POINT ( 'NONE',  ( -11.36959371680000075, 1503.847165134090119, 207.0750569533189775 ) ) ;
#52299=CARTESIAN_POINT ( 'NONE',  ( -1.636057583032799911, 1465.068318594939910, 198.2397572230070182 ) ) ;
#52307=EDGE_LOOP ( 'NONE', ( #83288, #17387, #73380, #65203 ) ) ;
#52310=EDGE_CURVE ( 'NONE', #43776, #72498, #96839, .T. ) ;
#52315=CARTESIAN_POINT ( 'NONE',  ( 4.905383437976600369, 1424.139022048180095, 193.2146529292390085 ) ) ;
#52320=DIRECTION ( 'NONE',  ( 1.224646799147350002E-16, -1.836970198721029688E-16, -1.000000000000000000 ) ) ;
#52326=CARTESIAN_POINT ( 'NONE',  ( -2.863667357675800496, 1428.996785130359967, 200.2011281577639750 ) ) ;
#52335=CARTESIAN_POINT ( 'NONE',  ( 10.52331109828659983, 1491.075809623180021, 212.3133573343550040 ) ) ;
#52337=B_SPLINE_CURVE_WITH_KNOTS ( 'NONE', 3,
 ( #62831, #53299, #104785, #61169 ),
 .UNSPECIFIED., .F., .F.,
 ( 4, 4 ),
 ( 0.000000000000000000, 1.000000000000000000 ),
 .UNSPECIFIED. ) ;
#52356=CARTESIAN_POINT ( 'NONE',  ( 6.039845038650000220, 1450.200509660590114, 208.6657063127539971 ) ) ;
#52360=FACE_OUTER_BOUND ( 'NONE', #66611, .T. ) ;
#52361=CARTESIAN_POINT ( 'NONE',  ( 10.57326081867249989, 1481.032691398090037, 210.7950195358730241 ) ) ;
#52362=CARTESIAN_POINT ( 'NONE',  ( -0.5682668705760020034, 1506.801775235190007, 221.9434713837989932 ) ) ;
#52363=CARTESIAN_POINT ( 'NONE',  ( -8.254331781353046793, 1448.308236332938350, 213.1040624623483950 ) ) ;
#52366=CARTESIAN_POINT ( 'NONE',  ( 3.392304019253070013, 1456.149158459580121, 219.1891682523919940 ) ) ;
#52367=CARTESIAN_POINT ( 'NONE',  ( 2.645773951119999801, 1485.597577325490192, 198.6813594259990055 ) ) ;
#52370=CARTESIAN_POINT ( 'NONE',  ( 11.49924241569999950, 1502.518364560089822, 209.1346295538230038 ) ) ;
#52376=CARTESIAN_POINT ( 'NONE',  ( 3.829620154741123716, 1515.551704408389696, 212.3304832152426229 ) ) ;
#52383=CARTESIAN_POINT ( 'NONE',  ( -6.817824598025731042, 1490.769479965739720, 213.3956848422870110 ) ) ;
#52386=CARTESIAN_POINT ( 'NONE',  ( -11.33475729309999913, 1500.341569084289858, 210.4138247025489932 ) ) ;
#52389=CARTESIAN_POINT ( 'NONE',  ( -9.972525074869899697, 1439.148125713659965, 209.2054671327859694 ) ) ;
#52390=CARTESIAN_POINT ( 'NONE',  ( 2.041884302589999756, 1451.400483888490044, 190.0484128324990252 ) ) ;
#52393=CARTESIAN_POINT ( 'NONE',  ( 7.535581150919999693, 1424.790543398920136, 212.1876082168290054 ) ) ;
#52394=CARTESIAN_POINT ( 'NONE',  ( 20.75865325819999896, 1455.056399776190119, 207.3304373729289978 ) ) ;
#52399=ORIENTED_EDGE ( 'NONE', *, *, #81097, .F. ) ;
#52400=VERTEX_POINT ( 'NONE', #57602 ) ;
#52406=CARTESIAN_POINT ( 'NONE',  ( -0.03257067699863269716, 1475.780217561950167, 197.6613938121659828 ) ) ;
#52413=VERTEX_POINT ( 'NONE', #6618 ) ;
#52414=CARTESIAN_POINT ( 'NONE',  ( 3.289090359600000291, 1441.224765589789968, 218.4797294130789851 ) ) ;
#52417=ORIENTED_EDGE ( 'NONE', *, *, #20601, .T. ) ;
#52423=ORIENTED_EDGE ( 'NONE', *, *, #100930, .F. ) ;
#52432=CARTESIAN_POINT ( 'NONE',  ( 9.698064461892839105, 1462.705242386489999, 208.0596150282290182 ) ) ;
#52436=CARTESIAN_POINT ( 'NONE',  ( 10.57993308616552319, 1425.618513008048012, 196.6680084146474599 ) ) ;
#52445=CARTESIAN_POINT ( 'NONE',  ( 16.33719110018399689, 1478.134947818610044, 222.4389267383260176 ) ) ;
#52446=CARTESIAN_POINT ( 'NONE',  ( -21.26809175218030035, 1485.919042415889862, 201.7808329802730327 ) ) ;
#52452=VERTEX_POINT ( 'NONE', #82774 ) ;
#52454=CARTESIAN_POINT ( 'NONE',  ( -3.586492549349999948, 1428.590318077689972, 200.4729775719390261 ) ) ;
#52459=FACE_OUTER_BOUND ( 'NONE', #12578, .T. ) ;
#52460=CARTESIAN_POINT ( 'NONE',  ( 9.694557698560979375, 1462.254025613590102, 208.2085395587480150 ) ) ;
#52462=CARTESIAN_POINT ( 'NONE',  ( 10.53169424880000093, 1481.128073908389979, 211.0447647956590060 ) ) ;
#52471=CARTESIAN_POINT ( 'NONE',  ( -12.85215753329999977, 1508.300510831589918, 209.4336657455189936 ) ) ;
#52474=CARTESIAN_POINT ( 'NONE',  ( 3.346707516019999940, 1443.005054410889898, 217.3642451189890323 ) ) ;
#52479=CARTESIAN_POINT ( 'NONE',  ( -7.317283160083440485, 1458.197890023347327, 215.2731315594757007 ) ) ;
#52482=CARTESIAN_POINT ( 'NONE',  ( -14.33183065600080042, 1418.593864405419936, 201.2805417143829914 ) ) ;
#52483=CARTESIAN_POINT ( 'NONE',  ( 8.062587302181759341, 1436.235894220949831, 206.1282943059349861 ) ) ;
#52493=CARTESIAN_POINT ( 'NONE',  ( -1.748695796902800081, 1488.269352622320184, 219.8525110836319811 ) ) ;
#52499=CARTESIAN_POINT ( 'NONE',  ( 10.40969047044820073, 1451.775060363849889, 207.5610707736619815 ) ) ;
#52500=ORIENTED_EDGE ( 'NONE', *, *, #15071, .T. ) ;
#52507=CARTESIAN_POINT ( 'NONE',  ( -18.10740131676499942, 1463.999236119600255, 217.9813976188680158 ) ) ;
#52511=CARTESIAN_POINT ( 'NONE',  ( 8.658448668542680693, 1437.810433862630134, 209.6180638252519941 ) ) ;
#52519=CARTESIAN_POINT ( 'NONE',  ( -10.73901725096249926, 1423.590975015609956, 204.3534390747859959 ) ) ;
#52522=VERTEX_POINT ( 'NONE', #11043 ) ;
#52524=CARTESIAN_POINT ( 'NONE',  ( 18.33936911297750072, 1473.566272301189883, 194.9299536566859956 ) ) ;
#52538=CARTESIAN_POINT ( 'NONE',  ( -8.087399829960000730, 1423.889215342339867, 210.5428868746689943 ) ) ;
#52544=CARTESIAN_POINT ( 'NONE',  ( 7.506693744642929822, 1425.950106240180048, 212.2988314193449924 ) ) ;
#52546=CARTESIAN_POINT ( 'NONE',  ( -1.933463630428559954, 1496.738328175310016, 221.3394013225409935 ) ) ;
#52553=CARTESIAN_POINT ( 'NONE',  ( -18.38283541797299847, 1508.551704415689983, 210.6369374182840204 ) ) ;
#52554=CARTESIAN_POINT ( 'NONE',  ( 0.6364662242309990781, 1454.894301978690009, 215.7249498071190033 ) ) ;
#52555=CARTESIAN_POINT ( 'NONE',  ( -8.245270369270169653, 1438.570843674859816, 206.3270951701919955 ) ) ;
#52577=CARTESIAN_POINT ( 'NONE',  ( 2.035102182640000201, 1443.701500078689833, 215.0273390923990178 ) ) ;
#52582=CARTESIAN_POINT ( 'NONE',  ( 4.487359741654660006, 1509.034536824670113, 206.0057093087000055 ) ) ;
#52589=B_SPLINE_CURVE_WITH_KNOTS ( 'NONE', 3,
 ( #13351, #48094, #63806, #90627, #14466, #97922 ),
 .UNSPECIFIED., .F., .F.,
 ( 4, 2, 4 ),
 ( 0.000000000000000000, 0.5000000000000000000, 1.000000000000000000 ),
 .UNSPECIFIED. ) ;
#52599=CARTESIAN_POINT ( 'NONE',  ( -8.956927351110008928, 1464.257504697786317, 226.7719248702087498 ) ) ;
#52602=CARTESIAN_POINT ( 'NONE',  ( -19.63485294834822525, 1508.289801357211218, 209.7406608497707339 ) ) ;
#52603=CARTESIAN_POINT ( 'NONE',  ( 0.7340478531541532181, 1421.248697517114806, 193.7332822046788010 ) ) ;
#52610=CARTESIAN_POINT ( 'NONE',  ( -14.54141060630000126, 1422.922756957550064, 196.4113455912990105 ) ) ;
#52611=CARTESIAN_POINT ( 'NONE',  ( 11.55003007508270052, 1421.422333198520164, 201.8131330578860059 ) ) ;
#52619=CARTESIAN_POINT ( 'NONE',  ( -16.96799521795757215, 1419.980406830895845, 207.7863820104928152 ) ) ;
#52622=CARTESIAN_POINT ( 'NONE',  ( 10.99043261664119875, 1479.494642963729802, 229.8297439004759894 ) ) ;
#52626=CARTESIAN_POINT ( 'NONE',  ( 3.718743811529999999, 1442.790811878290242, 217.1968316306989948 ) ) ;
#52630=CARTESIAN_POINT ( 'NONE',  ( -4.692099526989998992, 1474.463958302690116, 198.6947328130989945 ) ) ;
#52632=ORIENTED_EDGE ( 'NONE', *, *, #55715, .T. ) ;
#52633=CARTESIAN_POINT ( 'NONE',  ( -2.140641997699999965, 1508.551704408389924, 220.0635241299990241 ) ) ;
#52635=B_SPLINE_SURFACE_WITH_KNOTS ( 'NONE', 5, 5, ( 
 ( #1772, #70093, #86850, #95257, #70640, #96918 ),
 ( #86298, #104206, #10143, #68980, #87978, #96359 ),
 ( #19637, #36442, #44879, #18518, #52716, #26382 ),
 ( #11266, #20185, #103082, #44316, #79030, #54383 ),
 ( #88516, #104756, #78460, #11800, #79572, #2874 ),
 ( #45968, #28043, #80103, #77905, #12890, #3975 ),
 ( #56014, #29152, #81735, #63877, #98546, #13421 ),
 ( #20726, #30236, #14537, #38099, #108047, #57130 ),
 ( #47611, #48726, #80660, #63338, #89049, #81192 ) ),
 .UNSPECIFIED., .F., .F., .F.,
 ( 6, 3, 6 ),
 ( 6, 6 ),
 ( -0.01213293170383570110, 5.564709931820000399, 10.43218467589399978 ),
 ( -0.01218607079403309992, 1.000000000000000000 ),
 .UNSPECIFIED. ) ;
#52637=CARTESIAN_POINT ( 'NONE',  ( 7.308426574864255620, 1447.450532783193239, 203.7166947410731268 ) ) ;
#52640=CARTESIAN_POINT ( 'NONE',  ( -2.074854266390000035, 1432.268094214490020, 217.6750424900990026 ) ) ;
#52648=CARTESIAN_POINT ( 'NONE',  ( 11.45381602559669965, 1491.761437294190046, 209.6400631038679876 ) ) ;
#52650=ORIENTED_EDGE ( 'NONE', *, *, #86530, .F. ) ;
#52652=ORIENTED_EDGE ( 'NONE', *, *, #85746, .F. ) ;
#52655=CARTESIAN_POINT ( 'NONE',  ( -6.058024923110000515, 1495.048144898590181, 199.2280266695289868 ) ) ;
#52660=CARTESIAN_POINT ( 'NONE',  ( 3.375977075490000257, 1446.395221907989935, 199.5681765173089843 ) ) ;
#52665=B_SPLINE_CURVE_WITH_KNOTS ( 'NONE', 3,
 ( #44457, #27643, #27101, #69680, #103802, #86991, #78601, #3027, #19786, #71346 ),
 .UNSPECIFIED., .F., .F.,
 ( 4, 2, 2, 2, 4 ),
 ( 0.000000000000000000, 0.2500000000000107692, 0.3749999999999965028, 0.4999999999999821809, 1.000000000000000000 ),
 .UNSPECIFIED. ) ;
#52671=CARTESIAN_POINT ( 'NONE',  ( -3.805396659119999914, 1495.647976226690162, 219.6495707272989932 ) ) ;
#52674=ORIENTED_EDGE ( 'NONE', *, *, #4323, .T. ) ;
#52680=( BOUNDED_CURVE ( )  B_SPLINE_CURVE ( 3, ( #104944, #80299, #3066, #11444 ),
 .UNSPECIFIED., .F., .T. ) 
 B_SPLINE_CURVE_WITH_KNOTS ( ( 4, 4 ),
 ( 1.028502516659682176, 2.113090281714570029 ),
 .UNSPECIFIED. ) 
 CURVE ( )  GEOMETRIC_REPRESENTATION_ITEM ( )  RATIONAL_B_SPLINE_CURVE ( ( 1.000000000000000000, 0.9043513721624834023, 0.9043513721624834023, 1.000000000000000000 ) ) 
 REPRESENTATION_ITEM ( '' )  );
#52686=CARTESIAN_POINT ( 'NONE',  ( -5.177093926210000419, 1391.906305342289897, 214.5223142673890209 ) ) ;
#52687=B_SPLINE_CURVE_WITH_KNOTS ( 'NONE', 3,
 ( #43438, #16534, #102221, #85407, #94359, #17639, #26614, #35020, #9278, #77589, #896, #60810, #18207, #86527, #43990, #78125, #35571, #61366, #36140, #88748, #10937, #19868, #71439, #63572, #87085, #87650, #28282 ),
 .UNSPECIFIED., .F., .F.,
 ( 4, 2, 2, 2, 1, 1, 1, 1, 1, 2, 2, 2, 2, 2, 2, 4 ),
 ( 0.000000000000000000, 0.2500000000017412183, 0.3750000000026034730, 0.4375000000030318525, 0.4687500000032479575, 0.4843750000033510972, 0.4921875000034075520, 0.4960937500034376946, 0.4980468750034528491, 0.4990234375034622305, 0.5000000000034716674, 0.6250000000026062486, 0.6875000000021718183, 0.7500000000017372770, 0.8750000000008686385, 1.000000000000000000 ),
 .UNSPECIFIED. ) ;
#52689=ORIENTED_EDGE ( 'NONE', *, *, #11153, .F. ) ;
#52691=CARTESIAN_POINT ( 'NONE',  ( 9.668880095928939156, 1462.163648629059935, 207.9796277090590024 ) ) ;
#52695=CARTESIAN_POINT ( 'NONE',  ( 9.430278060304900123, 1452.926932606559831, 211.6524132603890109 ) ) ;
#52696=CARTESIAN_POINT ( 'NONE',  ( 9.237784538809998836, 1425.317541609140108, 195.2081299371990042 ) ) ;
#52706=CARTESIAN_POINT ( 'NONE',  ( 4.329341215434487466, 1515.068899831254157, 212.0800836860477432 ) ) ;
#52716=CARTESIAN_POINT ( 'NONE',  ( -6.461178696532821064, 1508.551704651539922, 219.4694278874889903 ) ) ;
#52722=CARTESIAN_POINT ( 'NONE',  ( -4.794937653589999904, 1475.260169187289875, 199.8527927719790114 ) ) ;
#52723=CARTESIAN_POINT ( 'NONE',  ( -2.298880634834130188, 1421.940747973940006, 193.2957375577259995 ) ) ;
#52727=CARTESIAN_POINT ( 'NONE',  ( 11.01815538213319989, 1470.097469558069861, 206.4145453267350092 ) ) ;
#52736=CARTESIAN_POINT ( 'NONE',  ( 3.648449339570000394, 1506.945873062889859, 220.2261837244989806 ) ) ;
#52737=CARTESIAN_POINT ( 'NONE',  ( -14.47535368149999968, 1416.023439710309958, 214.4146907853689754 ) ) ;
#52738=CARTESIAN_POINT ( 'NONE',  ( 1.768532852308550174, 1515.064792882589927, 204.7923971856590128 ) ) ;
#52740=CARTESIAN_POINT ( 'NONE',  ( -15.88354217481895425, 1415.957443832936178, 209.7362470719081102 ) ) ;
#52749=EDGE_CURVE ( 'NONE', #26525, #41801, #90634, .T. ) ;
#52750=CARTESIAN_POINT ( 'NONE',  ( -10.67770939150419984, 1481.275619385470236, 208.2056862302819980 ) ) ;
#52759=CARTESIAN_POINT ( 'NONE',  ( -15.62861149524349891, 1418.244676918490086, 203.0179538217920197 ) ) ;
#52760=CARTESIAN_POINT ( 'NONE',  ( 17.33107428800062522, 1477.785820313406475, 220.5162645747961108 ) ) ;
#52762=CARTESIAN_POINT ( 'NONE',  ( -15.57409121169999899, 1415.640300991889944, 209.4226310109950191 ) ) ;
#52766=CARTESIAN_POINT ( 'NONE',  ( 1.467075754108839503, 1432.098771012052794, 200.8278867525325495 ) ) ;
#52767=EDGE_LOOP ( 'NONE', ( #50473, #5999, #24569, #39587 ) ) ;
#52771=CARTESIAN_POINT ( 'NONE',  ( -13.12541650777430036, 1507.970701092599938, 209.3483060399670137 ) ) ;
#52776=VECTOR ( 'NONE', #91844, 1000.000000000000000 ) ;
#52791=CARTESIAN_POINT ( 'NONE',  ( 4.297912049859999861, 1484.403092702089907, 220.1616355836989953 ) ) ;
#52792=CARTESIAN_POINT ( 'NONE',  ( 4.582279963310000426, 1422.267990882979802, 194.3935423355989940 ) ) ;
#52797=CARTESIAN_POINT ( 'NONE',  ( -2.613520083516720049, 1448.739697532430000, 188.5780410999010144 ) ) ;
#52803=CARTESIAN_POINT ( 'NONE',  ( 9.816185060832909315, 1435.693060327849935, 209.5517428691599946 ) ) ;
#52804=CARTESIAN_POINT ( 'NONE',  ( -10.46250751100000009, 1491.356802620389999, 212.5409670600390086 ) ) ;
#52812=CARTESIAN_POINT ( 'NONE',  ( 9.849121764593530060, 1503.262452723809929, 216.7244655636139896 ) ) ;
#52816=ORIENTED_EDGE ( 'NONE', *, *, #19123, .T. ) ;
#52823=CARTESIAN_POINT ( 'NONE',  ( -0.7920961534389989733, 1444.349757015490013, 199.4831802694889973 ) ) ;
#52826=EDGE_CURVE ( 'NONE', #42035, #12639, #13074, .T. ) ;
#52828=CARTESIAN_POINT ( 'NONE',  ( 1.159955629579999981, 1469.039094341789905, 219.1201689042090095 ) ) ;
#52834=CARTESIAN_POINT ( 'NONE',  ( -9.970572234719458748, 1422.681531195490152, 209.6984921149189915 ) ) ;
#52835=( BOUNDED_CURVE ( )  B_SPLINE_CURVE ( 3, ( #46548, #38119, #55494, #56034 ),
 .UNSPECIFIED., .F., .T. ) 
 B_SPLINE_CURVE_WITH_KNOTS ( ( 4, 4 ),
 ( 1.010406472820884138, 2.131186328586304857 ),
 .UNSPECIFIED. ) 
 CURVE ( )  GEOMETRIC_REPRESENTATION_ITEM ( )  RATIONAL_B_SPLINE_CURVE ( ( 1.000000000000000000, 0.8980319481995078235, 0.8980319481995078235, 1.000000000000000000 ) ) 
 REPRESENTATION_ITEM ( '' )  );
#52839=CARTESIAN_POINT ( 'NONE',  ( 1.241329981776470026, 1432.830262692500128, 200.7618047978820073 ) ) ;
#52843=ORIENTED_EDGE ( 'NONE', *, *, #10589, .T. ) ;
#52847=CARTESIAN_POINT ( 'NONE',  ( -3.677613769069999778E-16, 1378.413060387289988, 209.1218459616989946 ) ) ;
#52848=CARTESIAN_POINT ( 'NONE',  ( 10.10905482369999930, 1461.386512506689996, 208.4426341976229935 ) ) ;
#52853=CARTESIAN_POINT ( 'NONE',  ( 8.631780704876279131, 1438.018275767699834, 210.0183142686710198 ) ) ;
#52867=CARTESIAN_POINT ( 'NONE',  ( -3.389245491280000078, 1507.871109296990198, 220.9917548405990146 ) ) ;
#52869=CARTESIAN_POINT ( 'NONE',  ( 1.247882269740000050, 1499.086923094689837, 200.6750383293390030 ) ) ;
#52877=CARTESIAN_POINT ( 'NONE',  ( -11.78126758929439966, 1482.336360767919814, 207.4553989261059996 ) ) ;
#52882=CARTESIAN_POINT ( 'NONE',  ( 10.57855775040389901, 1491.027229822649815, 212.1174194973030183 ) ) ;
#52903=LINE ( 'NONE', #106051, #5549 ) ;
#52904=CARTESIAN_POINT ( 'NONE',  ( 1.304943139099999927, 1431.126433557689779, 200.1249384120889943 ) ) ;
#52906=CARTESIAN_POINT ( 'NONE',  ( 3.561968680879999738, 1506.511571059590324, 220.3681565264990070 ) ) ;
#52912=CARTESIAN_POINT ( 'NONE',  ( 4.589161282302300471, 1466.737739933080093, 198.9391871293819918 ) ) ;
#52914=CARTESIAN_POINT ( 'NONE',  ( 11.49580466759999986, 1502.679721642689856, 209.6813715333399841 ) ) ;
#52916=CARTESIAN_POINT ( 'NONE',  ( 9.345713659299999421, 1422.635913846680069, 212.8840062826189978 ) ) ;
#52919=CARTESIAN_POINT ( 'NONE',  ( 12.49401126939999962, 1451.800774058590150, 193.6953293048989906 ) ) ;
#52923=ORIENTED_EDGE ( 'NONE', *, *, #89948, .F. ) ;
#52926=CARTESIAN_POINT ( 'NONE',  ( -2.782618081592460157, 1489.016425230830009, 216.8593202305619911 ) ) ;
#52932=CARTESIAN_POINT ( 'NONE',  ( 1.388898171294610018, 1456.630141039370073, 219.6509599159400068 ) ) ;
#52933=CARTESIAN_POINT ( 'NONE',  ( -0.2329163981069990175, 1457.935017252390253, 202.2546241818889996 ) ) ;
#52934=CARTESIAN_POINT ( 'NONE',  ( -9.466658637189999226, 1449.313965536590104, 207.5701179724289887 ) ) ;
#52936=CARTESIAN_POINT ( 'NONE',  ( 7.424089790420000057, 1424.882440436209890, 212.3756834930689763 ) ) ;
#52937=CARTESIAN_POINT ( 'NONE',  ( -8.229021304010000648, 1439.448076410589920, 228.6152058856989697 ) ) ;
#52943=EDGE_LOOP ( 'NONE', ( #50248, #97055, #15597, #9682 ) ) ;
#52953=CARTESIAN_POINT ( 'NONE',  ( -1.289615935422919968, 1475.477284819069837, 197.7490727346969948 ) ) ;
#52955=B_SPLINE_SURFACE_WITH_KNOTS ( 'NONE', 5, 5, ( 
 ( #44078, #26702, #26139, #60899, #18843, #60328 ),
 ( #78216, #1528, #69851, #53039, #87175, #10463 ),
 ( #100332, #53642, #94491, #95065, #78821, #104567 ),
 ( #27861, #3242, #87217, #105126, #69334, #60936 ),
 ( #71005, #36258, #2135, #26747, #95614, #17763 ),
 ( #18880, #43564, #37369, #45793, #70447, #2691 ) ),
 .UNSPECIFIED., .F., .F., .F.,
 ( 6, 6 ),
 ( 6, 6 ),
 ( 7.548656686110299496, 12.57640183248079957 ),
 ( 0.000000000000000000, 0.5000176499936439534 ),
 .UNSPECIFIED. ) ;
#52968=CARTESIAN_POINT ( 'NONE',  ( -4.336802270429999773, 1455.494076152190019, 200.7328417250689938 ) ) ;
#52988=CARTESIAN_POINT ( 'NONE',  ( 3.181172983203653715, 1442.605928314588482, 217.4126502573513164 ) ) ;
#52989=CARTESIAN_POINT ( 'NONE',  ( -9.359048371426943902, 1440.623807415093552, 205.4859881516416635 ) ) ;
#52992=B_SPLINE_CURVE_WITH_KNOTS ( 'NONE', 3,
 ( #89257, #22014, #91465, #38293, #63543, #64633, #65175, #48376, #73582, #13623, #107157, #23137, #39955, #106064, #98754, #13075, #29344, #80315, #47262, #47811, #4698, #20931, #74129, #81946, #73018, #65724, #30449, #71953 ),
 .UNSPECIFIED., .F., .F.,
 ( 4, 3, 3, 3, 3, 3, 3, 3, 3, 4 ),
 ( -7.748415063910000455, -7.637761903620339687, -7.426814887477540594, -7.105214711045070075, -6.860935728577989501, -6.655162690954419702, -5.895137996252290513, -5.135113301550160436, -4.241455848545670371, -3.182527802580000120 ),
 .UNSPECIFIED. ) ;
#52996=CARTESIAN_POINT ( 'NONE',  ( 2.801469573665160251, 1486.711816252329754, 216.6332114747600031 ) ) ;
#52997=CARTESIAN_POINT ( 'NONE',  ( -22.15968191147809918, 1485.573429526870086, 217.2083819532319922 ) ) ;
#52998=( BOUNDED_CURVE ( )  B_SPLINE_CURVE ( 3, ( #97861, #90568, #82169, #21136 ),
 .UNSPECIFIED., .F., .F. ) 
 B_SPLINE_CURVE_WITH_KNOTS ( ( 4, 4 ),
 ( 4.137179913343402404, 5.287886354397532074 ),
 .UNSPECIFIED. ) 
 CURVE ( )  GEOMETRIC_REPRESENTATION_ITEM ( )  RATIONAL_B_SPLINE_CURVE ( ( 1.000000000000000000, 0.8926667709749616098, 0.8926667709749616098, 1.000000000000000000 ) ) 
 REPRESENTATION_ITEM ( '' )  );
#53000=ORIENTED_EDGE ( 'NONE', *, *, #2530, .F. ) ;
#53006=CARTESIAN_POINT ( 'NONE',  ( -3.179433604570000238, 1429.659768554990023, 201.3028921480589872 ) ) ;
#53012=CARTESIAN_POINT ( 'NONE',  ( 2.330134126090000368, 1515.064792882589927, 213.4512947377390049 ) ) ;
#53018=ORIENTED_EDGE ( 'NONE', *, *, #100665, .T. ) ;
#53021=ORIENTED_EDGE ( 'NONE', *, *, #109801, .T. ) ;
#53023=CARTESIAN_POINT ( 'NONE',  ( 1.959285310369999866, 1474.800623465989929, 220.3715843581990157 ) ) ;
#53025=CARTESIAN_POINT ( 'NONE',  ( 2.931649531350000171, 1441.868998527789927, 217.8578126236290302 ) ) ;
#53028=EDGE_CURVE ( 'NONE', #98016, #5707, #15848, .T. ) ;
#53029=LINE ( 'NONE', #11565, #37772 ) ;
#53032=CARTESIAN_POINT ( 'NONE',  ( -3.100416393482220201, 1464.813281825060130, 198.5539054533549859 ) ) ;
#53034=CARTESIAN_POINT ( 'NONE',  ( 7.898231641030000638, 1488.783166887790003, 199.9435678271790096 ) ) ;
#53039=CARTESIAN_POINT ( 'NONE',  ( -4.556906923311959901, 1508.729448375579977, 212.2592363442360011 ) ) ;
#53044=CARTESIAN_POINT ( 'NONE',  ( -11.27974060871780004, 1470.421108576400002, 210.7070861076940105 ) ) ;
#53045=CARTESIAN_POINT ( 'NONE',  ( -9.827124267810660285, 1490.452494543219927, 214.0432529463710125 ) ) ;
#53047=CARTESIAN_POINT ( 'NONE',  ( -3.005245951399999615, 1450.300005596989877, 188.5532306447990152 ) ) ;
#53052=CARTESIAN_POINT ( 'NONE',  ( 10.54136348144620072, 1452.203475739079749, 208.5677207636399828 ) ) ;
#53058=VERTEX_POINT ( 'NONE', #22796 ) ;
#53061=CARTESIAN_POINT ( 'NONE',  ( -8.123537375139999739, 1500.423749094890127, 210.2681864885289826 ) ) ;
#53072=CARTESIAN_POINT ( 'NONE',  ( -1.842962231260000028, 1515.064792882589927, 213.4512947377390049 ) ) ;
#53074=CARTESIAN_POINT ( 'NONE',  ( -11.39291980906549995, 1423.225053426399882, 204.2085665321329770 ) ) ;
#53075=EDGE_CURVE ( 'NONE', #43039, #12262, #7385, .T. ) ;
#53077=CARTESIAN_POINT ( 'NONE',  ( 1.762362329279999917, 1472.996463562990130, 219.1807010226990258 ) ) ;
#53080=CARTESIAN_POINT ( 'NONE',  ( 10.67658260354509991, 1477.918112985820017, 229.9062897255660118 ) ) ;
#53082=CARTESIAN_POINT ( 'NONE',  ( -1.693092260590000064, 1443.235800063490160, 218.9922120262189935 ) ) ;
#53089=CARTESIAN_POINT ( 'NONE',  ( -9.007784044950000180, 1459.287865364090067, 212.7101983019389877 ) ) ;
#53094=CARTESIAN_POINT ( 'NONE',  ( -8.833145283479998611, 1423.402459408220011, 209.4147327117469786 ) ) ;
#53100=CARTESIAN_POINT ( 'NONE',  ( 7.158490357027510242, 1426.589113566749802, 213.0788671595350081 ) ) ;
#53103=VERTEX_POINT ( 'NONE', #22245 ) ;
#53110=CARTESIAN_POINT ( 'NONE',  ( 5.626793905219999559, 1472.332539098689949, 217.6352975007490045 ) ) ;
#53111=CARTESIAN_POINT ( 'NONE',  ( -8.768286811978629913, 1439.919956341389934, 206.3771518704159860 ) ) ;
#53116=CARTESIAN_POINT ( 'NONE',  ( 8.678482696542719310, 1436.053160561679988, 208.0948695542589917 ) ) ;
#53118=VERTEX_POINT ( 'NONE', #100621 ) ;
#53131=VERTEX_POINT ( 'NONE', #38520 ) ;
#53132=CARTESIAN_POINT ( 'NONE',  ( -0.05714988119310079884, 1445.012840177589851, 215.4090402065690171 ) ) ;
#53135=ORIENTED_EDGE ( 'NONE', *, *, #108035, .F. ) ;
#53136=CARTESIAN_POINT ( 'NONE',  ( 4.556906923312060265, 1508.729448375579977, 205.9844555791620166 ) ) ;
#53144=CARTESIAN_POINT ( 'NONE',  ( -3.829620154745601468, 1515.551704408389924, 205.9132087081559064 ) ) ;
#53149=CARTESIAN_POINT ( 'NONE',  ( 7.069913306463050162, 1426.666554464499995, 213.2414280066960259 ) ) ;
#53158=CARTESIAN_POINT ( 'NONE',  ( -10.79825500028279883, 1462.862626845389968, 206.7546097349500087 ) ) ;
#53163=CARTESIAN_POINT ( 'NONE',  ( -10.92059295481699976, 1461.979801184900225, 210.5672364399190144 ) ) ;
#53164=CARTESIAN_POINT ( 'NONE',  ( 14.43086985023570001, 1426.807458679940282, 195.4949786040619983 ) ) ;
#53166=CARTESIAN_POINT ( 'NONE',  ( 9.717826194827521746, 1463.678457587320054, 210.3770332206470073 ) ) ;
#53173=CARTESIAN_POINT ( 'NONE',  ( -15.79259793311170057, 1420.293458116122565, 210.0948661461389690 ) ) ;
#53176=CARTESIAN_POINT ( 'NONE',  ( -11.77905465891600123, 1483.168200228759815, 228.2502074522770101 ) ) ;
#53179=CARTESIAN_POINT ( 'NONE',  ( 8.930242950181860095, 1451.533433059749996, 211.6080513519700048 ) ) ;
#53180=CARTESIAN_POINT ( 'NONE',  ( 3.346695691219999880, 1443.005063871489938, 217.3642547372890022 ) ) ;
#53188=CARTESIAN_POINT ( 'NONE',  ( -2.158775737652639748, 1508.551704408389924, 220.0625486152149790 ) ) ;
#53191=CARTESIAN_POINT ( 'NONE',  ( 6.852456351503855458, 1447.063841582483519, 203.1720596810001780 ) ) ;
#53194=CARTESIAN_POINT ( 'NONE',  ( 0.2196276506829989983, 1429.899695672290136, 217.4576539075590063 ) ) ;
#53196=CARTESIAN_POINT ( 'NONE',  ( -10.43378839784119982, 1471.950490389920105, 207.0189331983069962 ) ) ;
#53204=CARTESIAN_POINT ( 'NONE',  ( 11.59720850580749918, 1491.204161894499975, 206.7870309651650018 ) ) ;
#53209=EDGE_LOOP ( 'NONE', ( #60153, #56219, #99539, #38639 ) ) ;
#53213=B_SPLINE_CURVE_WITH_KNOTS ( 'NONE', 5,
 ( #46285, #80413, #72568, #99944, #39508, #100507, #38392, #108364, #4787 ),
 .UNSPECIFIED., .F., .F.,
 ( 6, 3, 6 ),
 ( 0.000000000000000000, 0.4797001321658070916, 1.000000000000000000 ),
 .UNSPECIFIED. ) ;
#53216=CARTESIAN_POINT ( 'NONE',  ( 12.37353479079889951, 1427.152528082410072, 207.0190610342110062 ) ) ;
#53227=LINE ( 'NONE', #59974, #90585 ) ;
#53229=CARTESIAN_POINT ( 'NONE',  ( -1.228179860600000062, 1495.213118903489885, 220.2649180232990034 ) ) ;
#53238=EDGE_CURVE ( 'NONE', #15989, #107938, #36060, .T. ) ;
#53244=CARTESIAN_POINT ( 'NONE',  ( 3.012478497202149885, 1508.551704408389924, 214.0547362871380130 ) ) ;
#53248=CARTESIAN_POINT ( 'NONE',  ( 10.88300501365269923, 1460.705383129390157, 207.9797520299849793 ) ) ;
#53251=ORIENTED_EDGE ( 'NONE', *, *, #106862, .F. ) ;
#53253=CARTESIAN_POINT ( 'NONE',  ( 9.772779914185960592, 1453.284091914029887, 211.9285179305149995 ) ) ;
#53254=CARTESIAN_POINT ( 'NONE',  ( 9.147586507279999779, 1424.572281473970179, 196.5102056844989704 ) ) ;
#53255=ORIENTED_EDGE ( 'NONE', *, *, #2239, .T. ) ;
#53257=CARTESIAN_POINT ( 'NONE',  ( -6.910430994591643561, 1419.227950353617871, 195.3558243408897681 ) ) ;
#53258=DIRECTION ( 'NONE',  ( -0.8907681516580484571, 1.273087901431153894E-31, 0.4544580288560254311 ) ) ;
#53263=CARTESIAN_POINT ( 'NONE',  ( 9.394917065999061734, 1451.852087569300011, 209.9058690040849910 ) ) ;
#53264=CARTESIAN_POINT ( 'NONE',  ( -4.247299066680000124, 1502.738124400289962, 230.1067396463990065 ) ) ;
#53269=ORIENTED_EDGE ( 'NONE', *, *, #7195, .T. ) ;
#53276=CARTESIAN_POINT ( 'NONE',  ( -10.54306353004690067, 1469.936069848170064, 213.3750816242119868 ) ) ;
#53281=CARTESIAN_POINT ( 'NONE',  ( 10.03804068110000003, 1493.022037044190029, 214.8448302025189776 ) ) ;
#53283=CARTESIAN_POINT ( 'NONE',  ( 9.331170596321376465, 1425.274930616336405, 195.5633789865317453 ) ) ;
#53284=CARTESIAN_POINT ( 'NONE',  ( -17.68441402020000197, 1504.382480553090090, 209.0725129034710221 ) ) ;
#53285=CARTESIAN_POINT ( 'NONE',  ( 11.13973213087689906, 1470.272412021129867, 206.9146623043149873 ) ) ;
#53286=CARTESIAN_POINT ( 'NONE',  ( -3.249999999999999556, 1524.551704408390151, 209.1218459616989946 ) ) ;
#53290=ORIENTED_EDGE ( 'NONE', *, *, #6388, .T. ) ;
#53294=CARTESIAN_POINT ( 'NONE',  ( 3.838475640130000421, 1505.530984303090008, 221.3004008607989874 ) ) ;
#53296=CARTESIAN_POINT ( 'NONE',  ( 1.201530806705199961, 1515.093215458460008, 204.7931414570770130 ) ) ;
#53297=VERTEX_POINT ( 'NONE', #9197 ) ;
#53298=CARTESIAN_POINT ( 'NONE',  ( -15.77498267344473071, 1415.804408449163247, 209.6953390818695198 ) ) ;
#53299=CARTESIAN_POINT ( 'NONE',  ( -10.18374426391977039, 1473.001081400295334, 208.1334165208762386 ) ) ;
#53300=CARTESIAN_POINT ( 'NONE',  ( -15.94270011119999708, 1416.079343365249997, 209.7066342856829806 ) ) ;
#53301=CARTESIAN_POINT ( 'NONE',  ( -6.375523666339999451, 1460.280735373489961, 210.0338255622669976 ) ) ;
#53308=CARTESIAN_POINT ( 'NONE',  ( 9.982819585849640021, 1469.474122878060143, 210.3108196173600106 ) ) ;
#53319=CARTESIAN_POINT ( 'NONE',  ( -11.38916143032739825, 1500.505134839040011, 209.9622123043970134 ) ) ;
#53322=CARTESIAN_POINT ( 'NONE',  ( -15.88926427640000050, 1416.064503262980224, 209.5444336918569945 ) ) ;
#53333=CARTESIAN_POINT ( 'NONE',  ( -11.82991541994420004, 1481.593101321090217, 209.9800737738590044 ) ) ;
#53343=CARTESIAN_POINT ( 'NONE',  ( 5.161277877375379575, 1424.205378946189967, 193.2953230041809718 ) ) ;
#53344=CARTESIAN_POINT ( 'NONE',  ( 4.329448786299999519, 1515.064792490889886, 207.2788827064790098 ) ) ;
#53351=CARTESIAN_POINT ( 'NONE',  ( 10.50536461352409923, 1481.125266294730181, 208.0189701215730054 ) ) ;
#53354=CARTESIAN_POINT ( 'NONE',  ( 7.755360837189519962, 1459.738753866829938, 228.9106046784149839 ) ) ;
#53360=CARTESIAN_POINT ( 'NONE',  ( -10.97106033540000070, 1491.549773342590015, 210.1503302054390190 ) ) ;
#53368=CARTESIAN_POINT ( 'NONE',  ( -9.200421138165051360, 1422.937291722789951, 210.7384568321920142 ) ) ;
#53376=CARTESIAN_POINT ( 'NONE',  ( 11.01047161400000007, 1501.676453312990134, 205.9410319520989674 ) ) ;
#53379=CARTESIAN_POINT ( 'NONE',  ( 2.601659696316710235, 1468.435074765370018, 215.8528558269860298 ) ) ;
#53385=CARTESIAN_POINT ( 'NONE',  ( -4.646147438016499542, 1378.399971910029990, 214.5514622210689879 ) ) ;
#53387=VERTEX_POINT ( 'NONE', #78605 ) ;
#53389=CARTESIAN_POINT ( 'NONE',  ( 0.8791306092667371397, 1432.688050419320007, 200.7222455119930089 ) ) ;
#53392=ORIENTED_EDGE ( 'NONE', *, *, #21579, .T. ) ;
#53397=CARTESIAN_POINT ( 'NONE',  ( 1.665089994623440095, 1465.819159950360017, 198.2247081585720139 ) ) ;
#53398=CARTESIAN_POINT ( 'NONE',  ( -18.63793804202000004, 1508.544021955199923, 210.2772651711879917 ) ) ;
#53401=CARTESIAN_POINT ( 'NONE',  ( 8.602499828956750250, 1437.170389814990131, 208.2906584274039972 ) ) ;
#53404=ORIENTED_EDGE ( 'NONE', *, *, #32949, .F. ) ;
#53417=CARTESIAN_POINT ( 'NONE',  ( -6.569523906889999765, 1508.426336951290068, 219.8379881403990055 ) ) ;
#53419=CARTESIAN_POINT ( 'NONE',  ( 5.532282641970000192, 1438.101548169890066, 209.4569669644060355 ) ) ;
#53439=CARTESIAN_POINT ( 'NONE',  ( 5.161034791280000533, 1485.814572579490005, 218.5690567784690188 ) ) ;
#53456=CARTESIAN_POINT ( 'NONE',  ( 3.401546208480000111, 1468.225227913490016, 218.5224274127089927 ) ) ;
#53460=CARTESIAN_POINT ( 'NONE',  ( 1.038038148820000117, 1431.814275748890168, 200.6412883882290146 ) ) ;
#53462=CARTESIAN_POINT ( 'NONE',  ( -0.2520374592430009719, 1508.165742498189957, 220.8827497849989925 ) ) ;
#53468=CARTESIAN_POINT ( 'NONE',  ( 3.193605244039539937, 1466.133281249020001, 198.9725477671120188 ) ) ;
#53470=CARTESIAN_POINT ( 'NONE',  ( 6.263982046360000666, 1500.597020525990047, 203.1398415524789982 ) ) ;
#53484=CARTESIAN_POINT ( 'NONE',  ( -11.41402561306639996, 1500.969831351809944, 208.5831151434670119 ) ) ;
#53485=CARTESIAN_POINT ( 'NONE',  ( -13.58855293548379883, 1508.389930495940007, 209.7948077685939836 ) ) ;
#53488=CARTESIAN_POINT ( 'NONE',  ( -9.951253231297551238, 1438.974309065549960, 209.5953120751400149 ) ) ;
#53489=LINE ( 'NONE', #70308, #30700 ) ;
#53490=CARTESIAN_POINT ( 'NONE',  ( -9.231470400260000986, 1449.703074994190047, 207.7616675809790081 ) ) ;
#53493=CARTESIAN_POINT ( 'NONE',  ( 7.901745564190000515, 1424.856359000810016, 211.6778634635190031 ) ) ;
#53501=CARTESIAN_POINT ( 'NONE',  ( 5.741164914759999682, 1453.932054823290173, 216.5784219893689908 ) ) ;
#53503=ORIENTED_EDGE ( 'NONE', *, *, #76021, .T. ) ;
#53511=CARTESIAN_POINT ( 'NONE',  ( -1.625910793146879918, 1463.710942619060006, 199.4574199946389683 ) ) ;
#53521=EDGE_LOOP ( 'NONE', ( #42663, #51429, #90162, #73201 ) ) ;
#53524=CARTESIAN_POINT ( 'NONE',  ( -7.799999999999999822, 1412.913060387329779, 209.1218459616989946 ) ) ;
#53532=CARTESIAN_POINT ( 'NONE',  ( 7.944350852719999523, 1425.480812533560083, 211.5441705370589887 ) ) ;
#53536=EDGE_CURVE ( 'NONE', #82244, #777, #101126, .T. ) ;
#53539=CARTESIAN_POINT ( 'NONE',  ( 9.332531155627359354, 1462.059220043490086, 206.3768343672439869 ) ) ;
#53561=ADVANCED_FACE ( 'NONE', ( #673 ), #28438, .F. ) ;
#53576=CARTESIAN_POINT ( 'NONE',  ( 10.94950459731960102, 1470.725626738129904, 208.8250202921669825 ) ) ;
#53580=VERTEX_POINT ( 'NONE', #64980 ) ;
#53586=LINE ( 'NONE', #44624, #14575 ) ;
#53598=ORIENTED_EDGE ( 'NONE', *, *, #57715, .F. ) ;
#53603=CARTESIAN_POINT ( 'NONE',  ( -4.878045583760000525, 1484.465894326689977, 199.1376824933889793 ) ) ;
#53610=EDGE_CURVE ( 'NONE', #26627, #40693, #109896, .T. ) ;
#53611=CARTESIAN_POINT ( 'NONE',  ( -9.051675461232269626, 1490.533562533649956, 215.4358965029069850 ) ) ;
#53612=CARTESIAN_POINT ( 'NONE',  ( 5.076294927523219869, 1469.790098474529941, 187.8425670808459813 ) ) ;
#53617=CARTESIAN_POINT ( 'NONE',  ( 10.47377178300940059, 1451.946270717840207, 207.9508650615720171 ) ) ;
#53630=CARTESIAN_POINT ( 'NONE',  ( -3.613876939720699788, 1495.512358501490098, 197.3347655600630333 ) ) ;
#53638=CARTESIAN_POINT ( 'NONE',  ( -12.04274590166719960, 1422.870584108250114, 204.0708875435599907 ) ) ;
#53642=CARTESIAN_POINT ( 'NONE',  ( -4.544860949933259953, 1508.551704410290085, 213.0837902323600019 ) ) ;
#53643=CARTESIAN_POINT ( 'NONE',  ( -5.294782532323449864, 1489.664752326729968, 185.8873045459189939 ) ) ;
#53649=CARTESIAN_POINT ( 'NONE',  ( 4.329068131566989663, 1515.079329108569937, 210.5320604527299793 ) ) ;
#53653=CARTESIAN_POINT ( 'NONE',  ( -9.311658524700000328, 1460.574498714589936, 213.2399738195690304 ) ) ;
#53660=EDGE_LOOP ( 'NONE', ( #14360, #67847, #47049, #24017 ) ) ;
#53663=CARTESIAN_POINT ( 'NONE',  ( -8.928049104570000338, 1472.922707491090023, 201.8104512964389983 ) ) ;
#53673=CARTESIAN_POINT ( 'NONE',  ( 1.761008324855960039, 1487.196696357248584, 219.8036233159708388 ) ) ;
#53674=CARTESIAN_POINT ( 'NONE',  ( -17.13701823974819760, 1508.493192689929856, 212.9882043946190322 ) ) ;
#53676=CARTESIAN_POINT ( 'NONE',  ( 5.586191088959999718, 1473.645535070089863, 218.5932301067289814 ) ) ;
#53678=CARTESIAN_POINT ( 'NONE',  ( -8.248738497215569510, 1439.101388822510216, 206.2653402195520016 ) ) ;
#53683=CARTESIAN_POINT ( 'NONE',  ( 8.496650132276949208, 1436.860065467399863, 207.6057550149429858 ) ) ;
#53684=EDGE_CURVE ( 'NONE', #86033, #67895, #41226, .T. ) ;
#53686=ORIENTED_EDGE ( 'NONE', *, *, #17166, .T. ) ;
#53687=ORIENTED_EDGE ( 'NONE', *, *, #633, .F. ) ;
#53689=CARTESIAN_POINT ( 'NONE',  ( 0.03042691127746960031, 1467.462897955010249, 220.2118647206560240 ) ) ;
#53693=B_SPLINE_CURVE_WITH_KNOTS ( 'NONE', 3,
 ( #5230, #22544, #81927, #106048, #90882, #47791, #13054, #38273, #80296, #39383, #73560, #72457, #38821, #29325, #37735, #74107, #12533, #65703, #107693, #65153, #14169, #55662 ),
 .UNSPECIFIED., .F., .F.,
 ( 4, 2, 1, 1, 2, 2, 2, 2, 1, 1, 2, 2, 4 ),
 ( 0.000000000000000000, 0.1249999999998943900, 0.1874999999998415712, 0.2187499999998157307, 0.2343749999997886413, 0.2499999999997615241, 0.4999999999997214450, 0.6249999999997183364, 0.6874999999997178923, 0.7187499999997348787, 0.7343749999997226663, 0.7499999999997104538, 1.000000000000000000 ),
 .UNSPECIFIED. ) ;
#53701=CARTESIAN_POINT ( 'NONE',  ( 2.306961389589999634, 1443.485925623590219, 214.8977830156290167 ) ) ;
#53737=CARTESIAN_POINT ( 'NONE',  ( 2.788373426233030195, 1425.940953389439983, 188.8017441523220157 ) ) ;
#53749=B_SPLINE_CURVE_WITH_KNOTS ( 'NONE', 5,
 ( #24962, #85428, #100586, #42906, #59172, #93290 ),
 .UNSPECIFIED., .F., .F.,
 ( 6, 6 ),
 ( -1.999999843773010211, -1.697648102094717615E-07 ),
 .UNSPECIFIED. ) ;
#53750=CARTESIAN_POINT ( 'NONE',  ( -8.881784197000000993E-16, 1392.213060387289943, 209.1218459616989946 ) ) ;
#53751=CARTESIAN_POINT ( 'NONE',  ( 7.069913306463050162, 1426.666554464499995, 213.2414280066960259 ) ) ;
#53753=CARTESIAN_POINT ( 'NONE',  ( -4.833436910021659649, 1508.551704408290107, 205.8972885837780211 ) ) ;
#53763=CARTESIAN_POINT ( 'NONE',  ( -3.030734320792309422, 1508.551704408389924, 219.9920206123570097 ) ) ;
#53764=VERTEX_POINT ( 'NONE', #23779 ) ;
#53769=CARTESIAN_POINT ( 'NONE',  ( 0.7324858582209989866, 1431.361405734790196, 218.1975961472689960 ) ) ;
#53770=CARTESIAN_POINT ( 'NONE',  ( -15.59561454159999982, 1421.682133015659929, 211.4342267833790174 ) ) ;
#53775=CARTESIAN_POINT ( 'NONE',  ( 10.82765054261410143, 1427.328577260649809, 209.3704925542409967 ) ) ;
#53776=ORIENTED_EDGE ( 'NONE', *, *, #1108, .F. ) ;
#53777=CARTESIAN_POINT ( 'NONE',  ( 12.22822919944690057, 1491.662241031820031, 207.6548834463269770 ) ) ;
#53778=CARTESIAN_POINT ( 'NONE',  ( -1.815594625336599988, 1438.273795259480039, 227.6128410382069944 ) ) ;
#53783=CARTESIAN_POINT ( 'NONE',  ( 0.8769335050712490087, 1496.770081789519963, 196.7770485174839905 ) ) ;
#53789=CARTESIAN_POINT ( 'NONE',  ( 12.65728676410210163, 1420.119835224449844, 200.3472210950669989 ) ) ;
#53792=DIRECTION ( 'NONE',  ( 0.1484981130679619565, -0.4511266441233499069, 0.8800187846729518037 ) ) ;
#53808=CARTESIAN_POINT ( 'NONE',  ( 2.875920673130000438, 1485.134067338089835, 220.2246146252990115 ) ) ;
#53810=CARTESIAN_POINT ( 'NONE',  ( 20.12205423489999845, 1473.683723071389977, 208.1594102018889885 ) ) ;
#53817=ORIENTED_EDGE ( 'NONE', *, *, #90299, .T. ) ;
#53818=CARTESIAN_POINT ( 'NONE',  ( 9.020493505376890653, 1451.396381989520023, 211.2518042107480198 ) ) ;
#53819=CARTESIAN_POINT ( 'NONE',  ( 5.161277909749999893, 1424.205379146819951, 193.2953227953989881 ) ) ;
#53820=EDGE_LOOP ( 'NONE', ( #16617, #5872, #90947, #91272, #3660, #40413, #28597, #75161, #94568, #70748, #87395, #25361, #63174, #109387 ) ) ;
#53821=CARTESIAN_POINT ( 'NONE',  ( -2.769884583023930258, 1507.289917905509810, 221.6734208851810308 ) ) ;
#53822=CARTESIAN_POINT ( 'NONE',  ( -5.836690765424191518, 1419.530734798173626, 194.8705258415808430 ) ) ;
#53824=CARTESIAN_POINT ( 'NONE',  ( -1.430539248151910137, 1444.328264662749916, 199.1703804428329931 ) ) ;
#53827=CARTESIAN_POINT ( 'NONE',  ( 10.34950197149999873, 1451.639534151889848, 207.2650128789090047 ) ) ;
#53828=CARTESIAN_POINT ( 'NONE',  ( 3.956753969209999777, 1501.434984088090005, 230.1161809861990264 ) ) ;
#53838=CARTESIAN_POINT ( 'NONE',  ( -0.3329474807077908993, 1507.873469256806402, 221.0089344692910061 ) ) ;
#53839=EDGE_CURVE ( 'NONE', #5409, #31217, #10989, .T. ) ;
#53842=VECTOR ( 'NONE', #84420, 1000.000000000000114 ) ;
#53843=CARTESIAN_POINT ( 'NONE',  ( -10.33479253082609972, 1470.226221615439954, 212.6830489766190055 ) ) ;
#53847=CARTESIAN_POINT ( 'NONE',  ( -5.716297456320000414, 1474.267417701390059, 199.6561424594189873 ) ) ;
#53848=CARTESIAN_POINT ( 'NONE',  ( -2.351942935348799946, 1422.085795762910038, 193.1347480034229989 ) ) ;
#53851=CARTESIAN_POINT ( 'NONE',  ( -15.00012675720000033, 1503.680446340089929, 208.8094518185369850 ) ) ;
#53853=CARTESIAN_POINT ( 'NONE',  ( 11.29467570687139855, 1422.466426227199918, 207.0751064078369836 ) ) ;
#53857=VERTEX_POINT ( 'NONE', #92645 ) ;
#53863=CARTESIAN_POINT ( 'NONE',  ( 5.068064628910000202, 1505.106222020589939, 220.8372522273990057 ) ) ;
#53864=CARTESIAN_POINT ( 'NONE',  ( -14.95539309770000003, 1415.677402225710011, 211.5193032282590195 ) ) ;
#53865=CARTESIAN_POINT ( 'NONE',  ( 0.3115382523218440114, 1515.152701004710025, 204.7946991408759914 ) ) ;
#53867=CARTESIAN_POINT ( 'NONE',  ( -15.88437691653640726, 1415.959283172465575, 209.7365679856393399 ) ) ;
#53870=CARTESIAN_POINT ( 'NONE',  ( -15.92986844570000038, 1416.139044365829932, 209.7537133023089950 ) ) ;
#53879=CARTESIAN_POINT ( 'NONE',  ( 9.660635392548039491, 1469.975679021050155, 211.9824950547769902 ) ) ;
#53892=EDGE_CURVE ( 'NONE', #109119, #1510, #14278, .T. ) ;
#53903=CARTESIAN_POINT ( 'NONE',  ( -13.09068094276110017, 1508.241445731279782, 209.4862166979580138 ) ) ;
#53921=CARTESIAN_POINT ( 'NONE',  ( -0.4580525536099979700, 1421.902170014840067, 193.5483135711990030 ) ) ;
#53924=CARTESIAN_POINT ( 'NONE',  ( 10.22890245830000033, 1453.871432809989983, 189.8803906307990133 ) ) ;
#53930=CARTESIAN_POINT ( 'NONE',  ( -15.36119880041499997, 1420.424379057629949, 211.0657862475889885 ) ) ;
#53937=CARTESIAN_POINT ( 'NONE',  ( -9.241005602170000444, 1423.079004508810158, 209.8534315543390107 ) ) ;
#53942=CARTESIAN_POINT ( 'NONE',  ( -20.69303424980000372, 1486.764600954290017, 209.1218459616989946 ) ) ;
#53951=CARTESIAN_POINT ( 'NONE',  ( -1.131513733160000035, 1469.206973085589880, 219.1156501392690075 ) ) ;
#53956=CARTESIAN_POINT ( 'NONE',  ( -12.86537294912139906, 1421.504292501779901, 209.5023190072500086 ) ) ;
#53969=CARTESIAN_POINT ( 'NONE',  ( 1.334158748144050000, 1465.731125543059989, 198.1841065779290147 ) ) ;
#53970=AXIS2_PLACEMENT_3D ( 'NONE', #31241, #65424, #31791 ) ;
#53979=CARTESIAN_POINT ( 'NONE',  ( 11.75011454135350064, 1479.292909357789995, 208.4591119443479954 ) ) ;
#53985=CARTESIAN_POINT ( 'NONE',  ( 19.93504378490000306, 1473.377435931889750, 206.2335637307590162 ) ) ;
#53986=CARTESIAN_POINT ( 'NONE',  ( -8.414060040230721071, 1436.602101947940128, 214.1363812467849925 ) ) ;
#53990=CARTESIAN_POINT ( 'NONE',  ( -4.542951805869999582, 1507.945432530890002, 220.8303236145989956 ) ) ;
#53992=CARTESIAN_POINT ( 'NONE',  ( -1.661949936129999861, 1498.085228650090130, 200.7325862837689954 ) ) ;
#53993=STYLED_ITEM ( 'NONE', ( #102094 ), #17149 ) ;
#54000=B_SPLINE_CURVE_WITH_KNOTS ( 'NONE', 3,
 ( #90174, #74514, #40883, #58257, #109213, #15649, #83988, #31930, #49855, #66124, #13456, #7288, #22399, #100248, #47645, #23526, #81774, #72854, #57719, #56599, #106988, #90733 ),
 .UNSPECIFIED., .F., .F.,
 ( 4, 3, 3, 3, 3, 3, 3, 4 ),
 ( 5.710169621319999251E-17, 1.340335073529090204, 2.650534160768720060, 3.343413429321489883, 4.426679877969149857, 5.556753218544390194, 6.458769871279841368, 6.686826559119630531 ),
 .UNSPECIFIED. ) ;
#54001=CARTESIAN_POINT ( 'NONE',  ( -11.56497786232949920, 1482.641537608759791, 206.2850871889860116 ) ) ;
#54008=CARTESIAN_POINT ( 'NONE',  ( -11.02044644817170749, 1489.051081239631230, 214.3262939459677341 ) ) ;
#54009=CARTESIAN_POINT ( 'NONE',  ( -15.61208392800000055, 1415.847366682379970, 208.3828643427310112 ) ) ;
#54015=CARTESIAN_POINT ( 'NONE',  ( -9.279725527415630282, 1449.470959070069739, 208.1994392316480003 ) ) ;
#54020=CARTESIAN_POINT ( 'NONE',  ( -1.842962231260000028, 1515.219201591190085, 213.4472514034090125 ) ) ;
#54023=( BOUNDED_CURVE ( )  B_SPLINE_CURVE ( 3, ( #90905, #46730, #37760, #55682 ),
 .UNSPECIFIED., .F., .F. ) 
 B_SPLINE_CURVE_WITH_KNOTS ( ( 4, 4 ),
 ( 1.020731224408165883, 2.120869708383349650 ),
 .UNSPECIFIED. ) 
 CURVE ( )  GEOMETRIC_REPRESENTATION_ITEM ( )  RATIONAL_B_SPLINE_CURVE ( ( 1.000000000000000000, 0.9016588854088134486, 0.9016588854088134486, 1.000000000000000000 ) ) 
 REPRESENTATION_ITEM ( '' )  );
#54044=CARTESIAN_POINT ( 'NONE',  ( -10.13917572520000121, 1483.516014936390093, 202.7009691187589908 ) ) ;
#54048=CARTESIAN_POINT ( 'NONE',  ( -3.410009189096530058, 1508.551704408389924, 204.3096965353510086 ) ) ;
#54050=CARTESIAN_POINT ( 'NONE',  ( -5.100876313898289993, 1482.122728626309936, 228.9673692973009906 ) ) ;
#54051=ORIENTED_EDGE ( 'NONE', *, *, #69299, .T. ) ;
#54058=CARTESIAN_POINT ( 'NONE',  ( -4.877525054610000410, 1387.235930920489864, 203.5864774107689925 ) ) ;
#54059=CARTESIAN_POINT ( 'NONE',  ( 7.794108548359999666, 1424.952531890930004, 211.7688989986990009 ) ) ;
#54060=CARTESIAN_POINT ( 'NONE',  ( -21.26810766760000249, 1485.919195121089842, 201.7808564926190229 ) ) ;
#54062=CARTESIAN_POINT ( 'NONE',  ( 11.55221630640000008, 1480.217597331290108, 211.4789166796290090 ) ) ;
#54065=CARTESIAN_POINT ( 'NONE',  ( 7.973908635610000850, 1452.896654755889813, 214.0341050940890000 ) ) ;
#54067=ORIENTED_EDGE ( 'NONE', *, *, #43312, .T. ) ;
#54090=CARTESIAN_POINT ( 'NONE',  ( -7.219069869235789305, 1424.874073124720098, 212.8049191124847823 ) ) ;
#54095=CARTESIAN_POINT ( 'NONE',  ( 8.439944554000000210, 1428.238409027789885, 213.1498827361689905 ) ) ;
#54114=CARTESIAN_POINT ( 'NONE',  ( 13.80525599937890036, 1426.970508858360063, 197.4369866690030051 ) ) ;
#54115=CARTESIAN_POINT ( 'NONE',  ( -0.3862514052426599953, 1500.063116292059931, 233.1571727059169916 ) ) ;
#54135=CARTESIAN_POINT ( 'NONE',  ( -7.799999999999999822, 1402.913060387289988, 209.1218459616989946 ) ) ;
#54140=CARTESIAN_POINT ( 'NONE',  ( 1.941845906307360092, 1423.938214695210036, 191.2749242764670043 ) ) ;
#54152=VERTEX_POINT ( 'NONE', #42810 ) ;
#54155=ADVANCED_FACE ( 'NONE', ( #43916 ), #103238, .T. ) ;
#54157=CARTESIAN_POINT ( 'NONE',  ( -2.091756139799999747, 1484.248104535490029, 198.6248114345989677 ) ) ;
#54164=CARTESIAN_POINT ( 'NONE',  ( -6.225488187964329789, 1488.541277401709976, 218.3275497249479997 ) ) ;
#54165=CARTESIAN_POINT ( 'NONE',  ( -18.80014186020000011, 1505.319236276690162, 222.5373108268989881 ) ) ;
#54169=CARTESIAN_POINT ( 'NONE',  ( 5.571279536309999614, 1428.142529990690036, 215.3037492004590092 ) ) ;
#54181=CARTESIAN_POINT ( 'NONE',  ( 9.651063919191019025, 1425.440657924460083, 195.4941620015079877 ) ) ;
#54183=B_SPLINE_CURVE_WITH_KNOTS ( 'NONE', 3,
 ( #109772, #41476, #49877, #65024 ),
 .UNSPECIFIED., .F., .F.,
 ( 4, 4 ),
 ( 28.60746992390000187, 29.16358566613400072 ),
 .UNSPECIFIED. ) ;
#54184=CARTESIAN_POINT ( 'NONE',  ( 1.711549605159999876, 1487.306758494089991, 217.0375303586090183 ) ) ;
#54188=CARTESIAN_POINT ( 'NONE',  ( -1.384206943626949959, 1515.080800108630001, 213.4508755731779956 ) ) ;
#54190=CARTESIAN_POINT ( 'NONE',  ( -8.952478501675889433, 1478.958333138210037, 216.6003120932589923 ) ) ;
#54195=CARTESIAN_POINT ( 'NONE',  ( -11.66445033169999945, 1507.156462614389966, 208.0785273261190014 ) ) ;
#54198=CARTESIAN_POINT ( 'NONE',  ( -17.95741408820000018, 1489.793908604289982, 195.2635802347990079 ) ) ;
#54200=CARTESIAN_POINT ( 'NONE',  ( 7.477592609290000247, 1422.768710552009907, 195.6698503542990011 ) ) ;
#54207=EDGE_CURVE ( 'NONE', #35548, #32575, #23223, .T. ) ;
#54208=CARTESIAN_POINT ( 'NONE',  ( -7.607391025489999237, 1458.811203548390040, 215.0925692294790110 ) ) ;
#54212=CARTESIAN_POINT ( 'NONE',  ( -7.974153723309999720, 1424.391113290319936, 210.4473931630890036 ) ) ;
#54213=EDGE_CURVE ( 'NONE', #22689, #6446, #82517, .T. ) ;
#54216=CARTESIAN_POINT ( 'NONE',  ( -9.356374587081988992, 1447.096916614799966, 212.1461378009350085 ) ) ;
#54219=CARTESIAN_POINT ( 'NONE',  ( -2.992477406865740264, 1497.069668661619971, 221.1429599211379866 ) ) ;
#54222=ADVANCED_FACE ( 'NONE', ( #105482 ), #44510, .T. ) ;
#54224=CARTESIAN_POINT ( 'NONE',  ( 9.965113123260000094, 1472.070687861889837, 213.8432150078189977 ) ) ;
#54226=CARTESIAN_POINT ( 'NONE',  ( -8.377793394620750789, 1439.624820938689936, 206.1458744547390154 ) ) ;
#54237=CARTESIAN_POINT ( 'NONE',  ( 11.29696953253679936, 1471.442257073440032, 210.8247801971820081 ) ) ;
#54240=ADVANCED_FACE ( 'NONE', ( #23660 ), #49195, .T. ) ;
#54251=CARTESIAN_POINT ( 'NONE',  ( -4.992349863779999453, 1391.620913471789891, 214.4361776263990009 ) ) ;
#54265=CARTESIAN_POINT ( 'NONE',  ( -6.218708227939995226, 1463.827981907927779, 227.8629900557837402 ) ) ;
#54266=B_SPLINE_SURFACE_WITH_KNOTS ( 'NONE', 5, 5, ( 
 ( #2556, #43982, #103876, #60803, #26607, #94929 ),
 ( #9815, #51835, #86521, #1998, #96029, #890 ),
 ( #43432, #53501, #85972, #44536, #87644, #78119 ),
 ( #71432, #10930, #78681, #1423, #35563, #69760 ),
 ( #45106, #105547, #19862, #104985, #36679, #70872 ),
 ( #3105, #54065, #13101, #82545, #98777, #64660 ),
 ( #21495, #37787, #88742, #81407, #81967, #65201 ),
 ( #55708, #72496, #4184, #107182, #99314, #106625 ),
 ( #89829, #46206, #12577, #5839, #22040, #108286 ) ),
 .UNSPECIFIED., .F., .F., .F.,
 ( 6, 3, 6 ),
 ( 6, 6 ),
 ( 0.000000000000000000, 6.504696678220000194, 13.00939335640000039 ),
 ( 0.000000000000000000, 2.000000000000000000 ),
 .UNSPECIFIED. ) ;
#54273=CARTESIAN_POINT ( 'NONE',  ( -4.328264056532950654, 1515.110035495290049, 208.1359449714740038 ) ) ;
#54278=CARTESIAN_POINT ( 'NONE',  ( 11.21638122688047012, 1414.413060387330006, 209.8266014933970780 ) ) ;
#54286=B_SPLINE_CURVE_WITH_KNOTS ( 'NONE', 3,
 ( #47382, #81505, #63654, #20490, #71522, #97769, #80433, #70963, #4807, #105642, #38953, #3747, #98870, #21041, #11572, #73132 ),
 .UNSPECIFIED., .F., .F.,
 ( 4, 3, 3, 3, 3, 4 ),
 ( -7.319250911990000219, -7.043526182202069386, -6.032818062830740402, -5.022172799713979785, -4.011090015075000181, -2.998981459959999540 ),
 .UNSPECIFIED. ) ;
#54288=CARTESIAN_POINT ( 'NONE',  ( 11.90986840160970139, 1501.627808534720089, 211.5369186294690280 ) ) ;
#54294=CARTESIAN_POINT ( 'NONE',  ( 2.330134122034449806, 1515.551704408389924, 205.2922258479440245 ) ) ;
#54295=CARTESIAN_POINT ( 'NONE',  ( 9.045806960450768486, 1451.339811764609976, 211.1085978657239934 ) ) ;
#54296=CARTESIAN_POINT ( 'NONE',  ( 10.11452303199940062, 1452.508778506509771, 209.7496972492980092 ) ) ;
#54297=ORIENTED_EDGE ( 'NONE', *, *, #18770, .F. ) ;
#54304=CARTESIAN_POINT ( 'NONE',  ( -4.887556115857369932, 1508.551704408389924, 219.6953829590910061 ) ) ;
#54307=CARTESIAN_POINT ( 'NONE',  ( 3.179666502929999972, 1490.437437189990078, 188.4750071136990073 ) ) ;
#54311=CARTESIAN_POINT ( 'NONE',  ( 5.529365985937329420, 1466.685659397790005, 204.7973175625270130 ) ) ;
#54312=CARTESIAN_POINT ( 'NONE',  ( 1.338019038549999928, 1431.361301794989913, 218.5179653796290040 ) ) ;
#54313=CARTESIAN_POINT ( 'NONE',  ( 21.04236285220000013, 1494.763913780290068, 208.1091839946190021 ) ) ;
#54315=CARTESIAN_POINT ( 'NONE',  ( 0.6364662388029991291, 1454.894302228490005, 215.7249496973589942 ) ) ;
#54319=FACE_OUTER_BOUND ( 'NONE', #11769, .T. ) ;
#54324=CARTESIAN_POINT ( 'NONE',  ( -18.66135599109209764, 1441.829349819740173, 210.7852733701969896 ) ) ;
#54325=CARTESIAN_POINT ( 'NONE',  ( 2.475018581880529922, 1497.111080376900190, 196.9667223532030107 ) ) ;
#54331=CARTESIAN_POINT ( 'NONE',  ( 1.842962231260000028, 1515.551704408389924, 205.2922258481490303 ) ) ;
#54338=CARTESIAN_POINT ( 'NONE',  ( 0.1132302339970009813, 1498.032890047989895, 197.7962523521989908 ) ) ;
#54341=EDGE_CURVE ( 'NONE', #21520, #53297, #62307, .T. ) ;
#54351=LINE ( 'NONE', #29121, #10581 ) ;
#54362=CARTESIAN_POINT ( 'NONE',  ( 5.920277381630000058, 1423.127765564700212, 194.8707734773990126 ) ) ;
#54365=CARTESIAN_POINT ( 'NONE',  ( -8.080260711212272184, 1418.884620420010833, 195.9946716912613169 ) ) ;
#54370=CARTESIAN_POINT ( 'NONE',  ( 2.487924109712380094, 1508.884228866460035, 213.6131300634060040 ) ) ;
#54375=ORIENTED_EDGE ( 'NONE', *, *, #100062, .T. ) ;
#54383=CARTESIAN_POINT ( 'NONE',  ( -5.833099474469870316, 1508.551704408389924, 219.4902126349500122 ) ) ;
#54385=CARTESIAN_POINT ( 'NONE',  ( -2.916662559637150043, 1468.341157279690151, 219.5036260853820238 ) ) ;
#54388=CARTESIAN_POINT ( 'NONE',  ( 3.744312463839459593, 1509.032014876046560, 204.8809009122383600 ) ) ;
#54389=CARTESIAN_POINT ( 'NONE',  ( -7.437974795490000623, 1473.518143733989973, 200.3716835635890163 ) ) ;
#54390=CARTESIAN_POINT ( 'NONE',  ( 10.41203720280000056, 1493.307641990389811, 215.0005194938290174 ) ) ;
#54394=CARTESIAN_POINT ( 'NONE',  ( -17.64814166450000243, 1504.515913262890081, 208.9742322240140027 ) ) ;
#54406=CARTESIAN_POINT ( 'NONE',  ( 4.875788219060000372, 1505.619959711089905, 220.1093002778990240 ) ) ;
#54408=CARTESIAN_POINT ( 'NONE',  ( -17.83876811113470140, 1419.521416245730052, 206.8588588664190127 ) ) ;
#54413=CARTESIAN_POINT ( 'NONE',  ( 6.202741644639123031, 1439.658053187385121, 216.9645217985598435 ) ) ;
#54417=CARTESIAN_POINT ( 'NONE',  ( 6.282508756548999429, 1459.626149291560068, 201.6398963661700066 ) ) ;
#54422=CARTESIAN_POINT ( 'NONE',  ( -7.981287325994377291, 1424.856636039371779, 210.5242404286136377 ) ) ;
#54430=CARTESIAN_POINT ( 'NONE',  ( -3.168001005839999884, 1479.750044315889909, 229.3575515971990058 ) ) ;
#54433=DIRECTION ( 'NONE',  ( -1.000000000000000000, 0.000000000000000000, -1.224646799147351975E-16 ) ) ;
#54435=CARTESIAN_POINT ( 'NONE',  ( -15.42032581149999970, 1415.152828348040202, 209.2822251248840075 ) ) ;
#54442=CARTESIAN_POINT ( 'NONE',  ( 5.670155014969999741, 1477.128358946589969, 199.4032014051190060 ) ) ;
#54445=CARTESIAN_POINT ( 'NONE',  ( -4.748707386669323682, 1463.075551767410161, 200.5806828470055621 ) ) ;
#54448=CARTESIAN_POINT ( 'NONE',  ( -11.82625070047500060, 1481.580697255540144, 210.0186159470979987 ) ) ;
#54457=CARTESIAN_POINT ( 'NONE',  ( 4.123245670370000227, 1515.545044289889802, 208.3730318020869845 ) ) ;
#54461=CARTESIAN_POINT ( 'NONE',  ( -4.077284799680000127, 1495.755251076190007, 219.5524077617990315 ) ) ;
#54463=CARTESIAN_POINT ( 'NONE',  ( 0.4842866986810019925, 1421.662812042720134, 193.6869198051990111 ) ) ;
#54467=CARTESIAN_POINT ( 'NONE',  ( 20.81211029356619946, 1456.820296889740121, 206.9378353218430107 ) ) ;
#54474=CARTESIAN_POINT ( 'NONE',  ( -1766.069695707609526, -8382.262153571264207, -1964.859607327509593 ) ) ;
#54478=EDGE_CURVE ( 'NONE', #29958, #49356, #810, .T. ) ;
#54482=CARTESIAN_POINT ( 'NONE',  ( 11.15128118274900082, 1503.005909027870075, 212.1832507974499720 ) ) ;
#54483=CARTESIAN_POINT ( 'NONE',  ( -11.42514667305001730, 1422.040958530333455, 210.6386249240756854 ) ) ;
#54487=EDGE_CURVE ( 'NONE', #14695, #45310, #87670, .T. ) ;
#54495=DIRECTION ( 'NONE',  ( 0.02617694830785694329, 0.9996573249755577040, -1.920531143124581619E-16 ) ) ;
#54505=CARTESIAN_POINT ( 'NONE',  ( 19.03958014020000178, 1453.804227313890124, 200.7927590370090059 ) ) ;
#54507=ORIENTED_EDGE ( 'NONE', *, *, #44859, .T. ) ;
#54514=CARTESIAN_POINT ( 'NONE',  ( -1.207243347426069979, 1465.149812066310005, 198.1847202192419957 ) ) ;
#54516=ADVANCED_FACE ( 'NONE', ( #72845 ), #110008, .T. ) ;
#54533=CARTESIAN_POINT ( 'NONE',  ( 20.12874795999999833, 1473.837606016890049, 209.1218459616989946 ) ) ;
#54534=CARTESIAN_POINT ( 'NONE',  ( -9.678629675803538390, 1438.172449264850002, 211.2476436863910010 ) ) ;
#54538=CARTESIAN_POINT ( 'NONE',  ( -5.388545155500000128, 1508.534844389690079, 220.1281070202990122 ) ) ;
#54540=CARTESIAN_POINT ( 'NONE',  ( 5.501490042989999552, 1437.654011727689976, 208.9193339014500168 ) ) ;
#54554=CARTESIAN_POINT ( 'NONE',  ( -15.33858234790000097, 1415.710400555009983, 207.8621270138890225 ) ) ;
#54556=CARTESIAN_POINT ( 'NONE',  ( 7.374483138519999592, 1422.905762710230192, 195.5806561682990150 ) ) ;
#54557=AXIS2_PLACEMENT_3D ( 'NONE', #67612, #7139, #74911 ) ;
#54560=CARTESIAN_POINT ( 'NONE',  ( -9.811846248468439668, 1449.015403504370170, 207.4084956377189997 ) ) ;
#54566=CARTESIAN_POINT ( 'NONE',  ( 1.070047859700000048, 1515.100834970490041, 213.4503509424489778 ) ) ;
#54572=CARTESIAN_POINT ( 'NONE',  ( 10.34950188612880062, 1451.639534178259964, 207.2650128704659949 ) ) ;
#54574=CARTESIAN_POINT ( 'NONE',  ( 10.52570377039936567, 1462.363426962881704, 212.2902492825397474 ) ) ;
#54575=CARTESIAN_POINT ( 'NONE',  ( 0.8058486770669990307, 1507.409867506390128, 220.9636447390989815 ) ) ;
#54576=CARTESIAN_POINT ( 'NONE',  ( -5.313130013509999472, 1438.470987382389922, 207.5386937753289942 ) ) ;
#54577=ORIENTED_EDGE ( 'NONE', *, *, #70506, .T. ) ;
#54579=CARTESIAN_POINT ( 'NONE',  ( 10.91046689108939916, 1469.917267936679991, 205.8964561295520070 ) ) ;
#54586=CARTESIAN_POINT ( 'NONE',  ( -9.793579503809999309, 1482.279599785289975, 204.6454782706190088 ) ) ;
#54590=CARTESIAN_POINT ( 'NONE',  ( -2.994312402752280278, 1508.551704408389924, 204.1866477444860095 ) ) ;
#54594=CARTESIAN_POINT ( 'NONE',  ( -11.35404705328023844, 1501.711889457069674, 207.5713905607231027 ) ) ;
#54604=CARTESIAN_POINT ( 'NONE',  ( 7.537484560389999366, 1425.561342251899987, 212.1802124335790154 ) ) ;
#54605=CARTESIAN_POINT ( 'NONE',  ( -21.51339057090000040, 1505.551704408389924, 209.1218459616989946 ) ) ;
#54631=B_SPLINE_CURVE_WITH_KNOTS ( 'NONE', 3,
 ( #16180, #7256, #51463, #103508, #8894, #42504, #76664, #86167, #83956, #60999, #76117, #43073, #77233, #534, #59338, #92906, #84508, #43625, #7797, #110813, #110257, #59881, #34658, #68842, #33533, #102945, #68297, #34106, #41418, #101842, #25135, #93448, #32991, #77773, #1085, #26247, #75584, #102405, #16718, #60435, #50919, #85050, #94553, #17826, #35211, #95125, #67180, #71061, #97322 ),
 .UNSPECIFIED., .F., .F.,
 ( 4, 3, 3, 3, 3, 3, 3, 3, 3, 3, 3, 3, 3, 3, 3, 3, 4 ),
 ( -12.57638456930000004, -12.28317881154790037, -11.95680856226570121, -11.62570944429999997, -11.51472436866950133, -11.17721019273979977, -10.83638269430850087, -10.49376597961390090, -10.14927726971910005, -9.804494079901610704, -9.458815398425139520, -9.117616600358399381, -8.780289087992249719, -8.445887014764290157, -8.114782773701358920, -7.787209585419999414, -7.548674336829999554 ),
 .UNSPECIFIED. ) ;
#54636=CARTESIAN_POINT ( 'NONE',  ( 20.45347777980000004, 1495.695647834889996, 214.2365953844490036 ) ) ;
#54657=B_SPLINE_CURVE_WITH_KNOTS ( 'NONE', 3,
 ( #109649, #22855, #23961, #76594, #32926, #101773, #83886, #48660, #6080, #40232, #7730, #67115, #93384, #65463, #110192, #74415, #83335, #25064, #108541, #91735, #31830, #66017, #40785, #75516, #100140, #84976, #59267, #67666, #50848, #6631, #8271, #33465, #23426, #74962, #109112, #32392, #49756, #66573, #100678, #58156, #15556, #101216, #41348 ),
 .UNSPECIFIED., .F., .F.,
 ( 4, 3, 3, 3, 3, 3, 3, 3, 3, 3, 3, 3, 3, 3, 4 ),
 ( -77.98061142476200303, -77.46682292029849748, -77.28802957387100037, -76.91618970811789779, -75.85176799147379256, -74.38254242284349971, -72.90580023232000428, -71.43113070119559893, -69.96812857060400859, -68.52304788189539408, -67.09990280889999781, -66.55476356243740099, -65.17590846059749765, -63.76822099488400397, -62.33963421249379877 ),
 .UNSPECIFIED. ) ;
#54662=CARTESIAN_POINT ( 'NONE',  ( 13.28133272618789995, 1426.800456727919936, 196.8617550854280012 ) ) ;
#54680=CARTESIAN_POINT ( 'NONE',  ( -4.523944140811339665, 1455.378620635879997, 200.8408219016489795 ) ) ;
#54682=CARTESIAN_POINT ( 'NONE',  ( 10.23319004314000047, 1470.053042612599938, 209.0118140887069842 ) ) ;
#54683=ORIENTED_EDGE ( 'NONE', *, *, #24674, .T. ) ;
#54691=CARTESIAN_POINT ( 'NONE',  ( 0.3990618680159989662, 1443.956493356090050, 218.0653600664390126 ) ) ;
#54708=CARTESIAN_POINT ( 'NONE',  ( -16.69414477714984102, 1417.182685337895919, 207.2247089525174317 ) ) ;
#54713=CARTESIAN_POINT ( 'NONE',  ( -10.87802087445689914, 1489.387117259759862, 213.6045155262730191 ) ) ;
#54714=CARTESIAN_POINT ( 'NONE',  ( -12.04603691750549999, 1481.197963875999903, 227.9689184246500133 ) ) ;
#54718=CARTESIAN_POINT ( 'NONE',  ( 4.859679523539999657, 1428.484836093189870, 215.8649822896190074 ) ) ;
#54720=ORIENTED_EDGE ( 'NONE', *, *, #56458, .T. ) ;
#54732=CARTESIAN_POINT ( 'NONE',  ( 4.709520687179999499, 1480.407452823689937, 228.9869292435990076 ) ) ;
#54736=CARTESIAN_POINT ( 'NONE',  ( 0.4393421188271590117, 1515.147356017579796, 213.4491327457870113 ) ) ;
#54740=LINE ( 'NONE', #88869, #55082 ) ;
#54744=CARTESIAN_POINT ( 'NONE',  ( 9.611475570199999652, 1494.388845096189925, 188.1518348324989915 ) ) ;
#54752=CARTESIAN_POINT ( 'NONE',  ( -9.702736503189999695, 1460.950281053889967, 212.1761309882089961 ) ) ;
#54762=CARTESIAN_POINT ( 'NONE',  ( 1.382080682762369950, 1495.864354590530183, 221.3843093997170115 ) ) ;
#54763=VERTEX_POINT ( 'NONE', #90725 ) ;
#54765=CARTESIAN_POINT ( 'NONE',  ( 5.794788514299999527, 1472.774664811089906, 217.7075892082590087 ) ) ;
#54766=CARTESIAN_POINT ( 'NONE',  ( -8.474153735295640644, 1438.741029936910081, 207.0760172009069890 ) ) ;
#54778=CARTESIAN_POINT ( 'NONE',  ( 17.80990364915628632, 1474.300541546459954, 199.4615574247595760 ) ) ;
#54788=EDGE_LOOP ( 'NONE', ( #67319, #6568, #35731 ) ) ;
#54796=CARTESIAN_POINT ( 'NONE',  ( 10.20961878419999991, 1488.772996682489975, 205.0373668638989955 ) ) ;
#54804=CARTESIAN_POINT ( 'NONE',  ( -10.01326586723869916, 1481.014341800280135, 205.7823588363200145 ) ) ;
#54814=B_SPLINE_CURVE_WITH_KNOTS ( 'NONE', 5,
 ( #84408, #42970, #67082, #58668, #32888, #59232 ),
 .UNSPECIFIED., .F., .F.,
 ( 6, 6 ),
 ( 396.1714721989999930, 406.4187164909999979 ),
 .UNSPECIFIED. ) ;
#54815=CARTESIAN_POINT ( 'NONE',  ( -14.31200010202953621, 1415.739699867087893, 203.9225122205529885 ) ) ;
#54819=CARTESIAN_POINT ( 'NONE',  ( -9.588314140733929847, 1460.162249162269973, 210.2003709356519892 ) ) ;
#54830=CARTESIAN_POINT ( 'NONE',  ( 12.44780704128189974, 1501.268281525590055, 211.7240718234590133 ) ) ;
#54831=CARTESIAN_POINT ( 'NONE',  ( -15.98971164002714573, 1420.239571111833811, 209.6843301561163173 ) ) ;
#54837=FACE_OUTER_BOUND ( 'NONE', #57366, .T. ) ;
#54843=FACE_OUTER_BOUND ( 'NONE', #12526, .T. ) ;
#54846=CARTESIAN_POINT ( 'NONE',  ( -17.51439927794370277, 1442.104016966609834, 219.2287862311399920 ) ) ;
#54853=CARTESIAN_POINT ( 'NONE',  ( -5.883891048220000641, 1463.750324872290093, 200.7608182267589996 ) ) ;
#54854=CARTESIAN_POINT ( 'NONE',  ( -2.777734314609999977, 1432.637008328589900, 217.4880619237290205 ) ) ;
#54857=CARTESIAN_POINT ( 'NONE',  ( 5.225857906580000822, 1452.691914677890054, 212.7582739490889878 ) ) ;
#54862=CARTESIAN_POINT ( 'NONE',  ( 12.09532526841919875, 1491.441359186789896, 206.9399676582060010 ) ) ;
#54864=EDGE_LOOP ( 'NONE', ( #29481, #28021, #32702, #38194 ) ) ;
#54867=CARTESIAN_POINT ( 'NONE',  ( -2.900738715952500435, 1495.748930167899971, 197.1341948204009782 ) ) ;
#54880=CARTESIAN_POINT ( 'NONE',  ( 0.8568566378070020528, 1497.755226128189861, 197.7133750264989942 ) ) ;
#54881=CARTESIAN_POINT ( 'NONE',  ( -9.199712988752910547, 1490.512384490800059, 190.1963207482600069 ) ) ;
#54883=ORIENTED_EDGE ( 'NONE', *, *, #11153, .T. ) ;
#54898=EDGE_LOOP ( 'NONE', ( #61526, #70232, #91360, #27450, #104949, #50875, #72555, #1342 ) ) ;
#54899=CARTESIAN_POINT ( 'NONE',  ( 10.10398322925309955, 1452.602376352069996, 209.9919527220669977 ) ) ;
#54901=EDGE_CURVE ( 'NONE', #14236, #19394, #40838, .T. ) ;
#54902=VERTEX_POINT ( 'NONE', #51918 ) ;
#54906=EDGE_CURVE ( 'NONE', #33283, #77824, #71641, .T. ) ;
#54919=ORIENTED_EDGE ( 'NONE', *, *, #120, .T. ) ;
#54922=CARTESIAN_POINT ( 'NONE',  ( 4.483791294666029437, 1499.492573966179862, 198.5611395500710046 ) ) ;
#54924=CARTESIAN_POINT ( 'NONE',  ( -3.295469101731109962, 1470.146704297040060, 218.7056315512149922 ) ) ;
#54927=CARTESIAN_POINT ( 'NONE',  ( -3.394303741754500336, 1476.460482402099842, 220.0906546599869955 ) ) ;
#54931=CARTESIAN_POINT ( 'NONE',  ( -20.32281514509999809, 1505.121794388689977, 209.3836844847139957 ) ) ;
#54943=EDGE_CURVE ( 'NONE', #110516, #95904, #34676, .T. ) ;
#54950=CARTESIAN_POINT ( 'NONE',  ( 12.89505231660000106, 1420.989630775359956, 203.4267439564690108 ) ) ;
#54953=CARTESIAN_POINT ( 'NONE',  ( -0.3384141495062999994, 1430.231679807619912, 199.7147382543149945 ) ) ;
#54961=CARTESIAN_POINT ( 'NONE',  ( -3.523962691040000372, 1476.511731505490161, 220.0526012038990018 ) ) ;
#54972=CARTESIAN_POINT ( 'NONE',  ( -14.41990770658309984, 1417.158242887760025, 203.2539387402569844 ) ) ;
#54977=CARTESIAN_POINT ( 'NONE',  ( 9.237335364602959231, 1428.214395631979869, 212.7147833259940057 ) ) ;
#54978=CARTESIAN_POINT ( 'NONE',  ( -4.226426710960000221, 1515.477082012290111, 208.7508649547930020 ) ) ;
#54984=CARTESIAN_POINT ( 'NONE',  ( 3.265660027580000069, 1477.001235074189935, 198.7922852500990132 ) ) ;
#54988=CARTESIAN_POINT ( 'NONE',  ( 17.72039215071724172, 1432.779376552643726, 213.8336839905872750 ) ) ;
#54992=CARTESIAN_POINT ( 'NONE',  ( -11.81191611200530112, 1481.532780713840111, 210.1673330252230016 ) ) ;
#54998=CARTESIAN_POINT ( 'NONE',  ( -12.04329576969499982, 1491.114171671750000, 206.7787137245340148 ) ) ;
#54999=CARTESIAN_POINT ( 'NONE',  ( -3.605016531877470065, 1508.551704408389924, 204.3978405181830169 ) ) ;
#55002=DIRECTION ( 'NONE',  ( 0.9085883915379301401, 0.3022389680066620010, -0.2883032101465139996 ) ) ;
#55011=CARTESIAN_POINT ( 'NONE',  ( -13.05160664115349789, 1467.538620789039896, 191.8992768326569660 ) ) ;
#55017=DIRECTION ( 'NONE',  ( 9.500914144214121536E-47, -1.000000000000000000, 1.836970198721029688E-16 ) ) ;
#55024=CARTESIAN_POINT ( 'NONE',  ( -9.227567128520000495, 1423.503386125029920, 208.4707392769450109 ) ) ;
#55030=ORIENTED_EDGE ( 'NONE', *, *, #41387, .F. ) ;
#55036=B_SPLINE_CURVE_WITH_KNOTS ( 'NONE', 5,
 ( #57200, #72346, #63411, #98615, #47678, #38165 ),
 .UNSPECIFIED., .F., .F.,
 ( 6, 6 ),
 ( 0.000000000000000000, 0.9643540072699122723 ),
 .UNSPECIFIED. ) ;
#55040=CARTESIAN_POINT ( 'NONE',  ( 12.56049338238149815, 1501.076573751879778, 211.0976562363760252 ) ) ;
#55043=CARTESIAN_POINT ( 'NONE',  ( 3.823234350589999941, 1434.969202599190112, 204.8006882687589894 ) ) ;
#55045=CARTESIAN_POINT ( 'NONE',  ( 8.129477481277049833, 1461.711625216570155, 228.8738004967299844 ) ) ;
#55046=CARTESIAN_POINT ( 'NONE',  ( 6.485530625610728350, 1492.746195377240610, 218.1903392014115468 ) ) ;
#55055=DIRECTION ( 'NONE',  ( 9.230617842401318720E-47, -1.000000000000000000, 1.836970198721029688E-16 ) ) ;
#55058=CARTESIAN_POINT ( 'NONE',  ( -1.551174237339999928, 1463.265707418689999, 199.4651013571389910 ) ) ;
#55067=CARTESIAN_POINT ( 'NONE',  ( 11.57490036778929898, 1478.937116359260017, 207.0860133150080173 ) ) ;
#55070=CARTESIAN_POINT ( 'NONE',  ( 7.518776976417130165, 1428.948321996720097, 214.9051160645190066 ) ) ;
#55074=CARTESIAN_POINT ( 'NONE',  ( -7.691664047984310137, 1435.994123091719985, 215.1214903504479992 ) ) ;
#55082=VECTOR ( 'NONE', #69332, 1000.000000000000000 ) ;
#55089=CARTESIAN_POINT ( 'NONE',  ( 11.39861885689485277, 1453.593877275467094, 193.2142631562276449 ) ) ;
#55095=CARTESIAN_POINT ( 'NONE',  ( -10.22679430872973327, 1488.677234487174246, 215.7753183090639766 ) ) ;
#55096=CARTESIAN_POINT ( 'NONE',  ( -15.70353555820000047, 1415.826269415930028, 208.9425385408250122 ) ) ;
#55100=CIRCLE ( 'NONE', #94375, 1237.216328224680410 ) ;
#55110=CARTESIAN_POINT ( 'NONE',  ( 1.480872463499999903, 1515.456375364289897, 213.2974053764389737 ) ) ;
#55113=AXIS2_PLACEMENT_3D ( 'NONE', #103742, #44405, #97549 ) ;
#55117=LINE ( 'NONE', #5232, #56785 ) ;
#55127=CARTESIAN_POINT ( 'NONE',  ( 9.726769132718798616, 1469.060278453449882, 204.1925708335969887 ) ) ;
#55129=DIRECTION ( 'NONE',  ( -9.500021872036790217E-47, 1.000000000000000000, -1.836970198721029688E-16 ) ) ;
#55130=AXIS2_PLACEMENT_3D ( 'NONE', #72081, #106733, #38428 ) ;
#55131=CARTESIAN_POINT ( 'NONE',  ( -8.106555885276549134, 1438.741351455190170, 205.9368832915250209 ) ) ;
#55136=B_SPLINE_CURVE_WITH_KNOTS ( 'NONE', 5,
 ( #96981, #61199, #29214, #54988, #20244, #1264, #35965, #70154, #63402 ),
 .UNSPECIFIED., .F., .F.,
 ( 6, 3, 6 ),
 ( 0.000000000000000000, 0.02144875489016424136, 1.000000000000000000 ),
 .UNSPECIFIED. ) ;
#55138=CARTESIAN_POINT ( 'NONE',  ( -9.933553457609999526, 1481.595314920090004, 205.4496293638590032 ) ) ;
#55144=CARTESIAN_POINT ( 'NONE',  ( -11.35135138259924048, 1503.578306220690820, 207.0399780940998369 ) ) ;
#55153=CARTESIAN_POINT ( 'NONE',  ( 7.708772379780000072, 1427.786886959790081, 212.9376885971290108 ) ) ;
#55154=CARTESIAN_POINT ( 'NONE',  ( -11.77905477449999871, 1483.168199375790209, 228.2502073304989949 ) ) ;
#55156=LINE ( 'NONE', #54062, #11451 ) ;
#55169=CARTESIAN_POINT ( 'NONE',  ( -1.828126493375330064, 1464.537186451630077, 199.0653043791290031 ) ) ;
#55182=CARTESIAN_POINT ( 'NONE',  ( -17.26197377869999983, 1420.099051756930066, 204.7291993270589785 ) ) ;
#55188=ORIENTED_EDGE ( 'NONE', *, *, #30231, .T. ) ;
#55194=CARTESIAN_POINT ( 'NONE',  ( 11.01187563919999945, 1492.459055989690114, 212.4069243732789971 ) ) ;
#55208=CARTESIAN_POINT ( 'NONE',  ( 8.632538001083871038, 1425.507033873999944, 193.3055192643680016 ) ) ;
#55221=CARTESIAN_POINT ( 'NONE',  ( 12.74774243120000072, 1426.600000495550148, 203.5345172987589990 ) ) ;
#55224=CARTESIAN_POINT ( 'NONE',  ( -16.62689959340567114, 1417.072749475663613, 207.5381517451929483 ) ) ;
#55226=CARTESIAN_POINT ( 'NONE',  ( 9.953995014223000481, 1468.683952319419859, 207.9911765682120119 ) ) ;
#55231=CARTESIAN_POINT ( 'NONE',  ( 2.802883801854730184, 1485.536427198280080, 201.6817236178680162 ) ) ;
#55234=CARTESIAN_POINT ( 'NONE',  ( 7.993316216764522864, 1423.834663174395246, 195.8541102515277430 ) ) ;
#55235=CARTESIAN_POINT ( 'NONE',  ( 1.198395538569999808, 1443.136157641690033, 218.0744600652089957 ) ) ;
#55241=CARTESIAN_POINT ( 'NONE',  ( 17.68711869539999881, 1428.828027849089949, 204.9896315466789929 ) ) ;
#55251=CARTESIAN_POINT ( 'NONE',  ( -2.069830516030000123, 1485.439312555290144, 197.8250537956990058 ) ) ;
#55252=CIRCLE ( 'NONE', #15788, 16.53861382824159421 ) ;
#55258=CARTESIAN_POINT ( 'NONE',  ( 3.300283013599780269, 1494.041687248919970, 219.7877414054240148 ) ) ;
#55260=CARTESIAN_POINT ( 'NONE',  ( 0.9103409915569969924, 1462.760008604990162, 230.5111369474990113 ) ) ;
#55261=CARTESIAN_POINT ( 'NONE',  ( -15.31654147834860069, 1415.677402202140001, 208.8922298180530106 ) ) ;
#55272=CARTESIAN_POINT ( 'NONE',  ( -7.809009848659999697, 1492.243080287389830, 209.5285790274940041 ) ) ;
#55273=B_SPLINE_CURVE_WITH_KNOTS ( 'NONE', 3,
 ( #44543, #11492, #4192, #28841, #104990, #20411 ),
 .UNSPECIFIED., .F., .F.,
 ( 4, 2, 4 ),
 ( 0.000000000000000000, 0.5000000000000000000, 1.000000000000000000 ),
 .UNSPECIFIED. ) ;
#55278=CARTESIAN_POINT ( 'NONE',  ( 8.691006959535679144, 1437.158552202200099, 210.3927666437540154 ) ) ;
#55280=CARTESIAN_POINT ( 'NONE',  ( 2.774288201250000085, 1480.748952858089979, 229.3996213013989802 ) ) ;
#55282=CARTESIAN_POINT ( 'NONE',  ( 7.956123293573201138, 1465.862754146189900, 215.0084650448240211 ) ) ;
#55284=CARTESIAN_POINT ( 'NONE',  ( -0.9886889294026209862, 1515.109643008300054, 213.4501202958599890 ) ) ;
#55291=CARTESIAN_POINT ( 'NONE',  ( -13.37159485409999959, 1504.309599599390140, 208.8294216085490120 ) ) ;
#55292=CARTESIAN_POINT ( 'NONE',  ( -22.19118138694790332, 1483.601908343390051, 216.8115092454290220 ) ) ;
#55296=CARTESIAN_POINT ( 'NONE',  ( -4.992349863779999453, 1391.620913471789891, 209.1218459612989875 ) ) ;
#55297=CARTESIAN_POINT ( 'NONE',  ( 4.326992699989999913, 1515.158586642790169, 209.1218459614979963 ) ) ;
#55299=CARTESIAN_POINT ( 'NONE',  ( -4.698255939499999201, 1458.218207492389865, 217.8981937722389830 ) ) ;
#55317=CARTESIAN_POINT ( 'NONE',  ( 6.950546267860000071, 1473.247417472590087, 217.6958634347789712 ) ) ;
#55322=CARTESIAN_POINT ( 'NONE',  ( 9.788572749075168389, 1435.243968381529839, 208.4609852036589928 ) ) ;
#55327=CARTESIAN_POINT ( 'NONE',  ( -0.4964140083681939930, 1467.594909982409945, 220.2089270784179860 ) ) ;
#55330=AXIS2_PLACEMENT_3D ( 'NONE', #74481, #91255, #32989 ) ;
#55342=CARTESIAN_POINT ( 'NONE',  ( -5.199570074521043139, 1391.913060385946665, 214.4361776394624428 ) ) ;
#55358=EDGE_CURVE ( 'NONE', #97980, #109119, #80844, .T. ) ;
#55359=DIRECTION ( 'NONE',  ( -1.000000000000000000, 0.000000000000000000, 0.000000000000000000 ) ) ;
#55373=CARTESIAN_POINT ( 'NONE',  ( 10.66966122738459966, 1480.341429598930063, 208.7487408019889870 ) ) ;
#55380=CARTESIAN_POINT ( 'NONE',  ( -2.402260219255893059, 1429.560837414985372, 200.7439439027626236 ) ) ;
#55388=B_SPLINE_CURVE_WITH_KNOTS ( 'NONE', 5,
 ( #69266, #103372, #60875, #52462, #19934, #37306 ),
 .UNSPECIFIED., .F., .F.,
 ( 6, 6 ),
 ( -2.000000000000000000, 0.000000000000000000 ),
 .UNSPECIFIED. ) ;
#55390=CARTESIAN_POINT ( 'NONE',  ( -3.674130623179999944, 1476.125971546490064, 199.4510817715890312 ) ) ;
#55392=EDGE_LOOP ( 'NONE', ( #12542, #98093 ) ) ;
#55393=CARTESIAN_POINT ( 'NONE',  ( -3.071489522903089853, 1470.850346192869893, 187.3986287140659783 ) ) ;
#55394=ORIENTED_EDGE ( 'NONE', *, *, #83572, .T. ) ;
#55396=CARTESIAN_POINT ( 'NONE',  ( 0.1948465599140009885, 1484.368352875590062, 201.1680343295390117 ) ) ;
#55412=CARTESIAN_POINT ( 'NONE',  ( -5.445055359510000415, 1494.866998062989978, 198.0707221814990078 ) ) ;
#55440=CARTESIAN_POINT ( 'NONE',  ( -0.1956928720520010045, 1486.480037045490008, 220.3153739831990094 ) ) ;
#55443=CARTESIAN_POINT ( 'NONE',  ( 19.93609162699999970, 1473.378341243790146, 206.2392384464789927 ) ) ;
#55446=CARTESIAN_POINT ( 'NONE',  ( 11.86100282799569960, 1492.894947744830006, 212.5846961511890072 ) ) ;
#55452=CARTESIAN_POINT ( 'NONE',  ( 5.898946028590000168, 1423.982493417579917, 194.4067087233990208 ) ) ;
#55455=CARTESIAN_POINT ( 'NONE',  ( -12.09623089429489973, 1446.031664988779994, 193.6906620567080211 ) ) ;
#55459=ORIENTED_EDGE ( 'NONE', *, *, #28161, .F. ) ;
#55465=CARTESIAN_POINT ( 'NONE',  ( 9.534480203992039549, 1481.987763606179897, 216.0982299746490014 ) ) ;
#55468=ORIENTED_EDGE ( 'NONE', *, *, #54207, .T. ) ;
#55474=CARTESIAN_POINT ( 'NONE',  ( -3.364963321921979666, 1469.699125603920038, 218.6607286373120189 ) ) ;
#55477=CARTESIAN_POINT ( 'NONE',  ( 8.765535317279999461, 1421.152484001810080, 196.5454161687989938 ) ) ;
#55478=CARTESIAN_POINT ( 'NONE',  ( 1.874146057977200019, 1474.821289880090035, 220.3858797084459979 ) ) ;
#55479=CARTESIAN_POINT ( 'NONE',  ( -7.116694769601350501, 1494.227560407549845, 199.0721606401010035 ) ) ;
#55487=ORIENTED_EDGE ( 'NONE', *, *, #101556, .F. ) ;
#55493=CARTESIAN_POINT ( 'NONE',  ( -15.48550906000000005, 1416.155796905759871, 210.9866352200689903 ) ) ;
#55494=CARTESIAN_POINT ( 'NONE',  ( 3.422247113165846955, 1486.244152127078905, 198.8929547559257287 ) ) ;
#55496=CARTESIAN_POINT ( 'NONE',  ( 3.483866223379999738, 1429.087410406890058, 216.6553312436790009 ) ) ;
#55498=CARTESIAN_POINT ( 'NONE',  ( -5.569019969264549452, 1475.748224554402441, 217.8649781415279278 ) ) ;
#55499=CARTESIAN_POINT ( 'NONE',  ( 9.130411372029950456, 1437.290848551490399, 212.9268650149392670 ) ) ;
#55502=FACE_OUTER_BOUND ( 'NONE', #45773, .T. ) ;
#55503=CARTESIAN_POINT ( 'NONE',  ( 2.236590363472370058, 1458.510893503000034, 199.7494169500020007 ) ) ;
#55520=VECTOR ( 'NONE', #87014, 1000.000000000000114 ) ;
#55522=CARTESIAN_POINT ( 'NONE',  ( 0.1474424791818742808, 1484.358452256622058, 198.4190835461621134 ) ) ;
#55530=CARTESIAN_POINT ( 'NONE',  ( -11.04529535729999878, 1492.261561399990114, 209.4862125649669906 ) ) ;
#55541=CARTESIAN_POINT ( 'NONE',  ( -12.02398823846299791, 1491.147743522770043, 206.6805235778679730 ) ) ;
#55544=B_SPLINE_CURVE_WITH_KNOTS ( 'NONE', 5,
 ( #32889, #91153, #99536, #32358, #66537, #92256 ),
 .UNSPECIFIED., .F., .F.,
 ( 6, 6 ),
 ( 330.4685494459999973, 340.5245863399999848 ),
 .UNSPECIFIED. ) ;
#55550=CARTESIAN_POINT ( 'NONE',  ( -4.043437603129999225, 1495.741838748290093, 219.5649473730990167 ) ) ;
#55557=CARTESIAN_POINT ( 'NONE',  ( 0.9782357301829970320, 1463.155161847389991, 230.5295413522989918 ) ) ;
#55561=CARTESIAN_POINT ( 'NONE',  ( 19.84434320180000100, 1475.251313466289957, 205.2746163281789791 ) ) ;
#55571=CARTESIAN_POINT ( 'NONE',  ( 12.02500756018520178, 1501.456221950489862, 211.6043302210539991 ) ) ;
#55585=B_SPLINE_CURVE_WITH_KNOTS ( 'NONE', 3,
 ( #42236, #76384, #110533, #70792, #799, #95950, #60721, #1346, #36055, #2478, #8611, #42788, #35485, #76948, #26524, #61285, #257, #87564, #17549, #18664, #69679, #10279, #78038, #62379, #10853, #94843, #43894, #44456, #45025, #52315, #9729 ),
 .UNSPECIFIED., .F., .F.,
 ( 4, 3, 3, 3, 3, 3, 3, 3, 3, 3, 4 ),
 ( -14.48744219459999982, -13.44410458394230012, -12.37566277839809992, -11.18777881828939869, -9.902217085923059159, -8.626592106539620275, -8.281559019981870051, -7.395949616050979891, -6.456807838355668849, -5.467544445957390309, -4.410666364560000829 ),
 .UNSPECIFIED. ) ;
#55589=CARTESIAN_POINT ( 'NONE',  ( 10.94404851108689947, 1480.986328507249937, 213.6237919197210147 ) ) ;
#55595=CARTESIAN_POINT ( 'NONE',  ( -8.627754863869999014, 1437.492696374190018, 228.3379673428989918 ) ) ;
#55600=EDGE_CURVE ( 'NONE', #46077, #2310, #87459, .T. ) ;
#55604=CARTESIAN_POINT ( 'NONE',  ( 12.30351751032840113, 1499.827690331060012, 206.1221001624080031 ) ) ;
#55625=CARTESIAN_POINT ( 'NONE',  ( -7.163586313923399729, 1435.603035147609944, 215.7022475339200014 ) ) ;
#55639=CARTESIAN_POINT ( 'NONE',  ( -11.67352926041350081, 1482.512923242310080, 206.7897318267789899 ) ) ;
#55641=CARTESIAN_POINT ( 'NONE',  ( 14.63781025022767679, 1454.494882998578305, 195.9652644489082149 ) ) ;
#55642=CARTESIAN_POINT ( 'NONE',  ( -10.31471925920000032, 1423.142082606249915, 193.7320793877989900 ) ) ;
#55647=CARTESIAN_POINT ( 'NONE',  ( -15.11314298410000134, 1415.677402202029953, 207.9092237183590157 ) ) ;
#55649=CARTESIAN_POINT ( 'NONE',  ( 11.29707874440000026, 1420.194464914089849, 198.6147532060990102 ) ) ;
#55650=CARTESIAN_POINT ( 'NONE',  ( -1.736874410247479794, 1445.847355267769899, 215.2372654443830129 ) ) ;
#55654=ORIENTED_EDGE ( 'NONE', *, *, #43794, .F. ) ;
#55662=CARTESIAN_POINT ( 'NONE',  ( 3.350944662710000355, 1464.628126271390101, 199.8699733667390035 ) ) ;
#55664=CARTESIAN_POINT ( 'NONE',  ( -10.27502231191230031, 1447.498783342189881, 210.3549345117849896 ) ) ;
#55677=DIRECTION ( 'NONE',  ( 1.149679124779773953E-17, 1.000000000000000000, -1.829746454213089849E-16 ) ) ;
#55682=CARTESIAN_POINT ( 'NONE',  ( 0.7162863658319988946, 1429.709265593189912, 217.4063670190490143 ) ) ;
#55691=CARTESIAN_POINT ( 'NONE',  ( -6.907011062519999633, 1472.523400736590020, 209.7330543039639963 ) ) ;
#55692=CARTESIAN_POINT ( 'NONE',  ( -15.59264667799007498, 1415.962102148422218, 208.0126982715246697 ) ) ;
#55698=EDGE_CURVE ( 'NONE', #34842, #25016, #8698, .T. ) ;
#55701=CARTESIAN_POINT ( 'NONE',  ( 8.054683762439999839, 1427.717696033889979, 212.5858566009490005 ) ) ;
#55702=CARTESIAN_POINT ( 'NONE',  ( -4.705736654490000781, 1479.984769897790102, 230.9466533013989817 ) ) ;
#55708=CARTESIAN_POINT ( 'NONE',  ( 8.503372964620000474, 1452.005661874290126, 212.9202014103589988 ) ) ;
#55715=EDGE_CURVE ( 'NONE', #73362, #39044, #21965, .T. ) ;
#55717=CARTESIAN_POINT ( 'NONE',  ( 15.23962836178434799, 1416.181292664740113, 211.4166089860522106 ) ) ;
#55722=CARTESIAN_POINT ( 'NONE',  ( -2.280862363224759992, 1463.582457375659942, 199.5877073955589935 ) ) ;
#55727=DIRECTION ( 'NONE',  ( 1.224646799147350002E-16, -1.836970198721029688E-16, -1.000000000000000000 ) ) ;
#55734=CARTESIAN_POINT ( 'NONE',  ( 20.99932333639999982, 1495.227718574589971, 211.1881774286989923 ) ) ;
#55742=CARTESIAN_POINT ( 'NONE',  ( -17.90721988768679651, 1508.493835039639862, 211.9093185509239845 ) ) ;
#55745=TOROIDAL_SURFACE ( 'NONE', #57500, 12.73448142120000171, 1.000000000000000000 ) ;
#55749=CARTESIAN_POINT ( 'NONE',  ( -11.80334333584940154, 1489.554055793390035, 212.2407443684180066 ) ) ;
#55767=CARTESIAN_POINT ( 'NONE',  ( 10.29570781656459921, 1425.935951659160082, 194.3061580000300239 ) ) ;
#55778=CARTESIAN_POINT ( 'NONE',  ( 4.678155166859202296, 1508.611350403214146, 206.6339108396268784 ) ) ;
#55780=CARTESIAN_POINT ( 'NONE',  ( 10.94554652600000111, 1425.626382808379958, 206.1464673162289785 ) ) ;
#55781=CARTESIAN_POINT ( 'NONE',  ( 0.07104776210500948763, 1498.478595971874256, 197.7944178200672809 ) ) ;
#55784=CARTESIAN_POINT ( 'NONE',  ( 10.05617058044520107, 1469.475797196530038, 208.7796867827769915 ) ) ;
#55785=ORIENTED_EDGE ( 'NONE', *, *, #24089, .T. ) ;
#55788=ORIENTED_EDGE ( 'NONE', *, *, #92675, .F. ) ;
#55792=CARTESIAN_POINT ( 'NONE',  ( 7.762807725464860198, 1423.432002036965287, 195.8271426519320073 ) ) ;
#55793=CARTESIAN_POINT ( 'NONE',  ( 2.254749836789999851, 1442.631473631490053, 217.8400976104589972 ) ) ;
#55803=ORIENTED_EDGE ( 'NONE', *, *, #88465, .T. ) ;
#55805=CARTESIAN_POINT ( 'NONE',  ( -8.229715745860000098, 1508.551704408389924, 218.8951070726089938 ) ) ;
#55807=CARTESIAN_POINT ( 'NONE',  ( 11.32877768939290064, 1470.635785175149977, 208.0137898554069977 ) ) ;
#55808=CARTESIAN_POINT ( 'NONE',  ( -6.025153380789999957, 1484.743691390089907, 198.8560516573990071 ) ) ;
#55813=CARTESIAN_POINT ( 'NONE',  ( 2.551826806925589608, 1494.220102795730099, 219.9851886801529872 ) ) ;
#55814=CARTESIAN_POINT ( 'NONE',  ( -22.19118107542460194, 1483.601927841320048, 216.8115131704170153 ) ) ;
#55815=CARTESIAN_POINT ( 'NONE',  ( -14.78101880266670065, 1415.677402202059966, 206.5097581168130034 ) ) ;
#55817=CARTESIAN_POINT ( 'NONE',  ( 7.039730798329999928, 1428.888324978490118, 214.9446073011990279 ) ) ;
#55818=FACE_OUTER_BOUND ( 'NONE', #82007, .T. ) ;
#55831=LINE ( 'NONE', #65877, #106931 ) ;
#55835=CARTESIAN_POINT ( 'NONE',  ( -1.059358656752720007, 1515.104045403560121, 213.4502668743000129 ) ) ;
#55837=CARTESIAN_POINT ( 'NONE',  ( -7.722301029971450070, 1478.317878138009974, 217.8058796438500053 ) ) ;
#55842=ORIENTED_EDGE ( 'NONE', *, *, #9048, .F. ) ;
#55844=CARTESIAN_POINT ( 'NONE',  ( -22.17228250857910155, 1484.784770550770190, 217.0496227037889980 ) ) ;
#55846=CARTESIAN_POINT ( 'NONE',  ( 12.40160258794860049, 1420.584110727309962, 200.5244627772079866 ) ) ;
#55852=ADVANCED_FACE ( 'NONE', ( #77139 ), #27513, .T. ) ;
#55853=CARTESIAN_POINT ( 'NONE',  ( 4.371513128651370650, 1484.373699270089901, 220.1281034412249937 ) ) ;
#55855=CARTESIAN_POINT ( 'NONE',  ( -5.518833401969999386, 1458.218094844590041, 217.1129845543590022 ) ) ;
#55865=CARTESIAN_POINT ( 'NONE',  ( -17.62094095786948600, 1419.757685654823035, 206.8396910412140244 ) ) ;
#55867=EDGE_CURVE ( 'NONE', #39608, #35904, #69051, .T. ) ;
#55869=ORIENTED_EDGE ( 'NONE', *, *, #101556, .T. ) ;
#55881=CARTESIAN_POINT ( 'NONE',  ( 0.2255696094212939762, 1467.412027614160024, 220.2065905680840103 ) ) ;
#55892=ADVANCED_FACE ( 'NONE', ( #54837 ), #26155, .F. ) ;
#55903=CARTESIAN_POINT ( 'NONE',  ( 11.21247613359999917, 1490.926120241489798, 206.9376360906590264 ) ) ;
#55917=CARTESIAN_POINT ( 'NONE',  ( -0.4564753465201519811, 1455.552155115309915, 198.6001949275529910 ) ) ;
#55922=ORIENTED_EDGE ( 'NONE', *, *, #19245, .T. ) ;
#55923=ORIENTED_EDGE ( 'NONE', *, *, #20799, .F. ) ;
#55928=CARTESIAN_POINT ( 'NONE',  ( -1.506737911117850048, 1508.551704408389924, 220.0821560122830078 ) ) ;
#55933=CARTESIAN_POINT ( 'NONE',  ( -12.36724210910779931, 1502.518749642870034, 208.9800501045910153 ) ) ;
#55939=CARTESIAN_POINT ( 'NONE',  ( 4.141018395973380173, 1508.551704408389924, 204.7583302192930148 ) ) ;
#55942=CARTESIAN_POINT ( 'NONE',  ( 0.9103554862159439764, 1462.760092965149852, 230.5111408766040029 ) ) ;
#55943=ORIENTED_EDGE ( 'NONE', *, *, #26492, .T. ) ;
#55949=CARTESIAN_POINT ( 'NONE',  ( 7.739917900360000047, 1490.431902873490117, 209.0953228043489958 ) ) ;
#55952=CARTESIAN_POINT ( 'NONE',  ( 18.62883413325391047, 1458.551313265810677, 214.8531784976841550 ) ) ;
#55962=CARTESIAN_POINT ( 'NONE',  ( 12.62249134276009954, 1420.706334970369880, 201.4123180351149927 ) ) ;
#55964=CARTESIAN_POINT ( 'NONE',  ( -14.61959290290000091, 1420.357143390019928, 213.8552925859189884 ) ) ;
#55971=CARTESIAN_POINT ( 'NONE',  ( -8.796828982357618898, 1448.417242874349995, 211.5920706533679834 ) ) ;
#55976=CARTESIAN_POINT ( 'NONE',  ( 7.450732447323310303, 1425.217176014760071, 212.3482398299129841 ) ) ;
#55981=CARTESIAN_POINT ( 'NONE',  ( -15.22583482770000174, 1419.426620482320004, 199.2582349955389986 ) ) ;
#55986=CARTESIAN_POINT ( 'NONE',  ( -4.639453685896637758, 1378.135666831742583, 214.4485485313242066 ) ) ;
#55990=VERTEX_POINT ( 'NONE', #62714 ) ;
#55997=CARTESIAN_POINT ( 'NONE',  ( 6.339003235429999883, 1424.106680004219925, 194.5877290424989781 ) ) ;
#55998=VERTEX_POINT ( 'NONE', #95168 ) ;
#56002=CARTESIAN_POINT ( 'NONE',  ( -0.7790226144181949808, 1442.687261678630193, 200.2740145696140246 ) ) ;
#56009=CARTESIAN_POINT ( 'NONE',  ( 10.00658443562149991, 1481.688797028250065, 215.3953389918819710 ) ) ;
#56014=CARTESIAN_POINT ( 'NONE',  ( -3.238204166650680005, 1508.087190631079920, 220.8316669474850187 ) ) ;
#56015=CARTESIAN_POINT ( 'NONE',  ( 4.836615265953239096, 1498.177351943570102, 198.3432821877800052 ) ) ;
#56025=CARTESIAN_POINT ( 'NONE',  ( 10.72591451257290096, 1424.883072988620142, 206.5517914635169916 ) ) ;
#56028=VERTEX_POINT ( 'NONE', #18424 ) ;
#56033=CARTESIAN_POINT ( 'NONE',  ( -15.70029802240000016, 1416.147372738109880, 210.3646106849990076 ) ) ;
#56034=CARTESIAN_POINT ( 'NONE',  ( 3.629220049600000220, 1485.493215689190038, 199.0019176958990101 ) ) ;
#56036=CARTESIAN_POINT ( 'NONE',  ( 2.696703656820000017, 1429.897299915890017, 217.1506436859089888 ) ) ;
#56038=CARTESIAN_POINT ( 'NONE',  ( -8.749343725295464225, 1477.568838901969912, 214.8427604742473704 ) ) ;
#56042=CARTESIAN_POINT ( 'NONE',  ( 1.408266058077070060, 1457.262924391489832, 199.5821088331159956 ) ) ;
#56054=CARTESIAN_POINT ( 'NONE',  ( -14.75552471225380025, 1417.657372812460153, 203.2383312169210114 ) ) ;
#56066=CARTESIAN_POINT ( 'NONE',  ( 3.004219500040000046, 1486.176588069189847, 198.6256029144990123 ) ) ;
#56067=CARTESIAN_POINT ( 'NONE',  ( 7.415490016120000583, 1477.911609511289953, 201.0119040078689920 ) ) ;
#56069=CARTESIAN_POINT ( 'NONE',  ( -11.80902463480000009, 1490.509434397089990, 209.3574457513870186 ) ) ;
#56078=CARTESIAN_POINT ( 'NONE',  ( -12.11449315257920212, 1490.976347222529967, 207.1920171886079913 ) ) ;
#56087=CARTESIAN_POINT ( 'NONE',  ( 9.927196207040308806, 1470.874197623729970, 211.7260430095500112 ) ) ;
#56093=DIRECTION ( 'NONE',  ( 1.224646799147353207E-16, -1.836970198721029688E-16, -1.000000000000000000 ) ) ;
#56094=CARTESIAN_POINT ( 'NONE',  ( -18.73311320389999679, 1469.013380241389996, 201.1621679275489782 ) ) ;
#56104=CARTESIAN_POINT ( 'NONE',  ( 11.46293682908580003, 1502.175680543279896, 213.7711866132059981 ) ) ;
#56109=CARTESIAN_POINT ( 'NONE',  ( 4.086314401636647275, 1515.499673572144275, 207.2788822313456762 ) ) ;
#56111=CARTESIAN_POINT ( 'NONE',  ( -2.184771148224290194, 1486.435642548830174, 220.8481228361289936 ) ) ;
#56112=CARTESIAN_POINT ( 'NONE',  ( 12.41076581919999988, 1499.916734172390079, 206.5417464095490061 ) ) ;
#56119=CARTESIAN_POINT ( 'NONE',  ( 10.42050379654340020, 1481.382441556200092, 211.7093090774899906 ) ) ;
#56122=CARTESIAN_POINT ( 'NONE',  ( 2.487935123020000194, 1508.551704408389924, 204.1347675455010062 ) ) ;
#56124=ORIENTED_EDGE ( 'NONE', *, *, #41183, .T. ) ;
#56129=CARTESIAN_POINT ( 'NONE',  ( 12.21820660407649939, 1499.761928509490190, 205.8071831984830169 ) ) ;
#56134=CARTESIAN_POINT ( 'NONE',  ( -21.53565904410000087, 1506.077647802389947, 209.2113159668039941 ) ) ;
#56138=ORIENTED_EDGE ( 'NONE', *, *, #104725, .F. ) ;
#56139=CARTESIAN_POINT ( 'NONE',  ( 9.526054245020199929, 1462.325501871250026, 207.0857702337349906 ) ) ;
#56147=CARTESIAN_POINT ( 'NONE',  ( -17.96416104880992748, 1508.456897258907929, 211.9435951326316001 ) ) ;
#56149=CARTESIAN_POINT ( 'NONE',  ( -4.609549296629079862, 1434.018457786650060, 217.5596424976919820 ) ) ;
#56151=CARTESIAN_POINT ( 'NONE',  ( 0.8775825618903718706, 1380.371560387289946, 208.6424204230947907 ) ) ;
#56165=CARTESIAN_POINT ( 'NONE',  ( -13.33252017900000119, 1422.271663147810159, 196.2999248757990074 ) ) ;
#56170=CARTESIAN_POINT ( 'NONE',  ( -15.51493367179999971, 1415.867981975840166, 207.8251654569390325 ) ) ;
#56171=CARTESIAN_POINT ( 'NONE',  ( -8.228434171293290689, 1441.487951933999966, 203.2737819892520008 ) ) ;
#56179=VERTEX_POINT ( 'NONE', #95716 ) ;
#56182=CARTESIAN_POINT ( 'NONE',  ( 0.7398872337349989836, 1515.545288638290003, 213.2458252406289887 ) ) ;
#56183=DIRECTION ( 'NONE',  ( -0.1669062194215500117, 0.3715217273458689684, 0.9132983740423209484 ) ) ;
#56184=EDGE_CURVE ( 'NONE', #97980, #23359, #58110, .T. ) ;
#56188=CARTESIAN_POINT ( 'NONE',  ( 17.14319438672604434, 1499.112856636860215, 222.9242983244725167 ) ) ;
#56217=CARTESIAN_POINT ( 'NONE',  ( 12.51197819060429950, 1421.582269804420093, 207.2823425885030133 ) ) ;
#56219=ORIENTED_EDGE ( 'NONE', *, *, #27677, .F. ) ;
#56221=DIRECTION ( 'NONE',  ( 4.465978680329379737E-17, 1.000000000000000000, -2.349386720892264891E-16 ) ) ;
#56222=EDGE_CURVE ( 'NONE', #108882, #89343, #62590, .T. ) ;
#56223=CARTESIAN_POINT ( 'NONE',  ( 19.03958014025380052, 1453.804227312760077, 200.7927590372679845 ) ) ;
#56228=CARTESIAN_POINT ( 'NONE',  ( -5.788280361890000059, 1452.919697783089987, 200.3898760574089977 ) ) ;
#56230=CARTESIAN_POINT ( 'NONE',  ( 11.45577226660000036, 1502.286415424589904, 208.3140783707030153 ) ) ;
#56231=CARTESIAN_POINT ( 'NONE',  ( -18.80014186020000011, 1505.319236276690162, 222.5373108268989881 ) ) ;
#56233=CARTESIAN_POINT ( 'NONE',  ( -20.32951113500139684, 1418.531963503440011, 207.2355206635010063 ) ) ;
#56239=ORIENTED_EDGE ( 'NONE', *, *, #18001, .F. ) ;
#56258=FACE_OUTER_BOUND ( 'NONE', #106106, .T. ) ;
#56261=CARTESIAN_POINT ( 'NONE',  ( -15.22583482770000174, 1419.426620482320004, 199.2582349955389986 ) ) ;
#56268=CARTESIAN_POINT ( 'NONE',  ( -16.66297624725529758, 1508.551704407369925, 213.1726019329240103 ) ) ;
#56274=ORIENTED_EDGE ( 'NONE', *, *, #35047, .T. ) ;
#56283=VECTOR ( 'NONE', #22647, 1000.000000000000227 ) ;
#56286=EDGE_CURVE ( 'NONE', #8260, #51946, #108868, .T. ) ;
#56294=CARTESIAN_POINT ( 'NONE',  ( 11.86100282799569960, 1492.894947744830006, 212.5846961511890072 ) ) ;
#56306=DIRECTION ( 'NONE',  ( -0.02616798426450838572, 0.9993150019883944024, -0.02616798426450848286 ) ) ;
#56308=CARTESIAN_POINT ( 'NONE',  ( 10.66733264550000015, 1424.097486430830031, 205.6386333492189920 ) ) ;
#56323=CARTESIAN_POINT ( 'NONE',  ( 9.439522638037985303, 1425.330077423237753, 195.5546044094537876 ) ) ;
#56324=CARTESIAN_POINT ( 'NONE',  ( 2.723688281249999843, 1443.346472895189891, 217.6079121182089864 ) ) ;
#56328=EDGE_CURVE ( 'NONE', #51048, #37552, #37627, .T. ) ;
#56338=CARTESIAN_POINT ( 'NONE',  ( -11.44378878220000040, 1508.484295304989928, 218.0962685049790082 ) ) ;
#56340=EDGE_CURVE ( 'NONE', #98544, #43306, #49091, .T. ) ;
#56341=CARTESIAN_POINT ( 'NONE',  ( 10.82738100200000098, 1427.328250305469965, 209.3702396267119923 ) ) ;
#56346=B_SPLINE_SURFACE_WITH_KNOTS ( 'NONE', 5, 5, ( 
 ( #45629, #78651, #27694, #10332, #71396, #106058 ),
 ( #35534, #44504, #20374, #28802, #88165, #54579 ),
 ( #71946, #105512, #88714, #69729, #3075, #87613 ),
 ( #103847, #11994, #63537, #11453, #55127, #29336 ),
 ( #79216, #1966, #19830, #45073, #89249, #18716 ),
 ( #37202, #80857, #36103, #97653, #20923, #12545 ),
 ( #46723, #46177, #2524, #27147, #80307, #95451 ),
 ( #36646, #37752, #28243, #61880, #70289, #52912 ),
 ( #87044, #104399, #95996, #19265, #53468, #10900 ) ),
 .UNSPECIFIED., .F., .F., .F.,
 ( 6, 3, 6 ),
 ( 6, 6 ),
 ( 8.882670574839030664, 17.48889048929999745, 28.89006134397099856 ),
 ( -0.0006675929709739749978, 2.000000000000000000 ),
 .UNSPECIFIED. ) ;
#56351=CARTESIAN_POINT ( 'NONE',  ( -15.23530766198840247, 1415.677402202029953, 208.5045630004590009 ) ) ;
#56353=FACE_OUTER_BOUND ( 'NONE', #94472, .T. ) ;
#56354=CARTESIAN_POINT ( 'NONE',  ( -18.26023438560000045, 1443.256148476890075, 213.5656046648789754 ) ) ;
#56359=ORIENTED_EDGE ( 'NONE', *, *, #64067, .T. ) ;
#56360=CARTESIAN_POINT ( 'NONE',  ( -11.59590396400000145, 1501.577258705189934, 209.7806602242469864 ) ) ;
#56367=CARTESIAN_POINT ( 'NONE',  ( -3.744312463830716364, 1509.032014876046560, 213.3627910111590325 ) ) ;
#56369=CARTESIAN_POINT ( 'NONE',  ( 9.379383068953968561, 1464.448945081789816, 212.0712950165349753 ) ) ;
#56371=CARTESIAN_POINT ( 'NONE',  ( -1.364625987752019931, 1515.082030188920044, 213.4508433624550037 ) ) ;
#56374=CARTESIAN_POINT ( 'NONE',  ( -11.31069869211509982, 1480.704413556870122, 212.4820440049689978 ) ) ;
#56382=CARTESIAN_POINT ( 'NONE',  ( 24.14616426090000090, 1497.622512133290002, 206.6541300447790093 ) ) ;
#56384=CARTESIAN_POINT ( 'NONE',  ( 0.1569171403356077743, 1473.463532820902628, 219.3464626023122150 ) ) ;
#56390=CARTESIAN_POINT ( 'NONE',  ( -4.816250906239999630, 1456.991639154389986, 217.3233113361989979 ) ) ;
#56401=CARTESIAN_POINT ( 'NONE',  ( -17.63428006580305762, 1419.704475380900021, 206.9647618039389272 ) ) ;
#56410=CARTESIAN_POINT ( 'NONE',  ( -20.87069991009999725, 1506.658021081189872, 214.5368842940590071 ) ) ;
#56414=CARTESIAN_POINT ( 'NONE',  ( -11.15625518848249875, 1488.131838085029813, 191.4014358787470087 ) ) ;
#56427=CARTESIAN_POINT ( 'NONE',  ( 6.020898984694619038, 1441.354597694899894, 215.7047724842319667 ) ) ;
#56431=ORIENTED_EDGE ( 'NONE', *, *, #71701, .T. ) ;
#56447=ORIENTED_EDGE ( 'NONE', *, *, #54906, .T. ) ;
#56453=CARTESIAN_POINT ( 'NONE',  ( -0.3775284373670010352, 1473.627497755890090, 219.3729426502989952 ) ) ;
#56458=EDGE_CURVE ( 'NONE', #81793, #93757, #59505, .T. ) ;
#56462=CARTESIAN_POINT ( 'NONE',  ( -10.91660068633870040, 1470.741030163299911, 210.0515589738539859 ) ) ;
#56463=DIRECTION ( 'NONE',  ( 1.000000000000000000, 2.249639673992789970E-32, 1.224646799147350002E-16 ) ) ;
#56467=CARTESIAN_POINT ( 'NONE',  ( 11.31759557404070016, 1479.526143735280129, 208.6190374719330123 ) ) ;
#56468=EDGE_CURVE ( 'NONE', #1934, #70504, #91420, .T. ) ;
#56470=CARTESIAN_POINT ( 'NONE',  ( -3.888849094689999841, 1441.863784636489981, 201.1563154678690069 ) ) ;
#56472=LINE ( 'NONE', #90604, #60760 ) ;
#56474=CARTESIAN_POINT ( 'NONE',  ( -11.00301372470000061, 1492.094802143589959, 210.0154403701209844 ) ) ;
#56486=CARTESIAN_POINT ( 'NONE',  ( 2.801140078911729780, 1508.551704408389924, 204.1530204508169959 ) ) ;
#56489=CARTESIAN_POINT ( 'NONE',  ( -2.775532924494999776, 1468.867458220450089, 187.4507044347560054 ) ) ;
#56494=CARTESIAN_POINT ( 'NONE',  ( -3.542288683788669790, 1515.375307391110027, 205.1014397700139966 ) ) ;
#56498=CARTESIAN_POINT ( 'NONE',  ( 4.334458048930000196, 1466.050308755590095, 219.2818749650989787 ) ) ;
#56499=CARTESIAN_POINT ( 'NONE',  ( -10.06503061548759881, 1473.016423777250111, 207.3581855507599983 ) ) ;
#56508=ORIENTED_EDGE ( 'NONE', *, *, #83012, .F. ) ;
#56509=EDGE_LOOP ( 'NONE', ( #1604, #74180, #30420, #29815, #83360, #2019, #109312, #85402, #1210, #107345, #28171, #32244 ) ) ;
#56514=CARTESIAN_POINT ( 'NONE',  ( 12.87775475449820028, 1420.952780459589803, 203.1693138811060066 ) ) ;
#56516=CARTESIAN_POINT ( 'NONE',  ( -15.41602167210000118, 1420.398127465669859, 211.2285070405490046 ) ) ;
#56523=CARTESIAN_POINT ( 'NONE',  ( -9.035311967128309973, 1449.310921972689812, 210.7160965195329823 ) ) ;
#56528=CARTESIAN_POINT ( 'NONE',  ( 7.356777505606249434, 1425.075287227600029, 212.5424154620459944 ) ) ;
#56529=AXIS2_PLACEMENT_3D ( 'NONE', #103640, #79555, #53258 ) ;
#56533=CARTESIAN_POINT ( 'NONE',  ( -11.54280425992789993, 1491.460494414069899, 206.8284951956839848 ) ) ;
#56537=CARTESIAN_POINT ( 'NONE',  ( -2.298816249929999778, 1486.462377136390160, 220.8289805357989906 ) ) ;
#56542=CARTESIAN_POINT ( 'NONE',  ( 5.170554601400000116, 1484.055082523290139, 219.7711189574989703 ) ) ;
#56544=CARTESIAN_POINT ( 'NONE',  ( 11.45170634509999985, 1502.273088946489906, 208.2658935923350043 ) ) ;
#56549=EDGE_LOOP ( 'NONE', ( #35762, #1151, #77879, #13361 ) ) ;
#56561=CARTESIAN_POINT ( 'NONE',  ( 8.026143276357348810, 1482.798742743219918, 217.8006291142289967 ) ) ;
#56565=CARTESIAN_POINT ( 'NONE',  ( -10.53746316515110060, 1480.488129968620115, 209.0885347073749756 ) ) ;
#56570=CARTESIAN_POINT ( 'NONE',  ( 19.32263322520000060, 1455.378559704889767, 209.1218459616989946 ) ) ;
#56576=CARTESIAN_POINT ( 'NONE',  ( 10.98521726274509902, 1425.641609558600067, 206.4994411935269909 ) ) ;
#56577=CARTESIAN_POINT ( 'NONE',  ( -9.801729170509650757, 1440.029616514400004, 207.0728283516110082 ) ) ;
#56585=CARTESIAN_POINT ( 'NONE',  ( 9.687496139252409932, 1422.985733114659979, 210.5042674169859822 ) ) ;
#56586=CARTESIAN_POINT ( 'NONE',  ( -15.84429307296400147, 1419.853224566099925, 210.7451948333090002 ) ) ;
#56587=ORIENTED_EDGE ( 'NONE', *, *, #104725, .T. ) ;
#56593=DIRECTION ( 'NONE',  ( 0.06989148164378741757, -0.9716773222564312196, -0.2257395893639560502 ) ) ;
#56595=CARTESIAN_POINT ( 'NONE',  ( 1.676153920926429786, 1456.565163720139935, 199.0597771984899964 ) ) ;
#56597=DIRECTION ( 'NONE',  ( -9.056288633775531119E-47, 1.000000000000000000, -1.836970198721029688E-16 ) ) ;
#56599=CARTESIAN_POINT ( 'NONE',  ( 2.051922892142530319, 1474.778080336890071, 220.3551958197380145 ) ) ;
#56603=PRODUCT_DEFINITION_FORMATION_WITH_SPECIFIED_SOURCE ( 'ANY', '', #14279, .NOT_KNOWN. ) ;
#56608=CARTESIAN_POINT ( 'NONE',  ( -14.65960690603279915, 1417.542028598340039, 203.2496943021490097 ) ) ;
#56620=CARTESIAN_POINT ( 'NONE',  ( -0.6157351208539989518, 1485.064490564490143, 198.2544660199990005 ) ) ;
#56621=CARTESIAN_POINT ( 'NONE',  ( 5.452465356810000330, 1477.448037175989839, 199.6888371653989793 ) ) ;
#56623=CARTESIAN_POINT ( 'NONE',  ( -11.65409527809999979, 1491.241274884490167, 207.0635266648489790 ) ) ;
#56627=CARTESIAN_POINT ( 'NONE',  ( -5.080289282479999002, 1480.093209919690253, 228.8812397303989883 ) ) ;
#56636=FACE_OUTER_BOUND ( 'NONE', #36681, .T. ) ;
#56639=CARTESIAN_POINT ( 'NONE',  ( 11.16766711165429982, 1471.636180864200014, 211.5731661215769748 ) ) ;
#56646=DIRECTION ( 'NONE',  ( 0.000000000000000000, 1.000000000000000000, 0.000000000000000000 ) ) ;
#56647=CARTESIAN_POINT ( 'NONE',  ( -18.28219863529999856, 1466.655046000689936, 217.8387514274990053 ) ) ;
#56649=B_SPLINE_CURVE_WITH_KNOTS ( 'NONE', 1,
 ( #6390, #55717 ),
 .UNSPECIFIED., .F., .F.,
 ( 2, 2 ),
 ( -0.4927803034759909440, 3.525362120492052220 ),
 .UNSPECIFIED. ) ;
#56652=CARTESIAN_POINT ( 'NONE',  ( 20.14625858819999848, 1475.555764171690043, 207.1910292336289672 ) ) ;
#56655=CARTESIAN_POINT ( 'NONE',  ( -18.11269319780000231, 1504.989642490190136, 208.9951304212659977 ) ) ;
#56668=CARTESIAN_POINT ( 'NONE',  ( 11.15438547699999994, 1501.800732394090119, 206.4593492666689940 ) ) ;
#56674=CARTESIAN_POINT ( 'NONE',  ( 2.326513286163319538, 1476.258183507229887, 197.8633931498989966 ) ) ;
#56678=ORIENTED_EDGE ( 'NONE', *, *, #82141, .T. ) ;
#56679=CARTESIAN_POINT ( 'NONE',  ( 16.66442743440000029, 1492.498864364090196, 193.3249227319990098 ) ) ;
#56680=DIRECTION ( 'NONE',  ( 0.000000000000000000, 1.000000000000000000, 0.000000000000000000 ) ) ;
#56688=CIRCLE ( 'NONE', #35173, 11.73448142120001059 ) ;
#56696=CARTESIAN_POINT ( 'NONE',  ( 9.664422427686080397, 1462.605350418599983, 207.8072316276789877 ) ) ;
#56705=CARTESIAN_POINT ( 'NONE',  ( -9.403517712975409282, 1461.589092010630111, 206.6946280230779962 ) ) ;
#56706=B_SPLINE_CURVE_WITH_KNOTS ( 'NONE', 5,
 ( #48702, #20859, #40827, #56544, #75005, #90672, #6118, #66062, #13956, #99613, #48145, #109155 ),
 .UNSPECIFIED., .F., .F.,
 ( 6, 3, 3, 6 ),
 ( -7.762943620309999737, -7.625232449769999477, -3.361916338479999489, -3.182123501529999565 ),
 .UNSPECIFIED. ) ;
#56714=FACE_OUTER_BOUND ( 'NONE', #92580, .T. ) ;
#56717=ORIENTED_EDGE ( 'NONE', *, *, #28161, .T. ) ;
#56719=CARTESIAN_POINT ( 'NONE',  ( -10.01326586723869916, 1481.014341800280135, 205.7823588363200145 ) ) ;
#56723=CARTESIAN_POINT ( 'NONE',  ( -1.637258856660000150, 1483.893433971690001, 198.5669146070989939 ) ) ;
#56727=CARTESIAN_POINT ( 'NONE',  ( 1.871813672400000073, 1508.233053297490187, 220.5554446848989869 ) ) ;
#56736=CARTESIAN_POINT ( 'NONE',  ( -11.12625634799329966, 1482.488446798920222, 206.3854409893099842 ) ) ;
#56738=FACE_OUTER_BOUND ( 'NONE', #34922, .T. ) ;
#56749=CARTESIAN_POINT ( 'NONE',  ( -6.588623528374058402, 1439.966844091445864, 203.3438421578153168 ) ) ;
#56755=CARTESIAN_POINT ( 'NONE',  ( -3.829620175029999629, 1515.551704176389876, 210.9648099296190082 ) ) ;
#56767=CARTESIAN_POINT ( 'NONE',  ( 2.487935142314050108, 1509.038615934839981, 213.6090957367470082 ) ) ;
#56772=CARTESIAN_POINT ( 'NONE',  ( 12.65229159338619880, 1421.485625842520221, 206.6964318454880072 ) ) ;
#56777=CARTESIAN_POINT ( 'NONE',  ( -17.51440058699769864, 1442.103999578969933, 219.2287822569540197 ) ) ;
#56782=CARTESIAN_POINT ( 'NONE',  ( -4.668925449930000582, 1453.940455793189813, 200.5491111697690201 ) ) ;
#56784=CARTESIAN_POINT ( 'NONE',  ( 7.589021600739999762, 1426.918624641610222, 212.4071224751090199 ) ) ;
#56785=VECTOR ( 'NONE', #74109, 1000.000000000000227 ) ;
#56793=ORIENTED_EDGE ( 'NONE', *, *, #49993, .T. ) ;
#56800=CARTESIAN_POINT ( 'NONE',  ( 2.737982081959999814, 1444.818524895790006, 200.5605189733490192 ) ) ;
#56801=CARTESIAN_POINT ( 'NONE',  ( -21.53022416006009720, 1505.950189135809978, 209.2005961044559967 ) ) ;
#56814=FACE_OUTER_BOUND ( 'NONE', #99316, .T. ) ;
#56823=CARTESIAN_POINT ( 'NONE',  ( -12.78494549719999895, 1502.727917388590186, 208.9468085136539912 ) ) ;
#56832=EDGE_CURVE ( 'NONE', #61362, #41878, #27345, .T. ) ;
#56848=CARTESIAN_POINT ( 'NONE',  ( 12.32325568688510131, 1492.223109645010027, 209.7154455344569897 ) ) ;
#56861=CARTESIAN_POINT ( 'NONE',  ( 0.7236364578855678520, 1494.203192619447236, 220.2307484109624909 ) ) ;
#56863=CARTESIAN_POINT ( 'NONE',  ( 11.15048149399999922, 1425.206633195839913, 203.7517032637389889 ) ) ;
#56868=CARTESIAN_POINT ( 'NONE',  ( -1.249673188667893342, 1515.565594798684742, 205.1760501711441691 ) ) ;
#56872=CARTESIAN_POINT ( 'NONE',  ( 10.33096665759340027, 1480.828053585820044, 206.9964859125329895 ) ) ;
#56873=ORIENTED_EDGE ( 'NONE', *, *, #6407, .F. ) ;
#56876=CARTESIAN_POINT ( 'NONE',  ( 10.78336580500200093, 1461.892577084380036, 211.1578546862259884 ) ) ;
#56877=CARTESIAN_POINT ( 'NONE',  ( 9.412160733855756689, 1425.314313998383568, 195.5625766667135395 ) ) ;
#56878=CARTESIAN_POINT ( 'NONE',  ( 0.7253268807889989844, 1442.591808607289977, 218.6790638971189935 ) ) ;
#56880=CARTESIAN_POINT ( 'NONE',  ( 10.99882366966150116, 1470.803487868729917, 192.2106042945659965 ) ) ;
#56882=CARTESIAN_POINT ( 'NONE',  ( 6.857062643409833846, 1486.827203759812164, 200.7504989922479979 ) ) ;
#56884=EDGE_CURVE ( 'NONE', #86968, #53118, #83058, .T. ) ;
#56892=CARTESIAN_POINT ( 'NONE',  ( 11.22682033204820051, 1470.417118964590145, 207.3383776542460168 ) ) ;
#56893=CARTESIAN_POINT ( 'NONE',  ( -5.020870921430000244, 1483.991119631089987, 199.5319357661589947 ) ) ;
#56901=CARTESIAN_POINT ( 'NONE',  ( -17.18726318579999912, 1440.321463842890125, 217.4344804300990290 ) ) ;
#56908=CARTESIAN_POINT ( 'NONE',  ( -11.39916848899999913, 1500.963021451090071, 210.1012423875770025 ) ) ;
#56910=CARTESIAN_POINT ( 'NONE',  ( 5.126901366830000306, 1455.691003689690206, 218.4326852860489794 ) ) ;
#56918=CARTESIAN_POINT ( 'NONE',  ( -5.106893094710000192, 1391.877272790489997, 203.8075142969990168 ) ) ;
#56919=CARTESIAN_POINT ( 'NONE',  ( 9.492563787872798642, 1464.256798853970167, 211.6513489870939964 ) ) ;
#56922=CARTESIAN_POINT ( 'NONE',  ( -0.7783252048265130174, 1515.125841190099891, 213.4496961315290093 ) ) ;
#56923=CARTESIAN_POINT ( 'NONE',  ( -3.271538019026510202, 1454.292002138270163, 199.1638778078030043 ) ) ;
#56934=CARTESIAN_POINT ( 'NONE',  ( -0.1743923092878569836, 1501.248403096799848, 233.2153375875180075 ) ) ;
#56940=CIRCLE ( 'NONE', #26544, 11.73460161499999899 ) ;
#56944=CARTESIAN_POINT ( 'NONE',  ( -4.228037575960000183, 1457.658301557489949, 217.8226702182289785 ) ) ;
#56950=VERTEX_POINT ( 'NONE', #110464 ) ;
#56952=CARTESIAN_POINT ( 'NONE',  ( -8.866734544810560337, 1447.658174592660089, 212.1401281790719793 ) ) ;
#56977=CARTESIAN_POINT ( 'NONE',  ( 4.900781089548089220, 1426.655589109569746, 191.7260386988809842 ) ) ;
#56984=CARTESIAN_POINT ( 'NONE',  ( 7.716990237357959970, 1439.907775640959926, 213.4893468860780104 ) ) ;
#56990=CARTESIAN_POINT ( 'NONE',  ( -11.22397442029999937, 1471.293743228789936, 207.0223102294889941 ) ) ;
#56997=EDGE_CURVE ( 'NONE', #104898, #105852, #72575, .T. ) ;
#57002=EDGE_CURVE ( 'NONE', #50173, #2195, #81868, .T. ) ;
#57016=CARTESIAN_POINT ( 'NONE',  ( -16.43897083077359866, 1508.454179826399923, 213.9817428091590159 ) ) ;
#57017=CARTESIAN_POINT ( 'NONE',  ( 1.396949333800000081, 1473.097534632089946, 219.2356275978989970 ) ) ;
#57028=ORIENTED_EDGE ( 'NONE', *, *, #66126, .T. ) ;
#57029=ORIENTED_EDGE ( 'NONE', *, *, #70627, .F. ) ;
#57030=CARTESIAN_POINT ( 'NONE',  ( -2.487935123034410001, 1508.551704413348716, 213.9802063494123558 ) ) ;
#57032=CARTESIAN_POINT ( 'NONE',  ( -3.463912908579999783, 1443.361677142989947, 200.0971741339589869 ) ) ;
#57033=CARTESIAN_POINT ( 'NONE',  ( 11.81247832421080091, 1501.731194366300087, 211.4919564201209710 ) ) ;
#57036=CARTESIAN_POINT ( 'NONE',  ( 10.60523232130659999, 1422.322173433070020, 211.3613908351649968 ) ) ;
#57037=CARTESIAN_POINT ( 'NONE',  ( -11.00154618500000048, 1492.089968578990010, 210.0309033811119832 ) ) ;
#57046=CARTESIAN_POINT ( 'NONE',  ( -1.008560136250000072, 1456.416633368590055, 218.7046624972589939 ) ) ;
#57050=CARTESIAN_POINT ( 'NONE',  ( -3.739222493130000213, 1474.769836386989937, 198.3144648466990247 ) ) ;
#57055=CARTESIAN_POINT ( 'NONE',  ( -4.329448802989709577, 1515.064791341159889, 206.7919475917079808 ) ) ;
#57057=CARTESIAN_POINT ( 'NONE',  ( 5.597778194180000888, 1506.679269386989972, 219.3685102149989916 ) ) ;
#57059=EDGE_CURVE ( 'NONE', #35548, #21410, #64659, .T. ) ;
#57078=CARTESIAN_POINT ( 'NONE',  ( -15.32768421809999992, 1420.023183193880186, 211.9636741928989920 ) ) ;
#57090=CARTESIAN_POINT ( 'NONE',  ( 7.481606250500309585, 1425.290164852929820, 212.2841966316389914 ) ) ;
#57094=CARTESIAN_POINT ( 'NONE',  ( -6.466996272939999457, 1422.019461440550231, 192.0563668886989888 ) ) ;
#57097=CARTESIAN_POINT ( 'NONE',  ( -19.75056259240000145, 1465.177823603190063, 209.1218459616989946 ) ) ;
#57099=CARTESIAN_POINT ( 'NONE',  ( -4.642747618861698733, 1378.261778813269530, 214.5306460145334313 ) ) ;
#57103=ORIENTED_EDGE ( 'NONE', *, *, #35723, .F. ) ;
#57112=ORIENTED_EDGE ( 'NONE', *, *, #33184, .T. ) ;
#57117=CARTESIAN_POINT ( 'NONE',  ( 4.987078397334300028, 1508.551704408389924, 211.6097676058329853 ) ) ;
#57121=CARTESIAN_POINT ( 'NONE',  ( -6.632177051280000235, 1428.092653318189832, 204.0245593685589824 ) ) ;
#57127=ORIENTED_EDGE ( 'NONE', *, *, #96749, .T. ) ;
#57130=CARTESIAN_POINT ( 'NONE',  ( -2.636066701933580170, 1508.551704408389924, 220.0370691182650091 ) ) ;
#57132=CARTESIAN_POINT ( 'NONE',  ( 7.938530459438009501, 1504.028730547460100, 219.0969020694710139 ) ) ;
#57133=CARTESIAN_POINT ( 'NONE',  ( 12.24199275630000017, 1420.231738084499966, 199.7476432072489843 ) ) ;
#57135=CARTESIAN_POINT ( 'NONE',  ( 19.01172303400000274, 1456.124536704289767, 212.8719163663189988 ) ) ;
#57137=CARTESIAN_POINT ( 'NONE',  ( 10.33130932227850174, 1479.485470067400001, 205.9989652718629713 ) ) ;
#57141=CARTESIAN_POINT ( 'NONE',  ( 12.19798263851669873, 1426.952519236690023, 206.6044100701579680 ) ) ;
#57145=ORIENTED_EDGE ( 'NONE', *, *, #109801, .F. ) ;
#57146=CARTESIAN_POINT ( 'NONE',  ( 16.27172383310000114, 1476.104910058290216, 222.3698031616989965 ) ) ;
#57150=B_SPLINE_SURFACE_WITH_KNOTS ( 'NONE', 5, 5, ( 
 ( #98049, #108104, #73426, #81248, #89654, #65023 ),
 ( #72334, #20784, #4563, #54984, #22418, #106464 ),
 ( #21323, #31400, #38697, #96978, #107008, #30296 ),
 ( #14036, #20241, #64489, #56621, #54442, #88576 ),
 ( #98604, #21868, #46032, #56067, #90194, #13478 ),
 ( #48227, #82367, #47668, #81796, #5098, #40904 ),
 ( #110316, #59391, #57740, #41475, #42565, #49876 ),
 ( #8395, #91313, #66689, #42020, #33590, #75084 ),
 ( #84009, #33051, #7310, #91859, #24624, #15134 ) ),
 .UNSPECIFIED., .F., .F., .F.,
 ( 6, 3, 6 ),
 ( 6, 6 ),
 ( 13.60177910350000019, 23.50904048570000171, 33.41630186789999613 ),
 ( 0.000000000000000000, 2.000000000000000000 ),
 .UNSPECIFIED. ) ;
#57152=CARTESIAN_POINT ( 'NONE',  ( 10.14203510082409920, 1422.829087935100006, 209.7690348518279961 ) ) ;
#57153=CARTESIAN_POINT ( 'NONE',  ( 11.07868621362170103, 1422.904854153429824, 203.3190901071859855 ) ) ;
#57155=CARTESIAN_POINT ( 'NONE',  ( 1.398091756599999957, 1429.447055348990034, 217.3181151331990009 ) ) ;
#57158=CARTESIAN_POINT ( 'NONE',  ( -16.75075978319999948, 1417.136094290510073, 208.0073609310889822 ) ) ;
#57160=CARTESIAN_POINT ( 'NONE',  ( -17.54272989919999759, 1417.931783365949968, 206.8684744458689977 ) ) ;
#57165=CARTESIAN_POINT ( 'NONE',  ( 9.267170318294839504, 1460.193123049920132, 205.0415981645240038 ) ) ;
#57172=CARTESIAN_POINT ( 'NONE',  ( -20.61932039460000254, 1486.434366909889832, 211.1021073309690053 ) ) ;
#57173=FACE_OUTER_BOUND ( 'NONE', #31042, .T. ) ;
#57175=FACE_OUTER_BOUND ( 'NONE', #26516, .T. ) ;
#57187=ORIENTED_EDGE ( 'NONE', *, *, #106350, .T. ) ;
#57191=CARTESIAN_POINT ( 'NONE',  ( -12.25773961910000054, 1490.408449763890076, 209.0370346857240236 ) ) ;
#57193=CARTESIAN_POINT ( 'NONE',  ( -4.992349863779999453, 1391.620913471789891, 214.4361776263990009 ) ) ;
#57195=CIRCLE ( 'NONE', #46482, 9.341369339569999042 ) ;
#57196=CARTESIAN_POINT ( 'NONE',  ( 8.482142651180000215, 1423.325760005520124, 211.9865074947389871 ) ) ;
#57200=CARTESIAN_POINT ( 'NONE',  ( -9.200421138165051360, 1422.937291722789951, 210.7384568321920142 ) ) ;
#57201=CARTESIAN_POINT ( 'NONE',  ( -4.958796112629440422, 1508.551704408389924, 206.2486321841020072 ) ) ;
#57215=DIRECTION ( 'NONE',  ( 0.4826573169212934888, -0.01052729488162659072, -0.8757460193942152582 ) ) ;
#57216=CARTESIAN_POINT ( 'NONE',  ( -9.792514563870629019, 1462.664719234569930, 228.0127671146719877 ) ) ;
#57234=CARTESIAN_POINT ( 'NONE',  ( -1.104917627860029894, 1486.166445081519896, 220.9774509037769974 ) ) ;
#57241=AXIS2_PLACEMENT_3D ( 'NONE', #8862, #79828, #58736 ) ;
#57243=DIRECTION ( 'NONE',  ( -9.066331650111889066E-17, 1.000000000000000000, -7.714096702464409664E-17 ) ) ;
#57247=PRODUCT_DEFINITION_SHAPE ( 'NONE', 'NONE',  #61723 ) ;
#57251=CARTESIAN_POINT ( 'NONE',  ( 22.24401587272570069, 1475.958667601430079, 209.7631782834160106 ) ) ;
#57255=EDGE_LOOP ( 'NONE', ( #49125, #49237, #107922, #85294 ) ) ;
#57259=CARTESIAN_POINT ( 'NONE',  ( -2.330134118790000208, 1515.551704408389924, 212.9514660756190096 ) ) ;
#57279=CARTESIAN_POINT ( 'NONE',  ( -4.329448776040000446, 1515.064792882589927, 211.4519800877889963 ) ) ;
#57280=CARTESIAN_POINT ( 'NONE',  ( 8.212347910089999203, 1503.127208973789948, 210.4119479190490267 ) ) ;
#57288=CARTESIAN_POINT ( 'NONE',  ( 3.535327679399999923, 1487.160995988090008, 197.6951163675990131 ) ) ;
#57290=B_SPLINE_SURFACE_WITH_KNOTS ( 'NONE', 5, 5, ( 
 ( #12184, #29003, #54226, #86689, #35183, #9983 ),
 ( #28446, #53678, #95645, #53111, #45819, #80509 ),
 ( #52555, #18913, #44153, #37399, #103477, #62640 ),
 ( #78289, #88353, #63189, #1603, #11641, #35740 ),
 ( #79952, #54766, #18361, #44713, #79407, #2718 ),
 ( #78865, #26782, #20566, #61518, #46377, #3269 ),
 ( #60970, #71598, #69927, #95095, #104040, #105719 ),
 ( #27332, #87248, #87820, #36286, #36841, #71033 ),
 ( #70478, #96201, #104598, #27892, #62075, #19476 ) ),
 .UNSPECIFIED., .F., .F., .F.,
 ( 6, 3, 6 ),
 ( 6, 6 ),
 ( 3.013370279934989959, 5.176304934450000061, 7.339239588965010164 ),
 ( -1.897240500978929716E-05, 2.000000000000000000 ),
 .UNSPECIFIED. ) ;
#57298=CARTESIAN_POINT ( 'NONE',  ( 3.368571795365570054, 1515.551842517600107, 212.9003862705719996 ) ) ;
#57301=CARTESIAN_POINT ( 'NONE',  ( -12.35342891082190064, 1501.830731195820135, 211.5811800714079993 ) ) ;
#57307=CARTESIAN_POINT ( 'NONE',  ( -5.010111490926330013, 1441.342207431860061, 201.8184694356190221 ) ) ;
#57310=CARTESIAN_POINT ( 'NONE',  ( -9.360712814986960950, 1480.861369530930006, 227.8151877844180149 ) ) ;
#57317=CARTESIAN_POINT ( 'NONE',  ( 10.89207644999670066, 1489.857914366469913, 208.0657199684020213 ) ) ;
#57319=CARTESIAN_POINT ( 'NONE',  ( 3.111939779091150271, 1454.307961065650034, 217.9820244081379883 ) ) ;
#57325=CARTESIAN_POINT ( 'NONE',  ( 9.722206599239999747, 1428.114070706089933, 212.2005358146490153 ) ) ;
#57327=CARTESIAN_POINT ( 'NONE',  ( -4.217994498519999524, 1515.470302801990101, 209.8638807055999962 ) ) ;
#57328=VECTOR ( 'NONE', #23146, 999.9999999999998863 ) ;
#57335=CARTESIAN_POINT ( 'NONE',  ( -8.178330991719999332, 1439.186084948589951, 206.0664693636589959 ) ) ;
#57346=CARTESIAN_POINT ( 'NONE',  ( 12.91341498353999917, 1421.147458452220235, 204.5103631683240337 ) ) ;
#57351=CARTESIAN_POINT ( 'NONE',  ( -13.05162051234070120, 1467.538720776440186, 191.8992815354449988 ) ) ;
#57359=CARTESIAN_POINT ( 'NONE',  ( 7.517994368920000170, 1425.903866193129943, 212.2671131861389995 ) ) ;
#57362=CARTESIAN_POINT ( 'NONE',  ( -21.60434909035369699, 1417.942671029680014, 208.5651389465070054 ) ) ;
#57366=EDGE_LOOP ( 'NONE', ( #7301, #37476, #103557, #74274, #20976, #5178, #95192, #12185, #17095 ) ) ;
#57374=CARTESIAN_POINT ( 'NONE',  ( 2.925585596869999527, 1446.021080118789996, 199.8385306598290185 ) ) ;
#57378=CARTESIAN_POINT ( 'NONE',  ( -4.875278699166510243, 1464.496074833199827, 199.2309655485080100 ) ) ;
#57379=CARTESIAN_POINT ( 'NONE',  ( -17.19445149659999572, 1417.679469902730034, 207.4067394929689954 ) ) ;
#57389=CARTESIAN_POINT ( 'NONE',  ( -16.53125420670000167, 1418.541487540729804, 202.7561987471289910 ) ) ;
#57396=CARTESIAN_POINT ( 'NONE',  ( -8.998910544736714812, 1424.786834349990158, 213.7129700835037909 ) ) ;
#57398=ADVANCED_FACE ( 'NONE', ( #110616 ), #87432, .F. ) ;
#57401=ORIENTED_EDGE ( 'NONE', *, *, #36296, .T. ) ;
#57404=CARTESIAN_POINT ( 'NONE',  ( -8.320045427150200013, 1452.334357641350152, 204.9523858405019894 ) ) ;
#57405=EDGE_CURVE ( 'NONE', #4789, #37845, #101877, .T. ) ;
#57409=ORIENTED_EDGE ( 'NONE', *, *, #52057, .T. ) ;
#57421=CARTESIAN_POINT ( 'NONE',  ( 9.438883731854119219, 1434.537705308250224, 206.5784376637019761 ) ) ;
#57433=CARTESIAN_POINT ( 'NONE',  ( 11.90565451390000007, 1426.735011702260181, 206.1879629638889924 ) ) ;
#57439=CARTESIAN_POINT ( 'NONE',  ( 0.3104492304326414986, 1515.598602702714061, 205.0832592253421751 ) ) ;
#57446=CARTESIAN_POINT ( 'NONE',  ( 8.390996307492248008, 1424.412614569296466, 195.8273022863984067 ) ) ;
#57447=CARTESIAN_POINT ( 'NONE',  ( -0.6587146994840009651, 1442.893519126590036, 219.0943606518089837 ) ) ;
#57464=CARTESIAN_POINT ( 'NONE',  ( -9.536809216310290438, 1439.025537637410025, 209.1065069698359764 ) ) ;
#57465=CARTESIAN_POINT ( 'NONE',  ( 1.901515396933940005, 1494.834309937820080, 220.2474388463949992 ) ) ;
#57477=CARTESIAN_POINT ( 'NONE',  ( -11.42922335639999964, 1500.819224853989908, 209.0445494132570161 ) ) ;
#57481=CARTESIAN_POINT ( 'NONE',  ( -3.677001408430000229, 1443.877114344990105, 218.5311880179489776 ) ) ;
#57483=CYLINDRICAL_SURFACE ( 'NONE', #48131, 3.750000000000000000 ) ;
#57484=CARTESIAN_POINT ( 'NONE',  ( 9.643555441329038302, 1463.923096898180120, 210.9171137617960028 ) ) ;
#57493=EDGE_LOOP ( 'NONE', ( #11132, #48847, #27552, #63567 ) ) ;
#57496=CARTESIAN_POINT ( 'NONE',  ( -0.2450088331967839872, 1500.853325256900007, 233.1959501652279982 ) ) ;
#57498=CARTESIAN_POINT ( 'NONE',  ( -2.413383470617591620, 1474.356824845931897, 219.0989264923542521 ) ) ;
#57500=AXIS2_PLACEMENT_3D ( 'NONE', #41543, #101970, #58895 ) ;
#57505=CARTESIAN_POINT ( 'NONE',  ( -3.542891930950000212, 1457.744368643689995, 218.3958059026789726 ) ) ;
#57508=ORIENTED_EDGE ( 'NONE', *, *, #26859, .T. ) ;
#57509=CARTESIAN_POINT ( 'NONE',  ( -4.329294185584100063, 1515.070696454100016, 210.6909417500819757 ) ) ;
#57517=CARTESIAN_POINT ( 'NONE',  ( -17.64826220104147581, 1419.426078558765312, 207.1977041188345083 ) ) ;
#57535=CARTESIAN_POINT ( 'NONE',  ( 1.842963219480119985, 1515.064792700640055, 213.4512947425059792 ) ) ;
#57540=CARTESIAN_POINT ( 'NONE',  ( 6.042571514009714484, 1460.034219164688011, 201.6114123766374462 ) ) ;
#57542=CARTESIAN_POINT ( 'NONE',  ( 7.994156842015020636, 1438.386042044900250, 214.3897529291720048 ) ) ;
#57548=CARTESIAN_POINT ( 'NONE',  ( -8.809027987900540424, 1438.685400005079828, 208.2563316356740017 ) ) ;
#57557=CARTESIAN_POINT ( 'NONE',  ( 6.340491506960000301, 1486.594081419090116, 200.3538830581090053 ) ) ;
#57570=CARTESIAN_POINT ( 'NONE',  ( 0.6932908832194439874, 1423.656777452399865, 191.1977553446599813 ) ) ;
#57572=CARTESIAN_POINT ( 'NONE',  ( -3.990972504867622117, 1508.152871093448766, 220.6701910291383797 ) ) ;
#57574=CARTESIAN_POINT ( 'NONE',  ( 0.07025850623888389712, 1455.755685241430001, 198.5793256795659829 ) ) ;
#57575=CARTESIAN_POINT ( 'NONE',  ( -4.270716396233116718, 1515.320037055801777, 210.9648094544856178 ) ) ;
#57577=CARTESIAN_POINT ( 'NONE',  ( -11.25747325112660135, 1470.382999096749927, 210.8897107907189934 ) ) ;
#57578=CARTESIAN_POINT ( 'NONE',  ( 4.327403558811209194, 1515.142896577510101, 208.5979656133399942 ) ) ;
#57582=CARTESIAN_POINT ( 'NONE',  ( 8.565021413077344548, 1438.455202895904222, 210.8457856774827803 ) ) ;
#57585=CARTESIAN_POINT ( 'NONE',  ( -5.303263976000000213, 1442.879268891389984, 200.5942805944989971 ) ) ;
#57586=CARTESIAN_POINT ( 'NONE',  ( 8.228876175890000866, 1424.472806264060182, 195.8277277863990093 ) ) ;
#57587=B_SPLINE_CURVE_WITH_KNOTS ( 'NONE', 5,
 ( #91693, #14969, #102290, #93339, #32881, #101177 ),
 .UNSPECIFIED., .F., .F.,
 ( 6, 6 ),
 ( 496.9173868270000298, 501.6444997780000108 ),
 .UNSPECIFIED. ) ;
#57588=CARTESIAN_POINT ( 'NONE',  ( -2197.008826411130485, 11216.44053380570767, 1944.533671213028583 ) ) ;
#57592=EDGE_CURVE ( 'NONE', #43913, #94111, #19195, .T. ) ;
#57596=CARTESIAN_POINT ( 'NONE',  ( -12.49544828328139978, 1502.589285090969952, 208.9951533569199853 ) ) ;
#57598=CARTESIAN_POINT ( 'NONE',  ( 11.40015074134580075, 1491.987826722599948, 210.4762200410769992 ) ) ;
#57600=CARTESIAN_POINT ( 'NONE',  ( -3.179033953939999879, 1457.997354107289993, 219.3203918675989996 ) ) ;
#57602=CARTESIAN_POINT ( 'NONE',  ( 4.873735476160000246, 1472.089320948289924, 218.0431589096889695 ) ) ;
#57604=B_SPLINE_CURVE_WITH_KNOTS ( 'NONE', 5,
 ( #93715, #92626, #51756, #93177, #16447, #84228, #84773, #263, #78042 ),
 .UNSPECIFIED., .F., .F.,
 ( 6, 3, 6 ),
 ( -13.00939335640000039, -6.504696678220000194, 0.000000000000000000 ),
 .UNSPECIFIED. ) ;
#57607=CARTESIAN_POINT ( 'NONE',  ( 4.804127539630909105, 1508.551704408389924, 205.6959211417370170 ) ) ;
#57611=CARTESIAN_POINT ( 'NONE',  ( -4.138326088228239996, 1515.492270357839971, 206.7919250756299903 ) ) ;
#57612=CARTESIAN_POINT ( 'NONE',  ( -11.87908931286030167, 1481.928125358580019, 208.8953011241800084 ) ) ;
#57614=CARTESIAN_POINT ( 'NONE',  ( 11.77367730374300159, 1479.442738960109864, 208.9990535504570062 ) ) ;
#57618=CARTESIAN_POINT ( 'NONE',  ( -15.16921353568702102, 1420.050152274720858, 212.3982990353912328 ) ) ;
#57626=ORIENTED_EDGE ( 'NONE', *, *, #5898, .T. ) ;
#57639=CARTESIAN_POINT ( 'NONE',  ( 3.406450987864870328, 1507.508084575899829, 220.3277226881679951 ) ) ;
#57640=CARTESIAN_POINT ( 'NONE',  ( 3.959152859930000101, 1428.396642669490120, 216.3690266601789745 ) ) ;
#57641=CARTESIAN_POINT ( 'NONE',  ( -3.648559762950000174, 1443.531551953690041, 199.7293442341890000 ) ) ;
#57647=CARTESIAN_POINT ( 'NONE',  ( 7.506537366674529643, 1425.371641708889911, 212.2338419592690002 ) ) ;
#57673=CARTESIAN_POINT ( 'NONE',  ( 4.410752497883399847, 1508.610338626970133, 212.9872707138450210 ) ) ;
#57679=ORIENTED_EDGE ( 'NONE', *, *, #74922, .F. ) ;
#57680=CARTESIAN_POINT ( 'NONE',  ( -3.220674668504990290, 1433.265634988960073, 218.1214075394389909 ) ) ;
#57682=CARTESIAN_POINT ( 'NONE',  ( 7.605328049712762883, 1479.456294567033865, 201.8411987916495889 ) ) ;
#57684=CARTESIAN_POINT ( 'NONE',  ( -10.47977169157950073, 1480.135362529120130, 210.0653170854480152 ) ) ;
#57687=CARTESIAN_POINT ( 'NONE',  ( 9.054615469453679566, 1503.552526581200027, 218.0929084609520032 ) ) ;
#57688=CARTESIAN_POINT ( 'NONE',  ( 7.403717961100000799, 1422.895866474680133, 195.5966881380989832 ) ) ;
#57690=CARTESIAN_POINT ( 'NONE',  ( -8.429455138962469007, 1493.667170337469997, 200.1551273359310130 ) ) ;
#57691=CARTESIAN_POINT ( 'NONE',  ( 10.03076429248900148, 1480.391079390540199, 205.9105066912069617 ) ) ;
#57694=DIRECTION ( 'NONE',  ( 4.657277648632380671E-10, -1.836970198721029688E-16, -1.000000000000000000 ) ) ;
#57699=ORIENTED_EDGE ( 'NONE', *, *, #261, .F. ) ;
#57705=CARTESIAN_POINT ( 'NONE',  ( 9.089240498862510620, 1424.967503372909960, 209.7705479972250089 ) ) ;
#57706=CARTESIAN_POINT ( 'NONE',  ( 11.73306708689199951, 1421.776606475200197, 203.4167027637400338 ) ) ;
#57715=EDGE_CURVE ( 'NONE', #100441, #61012, #71708, .T. ) ;
#57717=CARTESIAN_POINT ( 'NONE',  ( 8.605022022878770827, 1464.162231465259993, 214.7347089345799986 ) ) ;
#57718=CARTESIAN_POINT ( 'NONE',  ( -10.97570570419999925, 1482.624300662889937, 205.8415957027289949 ) ) ;
#57719=CARTESIAN_POINT ( 'NONE',  ( 2.098165248435849950, 1474.766810392649859, 220.3465733394599795 ) ) ;
#57722=CARTESIAN_POINT ( 'NONE',  ( 15.66262490570000132, 1454.743832497789981, 196.6949010879989999 ) ) ;
#57724=CARTESIAN_POINT ( 'NONE',  ( 1.486478317020000217, 1515.456929490889934, 204.9468604023890066 ) ) ;
#57727=CARTESIAN_POINT ( 'NONE',  ( -9.104803375611409066, 1421.479062203829926, 192.1853131441990001 ) ) ;
#57731=VERTEX_POINT ( 'NONE', #11749 ) ;
#57740=CARTESIAN_POINT ( 'NONE',  ( 9.336549371730001212, 1479.069783892889973, 203.8813761292790048 ) ) ;
#57743=CARTESIAN_POINT ( 'NONE',  ( 0.1712571669960009924, 1463.663764520790210, 202.0829161578890023 ) ) ;
#57746=CARTESIAN_POINT ( 'NONE',  ( -17.54272989919999759, 1417.931783365949968, 206.8684744458689977 ) ) ;
#57751=CARTESIAN_POINT ( 'NONE',  ( 11.18429024643810088, 1422.356073855499972, 207.3872344669040331 ) ) ;
#57759=CARTESIAN_POINT ( 'NONE',  ( 4.475229445540000128, 1473.172248456590069, 218.4600389222289891 ) ) ;
#57760=CARTESIAN_POINT ( 'NONE',  ( 11.03246124568249975, 1471.772754036200013, 212.1253387598690097 ) ) ;
#57763=FACE_OUTER_BOUND ( 'NONE', #25199, .T. ) ;
#57768=CARTESIAN_POINT ( 'NONE',  ( 7.875427937609998708, 1449.003968285089968, 202.2333506183190082 ) ) ;
#57775=EDGE_CURVE ( 'NONE', #7587, #9541, #91223, .T. ) ;
#57776=CARTESIAN_POINT ( 'NONE',  ( -1.551161424019060098, 1463.265709907049995, 199.4650991780359846 ) ) ;
#57781=VERTEX_POINT ( 'NONE', #57639 ) ;
#57783=CARTESIAN_POINT ( 'NONE',  ( 12.67382636239999982, 1500.337692531689981, 208.3527651524340172 ) ) ;
#57789=CARTESIAN_POINT ( 'NONE',  ( 10.35181298299999852, 1478.133428305090092, 203.4857779180190107 ) ) ;
#57790=CARTESIAN_POINT ( 'NONE',  ( 12.65062378175580093, 1500.863489648990026, 210.3581148444430085 ) ) ;
#57791=CARTESIAN_POINT ( 'NONE',  ( 4.987078416198220232, 1508.551704408389924, 211.6097810847190033 ) ) ;
#57794=CARTESIAN_POINT ( 'NONE',  ( -21.59687355579729839, 1507.523430265019897, 209.4572628990989926 ) ) ;
#57799=CARTESIAN_POINT ( 'NONE',  ( 10.39188998415169962, 1453.184289048810115, 211.2438860691320031 ) ) ;
#57803=CARTESIAN_POINT ( 'NONE',  ( 2.330134126090001701, 1515.320037165148278, 204.8511296415418599 ) ) ;
#57819=CARTESIAN_POINT ( 'NONE',  ( -3.586377584040013833, 1515.071394843999997, 213.2045508750898364 ) ) ;
#57830=ORIENTED_EDGE ( 'NONE', *, *, #95886, .F. ) ;
#57837=CARTESIAN_POINT ( 'NONE',  ( -11.93094903640050042, 1501.580206583630115, 211.4284354873250038 ) ) ;
#57841=EDGE_CURVE ( 'NONE', #42229, #25915, #61886, .T. ) ;
#57843=CARTESIAN_POINT ( 'NONE',  ( -0.2348491764560019790, 1435.893188924790138, 227.6464390018990116 ) ) ;
#57844=CARTESIAN_POINT ( 'NONE',  ( -6.176626807815939202, 1440.736226183980079, 202.7885005142740056 ) ) ;
#57849=CARTESIAN_POINT ( 'NONE',  ( -10.01325982467770004, 1481.014320843050200, 205.7823435180839908 ) ) ;
#57851=ORIENTED_EDGE ( 'NONE', *, *, #11225, .F. ) ;
#57860=CARTESIAN_POINT ( 'NONE',  ( -15.58996755230000097, 1417.047973859700051, 206.0392561205590027 ) ) ;
#57864=CARTESIAN_POINT ( 'NONE',  ( -8.643932593178378809, 1437.446544997869978, 208.6934462458000041 ) ) ;
#57880=CARTESIAN_POINT ( 'NONE',  ( -2.469737631213410278, 1507.227429411520006, 221.7265308815400147 ) ) ;
#57883=CARTESIAN_POINT ( 'NONE',  ( 12.46461103178539886, 1421.611150248099875, 207.4535745979419801 ) ) ;
#57884=CARTESIAN_POINT ( 'NONE',  ( 10.10911558311959979, 1480.122050019980179, 206.2115462197010061 ) ) ;
#57888=CARTESIAN_POINT ( 'NONE',  ( 7.755379691283469157, 1459.738853292250042, 228.9106028236209909 ) ) ;
#57893=CARTESIAN_POINT ( 'NONE',  ( -4.267145232369999874, 1453.908306873689980, 199.9833667514089939 ) ) ;
#57899=CARTESIAN_POINT ( 'NONE',  ( -22.72857882966620124, 1417.467434011349951, 209.9112631640360007 ) ) ;
#57914=CARTESIAN_POINT ( 'NONE',  ( 0.1168726624490010052, 1443.529164943789965, 200.1804741532190235 ) ) ;
#57927=ORIENTED_EDGE ( 'NONE', *, *, #59785, .F. ) ;
#57933=CARTESIAN_POINT ( 'NONE',  ( -6.960528455329999531, 1472.781863690589944, 209.0507852043539856 ) ) ;
#57935=ORIENTED_EDGE ( 'NONE', *, *, #48738, .T. ) ;
#57936=CARTESIAN_POINT ( 'NONE',  ( -12.78943259969999957, 1502.708798733090134, 209.0180537489830215 ) ) ;
#57943=CARTESIAN_POINT ( 'NONE',  ( -7.000175857517819900, 1453.642846852349976, 202.9077934395569969 ) ) ;
#57947=ORIENTED_EDGE ( 'NONE', *, *, #18770, .T. ) ;
#57956=CARTESIAN_POINT ( 'NONE',  ( 3.074703527060000052, 1441.333178254290033, 218.5515148082390056 ) ) ;
#57960=CARTESIAN_POINT ( 'NONE',  ( -13.96267725510150193, 1502.379640760292432, 226.3091245870000989 ) ) ;
#57965=B_SPLINE_CURVE_WITH_KNOTS ( 'NONE', 5,
 ( #40033, #91544, #82025, #13701, #14268, #83684, #82597, #32735, #66915, #83144, #74215, #50108, #65803, #23218, #14821, #24322, #15908, #49008, #40584, #66369, #57956 ),
 .UNSPECIFIED., .F., .F.,
 ( 6, 3, 3, 3, 3, 3, 6 ),
 ( 0.000000000000000000, 0.3516404420329832248, 0.7013045389776026983, 0.8764775333732340856, 0.9202713844326411152, 0.9640652354931900092, 1.000000000000000000 ),
 .UNSPECIFIED. ) ;
#57969=CARTESIAN_POINT ( 'NONE',  ( 5.033939915584520364, 1484.257078321549898, 219.3935248400869966 ) ) ;
#57980=CARTESIAN_POINT ( 'NONE',  ( 19.60792669039999936, 1475.100271358290229, 204.3343059087790152 ) ) ;
#57984=CARTESIAN_POINT ( 'NONE',  ( -5.064702160787156515, 1462.535433854306575, 200.7801777857700074 ) ) ;
#57998=CARTESIAN_POINT ( 'NONE',  ( -8.542608682037007739, 1440.192411897979810, 205.6891261743860184 ) ) ;
#58004=CARTESIAN_POINT ( 'NONE',  ( -8.838558338096110134, 1438.385153647559946, 208.8793219489340061 ) ) ;
#58005=CARTESIAN_POINT ( 'NONE',  ( -2.958096254149490623, 1515.068899375750107, 213.4512612264969960 ) ) ;
#58009=CARTESIAN_POINT ( 'NONE',  ( -9.661041455239748998, 1460.496751011739889, 209.0910779832980211 ) ) ;
#58010=CARTESIAN_POINT ( 'NONE',  ( -2.586254832189999853, 1431.686802707190054, 214.1917715140089911 ) ) ;
#58015=EDGE_CURVE ( 'NONE', #70504, #7001, #73957, .T. ) ;
#58016=ORIENTED_EDGE ( 'NONE', *, *, #28969, .T. ) ;
#58020=CARTESIAN_POINT ( 'NONE',  ( 2.419279911200000299, 1454.975743091090180, 218.2344084821389743 ) ) ;
#58026=CARTESIAN_POINT ( 'NONE',  ( 6.826200034800000260, 1424.874072630889941, 213.4902541782590220 ) ) ;
#58028=CARTESIAN_POINT ( 'NONE',  ( -3.516555726533699744, 1454.164898032659949, 199.2503824040580014 ) ) ;
#58036=CARTESIAN_POINT ( 'NONE',  ( 13.97509019449999812, 1500.690698309590061, 227.7022812698990037 ) ) ;
#58044=CARTESIAN_POINT ( 'NONE',  ( 10.01013843233299916, 1469.369181467840008, 209.9819040969830155 ) ) ;
#58055=CARTESIAN_POINT ( 'NONE',  ( -8.630493275741649484, 1448.198865873919885, 212.2264116289769902 ) ) ;
#58056=CARTESIAN_POINT ( 'NONE',  ( 0.000000000000000000, 1420.119835273649869, 209.1218459616989946 ) ) ;
#58064=ORIENTED_EDGE ( 'NONE', *, *, #108035, .T. ) ;
#58071=CARTESIAN_POINT ( 'NONE',  ( -19.49652697766560294, 1485.947961896859852, 201.9289638760380114 ) ) ;
#58075=CARTESIAN_POINT ( 'NONE',  ( 18.79226589730000185, 1456.307606824690083, 213.7887498653890077 ) ) ;
#58077=CARTESIAN_POINT ( 'NONE',  ( 2.588573091324529951, 1426.130607012579958, 191.2585785401599878 ) ) ;
#58081=CARTESIAN_POINT ( 'NONE',  ( 4.689995948910178569, 1459.453669361078482, 200.6829600737077044 ) ) ;
#58083=CARTESIAN_POINT ( 'NONE',  ( 9.130434922834639977, 1437.290822646750030, 212.9268152338410118 ) ) ;
#58084=LINE ( 'NONE', #92217, #46792 ) ;
#58087=VERTEX_POINT ( 'NONE', #2994 ) ;
#58089=CARTESIAN_POINT ( 'NONE',  ( -10.74194912529999968, 1471.560973568090049, 206.8675636587589963 ) ) ;
#58092=ORIENTED_EDGE ( 'NONE', *, *, #85721, .F. ) ;
#58099=CARTESIAN_POINT ( 'NONE',  ( 5.823572337359999906, 1487.975078907890065, 198.5964445195989754 ) ) ;
#58103=CARTESIAN_POINT ( 'NONE',  ( -16.27770732761305794, 1446.651107274472906, 198.7459790681657807 ) ) ;
#58108=CARTESIAN_POINT ( 'NONE',  ( -16.76029352119999771, 1420.475925714450113, 203.3596836330289932 ) ) ;
#58110=B_SPLINE_CURVE_WITH_KNOTS ( 'NONE', 5,
 ( #11713, #104113, #80021, #3342, #63254, #97362 ),
 .UNSPECIFIED., .F., .F.,
 ( 6, 6 ),
 ( -0.5000000000000000000, 0.000000000000000000 ),
 .UNSPECIFIED. ) ;
#58111=CARTESIAN_POINT ( 'NONE',  ( -3.523962717220000318, 1476.511731497689880, 220.0526012939989755 ) ) ;
#58114=CARTESIAN_POINT ( 'NONE',  ( -11.17593228934340033, 1471.359546453119947, 206.7956388744609910 ) ) ;
#58115=CARTESIAN_POINT ( 'NONE',  ( -7.106047323496611945, 1508.384870682446717, 219.7310283353839111 ) ) ;
#58118=DIRECTION ( 'NONE',  ( 0.02616798426500960631, 0.9993150019883682011, 0.02616798426500950570 ) ) ;
#58120=CARTESIAN_POINT ( 'NONE',  ( -10.64861439574930024, 1470.416444257950161, 211.6181901305839972 ) ) ;
#58124=EDGE_LOOP ( 'NONE', ( #99315, #41082, #26727, #68899 ) ) ;
#58128=CARTESIAN_POINT ( 'NONE',  ( 11.36216713388179933, 1503.110266152410077, 211.0233809544849919 ) ) ;
#58132=CARTESIAN_POINT ( 'NONE',  ( 1.657045479016600042, 1508.551704408389924, 219.7501937159020144 ) ) ;
#58138=CARTESIAN_POINT ( 'NONE',  ( -8.589426147275000645, 1436.798469860880004, 209.9038450004319998 ) ) ;
#58139=CARTESIAN_POINT ( 'NONE',  ( 10.93677888065239934, 1490.434389039140115, 209.9320082733399886 ) ) ;
#58140=CARTESIAN_POINT ( 'NONE',  ( -3.084094934559999945, 1457.182013509390117, 218.2582506311690054 ) ) ;
#58146=VERTEX_POINT ( 'NONE', #86411 ) ;
#58149=CARTESIAN_POINT ( 'NONE',  ( -4.136749811987540326, 1515.492902828930028, 206.2237479538289904 ) ) ;
#58151=CARTESIAN_POINT ( 'NONE',  ( -2.723255399910000207, 1468.839623697090019, 189.3038879039989979 ) ) ;
#58152=CARTESIAN_POINT ( 'NONE',  ( 11.72068719049280006, 1479.848144395859890, 210.3626758944340054 ) ) ;
#58156=CARTESIAN_POINT ( 'NONE',  ( -8.519142658073340257, 1508.551704408389924, 218.7985387068179932 ) ) ;
#58160=CARTESIAN_POINT ( 'NONE',  ( -1.636741614903409969, 1469.777368438049962, 219.0527109355280118 ) ) ;
#58167=CARTESIAN_POINT ( 'NONE',  ( -19.27355791249999939, 1467.813399981289876, 204.3088842694490097 ) ) ;
#58170=CARTESIAN_POINT ( 'NONE',  ( 1.422097314359999976, 1477.081575188689840, 198.6901653669989969 ) ) ;
#58172=AXIS2_PLACEMENT_3D ( 'NONE', #68385, #2293, #86811 ) ;
#58175=CARTESIAN_POINT ( 'NONE',  ( 2.393091348901930093, 1429.053683011190060, 217.0555866711269744 ) ) ;
#58176=CARTESIAN_POINT ( 'NONE',  ( -8.742754168010000271, 1424.489613839150024, 206.0336725849989818 ) ) ;
#58177=ADVANCED_FACE ( 'NONE', ( #44429 ), #37392, .F. ) ;
#58182=CARTESIAN_POINT ( 'NONE',  ( 7.516502869536429543, 1425.414971123999749, 212.2146689648959921 ) ) ;
#58205=CARTESIAN_POINT ( 'NONE',  ( 4.554948888541289875, 1508.731372606449895, 211.6097697255310095 ) ) ;
#58206=ORIENTED_EDGE ( 'NONE', *, *, #10589, .F. ) ;
#58209=VECTOR ( 'NONE', #74408, 1000.000000000000000 ) ;
#58217=CARTESIAN_POINT ( 'NONE',  ( -0.9122102915526030253, 1444.513817941259958, 199.1093392106390070 ) ) ;
#58218=CARTESIAN_POINT ( 'NONE',  ( 1.282760155569999894, 1429.107748742090052, 214.5111769290890038 ) ) ;
#58220=CARTESIAN_POINT ( 'NONE',  ( -10.41578227499199905, 1479.949469769299867, 210.5455296413880149 ) ) ;
#58223=EDGE_CURVE ( 'NONE', #3165, #42483, #79320, .T. ) ;
#58225=CARTESIAN_POINT ( 'NONE',  ( 10.74159879227639891, 1502.696702000269852, 215.9649088173380278 ) ) ;
#58226=CARTESIAN_POINT ( 'NONE',  ( 8.209570662930000040, 1421.454114719120298, 196.1494337501989946 ) ) ;
#58227=CARTESIAN_POINT ( 'NONE',  ( -0.6675760093930949157, 1432.097311422259963, 218.6006162758970106 ) ) ;
#58228=CARTESIAN_POINT ( 'NONE',  ( -5.061893406920000338, 1495.006295643590192, 197.8849625455989951 ) ) ;
#58240=CARTESIAN_POINT ( 'NONE',  ( 11.41293808157470124, 1427.618755674339809, 209.6356236935340007 ) ) ;
#58243=CARTESIAN_POINT ( 'NONE',  ( 10.95522075352049995, 1424.091714785270142, 203.1699306280349901 ) ) ;
#58244=CARTESIAN_POINT ( 'NONE',  ( -10.89732850212739912, 1462.760389868430138, 207.2746260999839762 ) ) ;
#58249=CARTESIAN_POINT ( 'NONE',  ( -9.662959447710280259, 1460.558442627200066, 208.8701083130750078 ) ) ;
#58255=CARTESIAN_POINT ( 'NONE',  ( 4.647650363794389783, 1467.200465736529850, 217.9234417945369842 ) ) ;
#58257=CARTESIAN_POINT ( 'NONE',  ( 5.095760143028649658, 1474.009471786559970, 219.3429060835489963 ) ) ;
#58258=CARTESIAN_POINT ( 'NONE',  ( -4.487249770485409961, 1509.038615931769982, 206.6339108289169815 ) ) ;
#58263=CARTESIAN_POINT ( 'NONE',  ( -4.992349863779999453, 1391.620913471789891, 203.8075142969990168 ) ) ;
#58264=CARTESIAN_POINT ( 'NONE',  ( 5.140094623760980141, 1436.845495186209973, 228.7442485543419934 ) ) ;
#58273=ORIENTED_EDGE ( 'NONE', *, *, #77232, .F. ) ;
#58278=CARTESIAN_POINT ( 'NONE',  ( 19.52205534611780280, 1473.076231017440023, 204.3554433243390065 ) ) ;
#58282=CARTESIAN_POINT ( 'NONE',  ( 3.829620113550000315, 1515.551704408389924, 210.9648081929590262 ) ) ;
#58285=CARTESIAN_POINT ( 'NONE',  ( 10.64684366344270039, 1425.854810616539908, 207.2965554390950160 ) ) ;
#58291=ORIENTED_EDGE ( 'NONE', *, *, #81136, .T. ) ;
#58293=B_SPLINE_CURVE_WITH_KNOTS ( 'NONE', 5,
 ( #69659, #43336, #109975, #784, #11926, #79148 ),
 .UNSPECIFIED., .F., .F.,
 ( 6, 6 ),
 ( 434.5419185690000177, 439.7519038140000021 ),
 .UNSPECIFIED. ) ;
#58302=CARTESIAN_POINT ( 'NONE',  ( 10.34950180350000082, 1451.639534145589778, 207.2650128738690114 ) ) ;
#58305=CARTESIAN_POINT ( 'NONE',  ( -0.0007469751400547060965, 1455.736088183790116, 198.5579702233989963 ) ) ;
#58314=CARTESIAN_POINT ( 'NONE',  ( -17.53532366528470021, 1417.850058971930139, 206.8376673564200132 ) ) ;
#58315=ORIENTED_EDGE ( 'NONE', *, *, #82542, .F. ) ;
#58331=CARTESIAN_POINT ( 'NONE',  ( -9.838224505759999516, 1462.268909614690074, 227.9668215275989667 ) ) ;
#58338=CARTESIAN_POINT ( 'NONE',  ( -5.668982378084499452, 1507.922364110239869, 220.7207090108649936 ) ) ;
#58339=CARTESIAN_POINT ( 'NONE',  ( -16.88207931438999765, 1507.985365216929949, 209.4467744516990138 ) ) ;
#58340=CARTESIAN_POINT ( 'NONE',  ( 3.984081752360000284, 1515.551704408389924, 210.9648081929590262 ) ) ;
#58346=FACE_OUTER_BOUND ( 'NONE', #21496, .T. ) ;
#58359=CARTESIAN_POINT ( 'NONE',  ( -10.37041358865520024, 1462.696929687640022, 206.9223858279979993 ) ) ;
#58362=CARTESIAN_POINT ( 'NONE',  ( -10.74194911459999879, 1471.560973731990089, 206.8675634873690115 ) ) ;
#58363=CARTESIAN_POINT ( 'NONE',  ( -10.62228157299999864, 1490.415513672490079, 212.3812309668689977 ) ) ;
#58369=DIRECTION ( 'NONE',  ( -1.305148739725796033E-31, 1.000000000000000000, -1.836970198721029688E-16 ) ) ;
#58373=CARTESIAN_POINT ( 'NONE',  ( -4.378216884482949212, 1453.707746088449994, 199.6107954155660025 ) ) ;
#58377=CARTESIAN_POINT ( 'NONE',  ( 3.829164872245370166, 1515.551704201149960, 211.4518032850860152 ) ) ;
#58379=CARTESIAN_POINT ( 'NONE',  ( -11.72416936767639939, 1501.387581424680093, 211.3308819256019717 ) ) ;
#58380=ORIENTED_EDGE ( 'NONE', *, *, #98330, .T. ) ;
#58387=CARTESIAN_POINT ( 'NONE',  ( -8.316672828268760753, 1425.055149638239982, 204.9623390585310005 ) ) ;
#58391=CARTESIAN_POINT ( 'NONE',  ( -10.26804317657019894, 1481.277325295010087, 206.6051681627829737 ) ) ;
#58392=CARTESIAN_POINT ( 'NONE',  ( -4.018690540569999747, 1470.826407316289988, 215.3451084216990239 ) ) ;
#58401=CARTESIAN_POINT ( 'NONE',  ( 2.395226819458120104, 1454.514303657540040, 218.2121819530340190 ) ) ;
#58404=CARTESIAN_POINT ( 'NONE',  ( -15.01368523340000216, 1416.900385880339854, 204.9748714204190208 ) ) ;
#58406=CARTESIAN_POINT ( 'NONE',  ( -3.594043688008891291, 1496.396823991950669, 219.7606401984895967 ) ) ;
#58407=CARTESIAN_POINT ( 'NONE',  ( -15.89250414441243464, 1419.836041960068769, 210.6346457996376955 ) ) ;
#58412=CARTESIAN_POINT ( 'NONE',  ( -11.95661960621089825, 1507.899396442559919, 208.5587272349789885 ) ) ;
#58422=CARTESIAN_POINT ( 'NONE',  ( 4.290508147089998836, 1515.379315998089851, 208.7552087591940051 ) ) ;
#58423=DIRECTION ( 'NONE',  ( -8.832268201338159945E-47, 1.000000000000000000, -1.836970198721029688E-16 ) ) ;
#58430=CARTESIAN_POINT ( 'NONE',  ( -19.86701999479999969, 1444.364638085089837, 213.3580800903289969 ) ) ;
#58432=CARTESIAN_POINT ( 'NONE',  ( 14.17511108698380085, 1428.761363100300059, 195.0897028359609919 ) ) ;
#58434=LINE ( 'NONE', #93118, #64749 ) ;
#58435=FACE_OUTER_BOUND ( 'NONE', #6474, .T. ) ;
#58437=CARTESIAN_POINT ( 'NONE',  ( 8.129906402815519684, 1449.255237000160150, 202.7301597656260128 ) ) ;
#58454=CARTESIAN_POINT ( 'NONE',  ( -1.551161424019060098, 1463.265709907049995, 199.4650991780359846 ) ) ;
#58456=CARTESIAN_POINT ( 'NONE',  ( 3.912776123226219926, 1515.493282983300105, 205.6567928634579800 ) ) ;
#58457=CARTESIAN_POINT ( 'NONE',  ( 1.236701001219999929, 1445.191800647990021, 199.4886538942189986 ) ) ;
#58464=( NAMED_UNIT ( * ) PLANE_ANGLE_UNIT ( ) SI_UNIT ( $, .RADIAN. ) );
#58465=CARTESIAN_POINT ( 'NONE',  ( 8.134874095680000750, 1436.133436978890131, 226.1977348306990336 ) ) ;
#58480=EDGE_LOOP ( 'NONE', ( #43489, #5408, #108509, #76093, #13122 ) ) ;
#58481=CARTESIAN_POINT ( 'NONE',  ( -11.60962210859999821, 1502.036214399190158, 208.5035594193370230 ) ) ;
#58496=CARTESIAN_POINT ( 'NONE',  ( -16.03794089777630205, 1508.551704408389924, 210.3786724331339997 ) ) ;
#58505=CARTESIAN_POINT ( 'NONE',  ( 12.32608557850170072, 1492.201684892610047, 209.6317255076330071 ) ) ;
#58510=CARTESIAN_POINT ( 'NONE',  ( 0.000000000000000000, 1377.913060387289988, 209.1218459616989946 ) ) ;
#58516=CARTESIAN_POINT ( 'NONE',  ( 1.481577638361565530, 1494.010533848515024, 220.1478854846517947 ) ) ;
#58520=CARTESIAN_POINT ( 'NONE',  ( 0.2227148572559347062, 1444.496034457048154, 218.0821367963589239 ) ) ;
#58533=CARTESIAN_POINT ( 'NONE',  ( 10.95575241281549950, 1461.178150784580112, 209.3116150371660069 ) ) ;
#58535=CARTESIAN_POINT ( 'NONE',  ( -7.557465101040457434, 1461.895601300565204, 203.0080691329112881 ) ) ;
#58536=CARTESIAN_POINT ( 'NONE',  ( 4.440234083720000058, 1466.830466837689983, 218.1566789410989884 ) ) ;
#58549=CARTESIAN_POINT ( 'NONE',  ( 736.9598419237370308, 11220.04953453921007, 2047.362669009807405 ) ) ;
#58554=CARTESIAN_POINT ( 'NONE',  ( -8.724201986094810124, 1437.633551000330044, 210.3037638580349835 ) ) ;
#58555=CARTESIAN_POINT ( 'NONE',  ( -3.829222816047260114, 1515.551704203360032, 211.9228904752730216 ) ) ;
#58560=CARTESIAN_POINT ( 'NONE',  ( -4.660393612750000081, 1436.848553822789881, 227.0391165213990234 ) ) ;
#58568=CARTESIAN_POINT ( 'NONE',  ( 4.492546581380000958, 1453.878649273890005, 217.3453973181289882 ) ) ;
#58570=CARTESIAN_POINT ( 'NONE',  ( -7.499365986679999985, 1445.290603318090007, 216.2717625584189989 ) ) ;
#58574=CIRCLE ( 'NONE', #103224, 11.73843354579999954 ) ;
#58576=CARTESIAN_POINT ( 'NONE',  ( 7.308867546920000180, 1424.255848919720165, 212.7423161441389823 ) ) ;
#58578=CARTESIAN_POINT ( 'NONE',  ( -3.580429133039419565, 1454.131615231540081, 199.2738294499930021 ) ) ;
#58584=ORIENTED_EDGE ( 'NONE', *, *, #86267, .F. ) ;
#58586=CARTESIAN_POINT ( 'NONE',  ( 0.07276018598029700135, 1502.631145669490024, 233.2831920997990096 ) ) ;
#58588=CARTESIAN_POINT ( 'NONE',  ( -2.261284126934287819, 1474.298250304425210, 219.1320758864328013 ) ) ;
#58592=CARTESIAN_POINT ( 'NONE',  ( 9.944339257881379623, 1468.659659235959907, 207.9255319265940045 ) ) ;
#58595=CARTESIAN_POINT ( 'NONE',  ( -9.880950594389059205, 1447.806469747649999, 210.0498174535929934 ) ) ;
#58604=DIRECTION ( 'NONE',  ( 0.001041802705676860138, 1.836969201840314816E-16, 0.9999994573234139983 ) ) ;
#58606=CARTESIAN_POINT ( 'NONE',  ( 0.7564154366205578794, 1432.638783478930009, 200.7115661240650013 ) ) ;
#58610=VERTEX_POINT ( 'NONE', #10949 ) ;
#58613=EDGE_CURVE ( 'NONE', #19377, #39608, #97700, .T. ) ;
#58621=CARTESIAN_POINT ( 'NONE',  ( 12.67629937430701936, 1426.478869958664063, 202.7079000866955028 ) ) ;
#58630=CARTESIAN_POINT ( 'NONE',  ( -3.887263819049999736, 1491.372323727890034, 188.5673907495989852 ) ) ;
#58636=CARTESIAN_POINT ( 'NONE',  ( -8.834982911374369863, 1438.486838626130066, 208.6720045421899954 ) ) ;
#58642=CARTESIAN_POINT ( 'NONE',  ( -6.998115108689999531, 1413.756493170500107, 208.1001205746590017 ) ) ;
#58644=CARTESIAN_POINT ( 'NONE',  ( 4.403123731590000034, 1485.794562715689835, 199.2936768241389984 ) ) ;
#58645=CARTESIAN_POINT ( 'NONE',  ( 2.149719450999330039, 1431.090543968449992, 218.3651844143140011 ) ) ;
#58655=CARTESIAN_POINT ( 'NONE',  ( -17.28042313459999946, 1420.187471544980099, 203.7977315272489989 ) ) ;
#58657=CARTESIAN_POINT ( 'NONE',  ( -2.568249187049999716, 1475.995101164990047, 219.8900349392989995 ) ) ;
#58661=LINE ( 'NONE', #74918, #108594 ) ;
#58662=CARTESIAN_POINT ( 'NONE',  ( -5.016006900679014002, 1508.231295651743494, 220.4176492183756579 ) ) ;
#58667=CARTESIAN_POINT ( 'NONE',  ( -10.93690819593899910, 1470.800486576299818, 209.7884454878060012 ) ) ;
#58668=CARTESIAN_POINT ( 'NONE',  ( 1.180034279919999873, 1492.152004741890096, 188.0782235167989995 ) ) ;
#58674=CARTESIAN_POINT ( 'NONE',  ( -5.062152673029999939, 1439.003726787289906, 206.7420654048690096 ) ) ;
#58679=CARTESIAN_POINT ( 'NONE',  ( 9.357015822218050616, 1422.633417228330018, 212.8722094221120074 ) ) ;
#58684=VECTOR ( 'NONE', #63431, 1000.000000000000114 ) ;
#58687=CARTESIAN_POINT ( 'NONE',  ( 12.20128992515689959, 1492.563683748890071, 211.0969524153320265 ) ) ;
#58688=CARTESIAN_POINT ( 'NONE',  ( -3.286480964850000408, 1456.341185808290220, 218.0120306903490075 ) ) ;
#58700=CARTESIAN_POINT ( 'NONE',  ( -9.276944363820000206, 1461.680301575389876, 206.2489193930190083 ) ) ;
#58703=CARTESIAN_POINT ( 'NONE',  ( -11.16643436200000039, 1471.372555910990059, 206.7508257863089796 ) ) ;
#58705=CARTESIAN_POINT ( 'NONE',  ( -2.777756275229999794, 1456.209068913490000, 202.9659093387089968 ) ) ;
#58708=CARTESIAN_POINT ( 'NONE',  ( 3.212856134899739757, 1433.121553999790194, 201.2044923049280101 ) ) ;
#58716=CARTESIAN_POINT ( 'NONE',  ( -12.86990655680000017, 1502.949917638090028, 208.7255105242149682 ) ) ;
#58718=CARTESIAN_POINT ( 'NONE',  ( -2.424815126019999934, 1477.020009817290202, 199.0133905605989924 ) ) ;
#58723=CARTESIAN_POINT ( 'NONE',  ( 0.7162863658319988946, 1429.709265593189912, 217.4063670190490143 ) ) ;
#58724=CARTESIAN_POINT ( 'NONE',  ( -8.316701203199999171, 1425.055152618780085, 204.9623575238389890 ) ) ;
#58728=CARTESIAN_POINT ( 'NONE',  ( 7.492432155504880065, 1426.008877190969770, 212.3388350879999962 ) ) ;
#58732=CARTESIAN_POINT ( 'NONE',  ( -11.39217826018909996, 1491.610218127549842, 206.8972610507499894 ) ) ;
#58734=CARTESIAN_POINT ( 'NONE',  ( -0.7950140742365245927, 1488.007107121973604, 219.9546037614996123 ) ) ;
#58736=DIRECTION ( 'NONE',  ( -1.000000000000000000, 0.000000000000000000, 0.000000000000000000 ) ) ;
#58738=CARTESIAN_POINT ( 'NONE',  ( 4.932967056419999885, 1425.220831261190142, 209.6856336174119804 ) ) ;
#58742=CARTESIAN_POINT ( 'NONE',  ( 10.01433737459999840, 1462.389872936090114, 210.8954339908790132 ) ) ;
#58750=CIRCLE ( 'NONE', #64137, 8.800000000000000711 ) ;
#58752=CARTESIAN_POINT ( 'NONE',  ( 3.137390382537029954, 1508.729448375579977, 213.6787528850110220 ) ) ;
#58757=CARTESIAN_POINT ( 'NONE',  ( -3.707800473929999896, 1428.659817224090148, 200.9450977274489674 ) ) ;
#58762=CARTESIAN_POINT ( 'NONE',  ( 1.365811584579660121, 1445.431647728280041, 199.1348593500399886 ) ) ;
#58765=CARTESIAN_POINT ( 'NONE',  ( -11.76331255911069995, 1481.397599341149999, 210.5790801447900265 ) ) ;
#58769=DIRECTION ( 'NONE',  ( 9.056288633775531119E-47, -1.000000000000000000, 1.836970198721029688E-16 ) ) ;
#58771=CARTESIAN_POINT ( 'NONE',  ( 8.299847678909999971, 1421.312374491559922, 196.1635037195989923 ) ) ;
#58772=CARTESIAN_POINT ( 'NONE',  ( 0.5913408061856150200, 1431.617811701200026, 218.5945621063530098 ) ) ;
#58773=LINE ( 'NONE', #32469, #84133 ) ;
#58784=DIRECTION ( 'NONE',  ( -1.000000000000000000, 0.000000000000000000, 0.000000000000000000 ) ) ;
#58786=CARTESIAN_POINT ( 'NONE',  ( 8.663868365875391220, 1423.279983291419967, 211.7948421327720041 ) ) ;
#58787=CARTESIAN_POINT ( 'NONE',  ( 12.41549622805439945, 1426.345760381200080, 202.7472225575059781 ) ) ;
#58796=CARTESIAN_POINT ( 'NONE',  ( 12.14135103133349958, 1420.978590117220165, 201.7400648282489897 ) ) ;
#58797=CARTESIAN_POINT ( 'NONE',  ( 6.072417058032599790, 1467.015289949989892, 217.0523006129610053 ) ) ;
#58805=CARTESIAN_POINT ( 'NONE',  ( -1.842963808589999974, 1515.492058141890084, 204.9833025469089876 ) ) ;
#58806=CARTESIAN_POINT ( 'NONE',  ( -5.215016241880452874, 1391.913060387290443, 203.8075142969990168 ) ) ;
#58807=CARTESIAN_POINT ( 'NONE',  ( -19.34949478396210054, 1446.106506027710111, 200.0047807539029918 ) ) ;
#58808=CARTESIAN_POINT ( 'NONE',  ( -16.56680993899979981, 1420.259233108609806, 206.2549788483950124 ) ) ;
#58824=CARTESIAN_POINT ( 'NONE',  ( 18.18716276245509889, 1472.405785144279889, 200.2358052267980213 ) ) ;
#58833=CARTESIAN_POINT ( 'NONE',  ( 12.02790215590800038, 1427.361711468500062, 208.2118097891859918 ) ) ;
#58838=CARTESIAN_POINT ( 'NONE',  ( 2.280774907361240000, 1437.403108797190043, 227.5229878108619914 ) ) ;
#58839=VERTEX_POINT ( 'NONE', #45121 ) ;
#58840=CARTESIAN_POINT ( 'NONE',  ( 3.962210237229999432, 1474.305345705389982, 219.8526279916989949 ) ) ;
#58845=CARTESIAN_POINT ( 'NONE',  ( -10.99857202889999996, 1492.065341454889904, 207.0970296734990086 ) ) ;
#58852=CARTESIAN_POINT ( 'NONE',  ( 9.146237109299999446, 1449.998848175489911, 208.1168068839089926 ) ) ;
#58865=ORIENTED_EDGE ( 'NONE', *, *, #3599, .T. ) ;
#58884=CARTESIAN_POINT ( 'NONE',  ( -1.482599699759999945, 1431.767369128790051, 203.5535557080689841 ) ) ;
#58886=CARTESIAN_POINT ( 'NONE',  ( -4.244621079450020318, 1507.604642859460000, 221.2803215189360060 ) ) ;
#58887=CARTESIAN_POINT ( 'NONE',  ( -15.31725463369030038, 1507.984504716529955, 209.4225156325090040 ) ) ;
#58888=CARTESIAN_POINT ( 'NONE',  ( 4.217997304759999899, 1515.470303964289997, 209.8638434859140034 ) ) ;
#58890=CARTESIAN_POINT ( 'NONE',  ( -5.331678975189100278, 1454.863890310829902, 201.3635607548650057 ) ) ;
#58895=DIRECTION ( 'NONE',  ( 0.9824080081115887930, -2.243614313870717968E-31, 0.1867471702549210744 ) ) ;
#58902=CARTESIAN_POINT ( 'NONE',  ( 18.95766226850000180, 1454.628370232990164, 205.4382105502989759 ) ) ;
#58903=TOROIDAL_SURFACE ( 'NONE', #16021, 6.646318662569999702, 0.5000000000000000000 ) ;
#58905=ORIENTED_EDGE ( 'NONE', *, *, #44015, .T. ) ;
#58909=CARTESIAN_POINT ( 'NONE',  ( -2.330134127310790060, 1515.064792882719985, 213.4512947379739956 ) ) ;
#58910=CARTESIAN_POINT ( 'NONE',  ( -2.031407857746849732, 1468.162645372460020, 219.6586981276110180 ) ) ;
#58912=CARTESIAN_POINT ( 'NONE',  ( 10.20064331328789997, 1469.553217653640104, 207.2979568099669905 ) ) ;
#58914=CARTESIAN_POINT ( 'NONE',  ( -11.28649141220000018, 1489.673453124989919, 212.4368142099590102 ) ) ;
#58917=CARTESIAN_POINT ( 'NONE',  ( -20.74020547129999770, 1505.489868768189808, 209.1669152150809907 ) ) ;
#58919=CARTESIAN_POINT ( 'NONE',  ( 0.000000000000000000, 1378.013060387289897, 209.1218459616989946 ) ) ;
#58926=CARTESIAN_POINT ( 'NONE',  ( 5.517786218439999502, 1505.096896727989815, 220.1774552607989790 ) ) ;
#58928=CARTESIAN_POINT ( 'NONE',  ( -11.47725681950860022, 1501.043658996279873, 211.1773061387589792 ) ) ;
#58931=CARTESIAN_POINT ( 'NONE',  ( 0.7858030238929989419, 1508.037196299090056, 220.8608535643990081 ) ) ;
#58934=CARTESIAN_POINT ( 'NONE',  ( -10.98475441868929892, 1462.126042464299871, 210.0219236981780000 ) ) ;
#58935=CARTESIAN_POINT ( 'NONE',  ( -18.49530585604750144, 1445.106360394780040, 205.2817505082109903 ) ) ;
#58936=CARTESIAN_POINT ( 'NONE',  ( -6.708171328076900863, 1426.565319743190003, 202.6435997773789950 ) ) ;
#58940=CARTESIAN_POINT ( 'NONE',  ( -19.25698220359180368, 1504.759393713030022, 209.4658869119480187 ) ) ;
#58949=CARTESIAN_POINT ( 'NONE',  ( 2.200196402067729817, 1454.568881740520055, 218.2638029879659882 ) ) ;
#58951=CARTESIAN_POINT ( 'NONE',  ( -16.65376728669999906, 1508.454796204690183, 213.7212179624189901 ) ) ;
#58952=CARTESIAN_POINT ( 'NONE',  ( -14.34171585720000053, 1416.291316961129951, 203.4717140614689868 ) ) ;
#58960=CARTESIAN_POINT ( 'NONE',  ( -11.25663888305209959, 1508.421392267890042, 207.6010232658840096 ) ) ;
#58963=CARTESIAN_POINT ( 'NONE',  ( -18.82774374539999940, 1444.049758829389930, 210.0174085047549966 ) ) ;
#58969=B_SPLINE_SURFACE_WITH_KNOTS ( 'NONE', 5, 5, ( 
 ( #49860, #39800, #100253, #83994, #65010, #21855 ),
 ( #73960, #75620, #82894, #57724, #90742, #40888 ),
 ( #108650, #64475, #81781, #15120, #73411, #75070 ),
 ( #109218, #14022, #32504, #24069, #13463, #47653 ),
 ( #5083, #108090, #65566, #30283, #98590, #90180 ),
 ( #39234, #107547, #48213, #99677, #22968, #95164 ),
 ( #77270, #568, #68332, #26285, #68885, #101320 ),
 ( #1121, #102986, #42548, #12, #51504, #34147 ),
 ( #17310, #18421, #103551, #58805, #102439, #8937 ) ),
 .UNSPECIFIED., .F., .F., .F.,
 ( 6, 3, 6 ),
 ( 6, 6 ),
 ( 2.324858856900000159, 4.970096098089999970, 7.657659708029999734 ),
 ( 0.000000000000000000, 0.5000000000000000000 ),
 .UNSPECIFIED. ) ;
#58972=CARTESIAN_POINT ( 'NONE',  ( 12.17073519972539941, 1499.730396604210000, 205.6506567772970016 ) ) ;
#58973=ADVANCED_FACE ( 'NONE', ( #93686 ), #68071, .T. ) ;
#58976=ADVANCED_FACE ( 'NONE', ( #97036 ), #33146, .T. ) ;
#58978=CARTESIAN_POINT ( 'NONE',  ( 3.445653300429999621, 1486.078848993990050, 219.3336973419989988 ) ) ;
#58983=CARTESIAN_POINT ( 'NONE',  ( -6.076016477482709455, 1450.645068205029929, 208.7037722137420133 ) ) ;
#58985=CARTESIAN_POINT ( 'NONE',  ( -19.86464702156969864, 1441.435616204289772, 212.6459227002919761 ) ) ;
#58987=CARTESIAN_POINT ( 'NONE',  ( 13.52268460241299941, 1497.923627544540068, 227.8730058996700052 ) ) ;
#58989=CARTESIAN_POINT ( 'NONE',  ( -2.487934962309999776, 1508.551704408389924, 204.1347675205190058 ) ) ;
#58996=B_SPLINE_CURVE_WITH_KNOTS ( 'NONE', 3,
 ( #50803, #58114, #66529, #92247, #25021, #109068, #59224, #101178, #33993, #41302, #32350, #68186, #32882, #100633, #23919, #15517, #49714, #51347, #83846, #6040, #40192, #76547, #7145, #16606, #75475, #16068, #109608, #67073, #25574, #24473, #8226, #40742, #59768, #102291, #50271, #31786, #42392 ),
 .UNSPECIFIED., .F., .F.,
 ( 4, 3, 3, 3, 3, 3, 3, 3, 3, 3, 3, 3, 4 ),
 ( -7.474718202020000035, -7.256328811620320174, -6.989423022925070228, -6.695085830317820452, -6.368123258945879606, -5.921286250405219498, -5.573260391803679603, -5.269658889521529943, -5.196602558778829817, -4.761443928031699357, -4.253228966541860778, -3.623072494495270579, -3.064599166389999851 ),
 .UNSPECIFIED. ) ;
#59015=CARTESIAN_POINT ( 'NONE',  ( 3.329657646939999438, 1445.620183030290036, 200.6158394109289986 ) ) ;
#59020=CARTESIAN_POINT ( 'NONE',  ( 2.864776410889999791, 1467.969787444489839, 218.6984507715789903 ) ) ;
#59022=SURFACE_SIDE_STYLE ('',( #16417 ) ) ;
#59036=CARTESIAN_POINT ( 'NONE',  ( -10.07154918488590134, 1473.228065907060000, 207.4129428866500007 ) ) ;
#59040=CARTESIAN_POINT ( 'NONE',  ( -11.43590621159999898, 1501.508488288289982, 208.4755739533859753 ) ) ;
#59051=CARTESIAN_POINT ( 'NONE',  ( 4.163336342339999869E-15, 1416.177402202029953, 209.1218459616989946 ) ) ;
#59052=ORIENTED_EDGE ( 'NONE', *, *, #56997, .T. ) ;
#59059=CARTESIAN_POINT ( 'NONE',  ( 4.637787270109999582, 1462.124489585889933, 228.1829287868989979 ) ) ;
#59066=CARTESIAN_POINT ( 'NONE',  ( -11.86685402762820019, 1482.064906951660078, 208.4268465260890082 ) ) ;
#59071=VECTOR ( 'NONE', #78009, 1000.000000000000000 ) ;
#59072=B_SPLINE_SURFACE_WITH_KNOTS ( 'NONE', 5, 5, ( 
 ( #30480, #64668, #47842, #5283, #39439, #31028 ),
 ( #99322, #77462, #51155, #9689, #67423, #92584 ),
 ( #85851, #42201, #68523, #76352, #69081, #764 ),
 ( #24275, #93674, #110501, #58456, #109415, #33781 ),
 ( #67978, #50603, #34893, #60680, #9150, #102085 ),
 ( #25368, #93141, #100980, #94806, #101522, #32691 ) ),
 .UNSPECIFIED., .F., .F., .F.,
 ( 6, 6 ),
 ( 6, 6 ),
 ( 5.893388375706040350, 9.819929736133959253 ),
 ( 0.000000000000000000, 0.5002947206939659663 ),
 .UNSPECIFIED. ) ;
#59075=B_SPLINE_CURVE_WITH_KNOTS ( 'NONE', 5,
 ( #3448, #37578, #71780, #35372, #103680, #26980 ),
 .UNSPECIFIED., .F., .F.,
 ( 6, 6 ),
 ( 297.9944221590000097, 302.8993106099999864 ),
 .UNSPECIFIED. ) ;
#59078=CARTESIAN_POINT ( 'NONE',  ( -19.18813880309999931, 1465.797355387890093, 204.3301597990889888 ) ) ;
#59091=CARTESIAN_POINT ( 'NONE',  ( -1.194268154760000034, 1444.571194286590071, 218.0071140876989944 ) ) ;
#59099=CARTESIAN_POINT ( 'NONE',  ( 3.927179831460580139, 1507.318492355100034, 220.1472266827140061 ) ) ;
#59100=CARTESIAN_POINT ( 'NONE',  ( -1.073559340110749938, 1444.993510080170154, 218.0402162255370229 ) ) ;
#59107=CONICAL_SURFACE ( 'NONE', #73402, 6.911399307709998219, 0.04363323129990067523 ) ;
#59113=CARTESIAN_POINT ( 'NONE',  ( -4.020406191785280470, 1515.375307391110027, 212.6641346454879908 ) ) ;
#59126=ORIENTED_EDGE ( 'NONE', *, *, #68000, .F. ) ;
#59127=CARTESIAN_POINT ( 'NONE',  ( -0.6255756489468429216, 1435.976707381580127, 227.5909497020410015 ) ) ;
#59128=CARTESIAN_POINT ( 'NONE',  ( -14.93598579144041416, 1416.108359274850045, 205.2289421662831330 ) ) ;
#59129=CARTESIAN_POINT ( 'NONE',  ( 1.326715741870000187, 1454.806610190989886, 218.4390638076189930 ) ) ;
#59131=CARTESIAN_POINT ( 'NONE',  ( -1.591562321820000125, 1443.444047077889991, 218.6175910282489951 ) ) ;
#59136=CARTESIAN_POINT ( 'NONE',  ( 7.566081195099999768, 1424.291034983149984, 212.3491042945289848 ) ) ;
#59138=CARTESIAN_POINT ( 'NONE',  ( -4.251240061320140207, 1453.776278923900236, 199.5516788180739809 ) ) ;
#59146=ORIENTED_EDGE ( 'NONE', *, *, #89094, .F. ) ;
#59147=CARTESIAN_POINT ( 'NONE',  ( -2.140641997699999965, 1508.551704408389924, 220.0635241299990241 ) ) ;
#59150=DIRECTION ( 'NONE',  ( -0.9412234725396940727, 0.02592281343750019867, -0.3367883348392645138 ) ) ;
#59154=CARTESIAN_POINT ( 'NONE',  ( -0.4328695768656839471, 1475.687559908960111, 197.6741279352499987 ) ) ;
#59157=DIRECTION ( 'NONE',  ( -7.436362843295819681E-17, 1.000000000000000000, -1.457576885956999882E-16 ) ) ;
#59161=CARTESIAN_POINT ( 'NONE',  ( -4.327511837212590251, 1515.138761592190122, 209.7121513359620337 ) ) ;
#59167=CARTESIAN_POINT ( 'NONE',  ( 7.982669098950510467, 1424.960829083689987, 194.4768953556059898 ) ) ;
#59172=CARTESIAN_POINT ( 'NONE',  ( -9.702212350455228673, 1471.555838493580040, 212.0786635793400023 ) ) ;
#59181=CARTESIAN_POINT ( 'NONE',  ( -10.14857146045310010, 1472.086425147420186, 209.7191475320900054 ) ) ;
#59183=VERTEX_POINT ( 'NONE', #76772 ) ;
#59187=CARTESIAN_POINT ( 'NONE',  ( -8.922475182707978902, 1440.999127764592004, 204.4963557433056565 ) ) ;
#59194=CARTESIAN_POINT ( 'NONE',  ( 4.492546581380000958, 1453.878649273890005, 217.3453973181289882 ) ) ;
#59198=CARTESIAN_POINT ( 'NONE',  ( -10.13245368019999937, 1472.295917692089915, 207.1576018941290158 ) ) ;
#59201=CARTESIAN_POINT ( 'NONE',  ( 10.95098205620359977, 1471.837422849929908, 212.3987392730099657 ) ) ;
#59205=CARTESIAN_POINT ( 'NONE',  ( -12.35910314799999909, 1415.406472713659923, 208.4697927874989887 ) ) ;
#59207=CARTESIAN_POINT ( 'NONE',  ( 3.889852026509999838, 1485.593720051389937, 199.0907241709990103 ) ) ;
#59208=CARTESIAN_POINT ( 'NONE',  ( 3.610745725306120146, 1430.587129522550185, 217.8985349120129911 ) ) ;
#59214=ORIENTED_EDGE ( 'NONE', *, *, #8571, .T. ) ;
#59216=CARTESIAN_POINT ( 'NONE',  ( -16.90511930290000109, 1420.406826955899987, 203.3373784124190138 ) ) ;
#59220=CARTESIAN_POINT ( 'NONE',  ( -21.51339057090000040, 1505.551704408389924, 209.1218459616989946 ) ) ;
#59224=CARTESIAN_POINT ( 'NONE',  ( -11.22547157564759956, 1471.287375098959956, 207.0499038567439811 ) ) ;
#59225=CARTESIAN_POINT ( 'NONE',  ( -6.064879440841631997, 1508.311297157248646, 220.0963463610631834 ) ) ;
#59231=CARTESIAN_POINT ( 'NONE',  ( -14.75797601881649967, 1418.752372393509859, 201.0755002445320088 ) ) ;
#59232=CARTESIAN_POINT ( 'NONE',  ( 5.172586535390000684, 1492.767659076290101, 188.8148697515989909 ) ) ;
#59234=ORIENTED_EDGE ( 'NONE', *, *, #47348, .T. ) ;
#59235=VERTEX_POINT ( 'NONE', #88 ) ;
#59242=CARTESIAN_POINT ( 'NONE',  ( -4.636100717163651019, 1378.002096502181075, 203.9687531828620877 ) ) ;
#59246=CARTESIAN_POINT ( 'NONE',  ( -5.292247061280000331, 1391.913060387289988, 214.4361776263990009 ) ) ;
#59247=CARTESIAN_POINT ( 'NONE',  ( 11.86864872463300102, 1492.042928286840151, 209.5967942225589979 ) ) ;
#59249=CARTESIAN_POINT ( 'NONE',  ( -3.060197065649999715, 1457.550370828590076, 218.5492502934789911 ) ) ;
#59254=CARTESIAN_POINT ( 'NONE',  ( 4.984765438547570149, 1508.551704408389924, 206.5097441823970144 ) ) ;
#59256=ORIENTED_EDGE ( 'NONE', *, *, #14562, .T. ) ;
#59262=CARTESIAN_POINT ( 'NONE',  ( -10.61999428370000054, 1462.990852395989805, 206.0510139005290000 ) ) ;
#59264=CARTESIAN_POINT ( 'NONE',  ( 0.1713342119950009845, 1442.917349970689884, 202.9113549887590011 ) ) ;
#59267=CARTESIAN_POINT ( 'NONE',  ( -11.63919359464260062, 1508.551704408389924, 217.4554316303789960 ) ) ;
#59269=CARTESIAN_POINT ( 'NONE',  ( 1.604608372890350187, 1486.554689331300096, 197.3067947285690309 ) ) ;
#59270=CARTESIAN_POINT ( 'NONE',  ( 4.699465565660820410, 1432.335544942790193, 201.1496391276479869 ) ) ;
#59276=CARTESIAN_POINT ( 'NONE',  ( 10.75504506440890040, 1478.312245267059780, 229.8871532797240036 ) ) ;
#59278=DIRECTION ( 'NONE',  ( 0.000000000000000000, 1.000000000000000000, -1.836970198721029688E-16 ) ) ;
#59283=DIRECTION ( 'NONE',  ( -1.224646799147350002E-16, 1.836970198721029688E-16, 1.000000000000000000 ) ) ;
#59286=CARTESIAN_POINT ( 'NONE',  ( -3.046861489599999917, 1475.471994209789955, 198.8673666174990160 ) ) ;
#59292=CARTESIAN_POINT ( 'NONE',  ( 2.566509579899709959, 1428.984001205079949, 217.0000999674069817 ) ) ;
#59293=CARTESIAN_POINT ( 'NONE',  ( -8.412371419999999489, 1424.256181506120129, 208.0131652990489783 ) ) ;
#59299=CARTESIAN_POINT ( 'NONE',  ( -6.707757304198008086, 1470.964955385042231, 216.6951309197101239 ) ) ;
#59300=CARTESIAN_POINT ( 'NONE',  ( 7.244778264954490510, 1426.495820955630052, 212.9096779512760236 ) ) ;
#59305=CARTESIAN_POINT ( 'NONE',  ( -11.25957898075910002, 1491.777264728850014, 206.9688726115570034 ) ) ;
#59316=CARTESIAN_POINT ( 'NONE',  ( 8.316853310700460966, 1435.402407723380065, 206.5373084086480162 ) ) ;
#59317=ORIENTED_EDGE ( 'NONE', *, *, #16496, .F. ) ;
#59336=CARTESIAN_POINT ( 'NONE',  ( -10.45120302590630068, 1480.043455506409828, 210.3065010141500011 ) ) ;
#59337=CARTESIAN_POINT ( 'NONE',  ( 4.081077166763362740, 1433.956112075854662, 201.6265345710585279 ) ) ;
#59338=CARTESIAN_POINT ( 'NONE',  ( -3.466266129564929965, 1508.551704408389924, 213.9108720011500111 ) ) ;
#59340=CARTESIAN_POINT ( 'NONE',  ( 7.399151400400000078, 1422.280175886809957, 195.6034776983989900 ) ) ;
#59342=B_SPLINE_CURVE_WITH_KNOTS ( 'NONE', 3,
 ( #68746, #93904, #17171, #26142, #36226, #103403, #70411, #87180, #17728, #60334, #51363, #69296, #94450, #104530, #110719, #51930 ),
 .UNSPECIFIED., .F., .F.,
 ( 4, 3, 3, 3, 3, 4 ),
 ( -7.627871908653229838, -7.157619290633450149, -6.147716997384709892, -5.141165131806689992, -4.136155949588020242, -3.133321433589999927 ),
 .UNSPECIFIED. ) ;
#59343=CARTESIAN_POINT ( 'NONE',  ( -4.366144226260000316, 1495.418471743290183, 198.0199394070990024 ) ) ;
#59346=CARTESIAN_POINT ( 'NONE',  ( 1.702416261868870073, 1493.957958506549858, 220.1113518634800243 ) ) ;
#59356=CARTESIAN_POINT ( 'NONE',  ( 8.742631905043140250, 1426.622762530149885, 210.8844128420550135 ) ) ;
#59365=CARTESIAN_POINT ( 'NONE',  ( -16.78271819211574112, 1420.478864045909404, 203.1931770898623597 ) ) ;
#59366=CARTESIAN_POINT ( 'NONE',  ( -1.842962215208689303, 1515.492058412107781, 213.2603893544997504 ) ) ;
#59367=CARTESIAN_POINT ( 'NONE',  ( 8.885863169899998582, 1465.108758012390126, 213.4968473838789862 ) ) ;
#59373=CARTESIAN_POINT ( 'NONE',  ( -0.7263599678500212153, 1477.494758098099737, 198.7454087897867225 ) ) ;
#59375=CARTESIAN_POINT ( 'NONE',  ( 9.146237114798470458, 1449.998848199699978, 208.1168068718100130 ) ) ;
#59377=CARTESIAN_POINT ( 'NONE',  ( -13.05162046615980032, 1467.538720443550119, 191.8992815197879906 ) ) ;
#59379=CARTESIAN_POINT ( 'NONE',  ( -12.63495890147190082, 1422.290833888599991, 205.4229267067590285 ) ) ;
#59384=CARTESIAN_POINT ( 'NONE',  ( 9.722207004026980570, 1428.114070666289763, 212.2005352792010058 ) ) ;
#59391=CARTESIAN_POINT ( 'NONE',  ( 9.186645411349999790, 1479.540829827790049, 203.8650577567789810 ) ) ;
#59394=CARTESIAN_POINT ( 'NONE',  ( -5.543844742518439617, 1434.311283813799946, 216.1702177519260033 ) ) ;
#59396=CARTESIAN_POINT ( 'NONE',  ( -15.22200272170000090, 1417.314676559359896, 211.7966809115490037 ) ) ;
#59401=CARTESIAN_POINT ( 'NONE',  ( 10.40611076564779935, 1423.173680896260066, 208.2592473985839945 ) ) ;
#59408=CARTESIAN_POINT ( 'NONE',  ( 5.346297422500000174, 1473.360741859489963, 218.2967445439789742 ) ) ;
#59409=CARTESIAN_POINT ( 'NONE',  ( 5.983287317399999417, 1451.235340618889950, 210.0682002075799915 ) ) ;
#59411=CARTESIAN_POINT ( 'NONE',  ( -10.49113256600000099, 1492.581845576989963, 203.3991013598590030 ) ) ;
#59420=CARTESIAN_POINT ( 'NONE',  ( -0.5336398385289990998, 1457.451400674990055, 199.5863132090090062 ) ) ;
#59424=CARTESIAN_POINT ( 'NONE',  ( -3.467940627379999974, 1495.562067971789929, 197.2905559059990139 ) ) ;
#59440=CARTESIAN_POINT ( 'NONE',  ( 12.68801083313210043, 1500.413651417279880, 208.6561539661539939 ) ) ;
#59441=FACE_OUTER_BOUND ( 'NONE', #82546, .T. ) ;
#59450=CARTESIAN_POINT ( 'NONE',  ( 10.21346743305219995, 1453.430616332530008, 212.0093735090799782 ) ) ;
#59452=CARTESIAN_POINT ( 'NONE',  ( -14.17032501240000109, 1507.703614819789891, 209.3618925486269973 ) ) ;
#59454=CARTESIAN_POINT ( 'NONE',  ( 4.038582019099999698, 1515.598601288489817, 209.1218459617159908 ) ) ;
#59455=CARTESIAN_POINT ( 'NONE',  ( -6.508912761185129625, 1454.032954269330048, 202.3712805252700093 ) ) ;
#59458=CARTESIAN_POINT ( 'NONE',  ( 9.409271459137828586, 1451.760564006479854, 209.6856075121530125 ) ) ;
#59461=ORIENTED_EDGE ( 'NONE', *, *, #61791, .T. ) ;
#59470=CARTESIAN_POINT ( 'NONE',  ( -17.33881979142094920, 1508.455908737108757, 212.8389046703344434 ) ) ;
#59471=CARTESIAN_POINT ( 'NONE',  ( -7.130431368400969916, 1489.820748338716157, 217.4188096387678399 ) ) ;
#59474=CARTESIAN_POINT ( 'NONE',  ( -7.941319541319999509, 1469.154588994090091, 217.1846401660390029 ) ) ;
#59479=CARTESIAN_POINT ( 'NONE',  ( 7.159096167851838999, 1467.721109967099892, 200.5586486524099996 ) ) ;
#59486=FACE_OUTER_BOUND ( 'NONE', #21542, .T. ) ;
#59487=CARTESIAN_POINT ( 'NONE',  ( -14.40762303440000025, 1415.739699861750069, 214.0597611563689782 ) ) ;
#59488=CARTESIAN_POINT ( 'NONE',  ( -11.27716492698469963, 1500.448551123189873, 210.9498347538589940 ) ) ;
#59498=CARTESIAN_POINT ( 'NONE',  ( -9.350033435369999424, 1478.007838331189760, 213.9435157906089842 ) ) ;
#59505=B_SPLINE_CURVE_WITH_KNOTS ( 'NONE', 5,
 ( #101200, #92819, #16090, #50297, #84425, #7711 ),
 .UNSPECIFIED., .F., .F.,
 ( 6, 6 ),
 ( -2.000000000000000000, 0.000000000000000000 ),
 .UNSPECIFIED. ) ;
#59510=CARTESIAN_POINT ( 'NONE',  ( -8.372769162319999126, 1460.069700419990113, 216.1743697456390123 ) ) ;
#59513=CARTESIAN_POINT ( 'NONE',  ( -16.62627913534196367, 1419.615195795464842, 209.0779031733366082 ) ) ;
#59514=CARTESIAN_POINT ( 'NONE',  ( -3.607509927959999807, 1496.493923052690207, 219.8931759207989955 ) ) ;
#59515=ORIENTED_EDGE ( 'NONE', *, *, #102671, .F. ) ;
#59518=CARTESIAN_POINT ( 'NONE',  ( 10.56678653000900070, 1481.373476838040006, 208.8185995517700064 ) ) ;
#59528=CARTESIAN_POINT ( 'NONE',  ( -15.64577902933677400, 1415.699214057148765, 209.5376509458647831 ) ) ;
#59529=CARTESIAN_POINT ( 'NONE',  ( 1.842963721827329815, 1515.551704300040001, 212.9514659606769840 ) ) ;
#59532=CARTESIAN_POINT ( 'NONE',  ( 4.194095649580000362, 1484.606106053989834, 219.7768138602989723 ) ) ;
#59533=CARTESIAN_POINT ( 'NONE',  ( 10.67085484400129936, 1479.345408069779978, 206.7791535906509921 ) ) ;
#59535=CARTESIAN_POINT ( 'NONE',  ( -19.86607082145389924, 1443.193049015349970, 213.0732219199160227 ) ) ;
#59537=CARTESIAN_POINT ( 'NONE',  ( -21.59687425035849984, 1507.523446669369832, 209.4572656896989997 ) ) ;
#59544=CARTESIAN_POINT ( 'NONE',  ( 4.144219985687159991, 1446.806893490560014, 199.8398090959030071 ) ) ;
#59548=DIRECTION ( 'NONE',  ( 2.182550389754619197E-05, -9.529833270879996287E-07, -0.9999999997613695513 ) ) ;
#59558=CARTESIAN_POINT ( 'NONE',  ( -19.18813880309999931, 1465.797355387890093, 204.3301597990889888 ) ) ;
#59561=CARTESIAN_POINT ( 'NONE',  ( -0.8695030706469989434, 1444.523560491489889, 199.0910625714990090 ) ) ;
#59566=CARTESIAN_POINT ( 'NONE',  ( 1.902221077130000104, 1466.933671594890029, 220.0347825763990102 ) ) ;
#59568=SHAPE_REPRESENTATION_RELATIONSHIP ( 'NONE' , 'NONE' ,  #22211, #17149 ) ;
#59583=CARTESIAN_POINT ( 'NONE',  ( 11.20822254254120054, 1422.140100304710131, 210.4218750758840031 ) ) ;
#59590=B_SPLINE_CURVE_WITH_KNOTS ( 'NONE', 3,
 ( #67149, #15044, #101247, #24546, #58734, #92872, #95092, #95642, #77201, #27889, #96198, #44709, #59849, #60966, #503, #27329, #53673, #10535, #35179, #26213, #18910, #71031, #104595, #68812, #26779 ),
 .UNSPECIFIED., .F., .F.,
 ( 4, 2, 1, 1, 1, 2, 2, 2, 2, 2, 1, 1, 2, 2, 4 ),
 ( 0.000000000000000000, 0.1249999999994817756, 0.1874999999992220667, 0.2187499999990761834, 0.2343749999990034638, 0.2421874999989827582, 0.2499999999989620525, 0.3749999999991381894, 0.4999999999993144373, 0.6249999999994905187, 0.6874999999995785593, 0.7187499999996226352, 0.7343749999996446176, 0.7499999999996664890, 1.000000000000000000 ),
 .UNSPECIFIED. ) ;
#59597=CARTESIAN_POINT ( 'NONE',  ( -17.99551211388680017, 1508.551704408389924, 210.4093460685060109 ) ) ;
#59598=CARTESIAN_POINT ( 'NONE',  ( 1.145290945507940084, 1458.110487998910003, 199.6352770989870180 ) ) ;
#59599=DIRECTION ( 'NONE',  ( 0.02616798426500965835, 0.9993150019883683122, -0.02616798426500980754 ) ) ;
#59623=B_SPLINE_CURVE_WITH_KNOTS ( 'NONE', 3,
 ( #35530, #52363, #27143, #76430, #78086, #77545, #849, #68059, #102707, #59100 ),
 .UNSPECIFIED., .F., .F.,
 ( 4, 2, 2, 2, 4 ),
 ( 0.000000000000000000, 0.2500000000000000555, 0.5000000000000001110, 0.7500000000000002220, 1.000000000000000000 ),
 .UNSPECIFIED. ) ;
#59624=CARTESIAN_POINT ( 'NONE',  ( 20.54534055259999903, 1497.714303034489831, 214.2326470396490095 ) ) ;
#59630=CARTESIAN_POINT ( 'NONE',  ( -9.534866870576710340, 1508.435327360539986, 218.9526267747990005 ) ) ;
#59634=CARTESIAN_POINT ( 'NONE',  ( -7.000556739138234619, 1462.063838201012686, 202.3209658103452568 ) ) ;
#59636=CARTESIAN_POINT ( 'NONE',  ( -0.8181503024550010883, 1443.528514123589957, 218.3809319504590007 ) ) ;
#59637=CARTESIAN_POINT ( 'NONE',  ( 1.836834587526461560, 1468.808813678543174, 218.9756236043036779 ) ) ;
#59641=CARTESIAN_POINT ( 'NONE',  ( -2.435720382860000033, 1429.409294826790074, 200.4602887765989863 ) ) ;
#59644=CARTESIAN_POINT ( 'NONE',  ( 4.748711208231009451, 1507.009513748249901, 219.8044609659320088 ) ) ;
#59649=CARTESIAN_POINT ( 'NONE',  ( 1.875671004969999833, 1456.514200624189925, 219.5762891113990065 ) ) ;
#59655=CARTESIAN_POINT ( 'NONE',  ( 11.36216709560000027, 1503.110266136990049, 211.0233811791089806 ) ) ;
#59659=CARTESIAN_POINT ( 'NONE',  ( 2.135969990866780410, 1495.504088156479838, 220.8536837690359960 ) ) ;
#59668=ORIENTED_EDGE ( 'NONE', *, *, #24780, .F. ) ;
#59670=CARTESIAN_POINT ( 'NONE',  ( 3.434724471535389956, 1435.107767863380104, 227.2409729610280067 ) ) ;
#59671=CARTESIAN_POINT ( 'NONE',  ( -15.42684126378997078, 1416.006794007834969, 207.1724738609944723 ) ) ;
#59674=CARTESIAN_POINT ( 'NONE',  ( -1.466948456919999977, 1443.753574957790079, 218.3055264745389934 ) ) ;
#59678=CARTESIAN_POINT ( 'NONE',  ( 7.418387368310000340, 1424.469332702489965, 212.4790143585790076 ) ) ;
#59685=VERTEX_POINT ( 'NONE', #15590 ) ;
#59688=B_SPLINE_CURVE_WITH_KNOTS ( 'NONE', 3,
 ( #43736, #1196, #101396, #35328, #94121, #75692, #100857, #24690, #17392, #24148, #58338, #92462, #15733, #109835, #33115, #58886, #45947, #37534, #44861, #62782, #53821, #79551 ),
 .UNSPECIFIED., .F., .F.,
 ( 4, 3, 3, 3, 3, 3, 3, 4 ),
 ( -22.88731671675060042, -22.46512262839840091, -21.08674352509629912, -19.70521628440419803, -18.32242547603609850, -16.93931000582749746, -15.55731100368929987, -14.17748175460000049 ),
 .UNSPECIFIED. ) ;
#59697=CARTESIAN_POINT ( 'NONE',  ( -9.827940810840798846, 1446.801051858660003, 212.2330799875740013 ) ) ;
#59701=ORIENTED_EDGE ( 'NONE', *, *, #5309, .T. ) ;
#59708=CARTESIAN_POINT ( 'NONE',  ( 6.204876009399109549, 1424.478647642289843, 193.6606188949869818 ) ) ;
#59716=ADVANCED_FACE ( 'NONE', ( #102917 ), #75177, .T. ) ;
#59721=CARTESIAN_POINT ( 'NONE',  ( -8.502906657153658898, 1438.177461398969172, 207.2017738345354871 ) ) ;
#59728=CARTESIAN_POINT ( 'NONE',  ( -5.303285988883490454, 1442.879254652209966, 200.5943008362860098 ) ) ;
#59743=CARTESIAN_POINT ( 'NONE',  ( -3.812371268600000196, 1428.459941784990178, 200.5740418463989840 ) ) ;
#59747=CARTESIAN_POINT ( 'NONE',  ( -6.793605660180000783, 1414.360700121709897, 207.1411138948689938 ) ) ;
#59753=ADVANCED_FACE ( 'NONE', ( #2171 ), #57290, .T. ) ;
#59760=CONICAL_SURFACE ( 'NONE', #31124, 6.911399307709998219, 0.04363323129990067523 ) ;
#59761=FACE_OUTER_BOUND ( 'NONE', #80342, .T. ) ;
#59766=PLANE ( 'NONE',  #28799 ) ;
#59768=CARTESIAN_POINT ( 'NONE',  ( -11.40596013332580050, 1470.784863085199959, 209.0332487307530300 ) ) ;
#59769=CARTESIAN_POINT ( 'NONE',  ( -7.713101326021401860, 1508.427059880648358, 219.5098945182681121 ) ) ;
#59772=CARTESIAN_POINT ( 'NONE',  ( -7.884560102309425389, 1458.514255516424100, 214.6067317821517406 ) ) ;
#59775=CARTESIAN_POINT ( 'NONE',  ( -4.394042746799730281, 1420.918297765330180, 194.0393747012239771 ) ) ;
#59776=CARTESIAN_POINT ( 'NONE',  ( 4.327012684985810154, 1515.157823446690145, 208.9938042305240060 ) ) ;
#59785=EDGE_CURVE ( 'NONE', #77321, #42035, #71205, .T. ) ;
#59788=CARTESIAN_POINT ( 'NONE',  ( -4.638785869710670084, 1378.122666164550310, 203.7745336881851586 ) ) ;
#59789=CARTESIAN_POINT ( 'NONE',  ( -4.324092179420000015, 1515.269353058490196, 209.1218459618469865 ) ) ;
#59791=CARTESIAN_POINT ( 'NONE',  ( -10.76610300729999992, 1461.751116409589940, 211.3389343560589850 ) ) ;
#59794=CARTESIAN_POINT ( 'NONE',  ( 10.56687430813880013, 1452.631846242170013, 209.6720685516360163 ) ) ;
#59800=ORIENTED_EDGE ( 'NONE', *, *, #42680, .T. ) ;
#59807=CARTESIAN_POINT ( 'NONE',  ( 11.76251392144250119, 1479.675718945300105, 209.8000875804440284 ) ) ;
#59809=DIRECTION ( 'NONE',  ( 0.2766542314861598628, 0.3717636679784723786, 0.8861457054976875636 ) ) ;
#59810=CARTESIAN_POINT ( 'NONE',  ( 0.000000000000000000, 1378.013060387289897, 209.1218459616989946 ) ) ;
#59813=CARTESIAN_POINT ( 'NONE',  ( -0.01713803560704209999, 1486.114444591910114, 197.2146938469659858 ) ) ;
#59814=CARTESIAN_POINT ( 'NONE',  ( 10.52925756285159942, 1470.684013483499939, 209.6681956286249999 ) ) ;
#59815=CARTESIAN_POINT ( 'NONE',  ( 6.800214974479639629, 1435.261544033620112, 203.8159018546080290 ) ) ;
#59821=CARTESIAN_POINT ( 'NONE',  ( 4.722103809230000060, 1472.365862868290151, 187.6427232028989920 ) ) ;
#59828=CARTESIAN_POINT ( 'NONE',  ( -12.91325991898034786, 1507.673968545811704, 209.2392918446375063 ) ) ;
#59830=CARTESIAN_POINT ( 'NONE',  ( 1.329456730940000053, 1477.528821806389942, 198.7863296140990030 ) ) ;
#59836=CARTESIAN_POINT ( 'NONE',  ( -1.430539248151910137, 1444.328264662749916, 199.1703804428329931 ) ) ;
#59842=CARTESIAN_POINT ( 'NONE',  ( 7.205920432443370771, 1426.539681308049921, 212.9869048957809810 ) ) ;
#59849=CARTESIAN_POINT ( 'NONE',  ( 0.5238056268335857801, 1487.609062966209649, 219.9549396858940895 ) ) ;
#59850=FACE_OUTER_BOUND ( 'NONE', #23701, .T. ) ;
#59851=DIRECTION ( 'NONE',  ( 9.230617842401318720E-47, -1.000000000000000000, 1.836970198721029688E-16 ) ) ;
#59853=CARTESIAN_POINT ( 'NONE',  ( 4.333931798808769997, 1467.827050109060110, 218.1149461721859950 ) ) ;
#59860=VERTEX_POINT ( 'NONE', #2863 ) ;
#59861=VERTEX_POINT ( 'NONE', #12881 ) ;
#59875=CARTESIAN_POINT ( 'NONE',  ( 1.771184440399770077, 1445.612359891010101, 199.1903901163940134 ) ) ;
#59878=CARTESIAN_POINT ( 'NONE',  ( 2.487923159525660122, 1508.611354624159958, 204.4437017682370197 ) ) ;
#59881=CARTESIAN_POINT ( 'NONE',  ( -4.001327954982739854, 1508.551704408389924, 213.5978375056940024 ) ) ;
#59882=CARTESIAN_POINT ( 'NONE',  ( 12.41491102362930121, 1501.318694629519996, 211.8840886488729893 ) ) ;
#59884=CARTESIAN_POINT ( 'NONE',  ( 7.311826422820000282, 1422.546741514869836, 195.5507102769989842 ) ) ;
#59886=B_SPLINE_SURFACE_WITH_KNOTS ( 'NONE', 5, 5, ( 
 ( #13610, #100397, #30985, #23123, #90891, #65160 ),
 ( #99832, #74114, #14176, #82502, #91454, #5803 ),
 ( #47798, #39944, #108245, #6340, #83047, #31535 ),
 ( #65710, #34841, #100924, #84139, #43260, #51110 ),
 ( #713, #24759, #77407, #16904, #75757, #69032 ),
 ( #25870, #75216, #102031, #67922, #24222, #42151 ),
 ( #67373, #18029, #25317, #170, #50560, #52221 ),
 ( #7439, #7984, #84686, #109903, #6883, #85234 ),
 ( #41037, #15801, #59514, #26433, #103133, #16361 ) ),
 .UNSPECIFIED., .F., .F., .F.,
 ( 6, 3, 6 ),
 ( 6, 6 ),
 ( 14.73068219289999981, 30.91096027220000053, 36.02199544990000390 ),
 ( 0.000000000000000000, 2.000000000000000000 ),
 .UNSPECIFIED. ) ;
#59891=CARTESIAN_POINT ( 'NONE',  ( 3.829620113550000315, 1515.551704408389924, 210.9648081929590262 ) ) ;
#59901=DIRECTION ( 'NONE',  ( -9.138167445698339565E-47, 1.000000000000000000, -1.836970198721029688E-16 ) ) ;
#59902=ADVANCED_FACE ( 'NONE', ( #47601 ), #101994, .T. ) ;
#59905=CARTESIAN_POINT ( 'NONE',  ( 9.911722878192179564, 1428.067636776900144, 211.9710459987479965 ) ) ;
#59906=CARTESIAN_POINT ( 'NONE',  ( 0.4038046531345523271, 1421.163526409605765, 193.7214141364934221 ) ) ;
#59907=CARTESIAN_POINT ( 'NONE',  ( -10.93147186535690096, 1462.715198542749931, 207.4958911510919961 ) ) ;
#59908=FACE_OUTER_BOUND ( 'NONE', #80962, .T. ) ;
#59914=CARTESIAN_POINT ( 'NONE',  ( 18.34445210801149884, 1428.946210474640111, 201.3092770736820114 ) ) ;
#59916=CARTESIAN_POINT ( 'NONE',  ( 9.425093484676720479, 1420.682064370679882, 196.8057936142159861 ) ) ;
#59917=CARTESIAN_POINT ( 'NONE',  ( 10.15219587857820116, 1462.852240055779930, 213.4500398469340041 ) ) ;
#59922=CARTESIAN_POINT ( 'NONE',  ( -8.084570023343367495, 1425.034990034922430, 209.7848060853768573 ) ) ;
#59925=CARTESIAN_POINT ( 'NONE',  ( 9.923042118358591068, 1451.489751077119990, 207.3834753951100254 ) ) ;
#59928=CARTESIAN_POINT ( 'NONE',  ( 24.04367182619530041, 1494.655699650459837, 207.1743774084869756 ) ) ;
#59931=CARTESIAN_POINT ( 'NONE',  ( -17.84399408628319961, 1419.477046998499873, 208.9994865744390040 ) ) ;
#59933=CARTESIAN_POINT ( 'NONE',  ( 18.29188182340000068, 1431.768652859389704, 209.1218459616989946 ) ) ;
#59939=CARTESIAN_POINT ( 'NONE',  ( -7.559730510238970247, 1508.551704408389924, 219.0490070243000105 ) ) ;
#59941=CARTESIAN_POINT ( 'NONE',  ( -10.28013529000000048, 1471.607561406590094, 209.6293381294269977 ) ) ;
#59943=DIRECTION ( 'NONE',  ( 8.727810504445229884E-47, -1.000000000000000000, 1.836970198721029688E-16 ) ) ;
#59944=CARTESIAN_POINT ( 'NONE',  ( 3.601839739459999912, 1444.840594719589944, 200.9001243581789993 ) ) ;
#59945=CARTESIAN_POINT ( 'NONE',  ( -15.57808073540140015, 1420.358152465259991, 210.5578313205389804 ) ) ;
#59946=CARTESIAN_POINT ( 'NONE',  ( 0.6715583085099990912, 1506.489872953789927, 221.9351472385990007 ) ) ;
#59954=CARTESIAN_POINT ( 'NONE',  ( 11.82045713465280024, 1421.864468249930269, 207.3034728234389945 ) ) ;
#59955=ORIENTED_EDGE ( 'NONE', *, *, #53839, .F. ) ;
#59961=CARTESIAN_POINT ( 'NONE',  ( -18.27210413946250256, 1441.296816368030022, 213.1559958055480024 ) ) ;
#59963=CARTESIAN_POINT ( 'NONE',  ( -9.980038972539999165, 1493.754093306789855, 204.0458854781789739 ) ) ;
#59967=CARTESIAN_POINT ( 'NONE',  ( -9079.130222195200986, 5181.793945261120825, -1567.248257619579817 ) ) ;
#59968=CARTESIAN_POINT ( 'NONE',  ( 6.185074461130000145, 1447.943819131290184, 200.8573415407390144 ) ) ;
#59971=CARTESIAN_POINT ( 'NONE',  ( -2.817242487250000149, 1454.702949441090141, 199.4062663517090073 ) ) ;
#59974=CARTESIAN_POINT ( 'NONE',  ( 11.86100642208650058, 1492.894948804929982, 212.5846969273300147 ) ) ;
#59976=CARTESIAN_POINT ( 'NONE',  ( 1.792291835849999959, 1494.398898525389995, 220.1169104681989950 ) ) ;
#59991=CARTESIAN_POINT ( 'NONE',  ( 2.612101779301709836, 1508.551704408389924, 214.1066114002470044 ) ) ;
#59995=CARTESIAN_POINT ( 'NONE',  ( -19.42433358639999952, 1464.716960038490242, 212.6616036344889835 ) ) ;
#59999=CARTESIAN_POINT ( 'NONE',  ( -2.249657671790000091, 1425.043706724730100, 191.2451905349990113 ) ) ;
#60008=CARTESIAN_POINT ( 'NONE',  ( 10.04570719981230020, 1451.816709674880030, 208.0790574034220128 ) ) ;
#60017=FACE_OUTER_BOUND ( 'NONE', #52767, .T. ) ;
#60019=CARTESIAN_POINT ( 'NONE',  ( 7.214567273695688954, 1429.106908498430130, 215.2766334858309847 ) ) ;
#60023=CARTESIAN_POINT ( 'NONE',  ( -2.337589116788117760, 1488.423472059833557, 219.7633494153144511 ) ) ;
#60026=CARTESIAN_POINT ( 'NONE',  ( -3.950648164493409720, 1468.310338075048548, 219.6289969960776887 ) ) ;
#60031=CARTESIAN_POINT ( 'NONE',  ( 7.371950962006430075, 1467.810002177039905, 200.7277130371840030 ) ) ;
#60041=CARTESIAN_POINT ( 'NONE',  ( 1.384206944075679901, 1515.080800108599988, 204.7928163502200221 ) ) ;
#60042=VERTEX_POINT ( 'NONE', #71052 ) ;
#60044=CARTESIAN_POINT ( 'NONE',  ( -0.9490323356140020206, 1507.925252277690106, 221.0232043775990007 ) ) ;
#60048=CARTESIAN_POINT ( 'NONE',  ( -11.03313129935749792, 1462.309928051650104, 209.2979651268820191 ) ) ;
#60050=CARTESIAN_POINT ( 'NONE',  ( -3.812371247207599900, 1428.459941768050157, 200.5740418269730014 ) ) ;
#60052=CARTESIAN_POINT ( 'NONE',  ( 4.257623127619999615, 1479.092245966489827, 202.6254196850889855 ) ) ;
#60054=CARTESIAN_POINT ( 'NONE',  ( -10.44175186412380008, 1480.437295940329932, 207.7252335065300031 ) ) ;
#60068=CARTESIAN_POINT ( 'NONE',  ( -14.38020684849999853, 1416.780301525639970, 203.5793783887689870 ) ) ;
#60070=CARTESIAN_POINT ( 'NONE',  ( -6.025152189795589308, 1484.743689720570046, 198.8560543189699956 ) ) ;
#60071=B_SPLINE_SURFACE_WITH_KNOTS ( 'NONE', 5, 1, ( 
 ( #78115, #78676 ),
 ( #87074, #93791 ),
 ( #18743, #61357 ),
 ( #103295, #337 ),
 ( #42874, #9268 ),
 ( #95476, #104980 ),
 ( #103872, #94924 ),
 ( #10359, #27172 ),
 ( #1419, #70312 ),
 ( #1993, #70867 ),
 ( #69189, #52937 ),
 ( #26602, #26036 ),
 ( #85968, #44531 ),
 ( #36128, #104425 ),
 ( #17626, #77031 ),
 ( #85396, #35559 ),
 ( #34464, #68640 ),
 ( #35008, #27718 ),
 ( #52394, #102740 ),
 ( #60229, #94348 ),
 ( #60799, #61905 ),
 ( #96023, #69754 ),
 ( #36674, #8693 ),
 ( #19294, #10925 ),
 ( #885, #51263 ),
 ( #51831, #43976 ),
 ( #45101, #79241 ),
 ( #86517, #2549 ),
 ( #43428, #17066 ),
 ( #77577, #28269 ),
 ( #18197, #80883 ),
 ( #107175, #3652 ),
 ( #37781, #81402 ),
 ( #4714, #46752 ),
 ( #97676, #21490 ),
 ( #55702, #37229 ),
 ( #80335, #55154 ),
 ( #22034, #106620 ),
 ( #54060, #4179 ),
 ( #71970, #73600 ),
 ( #63026, #73036 ),
 ( #45655, #38858 ),
 ( #89823, #38312 ),
 ( #47829, #13639 ),
 ( #30467, #90361 ),
 ( #64653, #106082 ),
 ( #97131, #81962 ),
 ( #20400, #98772 ),
 ( #11479, #56231 ),
 ( #107730, #5268 ),
 ( #54605, #88737 ) ),
 .UNSPECIFIED., .F., .F., .F.,
 ( 6, 3, 3, 3, 3, 3, 3, 3, 3, 3, 3, 3, 3, 3, 3, 3, 6 ),
 ( 2, 2 ),
 ( 0.000000000000000000, 28.69702819429999963, 61.04778752440000034, 93.62768910810000023, 123.7336603250000024, 156.1762685979999787, 187.3272846180000215, 220.4669312460000015, 237.3878297990000021, 254.2938300590000154, 289.2398204710000300, 325.3030936050000150, 360.8626869010000178, 395.8828220460000011, 432.6128460950000090, 468.8934854820000169, 502.1482307969999965 ),
 ( -1.776356839400000001E-15, 2.001700839520000219 ),
 .UNSPECIFIED. ) ;
#60072=CARTESIAN_POINT ( 'NONE',  ( -16.25590069084343270, 1419.722612204563575, 209.8386441428618809 ) ) ;
#60077=CARTESIAN_POINT ( 'NONE',  ( -11.40049322445420010, 1508.551708765010062, 208.9769759148800006 ) ) ;
#60080=CARTESIAN_POINT ( 'NONE',  ( -18.83642247210000065, 1444.248298674089938, 209.1218459616989946 ) ) ;
#60092=CARTESIAN_POINT ( 'NONE',  ( 3.584507579370000308, 1486.500509928790052, 219.3043344553989868 ) ) ;
#60093=CARTESIAN_POINT ( 'NONE',  ( 10.52840799775919933, 1481.199580776819857, 208.2609754401459838 ) ) ;
#60094=CARTESIAN_POINT ( 'NONE',  ( -5.086186302109790169, 1453.993515012390162, 204.7329997213950037 ) ) ;
#60095=CARTESIAN_POINT ( 'NONE',  ( -8.029654524079999689, 1440.425766428789757, 228.7538251570989871 ) ) ;
#60102=CARTESIAN_POINT ( 'NONE',  ( -10.90735812309999986, 1491.858081601189951, 210.7852297805490025 ) ) ;
#60103=CARTESIAN_POINT ( 'NONE',  ( 8.291572064590001290, 1449.377284184440214, 202.9263957419950088 ) ) ;
#60108=CARTESIAN_POINT ( 'NONE',  ( 5.830794567472060486, 1434.584590126570220, 226.6688182991929921 ) ) ;
#60110=CARTESIAN_POINT ( 'NONE',  ( 9.463244449160031380, 1503.982580522659873, 216.1976177253470155 ) ) ;
#60119=CARTESIAN_POINT ( 'NONE',  ( -10.35066018003379895, 1448.307506586269938, 208.4121118022800090 ) ) ;
#60124=B_SPLINE_CURVE_WITH_KNOTS ( 'NONE', 5,
 ( #8191, #42357, #93848, #110116, #76511, #94397 ),
 .UNSPECIFIED., .F., .F.,
 ( 6, 6 ),
 ( -2.000000000000000000, -2.672797316805031187E-08 ),
 .UNSPECIFIED. ) ;
#60126=CARTESIAN_POINT ( 'NONE',  ( 3.135856758649999687, 1466.984112829190053, 218.9566971792889944 ) ) ;
#60152=CARTESIAN_POINT ( 'NONE',  ( -3.392699880776999688, 1433.356438688929984, 218.0666730085999916 ) ) ;
#60153=ORIENTED_EDGE ( 'NONE', *, *, #97397, .T. ) ;
#60155=CARTESIAN_POINT ( 'NONE',  ( -17.32634609470520104, 1508.551704408389924, 210.3986788274449680 ) ) ;
#60156=CARTESIAN_POINT ( 'NONE',  ( -4.019837105682418255, 1515.589591810382899, 208.5006405197344179 ) ) ;
#60161=CARTESIAN_POINT ( 'NONE',  ( -3.101981640767989656, 1428.864138099600041, 200.2836557281250123 ) ) ;
#60168=CARTESIAN_POINT ( 'NONE',  ( -11.85859649436589969, 1482.110477596389956, 208.2678370658890117 ) ) ;
#60175=EDGE_CURVE ( 'NONE', #27879, #101391, #55156, .T. ) ;
#60189=DIRECTION ( 'NONE',  ( -0.1652739736738010612, 0.3722510636888851088, 0.9132982312522922586 ) ) ;
#60190=CARTESIAN_POINT ( 'NONE',  ( 3.712013955199999771, 1466.291930614589774, 219.5294839965989979 ) ) ;
#60191=CARTESIAN_POINT ( 'NONE',  ( 2.144000416237634266, 1468.703099310448806, 218.9077027719663704 ) ) ;
#60195=CARTESIAN_POINT ( 'NONE',  ( -1.766639101469999806, 1429.583277275290129, 199.8949488872989946 ) ) ;
#60196=CARTESIAN_POINT ( 'NONE',  ( 11.60840177515349936, 1480.119960163069891, 211.2000821351769844 ) ) ;
#60200=VERTEX_POINT ( 'NONE', #3654 ) ;
#60206=CARTESIAN_POINT ( 'NONE',  ( 11.49286327549999953, 1502.439553125990187, 208.8615115388970196 ) ) ;
#60207=CARTESIAN_POINT ( 'NONE',  ( -11.20330708994425883, 1469.676918551309882, 192.3606680380646878 ) ) ;
#60209=CARTESIAN_POINT ( 'NONE',  ( 8.617375305610000424, 1422.946414101140135, 212.6945960971789873 ) ) ;
#60214=CARTESIAN_POINT ( 'NONE',  ( -6.858322662029999961, 1484.305021930289968, 199.8403620220989865 ) ) ;
#60221=ORIENTED_EDGE ( 'NONE', *, *, #45529, .F. ) ;
#60222=CARTESIAN_POINT ( 'NONE',  ( 2.262995014779219716, 1435.360232108469972, 227.4353352697579851 ) ) ;
#60225=CARTESIAN_POINT ( 'NONE',  ( -0.1159644321946630141, 1457.025002160060012, 219.7504842676799797 ) ) ;
#60228=CARTESIAN_POINT ( 'NONE',  ( 7.314450557279999821, 1425.029284243300026, 212.6285264488790006 ) ) ;
#60229=CARTESIAN_POINT ( 'NONE',  ( 18.68390456929999743, 1457.534965338390066, 220.6831945507989872 ) ) ;
#60242=LINE ( 'NONE', #70327, #28619 ) ;
#60243=EDGE_CURVE ( 'NONE', #87891, #81034, #98222, .T. ) ;
#60244=CARTESIAN_POINT ( 'NONE',  ( 1.035878012497590150, 1476.011601096869981, 197.6942168356959826 ) ) ;
#60253=ORIENTED_EDGE ( 'NONE', *, *, #37884, .T. ) ;
#60254=CARTESIAN_POINT ( 'NONE',  ( 3.500614145640000174, 1441.116913297490100, 218.4019928104889914 ) ) ;
#60264=ORIENTED_EDGE ( 'NONE', *, *, #97074, .F. ) ;
#60266=CARTESIAN_POINT ( 'NONE',  ( -4.660393612750000081, 1436.848553822789881, 227.0391165213990234 ) ) ;
#60294=CARTESIAN_POINT ( 'NONE',  ( -3.699859460309999903, 1428.525139549190044, 200.5225814697290048 ) ) ;
#60299=CARTESIAN_POINT ( 'NONE',  ( 3.451257193719999616, 1486.991677164690145, 198.1002659811989872 ) ) ;
#60312=CARTESIAN_POINT ( 'NONE',  ( -21.54121752360000031, 1506.208929616789874, 209.2336487591589957 ) ) ;
#60315=CARTESIAN_POINT ( 'NONE',  ( 1.352857657636009847, 1423.805410520770010, 191.2289116454009843 ) ) ;
#60317=CARTESIAN_POINT ( 'NONE',  ( -3.601377948332706413, 1508.124270563087748, 220.7476335447334748 ) ) ;
#60323=CARTESIAN_POINT ( 'NONE',  ( -14.38245154268600068, 1418.040796936970082, 202.3365336577070082 ) ) ;
#60327=CARTESIAN_POINT ( 'NONE',  ( -7.694565099120000085, 1508.539300327990077, 219.2224448576989744 ) ) ;
#60328=CARTESIAN_POINT ( 'NONE',  ( -4.487249066482500659, 1509.038643261319976, 211.6097700942569872 ) ) ;
#60334=CARTESIAN_POINT ( 'NONE',  ( -10.50525416227409892, 1479.903349258469916, 209.3106010834520134 ) ) ;
#60336=CARTESIAN_POINT ( 'NONE',  ( -11.15048904225209903, 1470.285759522020044, 211.3960241579200101 ) ) ;
#60338=CARTESIAN_POINT ( 'NONE',  ( 4.677543868301159868, 1434.888993089650057, 228.7640141638709963 ) ) ;
#60344=ORIENTED_EDGE ( 'NONE', *, *, #57002, .T. ) ;
#60351=CARTESIAN_POINT ( 'NONE',  ( -20.86254339170000094, 1504.682062816289999, 214.2159060785090219 ) ) ;
#60354=CARTESIAN_POINT ( 'NONE',  ( 4.031617629829999494, 1486.311417117990004, 219.1318982698989828 ) ) ;
#60355=CARTESIAN_POINT ( 'NONE',  ( -4.926245301684949673, 1495.054961305510005, 197.8234830982279959 ) ) ;
#60360=ADVANCED_FACE ( 'NONE', ( #2551 ), #30395, .T. ) ;
#60362=CARTESIAN_POINT ( 'NONE',  ( -1.398989223888390088, 1485.780538973669991, 197.3046819373520009 ) ) ;
#60364=CARTESIAN_POINT ( 'NONE',  ( -9.179256326701130675, 1450.524624793770045, 208.2094894903229942 ) ) ;
#60365=LINE ( 'NONE', #2686, #71646 ) ;
#60371=CARTESIAN_POINT ( 'NONE',  ( 18.29878862780000048, 1474.159682674189980, 194.8322854508990076 ) ) ;
#60374=EDGE_CURVE ( 'NONE', #65430, #63746, #85610, .T. ) ;
#60375=B_SPLINE_CURVE_WITH_KNOTS ( 'NONE', 3,
 ( #29760, #55541, #72883, #81807, #54998, #46594, #99703, #107021, #39263, #73437, #56078, #80729, #81258, #48237, #21878, #30309, #89121, #65033, #12410, #30858, #97526, #90204, #4037, #13488, #108114, #6210, #106475, #89665, #14607, #39823, #99151, #107572, #31408, #64499 ),
 .UNSPECIFIED., .F., .F.,
 ( 4, 3, 3, 3, 3, 3, 3, 3, 3, 3, 3, 4 ),
 ( -7.870238109499999801, -7.787503224266919766, -7.483736671101009819, -7.152628210470729719, -6.787049584866209351, -6.322373280637119564, -5.900059652451949965, -5.548137115487610238, -5.385973697081239742, -4.854088901389330246, -4.240705037260870114, -3.226035699099999654 ),
 .UNSPECIFIED. ) ;
#60376=CARTESIAN_POINT ( 'NONE',  ( -3.922072518270000252, 1476.187451415889882, 202.7181511965089840 ) ) ;
#60381=CARTESIAN_POINT ( 'NONE',  ( -1.779830841699999944, 1475.353704572689821, 197.8049865350990046 ) ) ;
#60387=CARTESIAN_POINT ( 'NONE',  ( -8.049617774310000584, 1424.935508317819995, 210.1093181517179858 ) ) ;
#60394=CARTESIAN_POINT ( 'NONE',  ( 7.535489564291699693, 1425.549448153189815, 212.1837449646579898 ) ) ;
#60397=ORIENTED_EDGE ( 'NONE', *, *, #47520, .F. ) ;
#60404=CARTESIAN_POINT ( 'NONE',  ( -2.458597632860000104, 1456.374695818690043, 215.3392858312989802 ) ) ;
#60411=CARTESIAN_POINT ( 'NONE',  ( 8.249102711688488299, 1435.329757872420032, 206.3470792129120071 ) ) ;
#60418=CARTESIAN_POINT ( 'NONE',  ( -17.25887910663729841, 1444.159329669600083, 200.5184087357610281 ) ) ;
#60431=CARTESIAN_POINT ( 'NONE',  ( 4.208243276966399549, 1434.939303095829928, 227.0652033583169782 ) ) ;
#60433=CARTESIAN_POINT ( 'NONE',  ( 3.788285567727110337, 1508.728291974460035, 204.8186037205090031 ) ) ;
#60435=CARTESIAN_POINT ( 'NONE',  ( -4.889439660197979265, 1508.551704408389924, 212.3011554026570025 ) ) ;
#60445=CARTESIAN_POINT ( 'NONE',  ( -15.57808073540140015, 1420.358152465259991, 210.5578313205389804 ) ) ;
#60456=CARTESIAN_POINT ( 'NONE',  ( 1.200868670922434989, 1421.369478736644396, 193.7619988307343704 ) ) ;
#60457=CARTESIAN_POINT ( 'NONE',  ( -4.326992699981060397, 1515.158586643130093, 209.1005884788399953 ) ) ;
#60462=CARTESIAN_POINT ( 'NONE',  ( -9.852457870043849653, 1461.554014673809888, 208.8474554947439970 ) ) ;
#60463=CARTESIAN_POINT ( 'NONE',  ( 20.10527571410489855, 1430.877954731940235, 215.1856771490429878 ) ) ;
#60464=CARTESIAN_POINT ( 'NONE',  ( 12.03775681428729882, 1426.191895615310159, 202.7989534666060081 ) ) ;
#60465=CARTESIAN_POINT ( 'NONE',  ( 9.660180252660660827, 1463.103700123790077, 211.4020709551699895 ) ) ;
#60470=CARTESIAN_POINT ( 'NONE',  ( -8.006373544986240987, 1424.874076710998452, 210.3858704081821145 ) ) ;
#60474=CARTESIAN_POINT ( 'NONE',  ( 9.145064077180329321, 1450.428955689400027, 207.9342079399700083 ) ) ;
#60476=CARTESIAN_POINT ( 'NONE',  ( -18.47518242017930135, 1466.235720257730009, 200.8822878153090130 ) ) ;
#60478=CARTESIAN_POINT ( 'NONE',  ( -16.48668639225170196, 1420.457505516819765, 204.7771018081849945 ) ) ;
#60487=CARTESIAN_POINT ( 'NONE',  ( -6.375118004043530462, 1508.551704408389924, 219.3472698286099956 ) ) ;
#60491=CARTESIAN_POINT ( 'NONE',  ( 8.244220094398297505, 1448.357206390987585, 205.1189572764488958 ) ) ;
#60494=CARTESIAN_POINT ( 'NONE',  ( -5.494816741715999875, 1433.961689851970050, 215.8643144989760003 ) ) ;
#60497=CARTESIAN_POINT ( 'NONE',  ( -10.31429908969579934, 1472.129925722029839, 207.0851132311250069 ) ) ;
#60502=CARTESIAN_POINT ( 'NONE',  ( -3.427918555806571455, 1475.607266589915980, 218.8585788157315335 ) ) ;
#60505=CARTESIAN_POINT ( 'NONE',  ( -4.682234856550000046, 1438.893385222290135, 227.1256850459990062 ) ) ;
#60509=CARTESIAN_POINT ( 'NONE',  ( 6.645104883328971646, 1422.852120593709969, 195.1791986883735035 ) ) ;
#60511=CARTESIAN_POINT ( 'NONE',  ( -10.02453695329999839, 1493.300892679689923, 203.8691444315089996 ) ) ;
#60516=CARTESIAN_POINT ( 'NONE',  ( 10855.50032577649290, 5181.793945261120825, -7093.638272652226078 ) ) ;
#60523=EDGE_CURVE ( 'NONE', #86013, #64533, #10886, .T. ) ;
#60547=CARTESIAN_POINT ( 'NONE',  ( 4.421669554984550388, 1508.551704408389924, 213.1944784729480205 ) ) ;
#60549=VERTEX_POINT ( 'NONE', #56542 ) ;
#60551=CARTESIAN_POINT ( 'NONE',  ( 9.636560193436579880, 1462.074131928580073, 207.7511217272350166 ) ) ;
#60558=ORIENTED_EDGE ( 'NONE', *, *, #95281, .F. ) ;
#60561=CARTESIAN_POINT ( 'NONE',  ( -11.35888576287617369, 1417.774827459571043, 198.7178256456102474 ) ) ;
#60562=EDGE_CURVE ( 'NONE', #1934, #109446, #38284, .T. ) ;
#60564=DIRECTION ( 'NONE',  ( -0.1867471702549219348, 2.391457216852619248E-16, 0.9824080081115885710 ) ) ;
#60566=CARTESIAN_POINT ( 'NONE',  ( 10.09897474760730063, 1452.024231682490154, 208.5505077355719834 ) ) ;
#60579=CARTESIAN_POINT ( 'NONE',  ( -9.642207540978898095, 1460.678569519029907, 208.4219211414859956 ) ) ;
#60582=CARTESIAN_POINT ( 'NONE',  ( 9.224062555858578705, 1450.491461610309898, 209.1237753033059903 ) ) ;
#60583=CARTESIAN_POINT ( 'NONE',  ( -4.845898873760000392, 1475.703792529090151, 200.0054992556989930 ) ) ;
#60584=CARTESIAN_POINT ( 'NONE',  ( 6.817812183760000089, 1493.124444775489792, 217.9221528793789844 ) ) ;
#60587=CARTESIAN_POINT ( 'NONE',  ( -21.53565904410000087, 1506.077647802689853, 209.2113159668479909 ) ) ;
#60597=CARTESIAN_POINT ( 'NONE',  ( -14.45258110980000055, 1415.677402202029953, 212.7925583635889950 ) ) ;
#60598=CARTESIAN_POINT ( 'NONE',  ( 0.1829789116263519921, 1515.156771665000178, 204.7948057348419866 ) ) ;
#60599=ORIENTED_EDGE ( 'NONE', *, *, #56832, .T. ) ;
#60600=CARTESIAN_POINT ( 'NONE',  ( -15.48888989581648623, 1415.677402280658725, 209.5875073814394796 ) ) ;
#60601=CARTESIAN_POINT ( 'NONE',  ( 1.760769565820000215, 1508.551704924790101, 220.0361975827989909 ) ) ;
#60608=CARTESIAN_POINT ( 'NONE',  ( 19.60792669039999936, 1475.100271358290229, 204.3343059087790152 ) ) ;
#60610=CARTESIAN_POINT ( 'NONE',  ( -9.297585099209999981, 1478.447333343590117, 214.0874750368789989 ) ) ;
#60616=VECTOR ( 'NONE', #80069, 1000.000000000000000 ) ;
#60626=CARTESIAN_POINT ( 'NONE',  ( 17.99383350722930075, 1429.161952351650143, 206.5116212249160128 ) ) ;
#60632=CARTESIAN_POINT ( 'NONE',  ( -10.61667206956300014, 1508.551704408270098, 207.6874843289959927 ) ) ;
#60644=CARTESIAN_POINT ( 'NONE',  ( 4.138993644310000164, 1515.551749209589843, 209.1218459616989946 ) ) ;
#60649=CARTESIAN_POINT ( 'NONE',  ( 3.678869892360000282, 1485.512442734190245, 219.3630818239989821 ) ) ;
#60650=CARTESIAN_POINT ( 'NONE',  ( 4.993626793399999819, 1423.332951346649907, 194.3851876207990017 ) ) ;
#60653=CARTESIAN_POINT ( 'NONE',  ( 7.905003682643709340, 1460.527882303560091, 228.8958833807890016 ) ) ;
#60655=CARTESIAN_POINT ( 'NONE',  ( -18.80013755969359934, 1505.319302960399909, 222.5373222880980109 ) ) ;
#60659=LINE ( 'NONE', #86381, #75243 ) ;
#60660=CARTESIAN_POINT ( 'NONE',  ( -11.88215827279999992, 1489.620311200989818, 211.9665674380289886 ) ) ;
#60661=CARTESIAN_POINT ( 'NONE',  ( 9.629035390439231179, 1450.586402395090090, 205.0971065227769827 ) ) ;
#60664=CARTESIAN_POINT ( 'NONE',  ( 3.959152859930000101, 1428.396642669490120, 216.3690266601789745 ) ) ;
#60665=CARTESIAN_POINT ( 'NONE',  ( 995.1856855245110864, 1453.395007294999914, 209.1431465539880037 ) ) ;
#60666=CARTESIAN_POINT ( 'NONE',  ( 10.30934595618430016, 1433.523148449839937, 224.4168098436820173 ) ) ;
#60669=VECTOR ( 'NONE', #40906, 1000.000000000000227 ) ;
#60672=VERTEX_POINT ( 'NONE', #92748 ) ;
#60674=ORIENTED_EDGE ( 'NONE', *, *, #100474, .F. ) ;
#60679=CARTESIAN_POINT ( 'NONE',  ( -10.34864842518480010, 1447.803587913199863, 209.5966951726140053 ) ) ;
#60680=CARTESIAN_POINT ( 'NONE',  ( 4.136749821589959630, 1515.492902831140100, 206.2237468939180189 ) ) ;
#60689=B_SPLINE_SURFACE_WITH_KNOTS ( 'NONE', 5, 1, ( 
 ( #108861, #106648 ),
 ( #38340, #107208 ),
 ( #97706, #29939 ),
 ( #65227, #55182 ),
 ( #98803, #4742 ),
 ( #108312, #90952 ) ),
 .UNSPECIFIED., .F., .F., .F.,
 ( 6, 6 ),
 ( 2, 2 ),
 ( 0.000000000000000000, 3.267792473789999708 ),
 ( 0.000000000000000000, 14.00000000000000000 ),
 .UNSPECIFIED. ) ;
#60692=CARTESIAN_POINT ( 'NONE',  ( -14.39765041480000107, 1420.835238719779909, 210.6164402859990048 ) ) ;
#60696=CARTESIAN_POINT ( 'NONE',  ( -0.7140353930058549459, 1431.991569043200116, 200.7371223997279799 ) ) ;
#60701=CARTESIAN_POINT ( 'NONE',  ( -11.74583952262180020, 1503.658476107915476, 208.1214586907342152 ) ) ;
#60703=CARTESIAN_POINT ( 'NONE',  ( 3.030007752585599956, 1466.220774424609772, 198.4981827063209892 ) ) ;
#60706=CARTESIAN_POINT ( 'NONE',  ( 12.13377226363930106, 1421.785238798449882, 208.4657368268529751 ) ) ;
#60710=EDGE_CURVE ( 'NONE', #37252, #29545, #87024, .T. ) ;
#60721=CARTESIAN_POINT ( 'NONE',  ( -0.8537895742897508855, 1422.738976114379966, 192.5159534119239879 ) ) ;
#60725=CARTESIAN_POINT ( 'NONE',  ( -3.945738874726128387, 1515.565581977718466, 207.8717498098853014 ) ) ;
#60726=CARTESIAN_POINT ( 'NONE',  ( -18.17365796220000007, 1441.208305948289762, 213.5442559039389891 ) ) ;
#60732=CARTESIAN_POINT ( 'NONE',  ( -3.625688031972540415, 1428.567653792310011, 200.4907183003010118 ) ) ;
#60736=CARTESIAN_POINT ( 'NONE',  ( -11.83148041523059923, 1482.212593895280179, 207.9057076157649817 ) ) ;
#60739=ORIENTED_EDGE ( 'NONE', *, *, #108907, .T. ) ;
#60742=CARTESIAN_POINT ( 'NONE',  ( 10.76075704858850024, 1490.821908851660055, 211.3234342363890050 ) ) ;
#60748=CARTESIAN_POINT ( 'NONE',  ( -9.244699677152100392, 1448.612501353059997, 209.9872400869060129 ) ) ;
#60754=AXIS2_PLACEMENT_3D ( 'NONE', #45979, #37562, #18530 ) ;
#60755=DIRECTION ( 'NONE',  ( 1.000000000000000000, 2.249639673992764790E-32, 1.224646799147350002E-16 ) ) ;
#60758=FACE_OUTER_BOUND ( 'NONE', #106700, .T. ) ;
#60760=VECTOR ( 'NONE', #37596, 1000.000000000000227 ) ;
#60764=CARTESIAN_POINT ( 'NONE',  ( 11.77838848180700104, 1479.583172727889860, 209.4916819176700074 ) ) ;
#60765=CARTESIAN_POINT ( 'NONE',  ( 5.095071723817279796, 1506.876855224960082, 219.6410062831469929 ) ) ;
#60774=CARTESIAN_POINT ( 'NONE',  ( 11.76282542499999906, 1501.584099486789910, 210.8989423168290216 ) ) ;
#60777=CARTESIAN_POINT ( 'NONE',  ( 7.984492602029999553, 1423.987908843459991, 211.8850966666189777 ) ) ;
#60790=CARTESIAN_POINT ( 'NONE',  ( 3.895917434060000240, 1499.417515733289974, 230.0327334827989887 ) ) ;
#60793=CARTESIAN_POINT ( 'NONE',  ( -1.299578229957530029, 1457.370843945099978, 219.6854510378979910 ) ) ;
#60794=CARTESIAN_POINT ( 'NONE',  ( -0.5711511081509990095, 1457.745025693589923, 202.2735493682390029 ) ) ;
#60797=CARTESIAN_POINT ( 'NONE',  ( 7.545761559389999817, 1424.826522491729975, 212.1621923280889916 ) ) ;
#60799=CARTESIAN_POINT ( 'NONE',  ( 7.755379691499999062, 1459.738853293389866, 228.9106028235989925 ) ) ;
#60803=CARTESIAN_POINT ( 'NONE',  ( 4.974027067470000674, 1455.144349094690142, 217.5915564868190017 ) ) ;
#60810=CARTESIAN_POINT ( 'NONE',  ( 7.568706834503317715, 1500.286747494142901, 200.6010021183646472 ) ) ;
#60823=EDGE_LOOP ( 'NONE', ( #95233, #82550, #106928, #24558 ) ) ;
#60837=TOROIDAL_SURFACE ( 'NONE', #93002, 10.71315034250000053, 1.000000000000000000 ) ;
#60850=CARTESIAN_POINT ( 'NONE',  ( 10.60194594222889819, 1460.225020076690043, 206.5389690418479915 ) ) ;
#60856=CARTESIAN_POINT ( 'NONE',  ( 7.334062741534030039, 1482.070311934039864, 210.1443595876939696 ) ) ;
#60866=CARTESIAN_POINT ( 'NONE',  ( -3.567860816820000114, 1429.016874681090030, 201.2351213331789950 ) ) ;
#60871=CARTESIAN_POINT ( 'NONE',  ( 1.869907053503540029, 1431.184470418000046, 218.4272402479099924 ) ) ;
#60875=CARTESIAN_POINT ( 'NONE',  ( 10.77497579070000100, 1480.716349263289885, 211.2103358511090221 ) ) ;
#60878=ORIENTED_EDGE ( 'NONE', *, *, #33065, .F. ) ;
#60880=DIRECTION ( 'NONE',  ( 9.500914144214121536E-47, -1.000000000000000000, 1.836970198721029688E-16 ) ) ;
#60881=ORIENTED_EDGE ( 'NONE', *, *, #6388, .F. ) ;
#60883=B_SPLINE_CURVE_WITH_KNOTS ( 'NONE', 5,
 ( #99211, #74048, #23056, #91392, #14670, #50501, #100335, #23622, #41540 ),
 .UNSPECIFIED., .F., .F.,
 ( 6, 3, 6 ),
 ( 0.000000000000000000, 0.9031158850279928929, 1.000000000000000000 ),
 .UNSPECIFIED. ) ;
#60884=CARTESIAN_POINT ( 'NONE',  ( -3.829620113550000315, 1515.551704408389924, 207.2788837304390199 ) ) ;
#60885=CARTESIAN_POINT ( 'NONE',  ( 2.774855403480000149, 1441.656174316490024, 218.2502874549990111 ) ) ;
#60891=CARTESIAN_POINT ( 'NONE',  ( -7.125888594031689394, 1458.093400128074336, 215.4885673113955136 ) ) ;
#60894=CARTESIAN_POINT ( 'NONE',  ( -10.14847552845580125, 1472.086894961059897, 209.7189879088959685 ) ) ;
#60895=CARTESIAN_POINT ( 'NONE',  ( 4.329089011153910427, 1515.078531749479907, 207.6981595341280240 ) ) ;
#60899=CARTESIAN_POINT ( 'NONE',  ( -4.554948924557931100, 1508.731372610989865, 211.6097697110380125 ) ) ;
#60904=CARTESIAN_POINT ( 'NONE',  ( -11.08201610607340015, 1470.229490766139861, 211.6946857826129929 ) ) ;
#60905=CARTESIAN_POINT ( 'NONE',  ( -4.633397090840619903, 1377.913060387289988, 204.3568503472270095 ) ) ;
#60906=CARTESIAN_POINT ( 'NONE',  ( 14.43086732081240164, 1426.807478003820052, 195.4949745959340248 ) ) ;
#60909=CARTESIAN_POINT ( 'NONE',  ( -5.105764674260594660, 1391.864935413667126, 214.6138670560712285 ) ) ;
#60911=CARTESIAN_POINT ( 'NONE',  ( 10.55831763905420040, 1452.305717713109971, 208.8223436732269818 ) ) ;
#60916=ORIENTED_EDGE ( 'NONE', *, *, #36296, .F. ) ;
#60919=CARTESIAN_POINT ( 'NONE',  ( -2.458567915935879533, 1456.374676718179899, 215.3392989940770121 ) ) ;
#60923=CARTESIAN_POINT ( 'NONE',  ( 8.589517928433638261, 1436.682903382349878, 208.3531420449839686 ) ) ;
#60928=CARTESIAN_POINT ( 'NONE',  ( -1.244053264164739936, 1485.816359186060026, 197.2880502459559864 ) ) ;
#60930=CARTESIAN_POINT ( 'NONE',  ( 8.091201492491240543, 1435.785803388039994, 206.2618594566330046 ) ) ;
#60932=AXIS2_PLACEMENT_3D ( 'NONE', #39395, #81376, #38831 ) ;
#60936=CARTESIAN_POINT ( 'NONE',  ( -3.744311016452680274, 1509.032041868229953, 213.3627935371090132 ) ) ;
#60937=CARTESIAN_POINT ( 'NONE',  ( -2.834728103336690008, 1469.264061671030049, 187.4402886115690023 ) ) ;
#60942=B_SPLINE_CURVE_WITH_KNOTS ( 'NONE', 5,
 ( #89620, #47089, #80682, #38665, #89074, #22386, #13442, #81215, #88540 ),
 .UNSPECIFIED., .F., .F.,
 ( 6, 3, 6 ),
 ( -24.98742667679999840, -15.52868752870000080, -11.38875369420000006 ),
 .UNSPECIFIED. ) ;
#60945=CARTESIAN_POINT ( 'NONE',  ( -13.36486944041102909, 1507.695946263434280, 209.3487293591950333 ) ) ;
#60953=VERTEX_POINT ( 'NONE', #103914 ) ;
#60954=CARTESIAN_POINT ( 'NONE',  ( -8.172692409730000662, 1424.011347619940125, 209.9196331268980202 ) ) ;
#60960=CARTESIAN_POINT ( 'NONE',  ( 7.539499508402939476, 1425.640709783210013, 212.1844604678450139 ) ) ;
#60964=CARTESIAN_POINT ( 'NONE',  ( -11.01047251046239772, 1492.285776553619826, 207.1645913320990076 ) ) ;
#60966=CARTESIAN_POINT ( 'NONE',  ( 0.7521604934737978754, 1487.535995793384245, 219.9383163343715637 ) ) ;
#60969=CARTESIAN_POINT ( 'NONE',  ( 0.3221681605929990200, 1455.007013527990011, 215.7786709544189989 ) ) ;
#60970=CARTESIAN_POINT ( 'NONE',  ( -8.534885686993231246, 1438.016363115470085, 207.5311831631819643 ) ) ;
#60995=CARTESIAN_POINT ( 'NONE',  ( 3.747824384289230260, 1508.879013859839915, 204.8753724212450038 ) ) ;
#60999=CARTESIAN_POINT ( 'NONE',  ( -3.219327822889010093, 1508.551704408389924, 213.9993814675680142 ) ) ;
#61004=DIRECTION ( 'NONE',  ( 0.9234275994329012027, -0.3778483828125600574, 0.06717193023519940631 ) ) ;
#61012=VERTEX_POINT ( 'NONE', #61395 ) ;
#61014=CARTESIAN_POINT ( 'NONE',  ( -9.721168970463079262, 1481.243685912169894, 204.9479208362279792 ) ) ;
#61017=CARTESIAN_POINT ( 'NONE',  ( -20.03233416495636021, 1508.143838515403331, 209.6381387959671088 ) ) ;
#61030=CONICAL_SURFACE ( 'NONE', #103915, 6.911399307709998219, 0.04363323129990067523 ) ;
#61031=CARTESIAN_POINT ( 'NONE',  ( 14.12397228379999881, 1429.152045054989912, 195.0086682020989883 ) ) ;
#61033=CARTESIAN_POINT ( 'NONE',  ( 9.634457963308390660, 1463.394280929989918, 210.8800767048959983 ) ) ;
#61039=CARTESIAN_POINT ( 'NONE',  ( -16.16965275211135022, 1420.192159313676257, 209.3182675821363148 ) ) ;
#61041=CARTESIAN_POINT ( 'NONE',  ( 3.408157919748749709, 1507.642492428714831, 220.3333379687577747 ) ) ;
#61042=CARTESIAN_POINT ( 'NONE',  ( 18.32584131703820063, 1473.764089907340121, 194.8973952594539867 ) ) ;
#61047=CARTESIAN_POINT ( 'NONE',  ( 3.500614145640000174, 1441.116913297490100, 218.4019928104889914 ) ) ;
#61048=ORIENTED_EDGE ( 'NONE', *, *, #63909, .F. ) ;
#61055=CARTESIAN_POINT ( 'NONE',  ( -2.691673115819169571, 1508.551704408389924, 220.0244384242639910 ) ) ;
#61061=CARTESIAN_POINT ( 'NONE',  ( 7.314234105809116038, 1447.455669405640265, 203.7241742676247327 ) ) ;
#61065=CARTESIAN_POINT ( 'NONE',  ( -3.139089597500000384, 1433.097404256189975, 217.7316571164689947 ) ) ;
#61066=CARTESIAN_POINT ( 'NONE',  ( -10.90103824469269966, 1471.515098176560059, 206.8303341461960088 ) ) ;
#61073=VECTOR ( 'NONE', #73799, 1000.000000000000114 ) ;
#61076=CARTESIAN_POINT ( 'NONE',  ( -2.992871990574130336, 1438.525994072939966, 227.4702121500120029 ) ) ;
#61078=CARTESIAN_POINT ( 'NONE',  ( 8.095719555432868475, 1465.757095899850128, 214.8014529992200039 ) ) ;
#61082=CARTESIAN_POINT ( 'NONE',  ( -7.769942807339999646, 1494.070509797290015, 200.0359136334189998 ) ) ;
#61091=CARTESIAN_POINT ( 'NONE',  ( 1.548977426030000215, 1456.873932682089844, 199.3713739669490224 ) ) ;
#61096=CARTESIAN_POINT ( 'NONE',  ( -1.011662833449999965, 1497.725169660189977, 197.8465252784990298 ) ) ;
#61097=CARTESIAN_POINT ( 'NONE',  ( 0.6251717133059989662, 1495.142630955389905, 220.4307413487989891 ) ) ;
#61105=ADVANCED_FACE ( 'NONE', ( #46286 ), #6301, .T. ) ;
#61112=CARTESIAN_POINT ( 'NONE',  ( -5.087359574289999742, 1391.865221655589949, 214.5720747206590033 ) ) ;
#61116=CARTESIAN_POINT ( 'NONE',  ( 9.493856384438370100, 1462.266385979010010, 206.9294982016510289 ) ) ;
#61118=ORIENTED_EDGE ( 'NONE', *, *, #74621, .T. ) ;
#61121=CARTESIAN_POINT ( 'NONE',  ( 8.771177098789999960, 1423.989855107869971, 196.4170041723990039 ) ) ;
#61133=VERTEX_POINT ( 'NONE', #107254 ) ;
#61141=ORIENTED_EDGE ( 'NONE', *, *, #68564, .T. ) ;
#61148=CARTESIAN_POINT ( 'NONE',  ( 1.916730757326210011, 1474.810910458910030, 220.3788423859229795 ) ) ;
#61149=CARTESIAN_POINT ( 'NONE',  ( -12.76143310688880028, 1502.479526517909790, 209.7877290102630070 ) ) ;
#61150=CARTESIAN_POINT ( 'NONE',  ( -2.386039747897999774, 1422.172641114239923, 193.0199730022190181 ) ) ;
#61164=CARTESIAN_POINT ( 'NONE',  ( -14.50669600419999838, 1415.739699861750069, 213.7658224764589932 ) ) ;
#61166=CARTESIAN_POINT ( 'NONE',  ( 0.5084571940859650141, 1515.143473212400067, 204.7944575026920120 ) ) ;
#61168=CARTESIAN_POINT ( 'NONE',  ( -4.487249772970000272, 1509.038615934189920, 211.6097810847190033 ) ) ;
#61169=CARTESIAN_POINT ( 'NONE',  ( -10.16240527536719895, 1472.558926193989919, 209.8189312950259762 ) ) ;
#61171=CARTESIAN_POINT ( 'NONE',  ( -16.30700481400000257, 1416.815860950479873, 208.9555291761199953 ) ) ;
#61173=CARTESIAN_POINT ( 'NONE',  ( -10.76791425542679903, 1461.753518644530004, 211.3311938081530172 ) ) ;
#61174=CARTESIAN_POINT ( 'NONE',  ( -0.7369207764249980919, 1448.730978137489956, 189.9692764656990107 ) ) ;
#61177=EDGE_CURVE ( 'NONE', #93500, #73642, #65621, .T. ) ;
#61178=CARTESIAN_POINT ( 'NONE',  ( -11.16953914029999950, 1480.956324499390121, 211.2841307966789941 ) ) ;
#61190=CARTESIAN_POINT ( 'NONE',  ( -16.79976345160000406, 1416.845603011260209, 208.5245642856469885 ) ) ;
#61199=CARTESIAN_POINT ( 'NONE',  ( 17.76252328105603695, 1432.742624752195979, 213.6654124838215694 ) ) ;
#61200=CARTESIAN_POINT ( 'NONE',  ( 3.584503077415259753, 1486.500511906220027, 219.3043361390229791 ) ) ;
#61213=CARTESIAN_POINT ( 'NONE',  ( 4.138543415650000057, 1515.492058123790002, 207.2788820903290059 ) ) ;
#61219=CARTESIAN_POINT ( 'NONE',  ( 3.771951471599999994, 1485.940416477589906, 219.2135237292989984 ) ) ;
#61220=CARTESIAN_POINT ( 'NONE',  ( 11.31762120106029990, 1479.526292956740008, 208.6195515253680242 ) ) ;
#61222=CARTESIAN_POINT ( 'NONE',  ( 20.77053033756469702, 1455.448302278209894, 207.2432090845329924 ) ) ;
#61227=CARTESIAN_POINT ( 'NONE',  ( -5.100030730249999422, 1391.870657718589882, 203.7628047703390166 ) ) ;
#61229=CARTESIAN_POINT ( 'NONE',  ( -15.53900113990620113, 1420.370647695649950, 210.6480565532440039 ) ) ;
#61231=CARTESIAN_POINT ( 'NONE',  ( 4.138543391158296281, 1515.492058413688710, 206.7917118350202088 ) ) ;
#61236=CARTESIAN_POINT ( 'NONE',  ( 2.147315937701882227, 1476.624887484032342, 198.5454470367664328 ) ) ;
#61238=CARTESIAN_POINT ( 'NONE',  ( 5.415999934931220672, 1505.806266447880034, 219.5704311486180131 ) ) ;
#61241=EDGE_LOOP ( 'NONE', ( #54507, #77037, #31038, #23481 ) ) ;
#61245=VERTEX_POINT ( 'NONE', #8061 ) ;
#61247=CARTESIAN_POINT ( 'NONE',  ( -10.35637635652009969, 1448.251843012599920, 208.5390742616600050 ) ) ;
#61251=CARTESIAN_POINT ( 'NONE',  ( 6.121488579075629488, 1465.717471025350051, 212.7485050010139958 ) ) ;
#61257=CARTESIAN_POINT ( 'NONE',  ( -10.55504723130449918, 1423.013874365220090, 207.2063886206990162 ) ) ;
#61270=CARTESIAN_POINT ( 'NONE',  ( 2.495485017165389952, 1466.055911289739925, 198.3720333978750148 ) ) ;
#61274=CARTESIAN_POINT ( 'NONE',  ( 8.654266642250069808, 1437.837011637059959, 209.6701303830640200 ) ) ;
#61285=CARTESIAN_POINT ( 'NONE',  ( 2.018257968592299889, 1423.421772701890177, 192.6172488092990136 ) ) ;
#61291=CARTESIAN_POINT ( 'NONE',  ( 8.249359711299819153, 1435.329571781400091, 206.3472986359390120 ) ) ;
#61293=CARTESIAN_POINT ( 'NONE',  ( -3.357462532821310131, 1428.720380741769986, 200.3803434257089862 ) ) ;
#61297=CARTESIAN_POINT ( 'NONE',  ( -11.80920141334000029, 1482.273830016230022, 207.6845722505150036 ) ) ;
#61312=CARTESIAN_POINT ( 'NONE',  ( -1.842963721827329815, 1515.551704300040001, 205.2922259627210053 ) ) ;
#61313=ORIENTED_EDGE ( 'NONE', *, *, #25079, .T. ) ;
#61320=CARTESIAN_POINT ( 'NONE',  ( 3.284535177480000012, 1466.923997773790006, 218.9072142754990011 ) ) ;
#61325=CARTESIAN_POINT ( 'NONE',  ( 0.8066343449330010129, 1430.937684729390185, 200.0727349034889926 ) ) ;
#61326=CARTESIAN_POINT ( 'NONE',  ( 4.758051368188402463, 1442.166524513745799, 216.6176570306145663 ) ) ;
#61327=CARTESIAN_POINT ( 'NONE',  ( -0.8454865857380020611, 1508.321029480389825, 220.8622050322990162 ) ) ;
#61331=CARTESIAN_POINT ( 'NONE',  ( 0.09726404165740129559, 1484.801171650590049, 198.3753413853989969 ) ) ;
#61334=CARTESIAN_POINT ( 'NONE',  ( 12.50980606740000134, 1501.173550771890177, 211.4238265534589800 ) ) ;
#61336=EDGE_CURVE ( 'NONE', #77903, #21803, #24121, .T. ) ;
#61346=CARTESIAN_POINT ( 'NONE',  ( -20.06572793885469963, 1485.934154802469948, 214.0281146234499943 ) ) ;
#61347=ORIENTED_EDGE ( 'NONE', *, *, #11516, .F. ) ;
#61348=CARTESIAN_POINT ( 'NONE',  ( -11.67169904690000060, 1501.458093416090151, 211.3450001677690295 ) ) ;
#61354=B_SPLINE_CURVE_WITH_KNOTS ( 'NONE', 5,
 ( #20498, #54708, #79338, #88834, #97775, #2649, #36777, #12120, #46312, #37887, #106185, #29467 ),
 .UNSPECIFIED., .F., .F.,
 ( 6, 3, 3, 6 ),
 ( 0.000000000000000000, 0.1473537928490198934, 0.5736768964245098079, 1.000000000000000000 ),
 .UNSPECIFIED. ) ;
#61356=CARTESIAN_POINT ( 'NONE',  ( 7.669609405850000172, 1425.609943377740137, 211.8990498311490001 ) ) ;
#61357=CARTESIAN_POINT ( 'NONE',  ( -14.38096556510000035, 1422.143733531690032, 196.2925564653990023 ) ) ;
#61362=VERTEX_POINT ( 'NONE', #104752 ) ;
#61366=CARTESIAN_POINT ( 'NONE',  ( 6.913706168296744892, 1500.103688322486505, 200.0567346946345708 ) ) ;
#61370=CARTESIAN_POINT ( 'NONE',  ( 7.799999999999999822, 1402.913060387289988, 209.1218459616989946 ) ) ;
#61395=CARTESIAN_POINT ( 'NONE',  ( 5.059013353549999259, 1501.257177412389865, 229.8390314845989906 ) ) ;
#61396=CARTESIAN_POINT ( 'NONE',  ( -8.327525192625062189, 1438.484961729265706, 206.5299198730474473 ) ) ;
#61415=CARTESIAN_POINT ( 'NONE',  ( -3.382909239710000016, 1428.856116242189955, 200.7987450405690026 ) ) ;
#61424=CARTESIAN_POINT ( 'NONE',  ( 6.824596843277944913, 1424.786834349993342, 213.4892281956427098 ) ) ;
#61435=CARTESIAN_POINT ( 'NONE',  ( 5.440512190109999757, 1424.738065781850082, 191.9794586101990319 ) ) ;
#61441=EDGE_CURVE ( 'NONE', #74194, #68962, #91906, .T. ) ;
#61447=ORIENTED_EDGE ( 'NONE', *, *, #81103, .F. ) ;
#61455=CARTESIAN_POINT ( 'NONE',  ( -10.47436587960249987, 1490.889567392339814, 212.4387624771430012 ) ) ;
#61456=CARTESIAN_POINT ( 'NONE',  ( -9.299417676539981414, 1446.922214017639817, 190.6945055697750036 ) ) ;
#61460=EDGE_CURVE ( 'NONE', #60549, #27879, #92165, .T. ) ;
#61461=CARTESIAN_POINT ( 'NONE',  ( 10.50858185005970036, 1452.061377940429793, 208.2223096714919848 ) ) ;
#61466=EDGE_LOOP ( 'NONE', ( #68559, #102370, #58064, #81190, #59234, #72935, #3604, #78149, #16325, #86705, #36842, #45001, #52500, #65784 ) ) ;
#61473=CARTESIAN_POINT ( 'NONE',  ( 8.616245162164020144, 1437.218212072470124, 208.3935038613939810 ) ) ;
#61481=CARTESIAN_POINT ( 'NONE',  ( -13.11765501578049964, 1422.301116625370014, 203.8560779122109921 ) ) ;
#61482=CARTESIAN_POINT ( 'NONE',  ( -11.00301372470000061, 1492.094802143589959, 210.0154403701209844 ) ) ;
#61486=CARTESIAN_POINT ( 'NONE',  ( 20.47195266477429954, 1476.322114778060040, 217.8381695920240020 ) ) ;
#61495=CARTESIAN_POINT ( 'NONE',  ( -9.447779140010000631, 1460.630169784690224, 214.7547266466890221 ) ) ;
#61500=CARTESIAN_POINT ( 'NONE',  ( -8.389049334679999248, 1423.485351373390131, 210.3439883204590046 ) ) ;
#61505=CARTESIAN_POINT ( 'NONE',  ( -17.61101880491722582, 1419.781712659406367, 206.7560216166721716 ) ) ;
#61508=CARTESIAN_POINT ( 'NONE',  ( -3.428237969637699667, 1497.215611306809706, 221.0357606766309857 ) ) ;
#61515=CARTESIAN_POINT ( 'NONE',  ( 11.18562212430000002, 1414.421228241719973, 205.5619752052589888 ) ) ;
#61517=CARTESIAN_POINT ( 'NONE',  ( 7.243833416339999332, 1473.411017056090031, 218.0151120354589978 ) ) ;
#61518=CARTESIAN_POINT ( 'NONE',  ( -9.056850508124879795, 1439.359654142089994, 207.7004169096410067 ) ) ;
#61523=FACE_OUTER_BOUND ( 'NONE', #23859, .T. ) ;
#61526=ORIENTED_EDGE ( 'NONE', *, *, #67477, .T. ) ;
#61550=CARTESIAN_POINT ( 'NONE',  ( -2.330134126090000368, 1515.551704408389924, 205.2922258481490303 ) ) ;
#61558=CARTESIAN_POINT ( 'NONE',  ( -17.04997523780000179, 1417.320533121529934, 207.2791714270889827 ) ) ;
#61561=CARTESIAN_POINT ( 'NONE',  ( -0.8395495568287499877, 1420.844234838699776, 193.7400646645540974 ) ) ;
#61568=CARTESIAN_POINT ( 'NONE',  ( 2.550034483959999765, 1426.916722803340235, 188.7149418613990122 ) ) ;
#61572=CARTESIAN_POINT ( 'NONE',  ( 9.680246906815670016, 1463.834245979629941, 210.7210319866079828 ) ) ;
#61577=CIRCLE ( 'NONE', #6159, 7.799999999999999822 ) ;
#61581=CARTESIAN_POINT ( 'NONE',  ( 18.68390451703509925, 1457.534965007319897, 220.6831946007679903 ) ) ;
#61583=CARTESIAN_POINT ( 'NONE',  ( 1732.234191736389675, 11221.53578756870047, 2410.535515148488230 ) ) ;
#61585=CARTESIAN_POINT ( 'NONE',  ( 3.251026391689999961, 1442.093601194490020, 217.4966399718589969 ) ) ;
#61592=CARTESIAN_POINT ( 'NONE',  ( -7.289512158268499853, 1508.551704406979979, 219.1144417387279759 ) ) ;
#61594=B_SPLINE_SURFACE_WITH_KNOTS ( 'NONE', 5, 5, ( 
 ( #86545, #3682, #19323, #87666, #61936, #103900 ),
 ( #52968, #9839, #44006, #70340, #1445, #27200 ),
 ( #44558, #79269, #10955, #78708, #2579, #78143 ),
 ( #46233, #95501, #36701, #71456, #87100, #96615 ),
 ( #10387, #70895, #2021, #62494, #19883, #88215 ),
 ( #79823, #3129, #105011, #80366, #36156, #11509 ) ),
 .UNSPECIFIED., .F., .F., .F.,
 ( 6, 6 ),
 ( 6, 6 ),
 ( 21.97924354190000074, 24.12443845669999831 ),
 ( 0.000000000000000000, 2.000000000000000000 ),
 .UNSPECIFIED. ) ;
#61599=CARTESIAN_POINT ( 'NONE',  ( -2.832025688439999911, 1432.290876391289885, 217.1988707364989750 ) ) ;
#61607=CARTESIAN_POINT ( 'NONE',  ( 12.29736470286800021, 1491.830670002519810, 208.2396171870099977 ) ) ;
#61610=CARTESIAN_POINT ( 'NONE',  ( 9.033634059603929956, 1464.908125515270058, 213.0612947626739810 ) ) ;
#61612=CARTESIAN_POINT ( 'NONE',  ( 1.842962215417941030, 1515.551704407336274, 205.1377642066082672 ) ) ;
#61614=CARTESIAN_POINT ( 'NONE',  ( -1.480799215376189970, 1496.171220128179812, 196.8656195411859926 ) ) ;
#61624=CARTESIAN_POINT ( 'NONE',  ( 0.7135562203500009915, 1457.486859021590135, 199.6029537853190163 ) ) ;
#61647=CARTESIAN_POINT ( 'NONE',  ( 4.751795985444269732, 1508.551704408389924, 212.6676576963480159 ) ) ;
#61652=CARTESIAN_POINT ( 'NONE',  ( 9.691001514874608702, 1460.607649338439842, 206.2887977507070048 ) ) ;
#61658=CARTESIAN_POINT ( 'NONE',  ( 8.185842985679999018, 1424.900152294199870, 195.0776991219990180 ) ) ;
#61667=CARTESIAN_POINT ( 'NONE',  ( 10.01188687081839923, 1451.710540692399945, 207.8449781661669817 ) ) ;
#61682=CARTESIAN_POINT ( 'NONE',  ( -2.546183590178249911, 1469.518995656580046, 218.8843719520340017 ) ) ;
#61685=CARTESIAN_POINT ( 'NONE',  ( 9.219719605386430317, 1450.420523551490078, 208.9716825880909994 ) ) ;
#61688=CARTESIAN_POINT ( 'NONE',  ( -2.243780305749810022, 1421.777182300220147, 193.4398524306369893 ) ) ;
#61691=CARTESIAN_POINT ( 'NONE',  ( -16.37972239500000171, 1503.881811289090138, 209.1238707911080041 ) ) ;
#61694=CARTESIAN_POINT ( 'NONE',  ( -9.950123583630629653, 1439.590930467720227, 208.1650611593379949 ) ) ;
#61701=CARTESIAN_POINT ( 'NONE',  ( 4.554577183490000181, 1505.451005863290220, 220.6211971874989786 ) ) ;
#61702=CARTESIAN_POINT ( 'NONE',  ( -14.25826133790000050, 1415.677402202029953, 214.0085705200789903 ) ) ;
#61703=CARTESIAN_POINT ( 'NONE',  ( -1.179283247376800015, 1515.094876538340031, 204.7931849540779865 ) ) ;
#61705=CARTESIAN_POINT ( 'NONE',  ( -17.31754310717619916, 1417.857287168520088, 205.5202013651170034 ) ) ;
#61723=PRODUCT_DEFINITION ( 'UNKNOWN', '', #56603, #21031 ) ;
#61727=DIRECTION ( 'NONE',  ( 0.000000000000000000, 0.000000000000000000, 1.000000000000000000 ) ) ;
#61734=ORIENTED_EDGE ( 'NONE', *, *, #51525, .F. ) ;
#61743=ADVANCED_FACE ( 'NONE', ( #96222 ), #100167, .T. ) ;
#61751=CARTESIAN_POINT ( 'NONE',  ( 4.217994498490000410, 1515.470302801990101, 208.3798112177819917 ) ) ;
#61757=CARTESIAN_POINT ( 'NONE',  ( 3.428010664469999913, 1421.954222488810274, 194.0794391570989887 ) ) ;
#61759=B_SPLINE_SURFACE_WITH_KNOTS ( 'NONE', 5, 5, ( 
 ( #46173, #78644, #52906, #1388, #104947, #105506 ),
 ( #3618, #19259, #62995, #10325, #35529, #79211 ),
 ( #69723, #1959, #28238, #27689, #61873, #88160 ),
 ( #97103, #80302, #28796, #87038, #37197, #103841 ),
 ( #94889, #45623, #54575, #36641, #10894, #79762 ),
 ( #27142, #53462, #70284, #20369, #18165, #52362 ),
 ( #88710, #61327, #36097, #86479, #95445, #87607 ),
 ( #45068, #2518, #3070, #11990, #107700, #64069 ),
 ( #99275, #91453, #81373, #30434, #47797, #73567 ) ),
 .UNSPECIFIED., .F., .F., .F.,
 ( 6, 3, 6 ),
 ( 6, 6 ),
 ( 3.503225402400000021, 8.166373431240000258, 13.04304411370000061 ),
 ( 0.000000000000000000, 2.000000000000000000 ),
 .UNSPECIFIED. ) ;
#61761=CARTESIAN_POINT ( 'NONE',  ( 20.84180957800000300, 1457.800270462289973, 206.7197162310789906 ) ) ;
#61765=CARTESIAN_POINT ( 'NONE',  ( -5.166416716789999697, 1391.906184330890028, 203.6779378933989904 ) ) ;
#61767=CARTESIAN_POINT ( 'NONE',  ( -11.36252066009999950, 1490.577502786289870, 210.2371618091489722 ) ) ;
#61776=CARTESIAN_POINT ( 'NONE',  ( 8.301429727154969740, 1503.992660670129908, 218.3431214713440056 ) ) ;
#61784=CARTESIAN_POINT ( 'NONE',  ( -0.02999094720359275421, 1457.653887067397136, 199.5863383128643420 ) ) ;
#61791=EDGE_CURVE ( 'NONE', #10311, #26525, #22234, .T. ) ;
#61798=CIRCLE ( 'NONE', #108270, 1.000000000000010436 ) ;
#61799=CARTESIAN_POINT ( 'NONE',  ( -4.877525059390000806, 1387.235931102789891, 214.6572145122790118 ) ) ;
#61800=CARTESIAN_POINT ( 'NONE',  ( -20.26516707829999930, 1485.407934329090040, 205.1093585495989942 ) ) ;
#61803=EDGE_LOOP ( 'NONE', ( #2267, #68400, #67488 ) ) ;
#61811=CARTESIAN_POINT ( 'NONE',  ( 9.727603105489999180, 1462.797525513090022, 208.2922963384270361 ) ) ;
#61812=EDGE_CURVE ( 'NONE', #28705, #28187, #17363, .T. ) ;
#61815=CARTESIAN_POINT ( 'NONE',  ( 2.840552573029999639, 1464.907901564989970, 199.6779196415990043 ) ) ;
#61816=CARTESIAN_POINT ( 'NONE',  ( 8.617688953975729760, 1437.241789755910077, 208.4440105384769879 ) ) ;
#61819=ORIENTED_EDGE ( 'NONE', *, *, #44595, .F. ) ;
#61835=CARTESIAN_POINT ( 'NONE',  ( 5.172586535390000684, 1492.767659076290101, 188.8148697515989909 ) ) ;
#61854=DIRECTION ( 'NONE',  ( -0.9235788661519466203, -0.3792384726311378018, -0.05639378400042227568 ) ) ;
#61861=CARTESIAN_POINT ( 'NONE',  ( 4.487249773072029768, 1509.038615930399828, 211.6097810847319920 ) ) ;
#61871=CARTESIAN_POINT ( 'NONE',  ( 1.799617396100000155, 1431.296477605490281, 200.2099161714889988 ) ) ;
#61872=CARTESIAN_POINT ( 'NONE',  ( 10.15211825780419197, 1462.852281282112926, 213.4500083841329854 ) ) ;
#61873=CARTESIAN_POINT ( 'NONE',  ( 2.444246758109999806, 1506.180962866889786, 221.2807778021990259 ) ) ;
#61879=CARTESIAN_POINT ( 'NONE',  ( -0.4112623051359989845, 1484.199768852090074, 198.4089546266989998 ) ) ;
#61880=CARTESIAN_POINT ( 'NONE',  ( 4.362527623401529553, 1466.289975156470064, 199.7053707134959950 ) ) ;
#61882=CARTESIAN_POINT ( 'NONE',  ( 5.172586535390000684, 1492.767659076290101, 188.8148697515989909 ) ) ;
#61886=B_SPLINE_CURVE_WITH_KNOTS ( 'NONE', 5,
 ( #82803, #13930, #23980, #39136, #73314, #74983 ),
 .UNSPECIFIED., .F., .F.,
 ( 6, 6 ),
 ( 0.000000000000000000, 1.000000000000000000 ),
 .UNSPECIFIED. ) ;
#61896=CARTESIAN_POINT ( 'NONE',  ( -15.85591190879999779, 1415.880081504350073, 209.4912631162540038 ) ) ;
#61897=CARTESIAN_POINT ( 'NONE',  ( -0.1314159319799989845, 1442.749364073790048, 202.9452834803589951 ) ) ;
#61899=CARTESIAN_POINT ( 'NONE',  ( -9.862207263486190811, 1438.620019707270103, 210.3541762680239913 ) ) ;
#61904=CARTESIAN_POINT ( 'NONE',  ( 7.681541415779999937, 1425.833909046620192, 211.9025755004689984 ) ) ;
#61905=CARTESIAN_POINT ( 'NONE',  ( 8.129467950829999623, 1461.711574958590063, 228.8738014342989970 ) ) ;
#61913=CIRCLE ( 'NONE', #90482, 7.146147325060000277 ) ;
#61922=CARTESIAN_POINT ( 'NONE',  ( -2.641120632158299841, 1464.700422726399893, 198.8576235399000041 ) ) ;
#61931=DIRECTION ( 'NONE',  ( 0.4428464831282420966, -0.8932998904726507927, -0.07682641513501356489 ) ) ;
#61933=ORIENTED_EDGE ( 'NONE', *, *, #48738, .F. ) ;
#61936=CARTESIAN_POINT ( 'NONE',  ( -4.267145199109999787, 1453.908306484889863, 199.9833665867990078 ) ) ;
#61943=CARTESIAN_POINT ( 'NONE',  ( 15.66449074470000014, 1427.615315534789943, 199.7467549911789888 ) ) ;
#61950=CARTESIAN_POINT ( 'NONE',  ( 9.481395134947719683, 1462.257910684749959, 206.9075228777909956 ) ) ;
#61954=EDGE_CURVE ( 'NONE', #37990, #43895, #27668, .T. ) ;
#61955=DIRECTION ( 'NONE',  ( -0.02616798426500960631, 0.9993150019883682011, 0.02616798426500950570 ) ) ;
#61960=ADVANCED_FACE ( 'NONE', ( #26098, #86025 ), #77633, .T. ) ;
#61964=CARTESIAN_POINT ( 'NONE',  ( -8.557209110492459914, 1448.617779613390212, 212.3361752075699940 ) ) ;
#61965=CARTESIAN_POINT ( 'NONE',  ( -13.67844609351699958, 1504.250379464319849, 227.6838296026270143 ) ) ;
#61968=DIRECTION ( 'NONE',  ( 9.230617842401318720E-47, -1.000000000000000000, 1.836970198721029688E-16 ) ) ;
#61977=CARTESIAN_POINT ( 'NONE',  ( 10.73803961559999998, 1423.675746264540066, 203.2436441965290044 ) ) ;
#61982=CARTESIAN_POINT ( 'NONE',  ( 10.73061977934889910, 1470.167071072400176, 207.1537691930359983 ) ) ;
#61983=ORIENTED_EDGE ( 'NONE', *, *, #37814, .T. ) ;
#61985=CARTESIAN_POINT ( 'NONE',  ( 9.018659374699888431, 1423.185120360550172, 211.3902366515449955 ) ) ;
#61987=ORIENTED_EDGE ( 'NONE', *, *, #23436, .F. ) ;
#61991=CARTESIAN_POINT ( 'NONE',  ( 3.015233801489999976, 1443.190137595490114, 217.5000105274690156 ) ) ;
#61999=CARTESIAN_POINT ( 'NONE',  ( -4.993938974811324094, 1391.677352696793832, 203.5345363725389802 ) ) ;
#62005=CARTESIAN_POINT ( 'NONE',  ( -4.450958129710000044, 1483.189406595490027, 199.4355188422489960 ) ) ;
#62010=CARTESIAN_POINT ( 'NONE',  ( -6.080444312649149197, 1488.995743380849945, 218.2866348719960001 ) ) ;
#62012=CARTESIAN_POINT ( 'NONE',  ( 18.68389199464829886, 1457.534885685930021, 220.6832065729649912 ) ) ;
#62015=CARTESIAN_POINT ( 'NONE',  ( -5.045364366626095887, 1391.811351688237664, 214.6675329302748594 ) ) ;
#62024=CARTESIAN_POINT ( 'NONE',  ( -20.69303424980000372, 1486.764600954290017, 209.1218459616989946 ) ) ;
#62030=CARTESIAN_POINT ( 'NONE',  ( -5.445054425793269814, 1494.866999379700246, 198.0707246423999948 ) ) ;
#62038=CARTESIAN_POINT ( 'NONE',  ( -14.29542475900360010, 1421.697851824200143, 203.6378746937919857 ) ) ;
#62040=CARTESIAN_POINT ( 'NONE',  ( 2.484906683780000236, 1472.794382616990106, 219.0213525527389891 ) ) ;
#62043=CARTESIAN_POINT ( 'NONE',  ( -17.81193786781770427, 1488.806627658329944, 195.1587721144809962 ) ) ;
#62045=CARTESIAN_POINT ( 'NONE',  ( 9.539810668950000405, 1420.903745483679813, 197.1733355697989793 ) ) ;
#62054=CARTESIAN_POINT ( 'NONE',  ( -6.496128480939999505, 1458.243874865590215, 216.1639725907290028 ) ) ;
#62067=CARTESIAN_POINT ( 'NONE',  ( 2.236830499208590339, 1495.676457082710158, 221.2569898128769807 ) ) ;
#62068=ORIENTED_EDGE ( 'NONE', *, *, #93114, .F. ) ;
#62072=CARTESIAN_POINT ( 'NONE',  ( -11.52804851922353890, 1414.677402202029953, 206.9304647618809270 ) ) ;
#62073=CARTESIAN_POINT ( 'NONE',  ( -17.76510163610419823, 1508.542006963650238, 211.8150015411889910 ) ) ;
#62074=CARTESIAN_POINT ( 'NONE',  ( 7.881803347790000025, 1471.528388462790190, 215.6156897165890030 ) ) ;
#62075=CARTESIAN_POINT ( 'NONE',  ( -9.522384955721390654, 1439.330048506679987, 208.4251047430030042 ) ) ;
#62080=CARTESIAN_POINT ( 'NONE',  ( 8.505169765932141246, 1436.416344830570097, 207.7641285517320000 ) ) ;
#62107=CARTESIAN_POINT ( 'NONE',  ( -3.750390061399999642, 1495.937738748590164, 198.1516812963990049 ) ) ;
#62117=CARTESIAN_POINT ( 'NONE',  ( -18.55121668013607206, 1466.210258097253245, 216.5807023832959999 ) ) ;
#62122=CARTESIAN_POINT ( 'NONE',  ( -4.327218846663630103, 1515.149950449780135, 208.7360365624930125 ) ) ;
#62126=CARTESIAN_POINT ( 'NONE',  ( -1.842963219480119985, 1515.064792700640055, 204.7923971808919816 ) ) ;
#62129=CARTESIAN_POINT ( 'NONE',  ( 3.026717173399090299, 1424.965164304149994, 188.8885481931689867 ) ) ;
#62133=CARTESIAN_POINT ( 'NONE',  ( 9.677599926597229896, 1463.237891885529962, 210.5383111002819874 ) ) ;
#62136=CARTESIAN_POINT ( 'NONE',  ( -1.532299087870000021, 1444.082491599790046, 199.5897746526189849 ) ) ;
#62139=CARTESIAN_POINT ( 'NONE',  ( -16.48256533165833204, 1420.110686815605959, 208.7021220505580743 ) ) ;
#62142=CARTESIAN_POINT ( 'NONE',  ( -3.865363954398979729, 1508.610338847399817, 204.7110934479420052 ) ) ;
#62146=CARTESIAN_POINT ( 'NONE',  ( 3.814972826460000022, 1441.101450695089852, 217.8538525646389985 ) ) ;
#62150=CARTESIAN_POINT ( 'NONE',  ( -3.951758682210000817, 1475.564030158489913, 199.4458604787490117 ) ) ;
#62153=CARTESIAN_POINT ( 'NONE',  ( -6.305951052519140454, 1508.551704408389924, 219.3648472223130170 ) ) ;
#62159=CARTESIAN_POINT ( 'NONE',  ( -3.220674682859999916, 1433.265634983390100, 218.1214075930489855 ) ) ;
#62160=CARTESIAN_POINT ( 'NONE',  ( -10.72965402270880020, 1471.641146218699987, 206.8906404078279877 ) ) ;
#62168=CARTESIAN_POINT ( 'NONE',  ( 10.95588612120169891, 1490.084719449429940, 208.7631480041860357 ) ) ;
#62169=CARTESIAN_POINT ( 'NONE',  ( -3.767448257705639847, 1438.693583706480013, 227.3301816780199829 ) ) ;
#62177=CARTESIAN_POINT ( 'NONE',  ( 11.98162358222930024, 1427.378834198339973, 208.3083443427269970 ) ) ;
#62187=DIRECTION ( 'NONE',  ( 1.224227143275421080E-16, 0.02617694830808806397, -0.9996573249755517088 ) ) ;
#62209=ORIENTED_EDGE ( 'NONE', *, *, #42040, .F. ) ;
#62212=CARTESIAN_POINT ( 'NONE',  ( 10.13538064839599961, 1453.511863947389884, 212.2751250215330003 ) ) ;
#62213=CARTESIAN_POINT ( 'NONE',  ( 9.146125554490000198, 1424.112737737530097, 196.6908568651990095 ) ) ;
#62223=CARTESIAN_POINT ( 'NONE',  ( 5.059013353549999259, 1501.257177412389865, 229.8390314845989906 ) ) ;
#62225=EDGE_LOOP ( 'NONE', ( #4130, #4938, #69313, #104230 ) ) ;
#62235=CARTESIAN_POINT ( 'NONE',  ( -8.848880573389370952, 1470.096389303520255, 214.8940742741490055 ) ) ;
#62238=CARTESIAN_POINT ( 'NONE',  ( 9.191577631451519181, 1450.202143376990080, 208.5180113977080225 ) ) ;
#62240=CARTESIAN_POINT ( 'NONE',  ( 10.46269290780000105, 1491.122602396189905, 212.5073314721190059 ) ) ;
#62243=CARTESIAN_POINT ( 'NONE',  ( -20.32158151839999860, 1505.095178026389931, 209.5373622212030114 ) ) ;
#62244=CARTESIAN_POINT ( 'NONE',  ( -1.541850711665649963E-13, 1515.064792882589927, 213.4512947377390049 ) ) ;
#62245=CARTESIAN_POINT ( 'NONE',  ( 10.97694524628009916, 1422.961345275170061, 206.9164947625000082 ) ) ;
#62247=CARTESIAN_POINT ( 'NONE',  ( -9.877301730868230933, 1439.855027102960094, 207.5146903145040085 ) ) ;
#62249=ORIENTED_EDGE ( 'NONE', *, *, #16467, .T. ) ;
#62254=CARTESIAN_POINT ( 'NONE',  ( 5.062625036090000030, 1505.549198612089867, 220.0219801153990034 ) ) ;
#62256=CARTESIAN_POINT ( 'NONE',  ( -1.629715277743620128, 1515.068677689339893, 204.7924989132399958 ) ) ;
#62258=CARTESIAN_POINT ( 'NONE',  ( -15.84040666245470064, 1415.881310014747442, 209.7199984178415093 ) ) ;
#62261=CARTESIAN_POINT ( 'NONE',  ( -19.15298488520000220, 1464.559837765089924, 213.8319524061190009 ) ) ;
#62268=CARTESIAN_POINT ( 'NONE',  ( -6.369643009819999868, 1476.618821349690052, 217.4015008671389921 ) ) ;
#62269=AXIS2_PLACEMENT_3D ( 'NONE', #88319, #11614, #45790 ) ;
#62280=DIRECTION ( 'NONE',  ( 4.465978680329379737E-17, 1.000000000000000000, -2.349386720892264891E-16 ) ) ;
#62294=CARTESIAN_POINT ( 'NONE',  ( -13.13536861967500080, 1507.686078907830051, 209.3105439006200186 ) ) ;
#62307=B_SPLINE_CURVE_WITH_KNOTS ( 'NONE', 5,
 ( #1801, #77930, #18003, #1237, #42675, #76278 ),
 .UNSPECIFIED., .F., .F.,
 ( 6, 6 ),
 ( 302.5784080160000258, 307.6101328560000070 ),
 .UNSPECIFIED. ) ;
#62310=CARTESIAN_POINT ( 'NONE',  ( 4.175269160410000069, 1515.456655180189955, 207.6381344832090008 ) ) ;
#62316=CARTESIAN_POINT ( 'NONE',  ( 0.3057263173670020096, 1422.515503742850115, 193.2688871159990072 ) ) ;
#62319=CARTESIAN_POINT ( 'NONE',  ( 0.5708501887139260100, 1460.784142812889968, 230.4191102857249973 ) ) ;
#62325=CARTESIAN_POINT ( 'NONE',  ( -11.10693645390000128, 1491.078836222690143, 210.0430879654600176 ) ) ;
#62332=CARTESIAN_POINT ( 'NONE',  ( -1778.470085355049832, -2339.246371527900010, 9314.971673131300122 ) ) ;
#62351=CARTESIAN_POINT ( 'NONE',  ( -9.873494421475939475, 1422.989223822590020, 208.5817921780659958 ) ) ;
#62352=CARTESIAN_POINT ( 'NONE',  ( 16.85775989529999919, 1430.051104475889815, 201.2392674849789955 ) ) ;
#62353=ORIENTED_EDGE ( 'NONE', *, *, #4323, .F. ) ;
#62354=CARTESIAN_POINT ( 'NONE',  ( -17.51440181060990042, 1442.103983326210027, 219.2287785421630133 ) ) ;
#62363=CARTESIAN_POINT ( 'NONE',  ( 10.94770426880000080, 1460.983543286389931, 208.7734656400390065 ) ) ;
#62379=CARTESIAN_POINT ( 'NONE',  ( 3.420678028885419941, 1423.764636203429973, 192.8424018407250173 ) ) ;
#62381=CARTESIAN_POINT ( 'NONE',  ( -5.102340803919999779, 1483.010473641589897, 199.7820758705289848 ) ) ;
#62383=CARTESIAN_POINT ( 'NONE',  ( -2.416613126590000160, 1507.334987533289905, 221.5267771657990181 ) ) ;
#62384=EDGE_CURVE ( 'NONE', #19394, #98779, #82028, .T. ) ;
#62386=CARTESIAN_POINT ( 'NONE',  ( 18.29188182340000068, 1431.768652859389704, 209.1218459616989946 ) ) ;
#62390=CARTESIAN_POINT ( 'NONE',  ( -0.5614708061910009818, 1469.825031502190086, 216.3963468629289935 ) ) ;
#62395=FACE_OUTER_BOUND ( 'NONE', #35891, .T. ) ;
#62396=CARTESIAN_POINT ( 'NONE',  ( -3.423171246829689984, 1483.455259025470241, 199.0242790757120019 ) ) ;
#62402=CARTESIAN_POINT ( 'NONE',  ( -14.83515152120000025, 1415.726119505169891, 205.6144808782789823 ) ) ;
#62407=CARTESIAN_POINT ( 'NONE',  ( -9.526026435753081500, 1449.078195667740147, 208.0234617775689969 ) ) ;
#62413=CARTESIAN_POINT ( 'NONE',  ( -1.129779230740000084, 1515.569191395689813, 213.0910028086289856 ) ) ;
#62431=EDGE_CURVE ( 'NONE', #36236, #76707, #16107, .T. ) ;
#62432=CARTESIAN_POINT ( 'NONE',  ( 2.998248178699999933, 1486.828675832889985, 197.9694548352990182 ) ) ;
#62451=CARTESIAN_POINT ( 'NONE',  ( -11.33467682473018989, 1502.178027852193054, 207.3042251687307669 ) ) ;
#62454=CARTESIAN_POINT ( 'NONE',  ( -17.28616084879999804, 1505.118892507889996, 223.1516167556989956 ) ) ;
#62456=CARTESIAN_POINT ( 'NONE',  ( -9.976093183941980413, 1439.379388325520040, 208.6707327245020167 ) ) ;
#62458=ADVANCED_FACE ( 'NONE', ( #40866 ), #83192, .T. ) ;
#62459=FACE_OUTER_BOUND ( 'NONE', #30261, .T. ) ;
#62462=CARTESIAN_POINT ( 'NONE',  ( 7.598639282229999736, 1424.430323257039845, 212.2253573777790052 ) ) ;
#62493=VERTEX_POINT ( 'NONE', #107519 ) ;
#62494=CARTESIAN_POINT ( 'NONE',  ( -3.410565249569999846, 1454.671646890489910, 199.9594833787289758 ) ) ;
#62496=VECTOR ( 'NONE', #9919, 999.9999999999998863 ) ;
#62511=ORIENTED_EDGE ( 'NONE', *, *, #43802, .F. ) ;
#62513=CARTESIAN_POINT ( 'NONE',  ( 3.060046442946298573, 1442.201648411282804, 217.5704250861406592 ) ) ;
#62523=CARTESIAN_POINT ( 'NONE',  ( -21.44637720709119577, 1506.412686512840082, 216.0243823771180018 ) ) ;
#62528=( BOUNDED_CURVE ( )  B_SPLINE_CURVE ( 3, ( #71925, #38809, #89770, #30965 ),
 .UNSPECIFIED., .F., .T. ) 
 B_SPLINE_CURVE_WITH_KNOTS ( ( 4, 4 ),
 ( 4.672237621782279859, 4.820400371478359425 ),
 .UNSPECIFIED. ) 
 CURVE ( )  GEOMETRIC_REPRESENTATION_ITEM ( )  RATIONAL_B_SPLINE_CURVE ( ( 1.000000000000000000, 0.9981714864442265966, 0.9981714864442265966, 1.000000000000000000 ) ) 
 REPRESENTATION_ITEM ( '' )  );
#62534=CARTESIAN_POINT ( 'NONE',  ( -2.480175237380000119, 1429.207669949490082, 200.0830572027790026 ) ) ;
#62544=CARTESIAN_POINT ( 'NONE',  ( 9.903643697897789977, 1469.012723375830092, 207.5198563789629986 ) ) ;
#62555=CARTESIAN_POINT ( 'NONE',  ( 2.907186931900000104, 1441.882235772590093, 217.8664262967990055 ) ) ;
#62568=CARTESIAN_POINT ( 'NONE',  ( -7.756912786389999148, 1508.430206397490110, 219.4938868140989996 ) ) ;
#62572=CARTESIAN_POINT ( 'NONE',  ( -1.954671169420000076, 1485.152615037190117, 198.1756556538989855 ) ) ;
#62574=CARTESIAN_POINT ( 'NONE',  ( -16.53125420670000167, 1418.541487540729804, 202.7561987471289910 ) ) ;
#62577=B_SPLINE_SURFACE_WITH_KNOTS ( 'NONE', 5, 5, ( 
 ( #69609, #1281, #42170, #51128, #70173, #102054 ),
 ( #34314, #103728, #110472, #102593, #25893, #69053 ),
 ( #76322, #50577, #18593, #27030, #84704, #33750 ),
 ( #8004, #103153, #77975, #67944, #77431, #16380 ),
 ( #9656, #34864, #25338, #16926, #59532, #52791 ),
 ( #43828, #85253, #52245, #17482, #93644, #86371 ),
 ( #35422, #61219, #60649, #94772, #24779, #26455 ),
 ( #8552, #732, #95333, #78536, #86925, #44394 ),
 ( #60092, #58978, #93109, #10216, #42724, #1847 ) ),
 .UNSPECIFIED., .F., .F., .F.,
 ( 6, 3, 6 ),
 ( 6, 6 ),
 ( 0.000000000000000000, 1.560949918229999955, 3.121899836449999910 ),
 ( 0.000000000000000000, 2.000000000000000000 ),
 .UNSPECIFIED. ) ;
#62581=EDGE_CURVE ( 'NONE', #26364, #86670, #26709, .T. ) ;
#62582=CARTESIAN_POINT ( 'NONE',  ( -4.237929439762339712, 1486.921074483630036, 220.3845766509240036 ) ) ;
#62583=CARTESIAN_POINT ( 'NONE',  ( -22.15968325629999924, 1485.573345355790025, 217.2083650093589995 ) ) ;
#62587=CARTESIAN_POINT ( 'NONE',  ( 7.069907484889999871, 1426.666557891380080, 213.2414385277990050 ) ) ;
#62590=CIRCLE ( 'NONE', #67919, 1.999999999999994227 ) ;
#62601=CARTESIAN_POINT ( 'NONE',  ( 9.390592470051840834, 1435.626267691329986, 208.9162517377799873 ) ) ;
#62603=CARTESIAN_POINT ( 'NONE',  ( 11.45577226660000036, 1502.286415424589904, 208.3140783707030153 ) ) ;
#62607=CARTESIAN_POINT ( 'NONE',  ( -1.475794679986299984, 1515.075282686699893, 213.4510200518020042 ) ) ;
#62610=CARTESIAN_POINT ( 'NONE',  ( -15.83806605205309914, 1420.932712493960025, 203.3750394557980314 ) ) ;
#62616=CARTESIAN_POINT ( 'NONE',  ( -22.18488176075830154, 1483.996195745850173, 216.8908803982089921 ) ) ;
#62618=CARTESIAN_POINT ( 'NONE',  ( 12.02531869610000115, 1420.571450649919825, 199.9272147486889821 ) ) ;
#62629=CARTESIAN_POINT ( 'NONE',  ( -7.961002066000000710, 1424.384911837800018, 210.5206767801589933 ) ) ;
#62639=CARTESIAN_POINT ( 'NONE',  ( 9.578155386300000629, 1471.786587761589772, 213.7186015179489971 ) ) ;
#62640=CARTESIAN_POINT ( 'NONE',  ( -9.671333196654149589, 1440.258410182710122, 206.4805632831669868 ) ) ;
#62641=ORIENTED_EDGE ( 'NONE', *, *, #3143, .F. ) ;
#62645=CARTESIAN_POINT ( 'NONE',  ( 9.528477832624719923, 1434.647097723040133, 206.8891366029810115 ) ) ;
#62650=CARTESIAN_POINT ( 'NONE',  ( 11.38585543042319870, 1471.209044977530084, 209.9613054878209937 ) ) ;
#62666=ADVANCED_FACE ( 'NONE', ( #79448 ), #5379, .T. ) ;
#62676=CARTESIAN_POINT ( 'NONE',  ( 17.76546875260000036, 1430.865606781589804, 204.9340536459789917 ) ) ;
#62680=CARTESIAN_POINT ( 'NONE',  ( -17.28926732269999889, 1417.627268025079957, 207.2086015117089914 ) ) ;
#62692=B_SPLINE_SURFACE_WITH_KNOTS ( 'NONE', 5, 5, ( 
 ( #58568, #83207, #48521, #82660, #5951, #74278 ),
 ( #49072, #33335, #31139, #14881, #84303, #56910 ),
 ( #110060, #107850, #65324, #40096, #66432, #75376 ),
 ( #74819, #5395, #31689, #24384, #40648, #41749 ),
 ( #82094, #65871, #99991, #100548, #50175, #108965 ),
 ( #23828, #58020, #93251, #92155, #49619, #75908 ),
 ( #39553, #83752, #7048, #99434, #41206, #23283 ),
 ( #32791, #67530, #7594, #91043, #101630, #24919 ),
 ( #59129, #73727, #78109, #95470, #43422, #8137 ) ),
 .UNSPECIFIED., .F., .F., .F.,
 ( 6, 3, 6 ),
 ( 6, 6 ),
 ( 6.826668448630000685E-15, 3.228996143019999820, 6.457992286039999641 ),
 ( 0.000000000000000000, 2.000000000000000000 ),
 .UNSPECIFIED. ) ;
#62693=CARTESIAN_POINT ( 'NONE',  ( -9.622986749620970670, 1460.696243629709898, 210.1029813304209881 ) ) ;
#62695=CARTESIAN_POINT ( 'NONE',  ( 10.57324062335630011, 1500.889090984059976, 204.6344996329069943 ) ) ;
#62696=ORIENTED_EDGE ( 'NONE', *, *, #101364, .F. ) ;
#62705=CARTESIAN_POINT ( 'NONE',  ( -13.53908046754547634, 1489.771924351148527, 192.3260543307453361 ) ) ;
#62709=CARTESIAN_POINT ( 'NONE',  ( -16.91899155701270629, 1419.993940084556698, 207.8764500463518630 ) ) ;
#62710=CARTESIAN_POINT ( 'NONE',  ( 7.156887453669999566, 1427.109879847909951, 213.1306117699590175 ) ) ;
#62712=CARTESIAN_POINT ( 'NONE',  ( -2.537545712159490652, 1430.163801573863793, 201.1758857049043741 ) ) ;
#62714=CARTESIAN_POINT ( 'NONE',  ( 5.597778194180000888, 1506.679269386989972, 219.3685102149989916 ) ) ;
#62715=CARTESIAN_POINT ( 'NONE',  ( -2.330134126628495839, 1515.551704408385831, 205.1377642093399061 ) ) ;
#62716=CARTESIAN_POINT ( 'NONE',  ( -2.873810095670000120, 1489.508126606890073, 188.4097326925989933 ) ) ;
#62717=EDGE_LOOP ( 'NONE', ( #16101, #78315, #41960, #5663 ) ) ;
#62720=CARTESIAN_POINT ( 'NONE',  ( -4.301547056329999563, 1475.041466652889994, 199.3382836939389904 ) ) ;
#62723=CARTESIAN_POINT ( 'NONE',  ( -6.236956084921230214, 1508.551704408389924, 219.3822772563589751 ) ) ;
#62727=CARTESIAN_POINT ( 'NONE',  ( 3.394586470828380165, 1484.752177860970050, 220.4731790445629827 ) ) ;
#62728=CARTESIAN_POINT ( 'NONE',  ( 3.219589608733330000, 1465.067515351920065, 202.8483799685759834 ) ) ;
#62729=CARTESIAN_POINT ( 'NONE',  ( -2.059804321870000177, 1432.536759692389978, 218.0320281295389861 ) ) ;
#62736=EDGE_CURVE ( 'NONE', #9292, #104222, #11601, .T. ) ;
#62739=CARTESIAN_POINT ( 'NONE',  ( 10.93211270434609972, 1490.535788348610140, 207.1035467188879977 ) ) ;
#62741=ORIENTED_EDGE ( 'NONE', *, *, #72026, .F. ) ;
#62744=CARTESIAN_POINT ( 'NONE',  ( -3.329590635812200272, 1495.609068625810096, 197.2492212534749854 ) ) ;
#62747=CARTESIAN_POINT ( 'NONE',  ( 12.11032223851909961, 1427.313662735290109, 207.9400900094899782 ) ) ;
#62754=B_SPLINE_CURVE_WITH_KNOTS ( 'NONE', 3,
 ( #36665, #106612, #72482, #2541, #104416, #45646, #79786, #21480, #47271, #3091, #81393, #36120, #27709, #19283, #53485, #104970, #5824, #92023, #83609, #90914, #108821, #74688, #14754, #30458, #31555, #100955, #6363, #83072, #40511, #74139, #32117, #66302, #107166, #64642 ),
 .UNSPECIFIED., .F., .F.,
 ( 4, 3, 3, 3, 3, 3, 3, 3, 3, 3, 3, 4 ),
 ( -1.000000000000000000, -0.9332700196348299171, -0.8419690754577389136, -0.7491820742414060375, -0.6555871093692909879, -0.5609708486710199837, -0.4660560511319400412, -0.3711766688345579102, -0.2766611810049399711, -0.1833255963325950422, -0.09105965716530861620, -9.978666077881115370E-07 ),
 .UNSPECIFIED. ) ;
#62758=CARTESIAN_POINT ( 'NONE',  ( 2.236830496430000537, 1495.676457072290077, 221.2569898083989699 ) ) ;
#62765=B_SPLINE_CURVE_WITH_KNOTS ( 'NONE', 3,
 ( #24549, #42476, #76633, #110785, #59853, #93977, #86688 ),
 .UNSPECIFIED., .F., .F.,
 ( 4, 3, 4 ),
 ( -2.813093253849999975, -1.406546626924999988, 0.000000000000000000 ),
 .UNSPECIFIED. ) ;
#62766=VECTOR ( 'NONE', #24415, 1000.000000000000114 ) ;
#62778=B_SPLINE_CURVE_WITH_KNOTS ( 'NONE', 3,
 ( #26726, #95043, #35680, #19420, #69871, #18312, #96142 ),
 .UNSPECIFIED., .F., .F.,
 ( 4, 3, 4 ),
 ( -9.215058517400001037, -7.151230857792230111, -3.489946704171289937 ),
 .UNSPECIFIED. ) ;
#62779=CARTESIAN_POINT ( 'NONE',  ( 8.977953201188558552, 1452.688148568789984, 212.1107650675139951 ) ) ;
#62781=VERTEX_POINT ( 'NONE', #96100 ) ;
#62782=CARTESIAN_POINT ( 'NONE',  ( -3.068245697174119879, 1507.352576251979826, 221.6096153556280228 ) ) ;
#62790=CARTESIAN_POINT ( 'NONE',  ( 19.33983739529999824, 1457.046864427589981, 207.2645132519189985 ) ) ;
#62801=FACE_OUTER_BOUND ( 'NONE', #26944, .T. ) ;
#62802=CARTESIAN_POINT ( 'NONE',  ( 5.854932897769000277, 1498.860406282120039, 199.1309772468239885 ) ) ;
#62804=CARTESIAN_POINT ( 'NONE',  ( -10.29448394224809959, 1469.837462831460016, 213.9188779471319890 ) ) ;
#62809=CARTESIAN_POINT ( 'NONE',  ( 9.090063749209999600, 1493.398504240489956, 216.3232041073590040 ) ) ;
#62810=CARTESIAN_POINT ( 'NONE',  ( 11.16991425404440008, 1478.699414125650037, 205.8835566445779932 ) ) ;
#62811=CARTESIAN_POINT ( 'NONE',  ( 9.152530698324561342, 1425.159826229013106, 195.6020820322053737 ) ) ;
#62812=CARTESIAN_POINT ( 'NONE',  ( -12.76080126299999939, 1502.832725690589996, 208.7536821347480043 ) ) ;
#62817=CARTESIAN_POINT ( 'NONE',  ( -9.927113458974829996, 1439.694740119939979, 207.9119407081149973 ) ) ;
#62820=EDGE_LOOP ( 'NONE', ( #75391, #32683, #106773, #12710 ) ) ;
#62825=CARTESIAN_POINT ( 'NONE',  ( 3.628818059389999906, 1505.602008401590183, 221.3635115024989943 ) ) ;
#62826=CARTESIAN_POINT ( 'NONE',  ( -14.60558100029999906, 1415.677402203979909, 212.8314178026089962 ) ) ;
#62827=CARTESIAN_POINT ( 'NONE',  ( -16.14632490511739960, 1420.004730576690008, 210.0172707792249867 ) ) ;
#62829=CARTESIAN_POINT ( 'NONE',  ( -15.81740104567429661, 1415.848495208088252, 209.7113497446936776 ) ) ;
#62831=CARTESIAN_POINT ( 'NONE',  ( -10.07154918488590134, 1473.228065907060000, 207.4129428866500007 ) ) ;
#62832=B_SPLINE_CURVE_WITH_KNOTS ( 'NONE', 5,
 ( #102763, #52414, #60254, #87662, #105006, #26628 ),
 .UNSPECIFIED., .F., .F.,
 ( 6, 6 ),
 ( -2.079987011550000098, 0.000000000000000000 ),
 .UNSPECIFIED. ) ;
#62833=CARTESIAN_POINT ( 'NONE',  ( -16.11828785200000169, 1416.352749337680279, 209.2475168326350001 ) ) ;
#62837=DIRECTION ( 'NONE',  ( -1.224646799147350002E-16, 1.836970198721029688E-16, 1.000000000000000000 ) ) ;
#62842=CARTESIAN_POINT ( 'NONE',  ( -7.980162432014145324, 1424.804287484062115, 210.5240428484218853 ) ) ;
#62851=ADVANCED_FACE ( 'NONE', ( #42772 ), #6231, .T. ) ;
#62854=CARTESIAN_POINT ( 'NONE',  ( -14.91495772972460010, 1417.818891793210014, 203.2118081904590099 ) ) ;
#62856=PLANE ( 'NONE',  #24118 ) ;
#62858=CARTESIAN_POINT ( 'NONE',  ( -16.31825947160000112, 1416.692283692869978, 208.5165952855510056 ) ) ;
#62860=EDGE_CURVE ( 'NONE', #69308, #27986, #29406, .T. ) ;
#62864=CARTESIAN_POINT ( 'NONE',  ( -15.46337246819999933, 1416.177402202029953, 209.5778879521189992 ) ) ;
#62869=CARTESIAN_POINT ( 'NONE',  ( -12.76561250770870082, 1508.446853715159932, 209.6296519742829787 ) ) ;
#62882=CARTESIAN_POINT ( 'NONE',  ( 4.045201229639999951, 1515.528102034789981, 207.6334507866089893 ) ) ;
#62890=CARTESIAN_POINT ( 'NONE',  ( 0.2516559519770019682, 1422.814445642939972, 192.8915334538990010 ) ) ;
#62893=CARTESIAN_POINT ( 'NONE',  ( 10.75633763354679928, 1451.138011284190043, 190.3409219236589820 ) ) ;
#62898=CARTESIAN_POINT ( 'NONE',  ( 3.074703616360000336, 1441.333178363689967, 218.5515150763889949 ) ) ;
#62899=CARTESIAN_POINT ( 'NONE',  ( -2201.413669186790685, 11221.53578756870047, 1941.356037698088358 ) ) ;
#62906=CARTESIAN_POINT ( 'NONE',  ( -9.215151402819998339, 1422.993424535609847, 210.2744618676390189 ) ) ;
#62907=CARTESIAN_POINT ( 'NONE',  ( -10.61736893638143187, 1422.368802841423076, 210.6403487152534240 ) ) ;
#62913=CARTESIAN_POINT ( 'NONE',  ( 0.4444123522354649358, 1457.844269246920703, 199.5878175327990505 ) ) ;
#62914=CARTESIAN_POINT ( 'NONE',  ( -10.61999665778870039, 1462.990853173620053, 206.0510134237090085 ) ) ;
#62917=CARTESIAN_POINT ( 'NONE',  ( 8.768196648836839913, 1461.433371597579935, 227.1471525255139738 ) ) ;
#62927=CARTESIAN_POINT ( 'NONE',  ( 10.37958320015649960, 1453.090533085269954, 190.0119578831939862 ) ) ;
#62928=CARTESIAN_POINT ( 'NONE',  ( -2.306705840230210303, 1431.167757009700154, 201.0655358790060063 ) ) ;
#62936=CARTESIAN_POINT ( 'NONE',  ( 9.739858402530000347, 1462.441346130390002, 208.6777580896069821 ) ) ;
#62938=CARTESIAN_POINT ( 'NONE',  ( -19.09790268268400126, 1508.458003811930212, 210.0050661408479868 ) ) ;
#62940=CARTESIAN_POINT ( 'NONE',  ( 3.194002131880000039, 1466.133465350190136, 198.9725194175989884 ) ) ;
#62947=ORIENTED_EDGE ( 'NONE', *, *, #7744, .F. ) ;
#62952=CARTESIAN_POINT ( 'NONE',  ( 6.768931359969999839, 1468.810414808390078, 208.2491176551630190 ) ) ;
#62953=CARTESIAN_POINT ( 'NONE',  ( -9.115524708650340813, 1437.332156617270130, 212.8456964132400060 ) ) ;
#62956=CARTESIAN_POINT ( 'NONE',  ( 21.04904418909999819, 1494.916427559390058, 209.1218459616989946 ) ) ;
#62957=CARTESIAN_POINT ( 'NONE',  ( -2.302358205750000053, 1507.635233240290063, 221.1829251670990004 ) ) ;
#62959=CARTESIAN_POINT ( 'NONE',  ( 8.062587302181759341, 1436.235894220949831, 206.1282943059349861 ) ) ;
#62965=CARTESIAN_POINT ( 'NONE',  ( 4.325403553846939531, 1515.219291385629958, 211.4517448047639903 ) ) ;
#62972=CARTESIAN_POINT ( 'NONE',  ( -14.56647635000000029, 1415.677402202029953, 205.6923038026590120 ) ) ;
#62978=CARTESIAN_POINT ( 'NONE',  ( -8.557209110492459914, 1448.617779613390212, 212.3361752075699940 ) ) ;
#62980=B_SPLINE_CURVE_WITH_KNOTS ( 'NONE', 5,
 ( #71385, #97643, #56188, #72458, #39384, #4683 ),
 .UNSPECIFIED., .F., .F.,
 ( 6, 6 ),
 ( 0.000000000000000000, 1.000000000000000000 ),
 .UNSPECIFIED. ) ;
#62984=CARTESIAN_POINT ( 'NONE',  ( -0.7508624519220009619, 1515.469918561789882, 213.3394464563290001 ) ) ;
#62993=CARTESIAN_POINT ( 'NONE',  ( -0.2087337655829990257, 1432.232251408790034, 200.6786074516889755 ) ) ;
#62995=CARTESIAN_POINT ( 'NONE',  ( 3.035243144599999887, 1506.705827820389914, 220.5430297552989884 ) ) ;
#63004=CARTESIAN_POINT ( 'NONE',  ( 7.868158389089999538, 1422.937290482379922, 214.1570520181389838 ) ) ;
#63008=CARTESIAN_POINT ( 'NONE',  ( 18.72979941119999836, 1454.437773883689943, 204.5413093961989830 ) ) ;
#63016=CARTESIAN_POINT ( 'NONE',  ( -11.37293999165238567, 1501.433396541875936, 207.8219951246407504 ) ) ;
#63017=CARTESIAN_POINT ( 'NONE',  ( -15.69712680692647666, 1415.932051713374676, 208.5727945051003189 ) ) ;
#63025=CARTESIAN_POINT ( 'NONE',  ( 7.892794852110000647, 1424.253103618490059, 211.9974886484589831 ) ) ;
#63026=CARTESIAN_POINT ( 'NONE',  ( -5.221955787189999754, 1489.269541098190075, 185.8916489435990229 ) ) ;
#63042=CARTESIAN_POINT ( 'NONE',  ( -1.842963721827329815, 1515.551704300040001, 205.2922259627210053 ) ) ;
#63051=ORIENTED_EDGE ( 'NONE', *, *, #38611, .T. ) ;
#63060=EDGE_CURVE ( 'NONE', #53857, #86947, #49177, .T. ) ;
#63062=EDGE_CURVE ( 'NONE', #106884, #15989, #40126, .T. ) ;
#63065=CARTESIAN_POINT ( 'NONE',  ( -12.22580320763990080, 1490.195274737109912, 209.7895498202320255 ) ) ;
#63066=ADVANCED_FACE ( 'NONE', ( #49388 ), #16140, .F. ) ;
#63081=CARTESIAN_POINT ( 'NONE',  ( 12.14778619052680142, 1426.452938115369989, 195.7521405516270079 ) ) ;
#63084=ORIENTED_EDGE ( 'NONE', *, *, #83590, .F. ) ;
#63089=VERTEX_POINT ( 'NONE', #33116 ) ;
#63091=CARTESIAN_POINT ( 'NONE',  ( -3.118868704080000054, 1430.676437493689946, 201.3658569193489996 ) ) ;
#63092=EDGE_CURVE ( 'NONE', #75688, #45421, #90893, .T. ) ;
#63100=CARTESIAN_POINT ( 'NONE',  ( -3.617573937782270210, 1497.333809982809953, 198.4503636364750037 ) ) ;
#63101=CARTESIAN_POINT ( 'NONE',  ( 9.939099051061740298, 1468.642790207840108, 207.8814491574680119 ) ) ;
#63105=ORIENTED_EDGE ( 'NONE', *, *, #65149, .T. ) ;
#63109=CARTESIAN_POINT ( 'NONE',  ( 2.438924525309999591, 1442.537362853589912, 217.7859099704189987 ) ) ;
#63121=CARTESIAN_POINT ( 'NONE',  ( -14.24647739600000129, 1508.551704408389924, 215.7238636938289744 ) ) ;
#63122=CARTESIAN_POINT ( 'NONE',  ( 3.829620113550000315, 1515.551704408389924, 210.9648081929590262 ) ) ;
#63129=CARTESIAN_POINT ( 'NONE',  ( 5.551017880412060457, 1493.954195658629942, 218.9115059150300056 ) ) ;
#63130=CARTESIAN_POINT ( 'NONE',  ( -9.512413405997190097, 1489.190735525819946, 215.4037021917559969 ) ) ;
#63132=CARTESIAN_POINT ( 'NONE',  ( 13.84583145400000070, 1499.900106662689723, 227.7510597354990125 ) ) ;
#63140=ORIENTED_EDGE ( 'NONE', *, *, #50004, .F. ) ;
#63149=EDGE_CURVE ( 'NONE', #15989, #100706, #38085, .T. ) ;
#63152=CARTESIAN_POINT ( 'NONE',  ( -9.318458176530000969, 1446.292171852890078, 213.7041144372790313 ) ) ;
#63153=EDGE_CURVE ( 'NONE', #38120, #86906, #98826, .T. ) ;
#63155=CARTESIAN_POINT ( 'NONE',  ( 0.5721718498293950628, 1515.139735159980091, 213.4493323049200058 ) ) ;
#63157=CARTESIAN_POINT ( 'NONE',  ( -4.856098619647529979, 1477.048158301180138, 219.5765844122289820 ) ) ;
#63159=CARTESIAN_POINT ( 'NONE',  ( 20.12874795999999833, 1473.837606016890049, 209.1218459616989946 ) ) ;
#63163=CARTESIAN_POINT ( 'NONE',  ( 16.52383693655309926, 1494.278885720349990, 193.0549977294350299 ) ) ;
#63165=DIRECTION ( 'NONE',  ( -1.156023075842281927E-31, 1.000000000000000000, -1.698192320643030073E-16 ) ) ;
#63171=CARTESIAN_POINT ( 'NONE',  ( -9.077703255249998548, 1460.186802329990087, 213.0212026448490121 ) ) ;
#63174=ORIENTED_EDGE ( 'NONE', *, *, #25483, .T. ) ;
#63179=LINE ( 'NONE', #36833, #51573 ) ;
#63181=CARTESIAN_POINT ( 'NONE',  ( -0.4989641633528249520, 1496.333062096209915, 221.4618052869690246 ) ) ;
#63188=CARTESIAN_POINT ( 'NONE',  ( 6.554685473990000233, 1473.611172115990030, 218.5142022801589974 ) ) ;
#63189=CARTESIAN_POINT ( 'NONE',  ( -8.567500621095319957, 1439.360189638610109, 206.7715929992849908 ) ) ;
#63196=ORIENTED_EDGE ( 'NONE', *, *, #101923, .F. ) ;
#63199=CARTESIAN_POINT ( 'NONE',  ( -1.841039239253470017, 1467.896901348140091, 220.0920151498449968 ) ) ;
#63204=CARTESIAN_POINT ( 'NONE',  ( 7.333575610579999626, 1455.004670275590115, 216.8632114976190053 ) ) ;
#63221=CARTESIAN_POINT ( 'NONE',  ( 11.23851827549999882, 1490.487975447490044, 204.0492753133389954 ) ) ;
#63229=CARTESIAN_POINT ( 'NONE',  ( -19.23853081770000273, 1466.576780668189940, 213.8528554934590034 ) ) ;
#63233=CARTESIAN_POINT ( 'NONE',  ( -20.94952978810714228, 1507.788843330700047, 209.4873209303592887 ) ) ;
#63242=CARTESIAN_POINT ( 'NONE',  ( 12.17090612297010033, 1499.730349834240087, 205.6507082230390040 ) ) ;
#63245=CARTESIAN_POINT ( 'NONE',  ( -2.487935123020000194, 1508.551704408389924, 214.1089243778970115 ) ) ;
#63248=CARTESIAN_POINT ( 'NONE',  ( -4.869818399669999742, 1491.215867106689984, 188.8099941780989752 ) ) ;
#63252=CARTESIAN_POINT ( 'NONE',  ( -21.51339055684400137, 1505.551704076410033, 209.1218459052249727 ) ) ;
#63254=CARTESIAN_POINT ( 'NONE',  ( -14.60558113189999929, 1415.677402202029953, 212.8314178170890045 ) ) ;
#63263=CARTESIAN_POINT ( 'NONE',  ( 20.33642002845060048, 1475.138300237510066, 218.0161321312470193 ) ) ;
#63268=CARTESIAN_POINT ( 'NONE',  ( 10.99882366966150116, 1470.803487868729917, 192.2106042945659965 ) ) ;
#63269=ADVANCED_FACE ( 'NONE', ( #21800, #99621 ), #48710, .F. ) ;
#63270=CARTESIAN_POINT ( 'NONE',  ( 1.124946299140000106, 1430.908435126590120, 217.7868728150889979 ) ) ;
#63277=CARTESIAN_POINT ( 'NONE',  ( 11.86864015205539857, 1492.043074283439864, 209.5973308918830185 ) ) ;
#63282=CARTESIAN_POINT ( 'NONE',  ( -1.132178478439539893, 1496.267470226739988, 196.8234858163660022 ) ) ;
#63286=CARTESIAN_POINT ( 'NONE',  ( -14.35646903299999799, 1420.584115152450067, 213.7701001417389932 ) ) ;
#63293=CARTESIAN_POINT ( 'NONE',  ( -3.558358604862239982, 1455.955982659530036, 200.3550966546550001 ) ) ;
#63295=CARTESIAN_POINT ( 'NONE',  ( 1.608613766090000174, 1497.503754473789968, 197.5580351143990185 ) ) ;
#63296=CARTESIAN_POINT ( 'NONE',  ( -19.57991515103069702, 1487.974510678529896, 201.8977438688889947 ) ) ;
#63305=CARTESIAN_POINT ( 'NONE',  ( 1.951646715579999913, 1485.466892314489996, 220.4400105658989730 ) ) ;
#63307=CARTESIAN_POINT ( 'NONE',  ( 12.89506042661790097, 1420.989630775050045, 203.4267427568519793 ) ) ;
#63313=DIRECTION ( 'NONE',  ( -1.156023075842281927E-31, 1.000000000000000000, -1.698192320643030073E-16 ) ) ;
#63316=CARTESIAN_POINT ( 'NONE',  ( 9.160265459600150706, 1451.053466593440135, 210.4056783562319879 ) ) ;
#63317=CARTESIAN_POINT ( 'NONE',  ( 7.326528841800000080, 1424.652172197859954, 194.6120463040990103 ) ) ;
#63321=CARTESIAN_POINT ( 'NONE',  ( -5.865854492251394880, 1419.522645696713653, 194.8824993499091534 ) ) ;
#63322=CARTESIAN_POINT ( 'NONE',  ( 19.17592663279999954, 1455.939271352290007, 211.9382291609089748 ) ) ;
#63326=EDGE_LOOP ( 'NONE', ( #90404, #10566, #9016, #5305 ) ) ;
#63332=ORIENTED_EDGE ( 'NONE', *, *, #57405, .F. ) ;
#63338=CARTESIAN_POINT ( 'NONE',  ( -2.157742269045689998, 1508.491635936170042, 220.5016648786540259 ) ) ;
#63340=CARTESIAN_POINT ( 'NONE',  ( -3.476578636579250148, 1469.245868782419848, 218.7387964245460239 ) ) ;
#63342=CARTESIAN_POINT ( 'NONE',  ( 9.209290677350001175, 1421.000200739789989, 196.8939171836989885 ) ) ;
#63347=AXIS2_PLACEMENT_3D ( 'NONE', #13820, #32302, #83802 ) ;
#63349=CARTESIAN_POINT ( 'NONE',  ( -14.19821127820000051, 1503.588220803689865, 208.7291843775310269 ) ) ;
#63352=CARTESIAN_POINT ( 'NONE',  ( -9.740768063862729420, 1440.142023887889991, 206.7831334340250180 ) ) ;
#63353=ADVANCED_FACE ( 'NONE', ( #73905 ), #93051, .T. ) ;
#63362=CARTESIAN_POINT ( 'NONE',  ( 4.158039145940000125, 1505.593071592290016, 220.7718859801990163 ) ) ;
#63363=EDGE_CURVE ( 'NONE', #34173, #52522, #99071, .T. ) ;
#63366=ORIENTED_EDGE ( 'NONE', *, *, #98653, .T. ) ;
#63367=CARTESIAN_POINT ( 'NONE',  ( -15.73068931088838340, 1415.766719735401921, 209.6787192454432329 ) ) ;
#63371=CARTESIAN_POINT ( 'NONE',  ( 0.4304708442563399684, 1430.546724899550100, 199.7002147614190051 ) ) ;
#63375=CARTESIAN_POINT ( 'NONE',  ( 8.185246060965688741, 1459.507010914890088, 203.1833342143360142 ) ) ;
#63378=CARTESIAN_POINT ( 'NONE',  ( -4.526773330479999302, 1476.791184819089949, 219.3260595622990081 ) ) ;
#63388=CARTESIAN_POINT ( 'NONE',  ( 12.64521106209990009, 1426.920070115170120, 205.6194074905729963 ) ) ;
#63392=CARTESIAN_POINT ( 'NONE',  ( 8.454790733525280544, 1428.363638633589972, 213.4109935021670026 ) ) ;
#63393=CARTESIAN_POINT ( 'NONE',  ( -4.325405441710000076, 1515.219201591190085, 207.2788837304390199 ) ) ;
#63398=EDGE_LOOP ( 'NONE', ( #78017, #9599, #51340, #66300 ) ) ;
#63402=CARTESIAN_POINT ( 'NONE',  ( 4.229167303610000594, 1436.983388288790138, 227.1518914930990150 ) ) ;
#63403=B_SPLINE_CURVE_WITH_KNOTS ( 'NONE', 5,
 ( #47373, #97211, #98863, #56880, #80426, #107267, #91010, #21590, #39521 ),
 .UNSPECIFIED., .F., .F.,
 ( 6, 3, 6 ),
 ( 0.000000000000000000, 0.5002376165324764479, 1.000000000000000000 ),
 .UNSPECIFIED. ) ;
#63411=CARTESIAN_POINT ( 'NONE',  ( -8.392515761190244561, 1423.425497820198871, 210.5964995326183384 ) ) ;
#63421=CARTESIAN_POINT ( 'NONE',  ( -1.506941832969999950, 1422.391778822009883, 192.9691301536989840 ) ) ;
#63424=CARTESIAN_POINT ( 'NONE',  ( -18.58572048804549937, 1467.426106157030063, 201.0022324237500015 ) ) ;
#63428=CARTESIAN_POINT ( 'NONE',  ( -5.188149647699999534, 1391.908650341390057, 203.7646307972290174 ) ) ;
#63431=DIRECTION ( 'NONE',  ( -0.9097196265265821147, 0.3041674008372309834, 0.2826524250387019710 ) ) ;
#63437=CARTESIAN_POINT ( 'NONE',  ( -8.477967594009999885, 1424.852341466620146, 205.3179503978689979 ) ) ;
#63439=AXIS2_PLACEMENT_3D ( 'NONE', #109396, #108826, #15835 ) ;
#63442=VERTEX_POINT ( 'NONE', #47594 ) ;
#63445=CARTESIAN_POINT ( 'NONE',  ( -0.4829651199533262496, 1457.465871680693226, 199.6046590496274575 ) ) ;
#63459=CARTESIAN_POINT ( 'NONE',  ( 20.33509144374850308, 1432.834507525260051, 214.7556780039420232 ) ) ;
#63460=CARTESIAN_POINT ( 'NONE',  ( 9.334683862901423268, 1491.782840251982861, 215.1527950542473491 ) ) ;
#63461=EDGE_LOOP ( 'NONE', ( #50758, #18314 ) ) ;
#63468=CARTESIAN_POINT ( 'NONE',  ( 10.05341040150000076, 1462.281908926990127, 210.6545760798489937 ) ) ;
#63469=AXIS2_PLACEMENT_3D ( 'NONE', #4190, #38323, #45110 ) ;
#63472=CARTESIAN_POINT ( 'NONE',  ( -1.720902727859999981, 1464.150605286389919, 199.3240545488989710 ) ) ;
#63484=CARTESIAN_POINT ( 'NONE',  ( -8.799999999999998934, 1413.913060387329779, 209.1218459616989946 ) ) ;
#63486=CARTESIAN_POINT ( 'NONE',  ( -17.34960988009670757, 1508.455927730609119, 212.8242482004856413 ) ) ;
#63488=CARTESIAN_POINT ( 'NONE',  ( -6.437876012944840021, 1435.112046181850019, 216.3672298223000041 ) ) ;
#63492=CARTESIAN_POINT ( 'NONE',  ( -5.797231311010000887, 1507.943299984489840, 220.7428112414989982 ) ) ;
#63498=CARTESIAN_POINT ( 'NONE',  ( 0.1666560433379990214, 1469.576466606489930, 216.4329724472190151 ) ) ;
#63510=CARTESIAN_POINT ( 'NONE',  ( 9.304705586386592842, 1483.500584759331105, 214.3952978072885003 ) ) ;
#63511=CARTESIAN_POINT ( 'NONE',  ( -15.43898598230000019, 1415.677402227490120, 208.9970960677119933 ) ) ;
#63515=B_SPLINE_CURVE_WITH_KNOTS ( 'NONE', 3,
 ( #59944, #26871, #1137, #103004, #86217, #26301, #53191, #77287, #1688, #34163, #93503, #102455, #52637, #61061, #7852, #60491, #76169, #94612, #67785 ),
 .UNSPECIFIED., .F., .F.,
 ( 4, 2, 2, 2, 1, 1, 1, 2, 2, 2, 4 ),
 ( 0.000000000000000000, 0.2500000000002982059, 0.3750000000004471978, 0.4375000000005346834, 0.4687500000005783707, 0.4843750000006000755, 0.4921875000006109002, 0.4960937500005973555, 0.5000000000005837553, 0.7500000000002919887, 1.000000000000000000 ),
 .UNSPECIFIED. ) ;
#63518=CARTESIAN_POINT ( 'NONE',  ( -9.009356499370060334, 1449.261709350619867, 210.8259634658180062 ) ) ;
#63524=CARTESIAN_POINT ( 'NONE',  ( -0.008608266642480520009, 1515.483924129489878, 213.3566978088589963 ) ) ;
#63531=CARTESIAN_POINT ( 'NONE',  ( 0.2719187923920010075, 1432.443060607389953, 200.6707351473390020 ) ) ;
#63534=DIRECTION ( 'NONE',  ( -9.462326934583649054E-47, 1.000000000000000000, -1.836970198721029688E-16 ) ) ;
#63537=CARTESIAN_POINT ( 'NONE',  ( 9.190374286110708724, 1468.398850889019968, 204.6732001591689993 ) ) ;
#63543=CARTESIAN_POINT ( 'NONE',  ( 12.06005565936200163, 1491.389938827579954, 206.7797953803130326 ) ) ;
#63554=CARTESIAN_POINT ( 'NONE',  ( 3.829620113920000346, 1515.551704408389924, 211.4519800804890224 ) ) ;
#63560=CARTESIAN_POINT ( 'NONE',  ( 7.996683413600000456, 1427.037929587379949, 212.0417767193789871 ) ) ;
#63567=ORIENTED_EDGE ( 'NONE', *, *, #107486, .F. ) ;
#63568=EDGE_LOOP ( 'NONE', ( #63105, #65021, #16176, #71336 ) ) ;
#63572=CARTESIAN_POINT ( 'NONE',  ( 3.738304505813290657, 1499.328994237659117, 198.3873084196136745 ) ) ;
#63574=CARTESIAN_POINT ( 'NONE',  ( -21.53299174964140050, 1506.014650851819852, 209.2005993430840078 ) ) ;
#63575=B_SPLINE_CURVE_WITH_KNOTS ( 'NONE', 5,
 ( #19440, #104004, #45233, #27301, #2688, #61482 ),
 .UNSPECIFIED., .F., .F.,
 ( 6, 6 ),
 ( -1.999999943015589920, 0.000000000000000000 ),
 .UNSPECIFIED. ) ;
#63584=EDGE_LOOP ( 'NONE', ( #16493, #88987, #83629, #20432 ) ) ;
#63588=ORIENTED_EDGE ( 'NONE', *, *, #56884, .T. ) ;
#63597=AXIS2_PLACEMENT_3D ( 'NONE', #2785, #88420, #64336 ) ;
#63600=CARTESIAN_POINT ( 'NONE',  ( -12.09982269103889863, 1489.891875091150041, 210.9072642413369749 ) ) ;
#63606=ORIENTED_EDGE ( 'NONE', *, *, #24097, .T. ) ;
#63608=DIRECTION ( 'NONE',  ( -0.8796244824232881676, -0.3860830610750210501, -0.2778500312623770063 ) ) ;
#63610=CARTESIAN_POINT ( 'NONE',  ( 19.55988977460000200, 1474.636381753090063, 214.0184790771390055 ) ) ;
#63617=CARTESIAN_POINT ( 'NONE',  ( 10.93200248603220004, 1426.108105161469894, 194.7599858398060064 ) ) ;
#63629=( BOUNDED_CURVE ( )  B_SPLINE_CURVE ( 3, ( #66181, #100301, #84592, #57776 ),
 .UNSPECIFIED., .F., .T. ) 
 B_SPLINE_CURVE_WITH_KNOTS ( ( 4, 4 ),
 ( 4.146398541727710274, 5.278376838302800245 ),
 .UNSPECIFIED. ) 
 CURVE ( )  GEOMETRIC_REPRESENTATION_ITEM ( )  RATIONAL_B_SPLINE_CURVE ( ( 1.000000000000000000, 0.8960390544622802711, 0.8960390544622802711, 1.000000000000000000 ) ) 
 REPRESENTATION_ITEM ( '' )  );
#63630=CARTESIAN_POINT ( 'NONE',  ( 4.487249775049700240, 1509.038615934839981, 206.6339108193819811 ) ) ;
#63632=CARTESIAN_POINT ( 'NONE',  ( 12.73217514220000091, 1421.428024357469894, 206.3441494772290241 ) ) ;
#63635=CARTESIAN_POINT ( 'NONE',  ( -16.39908139913352869, 1416.805070253819395, 208.0671872555761297 ) ) ;
#63637=CARTESIAN_POINT ( 'NONE',  ( 11.40429614103280187, 1470.873877624120041, 208.7845352330780315 ) ) ;
#63638=VERTEX_POINT ( 'NONE', #96774 ) ;
#63641=ORIENTED_EDGE ( 'NONE', *, *, #39061, .F. ) ;
#63643=CARTESIAN_POINT ( 'NONE',  ( 4.541133980909999757, 1426.446980476709996, 211.3175313701290179 ) ) ;
#63644=CARTESIAN_POINT ( 'NONE',  ( 8.133961203403233142, 1424.059811672474325, 195.8560981452540659 ) ) ;
#63645=CARTESIAN_POINT ( 'NONE',  ( 2.659511198940000209, 1441.714673586189974, 218.2865353327090077 ) ) ;
#63654=CARTESIAN_POINT ( 'NONE',  ( -10.15398179789089994, 1472.533710365230036, 209.9201027492950118 ) ) ;
#63658=CARTESIAN_POINT ( 'NONE',  ( 11.29267550753220029, 1470.546782610659875, 207.7331957881270057 ) ) ;
#63663=CYLINDRICAL_SURFACE ( 'NONE', #77075, 0.4999999999999449329 ) ;
#63664=CARTESIAN_POINT ( 'NONE',  ( 4.709068530708940159, 1495.147136111799909, 220.5787748165419941 ) ) ;
#63665=CARTESIAN_POINT ( 'NONE',  ( 22.24401329409999661, 1475.958617299990010, 209.7631870919539949 ) ) ;
#63666=CARTESIAN_POINT ( 'NONE',  ( -15.29087862775659978, 1415.677402202089979, 208.7697798501069997 ) ) ;
#63668=AXIS2_PLACEMENT_3D ( 'NONE', #39963, #56221, #23147 ) ;
#63669=EDGE_CURVE ( 'NONE', #21613, #104968, #44107, .T. ) ;
#63671=CARTESIAN_POINT ( 'NONE',  ( 3.959152859930000101, 1428.396642669490120, 216.3690266601789745 ) ) ;
#63672=CARTESIAN_POINT ( 'NONE',  ( 13.55421397129999939, 1497.816254223590022, 226.3870761728989862 ) ) ;
#63688=CARTESIAN_POINT ( 'NONE',  ( -3.026951662149999667, 1443.662240191790033, 218.7413276925990147 ) ) ;
#63690=CARTESIAN_POINT ( 'NONE',  ( -0.3770322115495070014, 1515.150283736280016, 213.4490560809049953 ) ) ;
#63697=ORIENTED_EDGE ( 'NONE', *, *, #38800, .F. ) ;
#63698=CARTESIAN_POINT ( 'NONE',  ( -11.48363738179999949, 1505.551007100490096, 207.2975035741290242 ) ) ;
#63700=CARTESIAN_POINT ( 'NONE',  ( -22.17858213466869799, 1484.390483148310068, 216.9702515509989951 ) ) ;
#63724=DIRECTION ( 'NONE',  ( 1.000000000000000000, 0.000000000000000000, 0.000000000000000000 ) ) ;
#63726=EDGE_LOOP ( 'NONE', ( #71365, #11397, #29482, #8884 ) ) ;
#63729=CARTESIAN_POINT ( 'NONE',  ( 9.281345480445999385, 1435.168664884130294, 207.8114304728740080 ) ) ;
#63732=EDGE_LOOP ( 'NONE', ( #105009, #58380, #92152, #99029 ) ) ;
#63734=CARTESIAN_POINT ( 'NONE',  ( 11.18756042069709977, 1471.604168298739978, 211.4504785696180136 ) ) ;
#63744=CARTESIAN_POINT ( 'NONE',  ( -7.703846517336140565, 1425.539117803745512, 205.4402351432403862 ) ) ;
#63746=VERTEX_POINT ( 'NONE', #4369 ) ;
#63749=CARTESIAN_POINT ( 'NONE',  ( -3.913149750709999708, 1414.000033450179899, 206.8545747367489867 ) ) ;
#63763=TOROIDAL_SURFACE ( 'NONE', #90508, 14.91144628110000170, 0.5000000000000000000 ) ;
#63764=DIRECTION ( 'NONE',  ( 9.341989762165448955E-47, -1.000000000000000000, 1.836970198721029688E-16 ) ) ;
#63786=CARTESIAN_POINT ( 'NONE',  ( -21.44637798829759845, 1506.412603150730092, 216.0243673054189912 ) ) ;
#63795=CARTESIAN_POINT ( 'NONE',  ( 3.856607047088039586, 1508.551704408389924, 204.5415913389130083 ) ) ;
#63798=CARTESIAN_POINT ( 'NONE',  ( -9.838242193716929762, 1462.268756451870104, 227.9668037484569822 ) ) ;
#63804=CARTESIAN_POINT ( 'NONE',  ( -2.031883580139580037, 1464.998375551469962, 198.3053770173009980 ) ) ;
#63806=CARTESIAN_POINT ( 'NONE',  ( 4.086314366965700273, 1515.499673594937576, 211.4519800836456795 ) ) ;
#63822=CARTESIAN_POINT ( 'NONE',  ( -0.1106396160836400078, 1496.533495305330007, 196.7588328172749925 ) ) ;
#63827=ADVANCED_FACE ( 'NONE', ( #87562 ), #89388, .T. ) ;
#63839=CARTESIAN_POINT ( 'NONE',  ( -11.20337388083980201, 1490.156468557539938, 191.3256793942369995 ) ) ;
#63846=CYLINDRICAL_SURFACE ( 'NONE', #49809, 0.4999999999999909517 ) ;
#63848=CARTESIAN_POINT ( 'NONE',  ( 0.1259222685549989951, 1487.739371776789994, 219.9965893379989836 ) ) ;
#63858=VERTEX_POINT ( 'NONE', #99226 ) ;
#63861=CARTESIAN_POINT ( 'NONE',  ( 7.703785732380000084, 1490.746146274789908, 209.8379679705590206 ) ) ;
#63864=CARTESIAN_POINT ( 'NONE',  ( 9.146299198640271300, 1461.861878385089767, 205.8341600298289791 ) ) ;
#63872=CARTESIAN_POINT ( 'NONE',  ( 7.816109785343320127, 1482.901617154930136, 217.9966951879339945 ) ) ;
#63877=CARTESIAN_POINT ( 'NONE',  ( -3.186928814199029958, 1508.501190230369957, 220.3905975803280057 ) ) ;
#63880=CARTESIAN_POINT ( 'NONE',  ( -9.262945410020661186, 1470.779016715980106, 213.5645637807399737 ) ) ;
#63882=CARTESIAN_POINT ( 'NONE',  ( 9.549927530160001510, 1420.582634806009992, 197.0246874367990131 ) ) ;
#63883=CARTESIAN_POINT ( 'NONE',  ( -0.2259745478316219913, 1475.391039426699990, 220.5480955931240032 ) ) ;
#63884=CARTESIAN_POINT ( 'NONE',  ( -6.883305316117739991, 1494.320249002219953, 198.9132838350930115 ) ) ;
#63889=CARTESIAN_POINT ( 'NONE',  ( 11.48916758364780044, 1422.248195443439954, 207.1589471795049917 ) ) ;
#63898=CARTESIAN_POINT ( 'NONE',  ( 4.706367361569999908, 1507.026273860589981, 219.8285751887989932 ) ) ;
#63900=CARTESIAN_POINT ( 'NONE',  ( -16.44718840435429996, 1420.035791990140069, 209.2215304830220077 ) ) ;
#63902=CARTESIAN_POINT ( 'NONE',  ( -17.01997119704033423, 1417.322295037478625, 207.6226155442043648 ) ) ;
#63904=ADVANCED_FACE ( 'NONE', ( #14685 ), #101070, .T. ) ;
#63906=CARTESIAN_POINT ( 'NONE',  ( -0.7759192619701910099, 1430.041485328890076, 199.7504914271860059 ) ) ;
#63909=EDGE_CURVE ( 'NONE', #39082, #25053, #97434, .T. ) ;
#63910=CARTESIAN_POINT ( 'NONE',  ( 1.269517173649849839, 1457.689354814089938, 199.6687979431409872 ) ) ;
#63922=CARTESIAN_POINT ( 'NONE',  ( -14.23398643054899892, 1416.596405885110016, 203.1904536488209772 ) ) ;
#63928=B_SPLINE_CURVE_WITH_KNOTS ( 'NONE', 5,
 ( #73681, #106695, #91563, #107808, #31095, #5348 ),
 .UNSPECIFIED., .F., .F.,
 ( 6, 6 ),
 ( 203.1089678689999971, 212.7664182919999973 ),
 .UNSPECIFIED. ) ;
#63929=CARTESIAN_POINT ( 'NONE',  ( -4.091836660730000297, 1515.531866980889845, 208.0024180612289797 ) ) ;
#63938=CARTESIAN_POINT ( 'NONE',  ( -12.25495820260000102, 1490.496248278489702, 208.7368242965009983 ) ) ;
#63939=B_SPLINE_CURVE_WITH_KNOTS ( 'NONE', 5,
 ( #18878, #45234, #37366, #44677, #35700, #62040, #69890, #53077, #97258 ),
 .UNSPECIFIED., .F., .F.,
 ( 6, 3, 6 ),
 ( 0.000000000000000000, 3.343413285960000092, 6.686826571920000184 ),
 .UNSPECIFIED. ) ;
#63940=CARTESIAN_POINT ( 'NONE',  ( 3.235048515759559873, 1466.472015849239824, 219.6884157167970102 ) ) ;
#63950=DIRECTION ( 'NONE',  ( 0.2958906675619759619, 0.3688552201855968549, 0.8811325322512856273 ) ) ;
#63953=ADVANCED_FACE ( 'NONE', ( #103084 ), #84102, .T. ) ;
#63955=CARTESIAN_POINT ( 'NONE',  ( -5.144873395449999443, 1502.885538352589947, 229.8910404859989853 ) ) ;
#63963=CARTESIAN_POINT ( 'NONE',  ( 7.201922804036379411, 1423.097602058059920, 196.0540625376380035 ) ) ;
#63964=CARTESIAN_POINT ( 'NONE',  ( -19.81119127480000230, 1468.787329907190042, 204.4917199178690055 ) ) ;
#63970=CARTESIAN_POINT ( 'NONE',  ( -234.5897387251999930, 11221.53578756869865, 2175.945776423289772 ) ) ;
#63979=CARTESIAN_POINT ( 'NONE',  ( 11.36217411025890023, 1503.110300770179720, 211.0233484295470134 ) ) ;
#63987=CARTESIAN_POINT ( 'NONE',  ( 0.5863727358502109910, 1485.693194848699932, 220.9873588030069982 ) ) ;
#63995=CARTESIAN_POINT ( 'NONE',  ( 10.25705989742519897, 1481.638279496849918, 212.3655552129939963 ) ) ;
#63998=CARTESIAN_POINT ( 'NONE',  ( -7.260870878720000476, 1480.575647549590030, 208.3277293783959863 ) ) ;
#64000=CARTESIAN_POINT ( 'NONE',  ( -9.573049153892020158, 1423.428015373189965, 192.3355766873849859 ) ) ;
#64001=DIRECTION ( 'NONE',  ( 1.000000000000000000, 2.249639673992764790E-32, 1.224646799147350002E-16 ) ) ;
#64003=ORIENTED_EDGE ( 'NONE', *, *, #105176, .T. ) ;
#64004=ORIENTED_EDGE ( 'NONE', *, *, #83012, .T. ) ;
#64012=CARTESIAN_POINT ( 'NONE',  ( 0.06822080563540121323, 1464.084053037690182, 199.2812091259889939 ) ) ;
#64026=CARTESIAN_POINT ( 'NONE',  ( -5.855016933008430513, 1434.745513377389898, 216.8132225448020165 ) ) ;
#64039=CARTESIAN_POINT ( 'NONE',  ( -11.41675697748640061, 1482.775670443970057, 205.7339590229720159 ) ) ;
#64041=CARTESIAN_POINT ( 'NONE',  ( -4.124984636820000716, 1429.048548944989989, 205.3222558022289945 ) ) ;
#64046=CARTESIAN_POINT ( 'NONE',  ( -15.53640578200000100, 1415.765361658500069, 208.3984121209330169 ) ) ;
#64061=CARTESIAN_POINT ( 'NONE',  ( 1.166977143170000009, 1471.376848498290201, 188.9924741841990112 ) ) ;
#64062=CARTESIAN_POINT ( 'NONE',  ( 21.13483499240000185, 1496.881468811689956, 208.7396410216740037 ) ) ;
#64063=EDGE_CURVE ( 'NONE', #5861, #18354, #49034, .T. ) ;
#64067=EDGE_CURVE ( 'NONE', #58087, #75158, #49253, .T. ) ;
#64069=CARTESIAN_POINT ( 'NONE',  ( -1.839380708780000040, 1507.096886517889970, 221.8368464039990045 ) ) ;
#64075=FACE_OUTER_BOUND ( 'NONE', #39889, .T. ) ;
#64081=EDGE_CURVE ( 'NONE', #11098, #15049, #54631, .T. ) ;
#64089=CARTESIAN_POINT ( 'NONE',  ( -6.668618179459999240, 1472.084049029690050, 211.0614949439089969 ) ) ;
#64095=CARTESIAN_POINT ( 'NONE',  ( -9.586136107779999804, 1449.725920977289888, 206.0133221225389946 ) ) ;
#64098=CARTESIAN_POINT ( 'NONE',  ( 8.220300753029999186, 1427.204169894219831, 212.0038158565590152 ) ) ;
#64101=DIRECTION ( 'NONE',  ( 0.8794237532950536229, -0.3862684439859148666, 0.2782275171889739274 ) ) ;
#64106=ORIENTED_EDGE ( 'NONE', *, *, #11821, .T. ) ;
#64118=CARTESIAN_POINT ( 'NONE',  ( -2.400179225536239969, 1464.934988852220158, 198.3730454101489897 ) ) ;
#64125=EDGE_LOOP ( 'NONE', ( #91793, #43031, #48242, #16159, #104162 ) ) ;
#64137=AXIS2_PLACEMENT_3D ( 'NONE', #98485, #106882, #91741 ) ;
#64147=CARTESIAN_POINT ( 'NONE',  ( -12.06562581462340056, 1489.842093712740052, 211.0982364962250131 ) ) ;
#64151=ORIENTED_EDGE ( 'NONE', *, *, #13319, .F. ) ;
#64155=CARTESIAN_POINT ( 'NONE',  ( 9.600864221749999317, 1470.542902921190034, 212.2537306481789869 ) ) ;
#64162=CARTESIAN_POINT ( 'NONE',  ( 9.633401174267049782, 1425.762329347420291, 193.8812324694129927 ) ) ;
#64170=CARTESIAN_POINT ( 'NONE',  ( -2.873525832259999913, 1429.447207211989962, 200.9398776307089918 ) ) ;
#64174=CARTESIAN_POINT ( 'NONE',  ( 11.23217089400000113, 1422.349028627020061, 203.7645952894689856 ) ) ;
#64177=CARTESIAN_POINT ( 'NONE',  ( -3.558358604862239982, 1455.955982659530036, 200.3550966546550001 ) ) ;
#64179=CARTESIAN_POINT ( 'NONE',  ( 10.46907846689019905, 1470.153368976490128, 208.0239820498049994 ) ) ;
#64185=CARTESIAN_POINT ( 'NONE',  ( 17.90653978779999989, 1430.488564755489961, 212.6866031076790193 ) ) ;
#64186=CARTESIAN_POINT ( 'NONE',  ( 7.937878408760115079, 1423.739882246193247, 195.8491950690135468 ) ) ;
#64187=CARTESIAN_POINT ( 'NONE',  ( 2.390248854959999836, 1443.517510617689823, 217.7159995093989835 ) ) ;
#64191=CARTESIAN_POINT ( 'NONE',  ( 7.896860026827476453, 1487.333077441552632, 201.7073600637725690 ) ) ;
#64199=CARTESIAN_POINT ( 'NONE',  ( -9.487584436799998855, 1508.516108850790033, 218.8016808830589923 ) ) ;
#64201=CARTESIAN_POINT ( 'NONE',  ( 11.17215557887869970, 1470.323562617609923, 207.0621806280969963 ) ) ;
#64202=CARTESIAN_POINT ( 'NONE',  ( -4.205583201319999631, 1483.725063651190112, 199.3005808441589863 ) ) ;
#64208=CIRCLE ( 'NONE', #55330, 419.2957457743311807 ) ;
#64209=CARTESIAN_POINT ( 'NONE',  ( 24.04366906972200013, 1494.655619859800026, 207.1743914002310021 ) ) ;
#64210=CARTESIAN_POINT ( 'NONE',  ( -14.30833984952479909, 1415.677402203010161, 204.8799990442770138 ) ) ;
#64213=CARTESIAN_POINT ( 'NONE',  ( -9.658233005175830499, 1460.589625460329898, 208.7565551244479991 ) ) ;
#64214=CARTESIAN_POINT ( 'NONE',  ( 6.092650983240000429, 1427.361657835570213, 214.7380281929690113 ) ) ;
#64215=CARTESIAN_POINT ( 'NONE',  ( 4.511930455219999914, 1492.982136831589969, 216.2205869640490050 ) ) ;
#64216=VERTEX_POINT ( 'NONE', #71625 ) ;
#64234=CARTESIAN_POINT ( 'NONE',  ( 0.6915095762648889588, 1515.131927850350166, 213.4495367465950153 ) ) ;
#64236=CARTESIAN_POINT ( 'NONE',  ( -4.594317082651300232, 1476.940951215450013, 219.6856609997009855 ) ) ;
#64237=B_SPLINE_CURVE_WITH_KNOTS ( 'NONE', 5,
 ( #35434, #20274, #61231, #80200, #27044, #27585 ),
 .UNSPECIFIED., .F., .F.,
 ( 6, 6 ),
 ( 0.000000000000000000, 1.000000000000000000 ),
 .UNSPECIFIED. ) ;
#64244=CARTESIAN_POINT ( 'NONE',  ( 16.57070253540619831, 1493.685518685909983, 193.1449767612709820 ) ) ;
#64246=CARTESIAN_POINT ( 'NONE',  ( 11.61220494760000044, 1420.579219889470096, 199.3493800206389892 ) ) ;
#64251=CARTESIAN_POINT ( 'NONE',  ( 1.408274608409999740, 1457.262919913989890, 199.5821060027690237 ) ) ;
#64257=ORIENTED_EDGE ( 'NONE', *, *, #103603, .T. ) ;
#64262=FILL_AREA_STYLE ('',( #30072 ) ) ;
#64265=DIRECTION ( 'NONE',  ( 0.4794255386042031719, 0.000000000000000000, 0.8775825618903726477 ) ) ;
#64277=CARTESIAN_POINT ( 'NONE',  ( 8.559887967433979838, 1437.031052010680014, 207.9845883466809937 ) ) ;
#64280=ORIENTED_EDGE ( 'NONE', *, *, #44202, .T. ) ;
#64282=CARTESIAN_POINT ( 'NONE',  ( 11.03771696505579847, 1471.764929341090237, 212.0955496467459795 ) ) ;
#64293=ORIENTED_EDGE ( 'NONE', *, *, #53892, .T. ) ;
#64302=CARTESIAN_POINT ( 'NONE',  ( -8.838153826319999240, 1416.011808640619847, 204.9871024205990011 ) ) ;
#64306=CARTESIAN_POINT ( 'NONE',  ( 10.79356334649999916, 1490.085259999289974, 207.2636451086090119 ) ) ;
#64322=CARTESIAN_POINT ( 'NONE',  ( 1.608912855160989919, 1456.301673701370191, 198.6631191214040086 ) ) ;
#64325=CARTESIAN_POINT ( 'NONE',  ( -10.88819247137429969, 1470.683299348469973, 210.3143062069100040 ) ) ;
#64327=ORIENTED_EDGE ( 'NONE', *, *, #11184, .T. ) ;
#64334=CARTESIAN_POINT ( 'NONE',  ( 8.051697842710000330, 1428.206416439490113, 213.2401734540090104 ) ) ;
#64336=DIRECTION ( 'NONE',  ( 1.000000000000000000, 0.000000000000000000, 0.000000000000000000 ) ) ;
#64346=CARTESIAN_POINT ( 'NONE',  ( 3.626138226495970063, 1508.551704408389924, 204.4076455118720048 ) ) ;
#64349=CARTESIAN_POINT ( 'NONE',  ( 18.94655651209840030, 1455.761357035959918, 200.3458043486710380 ) ) ;
#64353=CARTESIAN_POINT ( 'NONE',  ( -9.519358626507830934, 1460.477013633640126, 210.7621351857700063 ) ) ;
#64355=CARTESIAN_POINT ( 'NONE',  ( 9.860940659611273418, 1504.635452453244170, 215.2684308639460937 ) ) ;
#64359=CARTESIAN_POINT ( 'NONE',  ( 4.449807483899999916, 1453.291438929989909, 213.9306864722589978 ) ) ;
#64361=CYLINDRICAL_SURFACE ( 'NONE', #98005, 7.799999999999999822 ) ;
#64372=CARTESIAN_POINT ( 'NONE',  ( -15.83970063559999808, 1420.111466363800218, 210.7068694924290071 ) ) ;
#64380=CARTESIAN_POINT ( 'NONE',  ( -9.004371644888150783, 1448.775058266490078, 210.7636302426640214 ) ) ;
#64387=CARTESIAN_POINT ( 'NONE',  ( -13.58041510073769942, 1508.551704408389924, 210.3416170870220014 ) ) ;
#64388=CARTESIAN_POINT ( 'NONE',  ( 7.063366770386080518, 1424.901426757719946, 213.0980514803050028 ) ) ;
#64396=CARTESIAN_POINT ( 'NONE',  ( 0.8430514960859990525, 1485.625134838489885, 221.0008352635990150 ) ) ;
#64397=CARTESIAN_POINT ( 'NONE',  ( 20.05786438499999846, 1473.530630424389983, 207.1970391306990109 ) ) ;
#64417=CARTESIAN_POINT ( 'NONE',  ( -7.098697224140000372, 1427.010778451219949, 204.8644842388889913 ) ) ;
#64420=CARTESIAN_POINT ( 'NONE',  ( 10.26924672323419863, 1481.505245612710041, 214.9441554700569839 ) ) ;
#64426=CARTESIAN_POINT ( 'NONE',  ( -10.51530743187480077, 1480.028629462490017, 208.9546532503999856 ) ) ;
#64429=CARTESIAN_POINT ( 'NONE',  ( 2.474966857995990033, 1497.110993154729840, 196.9665763241029879 ) ) ;
#64434=CARTESIAN_POINT ( 'NONE',  ( 11.29707874440000026, 1420.194464914089849, 198.6147532060990102 ) ) ;
#64435=CARTESIAN_POINT ( 'NONE',  ( 0.4820566092233740108, 1475.187528322450135, 220.5330728396190239 ) ) ;
#64441=CARTESIAN_POINT ( 'NONE',  ( 11.78015744380379815, 1421.994974570560089, 207.2729246609449945 ) ) ;
#64442=CARTESIAN_POINT ( 'NONE',  ( -9.600701647585090370, 1440.346316946680190, 206.2437467786620005 ) ) ;
#64444=ORIENTED_EDGE ( 'NONE', *, *, #1488, .T. ) ;
#64446=TOROIDAL_SURFACE ( 'NONE', #78730, 8.800000000000000711, 1.000000000000000000 ) ;
#64451=FACE_OUTER_BOUND ( 'NONE', #27796, .T. ) ;
#64453=CARTESIAN_POINT ( 'NONE',  ( -17.30417025350569915, 1419.800952382169953, 207.6230020391829783 ) ) ;
#64462=CARTESIAN_POINT ( 'NONE',  ( 4.163173984530029514, 1457.139433339820016, 199.2031175087780070 ) ) ;
#64475=CARTESIAN_POINT ( 'NONE',  ( 1.093792492990000031, 1515.225200552689785, 204.7965979425590035 ) ) ;
#64476=CARTESIAN_POINT ( 'NONE',  ( -14.53046663459189958, 1417.356912740600137, 203.2574546587219970 ) ) ;
#64482=CARTESIAN_POINT ( 'NONE',  ( -4.327507137520000491, 1515.138941066290045, 208.4081369698370167 ) ) ;
#64486=CARTESIAN_POINT ( 'NONE',  ( 8.631780704876279131, 1438.018275767699834, 210.0183142686710198 ) ) ;
#64487=EDGE_LOOP ( 'NONE', ( #89155, #29253, #43054, #95940 ) ) ;
#64488=CARTESIAN_POINT ( 'NONE',  ( 2.564256839410000488, 1486.020400378790100, 198.5121203060990354 ) ) ;
#64489=CARTESIAN_POINT ( 'NONE',  ( 5.270386862360000535, 1477.861965715389942, 199.8733389948390027 ) ) ;
#64491=CARTESIAN_POINT ( 'NONE',  ( -11.73701470839999850, 1491.048748728590226, 207.6304560743390084 ) ) ;
#64492=CARTESIAN_POINT ( 'NONE',  ( -17.00797328670000397, 1417.537217351680056, 207.7155449971589860 ) ) ;
#64499=CARTESIAN_POINT ( 'NONE',  ( -12.23489732466240021, 1490.237667237379810, 209.6383001084460034 ) ) ;
#64500=CARTESIAN_POINT ( 'NONE',  ( -4.969384015369690211, 1508.551704408389924, 206.3370868630439929 ) ) ;
#64505=CARTESIAN_POINT ( 'NONE',  ( 10.02631634006560191, 1469.909548164330090, 210.1023831811019988 ) ) ;
#64513=CARTESIAN_POINT ( 'NONE',  ( -19.61848387020800288, 1466.208095908119958, 204.1942870921240001 ) ) ;
#64522=EDGE_CURVE ( 'NONE', #45555, #94338, #102088, .T. ) ;
#64527=CARTESIAN_POINT ( 'NONE',  ( -4.523944140811339665, 1455.378620635879997, 200.8408219016489795 ) ) ;
#64532=CARTESIAN_POINT ( 'NONE',  ( 3.829619994797929916, 1515.551704292389786, 207.2788821832570250 ) ) ;
#64533=VERTEX_POINT ( 'NONE', #12451 ) ;
#64534=CARTESIAN_POINT ( 'NONE',  ( 2.707841495209149851, 1485.005101276989990, 220.6627816910599904 ) ) ;
#64535=CARTESIAN_POINT ( 'NONE',  ( 11.55794785089999976, 1501.267050509989986, 208.2533511322130266 ) ) ;
#64543=CARTESIAN_POINT ( 'NONE',  ( 8.680203951845038901, 1482.515033173300026, 217.3319919233640007 ) ) ;
#64553=CARTESIAN_POINT ( 'NONE',  ( 5.031477915346656005, 1455.301335138442937, 217.6180370876550114 ) ) ;
#64570=AXIS2_PLACEMENT_3D ( 'NONE', #103113, #26414, #70128 ) ;
#64575=CARTESIAN_POINT ( 'NONE',  ( 7.934673110537849183, 1428.710417030969893, 214.3182389180220184 ) ) ;
#64577=CARTESIAN_POINT ( 'NONE',  ( -9.638453515383760717, 1462.007706823630087, 206.9654734332999908 ) ) ;
#64588=CARTESIAN_POINT ( 'NONE',  ( -8.716383294119999903, 1450.962816624490188, 203.1307156043189934 ) ) ;
#64592=CARTESIAN_POINT ( 'NONE',  ( 4.077242828495350579, 1515.224507406410112, 212.7046838410809926 ) ) ;
#64599=CARTESIAN_POINT ( 'NONE',  ( -14.67677013559999999, 1415.730435299999954, 205.0458841098590028 ) ) ;
#64603=CARTESIAN_POINT ( 'NONE',  ( -4.173142725735850433, 1447.222512570230037, 213.8729899181259952 ) ) ;
#64614=CARTESIAN_POINT ( 'NONE',  ( 4.989246313819999834, 1471.909539260290103, 189.7082128665990126 ) ) ;
#64633=CARTESIAN_POINT ( 'NONE',  ( 12.06965614970759937, 1491.404045832239945, 206.8238433162970011 ) ) ;
#64642=CARTESIAN_POINT ( 'NONE',  ( -13.59512407998240135, 1507.703338069740084, 209.3532897553030239 ) ) ;
#64644=AXIS2_PLACEMENT_3D ( 'NONE', #4421, #73267, #48071 ) ;
#64647=B_SPLINE_CURVE_WITH_KNOTS ( 'NONE', 3,
 ( #84030, #74553, #32539, #14620 ),
 .UNSPECIFIED., .F., .F.,
 ( 4, 4 ),
 ( 0.000000000000000000, 1.000000000000000000 ),
 .UNSPECIFIED. ) ;
#64650=ADVANCED_FACE ( 'NONE', ( #10815 ), #51071, .T. ) ;
#64652=CARTESIAN_POINT ( 'NONE',  ( 11.44311708778599979, 1501.817457278790016, 208.4257042484660190 ) ) ;
#64653=CARTESIAN_POINT ( 'NONE',  ( 13.52268460260000005, 1497.923627545689897, 227.8730058995990078 ) ) ;
#64654=CARTESIAN_POINT ( 'NONE',  ( -3.617573937782270210, 1497.333809982809953, 198.4503636364750037 ) ) ;
#64659=B_SPLINE_CURVE_WITH_KNOTS ( 'NONE', 3,
 ( #13913, #48098, #66020, #26740, #67669, #60362, #60928, #77165, #102336, #25621, #84447, #33468, #8822, #59813, #94484, #17756, #41352, #93933, #43007, #41894, #35143, #59269, #102877, #26175, #7194, #50320, #95058, #110195, #76597, #76051, #51959, #67118, #101219, #86101 ),
 .UNSPECIFIED., .F., .F.,
 ( 4, 3, 3, 3, 3, 3, 3, 3, 3, 3, 3, 4 ),
 ( -13.43342673250000097, -12.68470386051800070, -11.93598098853600042, -11.14531161610780075, -10.30911549555539963, -9.267678416573820854, -8.124443764497049969, -7.336535162872540816, -6.414797305390919746, -5.580366644398009335, -4.830730724985089708, -4.119224442280000176 ),
 .UNSPECIFIED. ) ;
#64660=CARTESIAN_POINT ( 'NONE',  ( 9.247631459069999948, 1454.170661380389902, 214.4254682548290134 ) ) ;
#64668=CARTESIAN_POINT ( 'NONE',  ( 2.329898843065079994, 1515.219291385629958, 204.7964424078519983 ) ) ;
#64673=CARTESIAN_POINT ( 'NONE',  ( -5.077909815922139636, 1463.916899788050159, 200.2638641301039968 ) ) ;
#64692=CARTESIAN_POINT ( 'NONE',  ( -17.69166861870969853, 1508.551704428830135, 211.7662683139330113 ) ) ;
#64700=CARTESIAN_POINT ( 'NONE',  ( -9.090368357078379091, 1450.929620059189801, 207.4549948248679812 ) ) ;
#64712=CIRCLE ( 'NONE', #45049, 6.646318662569999702 ) ;
#64731=LINE ( 'NONE', #22106, #100433 ) ;
#64733=CARTESIAN_POINT ( 'NONE',  ( 12.20133708979999909, 1421.549213611169989, 205.4486904848489814 ) ) ;
#64748=CARTESIAN_POINT ( 'NONE',  ( 9.292547705917240108, 1425.240615715940748, 195.5975308281553566 ) ) ;
#64749=VECTOR ( 'NONE', #108273, 1000.000000000000000 ) ;
#64750=CARTESIAN_POINT ( 'NONE',  ( 1.021942164559999977, 1443.686436469889713, 217.9982604250890006 ) ) ;
#64762=CARTESIAN_POINT ( 'NONE',  ( -15.65196091179999982, 1508.451915991289980, 214.9530002531589901 ) ) ;
#64764=DIRECTION ( 'NONE',  ( 0.000000000000000000, 1.000000000000000000, 0.000000000000000000 ) ) ;
#64765=CARTESIAN_POINT ( 'NONE',  ( -5.345848780929999933, 1483.903127912989930, 199.7205304764490279 ) ) ;
#64775=CARTESIAN_POINT ( 'NONE',  ( 7.242271949250000063, 1428.269950913389948, 213.9693205564990137 ) ) ;
#64782=CARTESIAN_POINT ( 'NONE',  ( -11.92256551290000033, 1502.127826907089911, 209.4204567382010111 ) ) ;
#64790=DIRECTION ( 'NONE',  ( -1.000000000000000000, 0.000000000000000000, 0.000000000000000000 ) ) ;
#64794=CARTESIAN_POINT ( 'NONE',  ( 0.6118612315922750122, 1515.137305168469993, 213.4493959364910154 ) ) ;
#64796=CARTESIAN_POINT ( 'NONE',  ( -8.543213252583260697, 1478.735612270709908, 217.0402877408899940 ) ) ;
#64800=ORIENTED_EDGE ( 'NONE', *, *, #9616, .T. ) ;
#64802=CARTESIAN_POINT ( 'NONE',  ( -11.51580851839999831, 1504.609797615890102, 207.7314770397890129 ) ) ;
#64803=CARTESIAN_POINT ( 'NONE',  ( -21.46486267529380143, 1504.440111944700220, 215.6677449661270032 ) ) ;
#64805=CARTESIAN_POINT ( 'NONE',  ( 1.193369943926424703, 1473.153843175627799, 219.2662284112174120 ) ) ;
#64812=CARTESIAN_POINT ( 'NONE',  ( 10.03610466974719984, 1469.085538504640226, 209.1195785090949926 ) ) ;
#64814=CARTESIAN_POINT ( 'NONE',  ( -4.329473944230000093, 1458.307963197089975, 218.4835595929489784 ) ) ;
#64817=ORIENTED_EDGE ( 'NONE', *, *, #100705, .F. ) ;
#64830=ADVANCED_FACE ( 'NONE', ( #5937 ), #34066, .F. ) ;
#64834=CARTESIAN_POINT ( 'NONE',  ( -14.78755727007779974, 1487.414112128270062, 194.1688363173670098 ) ) ;
#64840=CARTESIAN_POINT ( 'NONE',  ( 0.3759925524705069466, 1425.634515328159978, 191.1019336871629832 ) ) ;
#64846=CARTESIAN_POINT ( 'NONE',  ( 8.409376565895700040, 1438.261224657589764, 211.4481330912490193 ) ) ;
#64853=ORIENTED_EDGE ( 'NONE', *, *, #60523, .T. ) ;
#64854=CARTESIAN_POINT ( 'NONE',  ( -2.157536728407475568, 1397.913060387289988, 210.3005136483574518 ) ) ;
#64858=B_SPLINE_CURVE_WITH_KNOTS ( 'NONE', 3,
 ( #97892, #4940, #99540, #81098, #57030, #63245 ),
 .UNSPECIFIED., .F., .F.,
 ( 4, 2, 4 ),
 ( 0.000000000000000000, 0.5000000000000000000, 1.000000000000000000 ),
 .UNSPECIFIED. ) ;
#64859=CARTESIAN_POINT ( 'NONE',  ( -6.273787032870000502, 1415.168582340579860, 205.7307369784189746 ) ) ;
#64868=CARTESIAN_POINT ( 'NONE',  ( -17.72676975039999903, 1418.059941342760112, 206.6000183712389742 ) ) ;
#64872=CARTESIAN_POINT ( 'NONE',  ( -3.118824320620000368, 1475.108726717689933, 218.9463081056090061 ) ) ;
#64873=ADVANCED_FACE ( 'NONE', ( #17046 ), #106364, .F. ) ;
#64877=CARTESIAN_POINT ( 'NONE',  ( -2.426602077163350302, 1454.706936359410065, 198.9117694354199841 ) ) ;
#64888=CARTESIAN_POINT ( 'NONE',  ( 7.886556196039999911, 1423.699161883410170, 195.9191256520989839 ) ) ;
#64890=CARTESIAN_POINT ( 'NONE',  ( 1.997239979113719865, 1508.551704408389924, 219.6740723297500040 ) ) ;
#64894=CARTESIAN_POINT ( 'NONE',  ( -12.24467222372750008, 1502.437705295270007, 208.9618294917469825 ) ) ;
#64896=CARTESIAN_POINT ( 'NONE',  ( -4.844790491859999548, 1489.192796749890022, 188.8948260823989926 ) ) ;
#64900=CARTESIAN_POINT ( 'NONE',  ( -3.269263786600000277, 1476.740800597890029, 199.2818572616789936 ) ) ;
#64902=EDGE_LOOP ( 'NONE', ( #79268, #110413, #83122, #28952 ) ) ;
#64903=CARTESIAN_POINT ( 'NONE',  ( 5.076304971681840250, 1469.790025430949981, 187.8425727480230023 ) ) ;
#64906=CARTESIAN_POINT ( 'NONE',  ( -2.329939114882829898, 1515.551844914359890, 205.1381281626180169 ) ) ;
#64910=FACE_OUTER_BOUND ( 'NONE', #73686, .T. ) ;
#64927=CARTESIAN_POINT ( 'NONE',  ( 1.514120561980000183E-16, 1515.551704408389924, 209.1218459616989946 ) ) ;
#64930=CARTESIAN_POINT ( 'NONE',  ( -9.622749971728280727, 1447.247763375919931, 211.4452405505059858 ) ) ;
#64935=CARTESIAN_POINT ( 'NONE',  ( 7.183386785930029994, 1424.944879424049986, 212.8809111208099694 ) ) ;
#64939=CARTESIAN_POINT ( 'NONE',  ( -11.70942943321529839, 1491.329393039050046, 206.7632756908639919 ) ) ;
#64947=ORIENTED_EDGE ( 'NONE', *, *, #82259, .T. ) ;
#64953=CARTESIAN_POINT ( 'NONE',  ( 9.380465540465371177, 1451.944138759889938, 210.1274675918040202 ) ) ;
#64954=CARTESIAN_POINT ( 'NONE',  ( 6.016568497259999759, 1422.672370635280004, 194.9161982602989838 ) ) ;
#64957=CARTESIAN_POINT ( 'NONE',  ( 20.99949974029999922, 1495.227265342490000, 211.1851663224690014 ) ) ;
#64967=CARTESIAN_POINT ( 'NONE',  ( 10.19012721036619951, 1481.561516676249994, 215.0834239772050012 ) ) ;
#64971=CARTESIAN_POINT ( 'NONE',  ( -10.70617203047970101, 1481.026974688039900, 208.9677961751969804 ) ) ;
#64975=CARTESIAN_POINT ( 'NONE',  ( 12.62890211870000101, 1420.357139060750114, 200.3668987843989839 ) ) ;
#64980=CARTESIAN_POINT ( 'NONE',  ( 5.009886284249999377, 1430.069699660889910, 217.1776678749689893 ) ) ;
#64982=CARTESIAN_POINT ( 'NONE',  ( 10.76705900790449988, 1423.512433835739785, 206.7766633243239767 ) ) ;
#64990=CARTESIAN_POINT ( 'NONE',  ( 11.02890202689059862, 1422.198172311190092, 210.7302511592479846 ) ) ;
#64991=CARTESIAN_POINT ( 'NONE',  ( -16.89965117564359787, 1419.540396951069852, 208.5087401362400215 ) ) ;
#64993=CARTESIAN_POINT ( 'NONE',  ( 1.865807842320000187, 1429.738386184189949, 217.2385783028290120 ) ) ;
#64995=CARTESIAN_POINT ( 'NONE',  ( -16.69591095510000045, 1417.051168577799899, 207.9278418973390217 ) ) ;
#64999=CARTESIAN_POINT ( 'NONE',  ( 3.776171005225210209, 1457.654323051970096, 199.8439998585350281 ) ) ;
#65000=CARTESIAN_POINT ( 'NONE',  ( 7.722830810765720422, 1424.481984735209835, 195.1132992968850033 ) ) ;
#65008=CARTESIAN_POINT ( 'NONE',  ( 8.800740351439999998, 1452.938977316690170, 191.5447439844990072 ) ) ;
#65010=CARTESIAN_POINT ( 'NONE',  ( 1.842962231260000028, 1515.551704408389924, 205.1377642093389966 ) ) ;
#65011=CARTESIAN_POINT ( 'NONE',  ( -14.35822996286229980, 1417.017622938350087, 203.2444471570910025 ) ) ;
#65017=CARTESIAN_POINT ( 'NONE',  ( 1.010561960472377230, 1484.609605269575013, 198.4571475875856663 ) ) ;
#65020=DIRECTION ( 'NONE',  ( 0.4794255386042031719, 0.000000000000000000, 0.8775825618903726477 ) ) ;
#65021=ORIENTED_EDGE ( 'NONE', *, *, #106934, .T. ) ;
#65023=CARTESIAN_POINT ( 'NONE',  ( 2.326513307810000430, 1476.258183369789776, 197.8633931413990013 ) ) ;
#65024=CARTESIAN_POINT ( 'NONE',  ( -16.79355120555579717, 1420.470915846049820, 203.2250788671829866 ) ) ;
#65026=FACE_OUTER_BOUND ( 'NONE', #47443, .T. ) ;
#65033=CARTESIAN_POINT ( 'NONE',  ( -12.19432067802980058, 1490.774705066830165, 207.8227360995649917 ) ) ;
#65034=CARTESIAN_POINT ( 'NONE',  ( -4.985290750076490696, 1508.551704408389924, 206.5066873982580091 ) ) ;
#65042=CARTESIAN_POINT ( 'NONE',  ( 10.15612571795790053, 1470.518962983220035, 210.4951917859000048 ) ) ;
#65050=DIRECTION ( 'NONE',  ( -0.02616798426450828510, 0.9993150019883944024, -0.02616798426450858348 ) ) ;
#65052=CARTESIAN_POINT ( 'NONE',  ( -9.632490594537660655, 1464.050392106980098, 228.1736160443419976 ) ) ;
#65068=ORIENTED_EDGE ( 'NONE', *, *, #78924, .F. ) ;
#65072=CARTESIAN_POINT ( 'NONE',  ( 12.61744324630000058, 1500.191175618890156, 207.7465061732789877 ) ) ;
#65080=CARTESIAN_POINT ( 'NONE',  ( 11.13185944637359803, 1480.405602026969973, 211.3596403160480008 ) ) ;
#65086=CARTESIAN_POINT ( 'NONE',  ( 4.803830733223059646, 1471.771524698999883, 187.6888356675239891 ) ) ;
#65093=DIRECTION ( 'NONE',  ( -0.02616798426500960631, 0.9993150019883683122, -0.02616798426500990815 ) ) ;
#65095=CARTESIAN_POINT ( 'NONE',  ( -21.10721348755030036, 1508.551704408389924, 210.4652812066999843 ) ) ;
#65116=CARTESIAN_POINT ( 'NONE',  ( -8.281161535991449441, 1436.480211923179922, 214.3424743920830053 ) ) ;
#65126=CARTESIAN_POINT ( 'NONE',  ( -7.405436629479999588, 1451.940595730289942, 201.5764829818989767 ) ) ;
#65135=CARTESIAN_POINT ( 'NONE',  ( 2.245848864970000136, 1508.551704888590166, 219.9346363045989960 ) ) ;
#65137=CARTESIAN_POINT ( 'NONE',  ( -1.845809110569999856, 1431.027514053989762, 214.5308736330090085 ) ) ;
#65138=CARTESIAN_POINT ( 'NONE',  ( -4.227481132736940594, 1441.218242348629929, 201.3833600324580289 ) ) ;
#65140=CARTESIAN_POINT ( 'NONE',  ( 7.682163124739999738, 1421.658071144350060, 195.7645034974990210 ) ) ;
#65141=CARTESIAN_POINT ( 'NONE',  ( -18.26024740272439928, 1443.256143005099830, 213.5656067199900008 ) ) ;
#65144=CARTESIAN_POINT ( 'NONE',  ( -14.30379464810000023, 1503.190943967589874, 209.1271418435919998 ) ) ;
#65146=ORIENTED_EDGE ( 'NONE', *, *, #45919, .T. ) ;
#65149=EDGE_CURVE ( 'NONE', #20110, #102270, #73236, .T. ) ;
#65153=CARTESIAN_POINT ( 'NONE',  ( 2.587518041203992425, 1464.354613572267681, 199.6306109175279460 ) ) ;
#65157=CARTESIAN_POINT ( 'NONE',  ( -5.881379503709999845, 1428.766218426890191, 203.1321793329989873 ) ) ;
#65160=CARTESIAN_POINT ( 'NONE',  ( -12.48995958559999941, 1501.883328862989856, 211.6213070104490157 ) ) ;
#65167=CARTESIAN_POINT ( 'NONE',  ( 10.13545575494789830, 1453.511789163979984, 212.2748783515349942 ) ) ;
#65174=B_SPLINE_SURFACE_WITH_KNOTS ( 'NONE', 5, 1, ( 
 ( #28192, #54533 ),
 ( #79718, #89200 ),
 ( #71344, #99630 ),
 ( #14532, #53985 ),
 ( #22918, #19784 ),
 ( #62952, #105458 ) ),
 .UNSPECIFIED., .F., .F., .F.,
 ( 6, 6 ),
 ( 2, 2 ),
 ( 0.000000000000000000, 3.689078941800000067 ),
 ( 0.000000000000000000, 14.00000000000000000 ),
 .UNSPECIFIED. ) ;
#65175=CARTESIAN_POINT ( 'NONE',  ( 12.07900496321360073, 1491.418085619319982, 206.8679904804870091 ) ) ;
#65187=CARTESIAN_POINT ( 'NONE',  ( -9.609620985028570317, 1464.248423674519927, 228.1966035519590150 ) ) ;
#65191=CARTESIAN_POINT ( 'NONE',  ( -4.944749881069999908, 1455.119008683790071, 201.0836254654890070 ) ) ;
#65194=CARTESIAN_POINT ( 'NONE',  ( 7.786818409689999498, 1426.121526212180015, 211.8122417738590002 ) ) ;
#65197=CARTESIAN_POINT ( 'NONE',  ( -19.06854921284269722, 1419.167091098079936, 205.9066248690829752 ) ) ;
#65201=CARTESIAN_POINT ( 'NONE',  ( 9.609447197979999800, 1453.954725363390025, 213.7354802858189942 ) ) ;
#65203=ORIENTED_EDGE ( 'NONE', *, *, #7195, .F. ) ;
#65224=ORIENTED_EDGE ( 'NONE', *, *, #8810, .T. ) ;
#65225=ADVANCED_FACE ( 'NONE', ( #96289 ), #81340, .T. ) ;
#65227=CARTESIAN_POINT ( 'NONE',  ( -5.004100793020000104, 1425.392060909700149, 209.0067307068910054 ) ) ;
#65259=CARTESIAN_POINT ( 'NONE',  ( 12.31397506763359928, 1492.288124162400209, 209.9699710670110164 ) ) ;
#65264=CARTESIAN_POINT ( 'NONE',  ( -7.217374241420609238, 1424.786834349990158, 212.8040540257917712 ) ) ;
#65271=CARTESIAN_POINT ( 'NONE',  ( 5.826428076080000906, 1473.811884028689974, 218.9454251420289950 ) ) ;
#65272=CARTESIAN_POINT ( 'NONE',  ( 11.06028399019999853, 1425.506596454839837, 205.4898845224990112 ) ) ;
#65273=CARTESIAN_POINT ( 'NONE',  ( -1.700022450220517012, 1497.975818191871895, 197.9538752838212474 ) ) ;
#65281=CARTESIAN_POINT ( 'NONE',  ( 10.14133495641580041, 1480.626569447219936, 206.2493899992390141 ) ) ;
#65287=CARTESIAN_POINT ( 'NONE',  ( 2.852546465570000134, 1442.789416142390110, 217.5399594921489950 ) ) ;
#65302=CARTESIAN_POINT ( 'NONE',  ( 11.19147557906589974, 1422.145537183640045, 210.4506353095700035 ) ) ;
#65307=CARTESIAN_POINT ( 'NONE',  ( -8.756504656448949930, 1437.746547805949831, 210.1047563292509892 ) ) ;
#65313=B_SPLINE_CURVE_WITH_KNOTS ( 'NONE', 3,
 ( #90296, #13029, #81897, #38796, #73531, #98708, #65677, #39357, #13576, #72971, #31496, #56719 ),
 .UNSPECIFIED., .F., .F.,
 ( 4, 2, 1, 1, 2, 2, 4 ),
 ( 0.000000000000000000, 0.2499999999996412869, 0.3749999999994620414, 0.4374999999993723909, 0.4687499999993651745, 0.4999999999993579580, 1.000000000000000000 ),
 .UNSPECIFIED. ) ;
#65315=ORIENTED_EDGE ( 'NONE', *, *, #85746, .T. ) ;
#65320=ORIENTED_EDGE ( 'NONE', *, *, #30388, .T. ) ;
#65324=CARTESIAN_POINT ( 'NONE',  ( 4.157308324739999783, 1454.950057953289843, 217.7287963511690236 ) ) ;
#65328=CARTESIAN_POINT ( 'NONE',  ( 4.329448776040000446, 1515.064792882589927, 206.7917118356089929 ) ) ;
#65332=CARTESIAN_POINT ( 'NONE',  ( 9.345710454894810226, 1422.635914553260136, 212.8840094578699791 ) ) ;
#65335=CARTESIAN_POINT ( 'NONE',  ( 1.179283247357060027, 1515.094876538340031, 213.4505069693209975 ) ) ;
#65337=CARTESIAN_POINT ( 'NONE',  ( -7.505040120567149309, 1478.213044889750108, 217.9841396579450077 ) ) ;
#65339=EDGE_CURVE ( 'NONE', #38113, #26627, #75819, .T. ) ;
#65345=CIRCLE ( 'NONE', #63668, 11.73448142120001059 ) ;
#65346=CARTESIAN_POINT ( 'NONE',  ( -21.44822655731880090, 1506.215343320510101, 215.9887031352290023 ) ) ;
#65348=CARTESIAN_POINT ( 'NONE',  ( -1.609854712855105952, 1474.055975362519348, 219.2485333660200126 ) ) ;
#65354=CARTESIAN_POINT ( 'NONE',  ( -3.391530762879999994, 1456.859262623989935, 218.0010147046889983 ) ) ;
#65367=SURFACE_STYLE_FILL_AREA ( #64262 ) ;
#65389=CARTESIAN_POINT ( 'NONE',  ( 2.143373558913630461, 1458.476679308760822, 199.7396688924466446 ) ) ;
#65391=CARTESIAN_POINT ( 'NONE',  ( 3.962577075963499507, 1441.289921133800135, 217.4194056301390106 ) ) ;
#65397=CARTESIAN_POINT ( 'NONE',  ( -10.87812260669999986, 1471.332318691390128, 207.6541763658389925 ) ) ;
#65403=CARTESIAN_POINT ( 'NONE',  ( 4.329448776040000446, 1515.064792882589927, 209.0973262533439936 ) ) ;
#65406=CARTESIAN_POINT ( 'NONE',  ( 10.94557456650000127, 1490.490906152089792, 205.6963937967290121 ) ) ;
#65410=CARTESIAN_POINT ( 'NONE',  ( 9.682514688702729799, 1436.279831273820037, 210.8541350352949735 ) ) ;
#65413=CARTESIAN_POINT ( 'NONE',  ( -17.70265010310000164, 1417.829914391519878, 206.4711793681690040 ) ) ;
#65418=CARTESIAN_POINT ( 'NONE',  ( 1.247885727509999931, 1474.780154000190123, 220.0763491201989837 ) ) ;
#65423=CARTESIAN_POINT ( 'NONE',  ( 0.9489938987924170233, 1456.076817772840059, 198.6004356744230108 ) ) ;
#65424=DIRECTION ( 'NONE',  ( 9.158755289808628626E-47, -1.000000000000000000, 1.836970198721029688E-16 ) ) ;
#65425=B_SPLINE_SURFACE_WITH_KNOTS ( 'NONE', 5, 5, ( 
 ( #18542, #67892, #7408, #101439, #58926, #93057 ),
 ( #72298, #37573, #89071, #28065, #106429, #37016 ),
 ( #78480, #36468, #96940, #62254, #96381, #20206 ),
 ( #1793, #38117, #3443, #54406, #35930, #53863 ),
 ( #63898, #88538, #12358, #105331, #61701, #11822 ),
 ( #46546, #45992, #3993, #98013, #63362, #10163 ),
 ( #80680, #27515, #79050, #86870, #44337, #29714 ),
 ( #19659, #70114, #95822, #70665, #80123, #53294 ),
 ( #71774, #52736, #104779, #88000, #71210, #62825 ) ),
 .UNSPECIFIED., .F., .F., .F.,
 ( 6, 3, 6 ),
 ( 6, 6 ),
 ( 0.000000000000000000, 1.710105857910000138, 3.420211715829999832 ),
 ( 0.000000000000000000, 2.000000000000000000 ),
 .UNSPECIFIED. ) ;
#65427=CARTESIAN_POINT ( 'NONE',  ( -9.839102621363029044, 1472.123545760580100, 211.7008534868720062 ) ) ;
#65428=CARTESIAN_POINT ( 'NONE',  ( -5.478760788770000723, 1476.176840370589844, 217.9931547433689900 ) ) ;
#65430=VERTEX_POINT ( 'NONE', #51139 ) ;
#65434=CARTESIAN_POINT ( 'NONE',  ( -1.620287784100000295, 1443.296048881190018, 200.2316306629689677 ) ) ;
#65435=CARTESIAN_POINT ( 'NONE',  ( 8.260488040129999376, 1424.458407895899882, 195.8858451325990302 ) ) ;
#65446=CARTESIAN_POINT ( 'NONE',  ( -2.673754402869999769, 1457.395679039389961, 218.6654034043990009 ) ) ;
#65449=ADVANCED_FACE ( 'NONE', ( #100425 ), #45532, .T. ) ;
#65452=CARTESIAN_POINT ( 'NONE',  ( -4.011846058889999789, 1474.851293822189973, 198.8411774138990040 ) ) ;
#65463=CARTESIAN_POINT ( 'NONE',  ( -15.07989985220060092, 1508.551704408389924, 214.8207627136849851 ) ) ;
#65469=ADVANCED_FACE ( 'NONE', ( #50040 ), #32672, .T. ) ;
#65473=DIRECTION ( 'NONE',  ( 9.230617842401318720E-47, -1.000000000000000000, 1.836970198721029688E-16 ) ) ;
#65488=CARTESIAN_POINT ( 'NONE',  ( 7.452937308169480524, 1425.221714708150103, 212.3436467550869793 ) ) ;
#65491=CARTESIAN_POINT ( 'NONE',  ( 10.56407631929999980, 1452.658139941989930, 209.7432180256290053 ) ) ;
#65500=VERTEX_POINT ( 'NONE', #49491 ) ;
#65514=CIRCLE ( 'NONE', #17174, 8.104319688360000384 ) ;
#65515=ORIENTED_EDGE ( 'NONE', *, *, #53839, .T. ) ;
#65519=CARTESIAN_POINT ( 'NONE',  ( -7.514943502940000464, 1426.327996137909849, 205.9160340660789927 ) ) ;
#65522=CARTESIAN_POINT ( 'NONE',  ( 10.86020916433990102, 1481.036884354570020, 213.7433009987580022 ) ) ;
#65527=CARTESIAN_POINT ( 'NONE',  ( -11.41773502901409998, 1481.611637904830104, 209.4132993426249811 ) ) ;
#65530=CARTESIAN_POINT ( 'NONE',  ( 9.260035559154880858, 1503.457705115180033, 217.8739325455829885 ) ) ;
#65531=CARTESIAN_POINT ( 'NONE',  ( 12.02531869610000115, 1420.571450649919825, 199.9272147486889821 ) ) ;
#65532=CARTESIAN_POINT ( 'NONE',  ( 0.1435280708731850041, 1475.283311921460154, 220.5458192635479975 ) ) ;
#65535=CARTESIAN_POINT ( 'NONE',  ( -5.215695737369999918, 1495.379815458989924, 198.7908035812990022 ) ) ;
#65539=CARTESIAN_POINT ( 'NONE',  ( 11.30538286922199909, 1426.159524226919984, 206.5002785976879807 ) ) ;
#65543=CARTESIAN_POINT ( 'NONE',  ( 5.120453548759999585, 1471.466545119689954, 214.4276395123089856 ) ) ;
#65547=CARTESIAN_POINT ( 'NONE',  ( 9.517773336257400629, 1423.536455532770105, 209.9636451762389981 ) ) ;
#65548=CARTESIAN_POINT ( 'NONE',  ( 11.65242884602639961, 1425.717965413690081, 202.8942723744929992 ) ) ;
#65550=CARTESIAN_POINT ( 'NONE',  ( 2.398699649889999730, 1429.053736725890076, 217.0724297081890199 ) ) ;
#65552=CARTESIAN_POINT ( 'NONE',  ( -4.685705521985438438, 1475.329346039780148, 218.3671617030974801 ) ) ;
#65564=CARTESIAN_POINT ( 'NONE',  ( 17.78630097849999814, 1455.623587567290087, 200.4657979530790044 ) ) ;
#65566=CARTESIAN_POINT ( 'NONE',  ( 0.008453540420540530190, 1515.389376838289991, 204.8287432943390058 ) ) ;
#65568=CARTESIAN_POINT ( 'NONE',  ( 2.292469808877632520, 1497.477225423111577, 197.6467893764333326 ) ) ;
#65578=VERTEX_POINT ( 'NONE', #74693 ) ;
#65582=CARTESIAN_POINT ( 'NONE',  ( -11.14576561989999881, 1491.244072761289999, 209.5089610898519936 ) ) ;
#65586=CARTESIAN_POINT ( 'NONE',  ( -13.35310380080168002, 1481.629060506388441, 225.5919806602003064 ) ) ;
#65596=CARTESIAN_POINT ( 'NONE',  ( 2.023323367690000207, 1501.741525076489779, 230.4104378513989957 ) ) ;
#65599=CARTESIAN_POINT ( 'NONE',  ( 10.04076066863449945, 1469.831999276539818, 209.8600323314049945 ) ) ;
#65600=CARTESIAN_POINT ( 'NONE',  ( 17.83968203154910270, 1430.541692949039998, 212.9271915631379954 ) ) ;
#65607=CARTESIAN_POINT ( 'NONE',  ( -9.518190392760001117, 1465.040135640790140, 228.2885054898990234 ) ) ;
#65609=CARTESIAN_POINT ( 'NONE',  ( 5.216723163609201741, 1497.653739079350316, 197.6766713243789013 ) ) ;
#65611=CARTESIAN_POINT ( 'NONE',  ( 7.015117299519999960, 1480.620769302089911, 206.9956269080190054 ) ) ;
#65621=B_SPLINE_CURVE_WITH_KNOTS ( 'NONE', 3,
 ( #75334, #83706, #107809, #23240, #57439, #31096, #99390, #56868, #33851, #61312 ),
 .UNSPECIFIED., .F., .F.,
 ( 4, 2, 2, 2, 4 ),
 ( 0.000000000000000000, 0.2500000000000000555, 0.5000000000000001110, 0.7500000000000002220, 1.000000000000000000 ),
 .UNSPECIFIED. ) ;
#65627=CARTESIAN_POINT ( 'NONE',  ( -2.848799080821822205, 1456.353470596306806, 200.0717474131963343 ) ) ;
#65628=CARTESIAN_POINT ( 'NONE',  ( 11.81504872310000032, 1500.768363563890034, 208.0408261944689912 ) ) ;
#65633=CARTESIAN_POINT ( 'NONE',  ( 4.757611653739999724, 1476.697157691990014, 198.4937409947989977 ) ) ;
#65638=CARTESIAN_POINT ( 'NONE',  ( -4.354848045695810299, 1481.954746482949986, 231.1149966751839884 ) ) ;
#65645=CARTESIAN_POINT ( 'NONE',  ( -20.35012269109810035, 1508.551704411970150, 210.1667554882619982 ) ) ;
#65663=CARTESIAN_POINT ( 'NONE',  ( -18.92577228117313481, 1508.457812386920523, 210.3413885190254859 ) ) ;
#65664=CARTESIAN_POINT ( 'NONE',  ( -9.730115140653261108, 1461.904593459310036, 207.4327562979160291 ) ) ;
#65677=CARTESIAN_POINT ( 'NONE',  ( -10.34125195379056450, 1480.634459757738796, 207.0903537657474658 ) ) ;
#65682=CARTESIAN_POINT ( 'NONE',  ( -11.28871479695359881, 1500.517265169780103, 210.9741532246169982 ) ) ;
#65694=CARTESIAN_POINT ( 'NONE',  ( -10.97569758906830018, 1482.624302103220089, 205.8415845986210115 ) ) ;
#65701=CARTESIAN_POINT ( 'NONE',  ( 10.93679547204000002, 1490.434980368090010, 209.9321327948960061 ) ) ;
#65703=CARTESIAN_POINT ( 'NONE',  ( 2.113994577280214227, 1464.204615851377184, 199.5304910285045992 ) ) ;
#65705=CARTESIAN_POINT ( 'NONE',  ( -6.790400283243552160, 1439.837278262902373, 203.5909105148159313 ) ) ;
#65710=CARTESIAN_POINT ( 'NONE',  ( -9.234075267490000627, 1498.091069991990025, 216.0247435465689989 ) ) ;
#65724=CARTESIAN_POINT ( 'NONE',  ( 12.33229080803599942, 1492.071651757490145, 209.1313924691960153 ) ) ;
#65728=CARTESIAN_POINT ( 'NONE',  ( 12.88825199978909986, 1421.219518988400068, 204.9917899569869917 ) ) ;
#65730=ORIENTED_EDGE ( 'NONE', *, *, #20207, .F. ) ;
#65731=EDGE_CURVE ( 'NONE', #43895, #13558, #8957, .T. ) ;
#65734=CARTESIAN_POINT ( 'NONE',  ( 11.27339694765309908, 1433.557990533659904, 225.8166789516029951 ) ) ;
#65742=CARTESIAN_POINT ( 'NONE',  ( 7.800031391840000161, 1426.737474522780076, 212.0503234373089754 ) ) ;
#65762=CARTESIAN_POINT ( 'NONE',  ( -4.675548249330949702, 1462.620864918090092, 200.5633472018479893 ) ) ;
#65763=CARTESIAN_POINT ( 'NONE',  ( 1.362472229929999834, 1423.807295244410170, 191.1810882058989876 ) ) ;
#65768=EDGE_LOOP ( 'NONE', ( #67989, #47592, #19302, #20406 ) ) ;
#65771=ORIENTED_EDGE ( 'NONE', *, *, #25483, .F. ) ;
#65773=ADVANCED_FACE ( 'NONE', ( #19730 ), #108204, .T. ) ;
#65781=CARTESIAN_POINT ( 'NONE',  ( -12.33713420429999985, 1502.629388698589992, 208.8300189963289881 ) ) ;
#65784=ORIENTED_EDGE ( 'NONE', *, *, #9946, .T. ) ;
#65786=ORIENTED_EDGE ( 'NONE', *, *, #21486, .F. ) ;
#65803=CARTESIAN_POINT ( 'NONE',  ( 2.634457758659999538, 1441.548974666690128, 218.6895019696289921 ) ) ;
#65809=CARTESIAN_POINT ( 'NONE',  ( 9.658808656759559241, 1434.868392548590009, 207.4898433114610157 ) ) ;
#65812=EDGE_CURVE ( 'NONE', #74706, #95667, #61577, .T. ) ;
#65814=ORIENTED_EDGE ( 'NONE', *, *, #16467, .F. ) ;
#65819=ADVANCED_FACE ( 'NONE', ( #37085 ), #22545, .F. ) ;
#65821=CARTESIAN_POINT ( 'NONE',  ( 12.72079913470000001, 1426.539370631579914, 203.1228655698189982 ) ) ;
#65834=CARTESIAN_POINT ( 'NONE',  ( 10.93915268089999948, 1461.376312761390182, 209.8459655709470155 ) ) ;
#65835=CARTESIAN_POINT ( 'NONE',  ( 8.462050346931258460, 1424.499487015235445, 195.8146675219503265 ) ) ;
#65841=CARTESIAN_POINT ( 'NONE',  ( 8.324709289579081073, 1487.559664528698477, 202.1769454163824946 ) ) ;
#65848=CARTESIAN_POINT ( 'NONE',  ( -9.157162863174900025, 1440.811664631680060, 204.9830593813619828 ) ) ;
#65855=CARTESIAN_POINT ( 'NONE',  ( -8.783092974434230982, 1437.856998031400053, 209.9037047230029884 ) ) ;
#65856=CARTESIAN_POINT ( 'NONE',  ( -3.582837879391600033, 1515.224507406410112, 213.1990887901850158 ) ) ;
#65859=CARTESIAN_POINT ( 'NONE',  ( -15.17835049509060141, 1415.677402202029953, 208.2345230821440225 ) ) ;
#65871=CARTESIAN_POINT ( 'NONE',  ( 3.067487128190000245, 1454.793378140790082, 218.0351595015090140 ) ) ;
#65873=B_SPLINE_CURVE_WITH_KNOTS ( 'NONE', 5,
 ( #40543, #83642, #99879, #57379, #90942, #6937, #91506, #74718, #100449, #23732, #32145, #41094 ),
 .UNSPECIFIED., .F., .F.,
 ( 6, 3, 3, 6 ),
 ( 22.07912247049999976, 24.05556723879999836, 24.39387767419999875, 25.37426196462180172 ),
 .UNSPECIFIED. ) ;
#65874=CARTESIAN_POINT ( 'NONE',  ( -2.707190781069999996, 1444.178722878989902, 218.0787341613589945 ) ) ;
#65877=CARTESIAN_POINT ( 'NONE',  ( 12.68801352610000066, 1500.413650637289948, 208.6561538998189747 ) ) ;
#65878=CARTESIAN_POINT ( 'NONE',  ( 9.674883418626309961, 1463.833330980269920, 210.7190143815600152 ) ) ;
#65883=CARTESIAN_POINT ( 'NONE',  ( -11.54258847144769895, 1481.005615187450076, 211.6768298937909947 ) ) ;
#65884=VECTOR ( 'NONE', #109365, 999.9999999999998863 ) ;
#65890=ORIENTED_EDGE ( 'NONE', *, *, #45419, .T. ) ;
#65893=ADVANCED_FACE ( 'NONE', ( #16260 ), #48259, .F. ) ;
#65894=CARTESIAN_POINT ( 'NONE',  ( 13.65193357110329941, 1498.714159422929924, 227.8242311217019846 ) ) ;
#65900=CARTESIAN_POINT ( 'NONE',  ( -20.22049527400000102, 1484.072692924690045, 213.0524004518590004 ) ) ;
#65902=CARTESIAN_POINT ( 'NONE',  ( -3.840466235669999673, 1457.048098735890107, 217.8269071805590045 ) ) ;
#65906=CARTESIAN_POINT ( 'NONE',  ( -4.328976357965290234, 1515.082833801179959, 210.4724564393140156 ) ) ;
#65908=ORIENTED_EDGE ( 'NONE', *, *, #20676, .T. ) ;
#65933=CARTESIAN_POINT ( 'NONE',  ( -4.993214560040000194, 1391.653934889589891, 203.5347113830289913 ) ) ;
#65934=CARTESIAN_POINT ( 'NONE',  ( 10.75296554538699922, 1460.440714502600031, 207.1959050312180182 ) ) ;
#65938=CARTESIAN_POINT ( 'NONE',  ( 8.852952242565432783, 1461.582927576305110, 205.0540815658535507 ) ) ;
#65940=CARTESIAN_POINT ( 'NONE',  ( 4.948204956154519607, 1440.721229042110053, 216.9276863776850064 ) ) ;
#65947=FACE_OUTER_BOUND ( 'NONE', #17541, .T. ) ;
#65958=CARTESIAN_POINT ( 'NONE',  ( 7.646098387520000372, 1488.620979909889911, 200.2919901690490008 ) ) ;
#65959=CARTESIAN_POINT ( 'NONE',  ( -4.958564224928870168, 1476.141795758730041, 200.0452580833139962 ) ) ;
#65963=CIRCLE ( 'NONE', #94537, 11.71219856409999949 ) ;
#65966=ORIENTED_EDGE ( 'NONE', *, *, #93216, .T. ) ;
#65972=ADVANCED_FACE ( 'NONE', ( #36409 ), #38421, .T. ) ;
#65974=CARTESIAN_POINT ( 'NONE',  ( -14.09074480600290080, 1508.447712472369858, 216.3025742391060078 ) ) ;
#65975=CARTESIAN_POINT ( 'NONE',  ( -2.405152095979999682, 1474.348779541090153, 219.1148944409090120 ) ) ;
#65978=CARTESIAN_POINT ( 'NONE',  ( -3.811293930937523111, 1508.139652414328793, 220.7071210997668516 ) ) ;
#65984=CARTESIAN_POINT ( 'NONE',  ( -10.81513955013129902, 1470.571292273900099, 210.8385438386609962 ) ) ;
#65985=CARTESIAN_POINT ( 'NONE',  ( 4.327308595631699895, 1515.146523075020013, 208.6641484814759906 ) ) ;
#65988=ORIENTED_EDGE ( 'NONE', *, *, #65812, .T. ) ;
#65989=CARTESIAN_POINT ( 'NONE',  ( 10.53557798318139938, 1481.859448200410043, 210.2581152848169950 ) ) ;
#65995=EDGE_CURVE ( 'NONE', #53764, #3178, #97222, .T. ) ;
#65998=CARTESIAN_POINT ( 'NONE',  ( -1.995807793896930082, 1508.551704408389924, 220.0704850252740243 ) ) ;
#66002=CARTESIAN_POINT ( 'NONE',  ( -12.12616446094680001, 1502.349690982020093, 208.9415299542270077 ) ) ;
#66003=CARTESIAN_POINT ( 'NONE',  ( 10.86502470147939903, 1490.656646050969812, 210.7146857633749732 ) ) ;
#66004=CARTESIAN_POINT ( 'NONE',  ( 0.4663913465019989824, 1455.963574820090116, 218.7208018874689799 ) ) ;
#66008=CARTESIAN_POINT ( 'NONE',  ( -3.076050021859999983, 1475.159716099690058, 198.5224445511989870 ) ) ;
#66012=CARTESIAN_POINT ( 'NONE',  ( -4.259777688362290426, 1515.374151772610048, 206.1850293956469784 ) ) ;
#66014=CARTESIAN_POINT ( 'NONE',  ( -9.234136244889999290, 1461.205488667689906, 206.1827751366290045 ) ) ;
#66017=CARTESIAN_POINT ( 'NONE',  ( -13.01051159769479959, 1508.551704408389924, 216.5695640764339771 ) ) ;
#66020=CARTESIAN_POINT ( 'NONE',  ( -1.862709314156860030, 1485.677233011570252, 197.3688579391329938 ) ) ;
#66029=CIRCLE ( 'NONE', #28443, 0.5000016051842596232 ) ;
#66032=CARTESIAN_POINT ( 'NONE',  ( -15.09297716350000051, 1420.200853339370269, 212.5836862043790063 ) ) ;
#66039=CARTESIAN_POINT ( 'NONE',  ( -10.22078022364619976, 1448.827725899079724, 207.2905427559460065 ) ) ;
#66044=CARTESIAN_POINT ( 'NONE',  ( 7.455126725186649317, 1425.226345695840109, 212.3390874243399935 ) ) ;
#66049=CARTESIAN_POINT ( 'NONE',  ( 0.5086982323670009576, 1417.713718859019764, 204.0301965041890071 ) ) ;
#66054=CARTESIAN_POINT ( 'NONE',  ( -4.640277423280045888, 1378.166137044523111, 214.4725589679636641 ) ) ;
#66058=VERTEX_POINT ( 'NONE', #7495 ) ;
#66061=PLANE ( 'NONE',  #22137 ) ;
#66062=CARTESIAN_POINT ( 'NONE',  ( 11.10442532319999920, 1501.746131285089859, 206.2421527516889626 ) ) ;
#66075=CARTESIAN_POINT ( 'NONE',  ( -5.731568358319999668, 1428.367353358390119, 203.0107280175789981 ) ) ;
#66081=ORIENTED_EDGE ( 'NONE', *, *, #36574, .F. ) ;
#66082=CARTESIAN_POINT ( 'NONE',  ( -10.55763132505339996, 1480.395020916429985, 210.7122116074530140 ) ) ;
#66088=CARTESIAN_POINT ( 'NONE',  ( 7.423896801969999792, 1422.288457550600015, 195.6224997975990334 ) ) ;
#66089=CARTESIAN_POINT ( 'NONE',  ( -0.1950599852922330069, 1431.910904562789938, 218.6163528922420198 ) ) ;
#66090=B_SPLINE_SURFACE_WITH_KNOTS ( 'NONE', 5, 1, ( 
 ( #60856, #18800 ),
 ( #8196, #34516 ),
 ( #77089, #52445 ),
 ( #85450, #26657 ),
 ( #44033, #8748 ),
 ( #52996, #68155 ) ),
 .UNSPECIFIED., .F., .F., .F.,
 ( 6, 6 ),
 ( 2, 2 ),
 ( -8.364788202518770371E-05, 17.30286250248200020 ),
 ( 0.000000000000000000, 14.00008364788200055 ),
 .UNSPECIFIED. ) ;
#66091=CARTESIAN_POINT ( 'NONE',  ( -9.389251474311459233, 1493.203009381459879, 201.1804961733769801 ) ) ;
#66092=CARTESIAN_POINT ( 'NONE',  ( 10.29233424086269899, 1479.549769955249985, 205.9985512849049769 ) ) ;
#66096=CARTESIAN_POINT ( 'NONE',  ( 10.86483302107700055, 1425.362906770059908, 206.5122574745630004 ) ) ;
#66108=CARTESIAN_POINT ( 'NONE',  ( 10.31893549361520002, 1422.402437340219876, 211.7674958658010098 ) ) ;
#66110=CARTESIAN_POINT ( 'NONE',  ( 12.02395472744730043, 1421.496668670510189, 203.4303483181410002 ) ) ;
#66114=CARTESIAN_POINT ( 'NONE',  ( -8.079136863727587325, 1477.137875895455636, 215.6487954345820128 ) ) ;
#66122=CARTESIAN_POINT ( 'NONE',  ( 0.000000000000000000, 1397.913060387289988, 209.1218459616989946 ) ) ;
#66124=CARTESIAN_POINT ( 'NONE',  ( 3.955903661833950036, 1474.305422501160137, 219.8349303349459944 ) ) ;
#66126=EDGE_CURVE ( 'NONE', #23318, #36047, #39709, .T. ) ;
#66132=CARTESIAN_POINT ( 'NONE',  ( 12.70077814543349959, 1426.512147001669973, 202.9361290949429986 ) ) ;
#66133=CARTESIAN_POINT ( 'NONE',  ( -19.86622903098490056, 1443.388331107859813, 213.1207024752020232 ) ) ;
#66137=CARTESIAN_POINT ( 'NONE',  ( 8.769621322867079627, 1467.226126602908835, 204.3312691679350905 ) ) ;
#66143=CARTESIAN_POINT ( 'NONE',  ( -2.594026038730000039, 1450.364277435190161, 190.1050478246989996 ) ) ;
#66149=CARTESIAN_POINT ( 'NONE',  ( 1.877783507969999821, 1464.338560063190016, 202.3121933697890142 ) ) ;
#66158=CARTESIAN_POINT ( 'NONE',  ( -4.987078423031819696, 1508.551704408389924, 206.6198795153389938 ) ) ;
#66162=CARTESIAN_POINT ( 'NONE',  ( 2.980039776149999931, 1507.572950449990003, 217.5187685084390239 ) ) ;
#66164=CARTESIAN_POINT ( 'NONE',  ( 4.322866002579999645, 1473.654522927490007, 218.8408954872590186 ) ) ;
#66165=CARTESIAN_POINT ( 'NONE',  ( 10.21480549290979845, 1470.289156061989843, 209.7505692248130060 ) ) ;
#66178=B_SPLINE_CURVE_WITH_KNOTS ( 'NONE', 3,
 ( #77268, #8935, #15653, #25169, #92381, #101318, #51502, #7832, #42546, #10, #566, #85086, #33573, #49858, #35249, #94590, #50959, #59373, #110297, #102437, #17869 ),
 .UNSPECIFIED., .F., .F.,
 ( 4, 2, 1, 1, 1, 2, 2, 2, 1, 1, 2, 2, 4 ),
 ( 0.000000000000000000, 0.1250000000002345901, 0.1875000000003518852, 0.2187500000004230782, 0.2343750000004451162, 0.2421875000004429790, 0.2500000000004408141, 0.3750000000004406475, 0.4375000000004405365, 0.4687500000004408696, 0.4843750000004405920, 0.5000000000004402034, 1.000000000000000000 ),
 .UNSPECIFIED. ) ;
#66181=CARTESIAN_POINT ( 'NONE',  ( -2.031883580139580037, 1464.998375551469962, 198.3053770173009980 ) ) ;
#66185=ORIENTED_EDGE ( 'NONE', *, *, #63363, .F. ) ;
#66197=CARTESIAN_POINT ( 'NONE',  ( 12.68863146979170153, 1500.713416596689967, 209.8116292722930041 ) ) ;
#66200=B_SPLINE_CURVE_WITH_KNOTS ( 'NONE', 3,
 ( #86234, #85125, #60509, #70575 ),
 .UNSPECIFIED., .F., .F.,
 ( 4, 4 ),
 ( 0.000000000000000000, 1.000000000000000000 ),
 .UNSPECIFIED. ) ;
#66202=CARTESIAN_POINT ( 'NONE',  ( -12.04602610249999906, 1481.198043686990104, 227.9689298191989622 ) ) ;
#66204=CARTESIAN_POINT ( 'NONE',  ( -3.994937574034520100, 1430.106198372560129, 201.8091617894969829 ) ) ;
#66207=DIRECTION ( 'NONE',  ( 0.000000000000000000, 1.000000000000000000, -1.836970198721029688E-16 ) ) ;
#66210=CARTESIAN_POINT ( 'NONE',  ( -20.35522600081170097, 1508.452240834250006, 209.8847156256999824 ) ) ;
#66213=CARTESIAN_POINT ( 'NONE',  ( 4.324479010949999314, 1515.254596385190098, 209.8453191605230188 ) ) ;
#66231=CARTESIAN_POINT ( 'NONE',  ( -9.234024398008379819, 1461.205035371770009, 206.1824885990050120 ) ) ;
#66233=CARTESIAN_POINT ( 'NONE',  ( 10.28237718578049886, 1469.669003181509879, 207.2474476084789785 ) ) ;
#66234=CARTESIAN_POINT ( 'NONE',  ( -8.233416563630001406, 1473.844808855489873, 202.6267445639990115 ) ) ;
#66248=CARTESIAN_POINT ( 'NONE',  ( 3.912777227685470205, 1515.493283046529996, 212.5869276274669915 ) ) ;
#66254=CARTESIAN_POINT ( 'NONE',  ( 2.727892099239999979, 1508.551704408389924, 219.8158444027990015 ) ) ;
#66270=CARTESIAN_POINT ( 'NONE',  ( 10.82854844483479972, 1489.698305903909841, 207.5992399318249966 ) ) ;
#66280=CARTESIAN_POINT ( 'NONE',  ( -8.631581796184160993, 1437.055567594220065, 209.4405929349389908 ) ) ;
#66281=FACE_OUTER_BOUND ( 'NONE', #85918, .T. ) ;
#66300=ORIENTED_EDGE ( 'NONE', *, *, #44902, .F. ) ;
#66302=CARTESIAN_POINT ( 'NONE',  ( -13.59488878742559947, 1507.788032636909975, 209.3690985338880068 ) ) ;
#66303=CARTESIAN_POINT ( 'NONE',  ( -19.34950487613039627, 1446.106571107670106, 200.0047943255200096 ) ) ;
#66314=CARTESIAN_POINT ( 'NONE',  ( -19.96805577914620144, 1418.682940182010043, 207.2801514309879849 ) ) ;
#66319=ORIENTED_EDGE ( 'NONE', *, *, #70627, .T. ) ;
#66327=CARTESIAN_POINT ( 'NONE',  ( 0.2941023281940010059, 1444.784487645989884, 199.4356807887090213 ) ) ;
#66331=CARTESIAN_POINT ( 'NONE',  ( -4.885459850415359462, 1463.524421287130053, 200.4816849840370026 ) ) ;
#66340=EDGE_LOOP ( 'NONE', ( #35549, #90487, #12179, #84633 ) ) ;
#66348=CARTESIAN_POINT ( 'NONE',  ( -11.34379066580000028, 1503.466875535689951, 207.0254393924689964 ) ) ;
#66353=ORIENTED_EDGE ( 'NONE', *, *, #9946, .F. ) ;
#66363=CARTESIAN_POINT ( 'NONE',  ( -14.42498423343375791, 1415.918606729107523, 214.3962734341573366 ) ) ;
#66369=CARTESIAN_POINT ( 'NONE',  ( 3.039942922830000338, 1441.350710123290128, 218.5632362648489959 ) ) ;
#66377=ORIENTED_EDGE ( 'NONE', *, *, #20676, .F. ) ;
#66382=CARTESIAN_POINT ( 'NONE',  ( 0.3578367916707796414, 1494.301120918491051, 220.2517076097725806 ) ) ;
#66383=CARTESIAN_POINT ( 'NONE',  ( 7.885640402109895142, 1473.211498812089985, 217.4524272520788486 ) ) ;
#66385=CARTESIAN_POINT ( 'NONE',  ( 1.744489195120649150, 1498.886263367861602, 197.9188166206191113 ) ) ;
#66395=CARTESIAN_POINT ( 'NONE',  ( 10.78248285070100110, 1461.894572756529897, 211.1626650880500051 ) ) ;
#66396=CARTESIAN_POINT ( 'NONE',  ( -7.727640881871497669, 1461.842851176162412, 203.2269185635026076 ) ) ;
#66397=CARTESIAN_POINT ( 'NONE',  ( -1.466944312100000092, 1443.753574183790079, 218.3055266773990013 ) ) ;
#66402=CARTESIAN_POINT ( 'NONE',  ( 9.275324149480784541, 1488.103561708918050, 203.3811522517966068 ) ) ;
#66417=CARTESIAN_POINT ( 'NONE',  ( 2.236820334746699945, 1495.676459233159903, 221.2569916761739819 ) ) ;
#66421=CARTESIAN_POINT ( 'NONE',  ( -9.659635694953360385, 1460.543239006349950, 208.9236336851400040 ) ) ;
#66428=ORIENTED_EDGE ( 'NONE', *, *, #68530, .F. ) ;
#66432=CARTESIAN_POINT ( 'NONE',  ( 4.573885314059999985, 1455.617763203289996, 218.2506144138390027 ) ) ;
#66434=CARTESIAN_POINT ( 'NONE',  ( -3.499767445780000319, 1444.082658218989764, 218.1757574250489995 ) ) ;
#66436=CARTESIAN_POINT ( 'NONE',  ( -4.487357219411578946, 1509.034509700538365, 212.2379894419900381 ) ) ;
#66438=CARTESIAN_POINT ( 'NONE',  ( 7.190134108680000580, 1424.106784181189823, 213.0072132442990096 ) ) ;
#66451=CARTESIAN_POINT ( 'NONE',  ( -21.43713612259999834, 1507.398797767890073, 216.2026692569289992 ) ) ;
#66453=CARTESIAN_POINT ( 'NONE',  ( -2.338275166668102756, 1474.327831861476170, 219.1154912885318709 ) ) ;
#66456=EDGE_CURVE ( 'NONE', #6446, #77864, #99785, .T. ) ;
#66461=EDGE_CURVE ( 'NONE', #43603, #15017, #94416, .T. ) ;
#66463=CARTESIAN_POINT ( 'NONE',  ( -4.468118146560000170, 1458.475370017489922, 218.8772509106790096 ) ) ;
#66466=ORIENTED_EDGE ( 'NONE', *, *, #41772, .T. ) ;
#66467=CARTESIAN_POINT ( 'NONE',  ( -4.327620191588679610, 1515.134623705510194, 209.7786229697130125 ) ) ;
#66469=ORIENTED_EDGE ( 'NONE', *, *, #77703, .F. ) ;
#66483=CARTESIAN_POINT ( 'NONE',  ( 9.877435263969999824, 1471.593449360889963, 212.9802648889690033 ) ) ;
#66490=ORIENTED_EDGE ( 'NONE', *, *, #46868, .F. ) ;
#66502=CARTESIAN_POINT ( 'NONE',  ( 4.010670133484330435, 1440.993182668509917, 217.7599716824630036 ) ) ;
#66507=CARTESIAN_POINT ( 'NONE',  ( -8.663672900706190561, 1438.058509006810027, 208.5115941168539848 ) ) ;
#66517=CARTESIAN_POINT ( 'NONE',  ( 4.747050408260000687, 1486.851065980389876, 199.2547198969290037 ) ) ;
#66518=CARTESIAN_POINT ( 'NONE',  ( -3.269259737218870310, 1476.740802116999930, 199.2818558394819775 ) ) ;
#66520=CARTESIAN_POINT ( 'NONE',  ( -1.842963787330039960, 1515.551704393028331, 205.1635077660893387 ) ) ;
#66523=ORIENTED_EDGE ( 'NONE', *, *, #7521, .T. ) ;
#66527=CARTESIAN_POINT ( 'NONE',  ( -0.2610938271800009591, 1474.054394607790073, 219.3955652254989843 ) ) ;
#66529=CARTESIAN_POINT ( 'NONE',  ( -11.18513414810809969, 1471.346656141509811, 206.8404382864960098 ) ) ;
#66532=CARTESIAN_POINT ( 'NONE',  ( 0.3799711347515690174, 1455.871197009739944, 198.5797350333110103 ) ) ;
#66535=CARTESIAN_POINT ( 'NONE',  ( -10.10799952816689995, 1471.968561594289895, 210.1976632032360044 ) ) ;
#66537=CARTESIAN_POINT ( 'NONE',  ( -3.179847367899999888, 1481.779546599790137, 229.4457135908990040 ) ) ;
#66540=CARTESIAN_POINT ( 'NONE',  ( 10.47512669263509899, 1482.041014330849976, 210.7459474806360049 ) ) ;
#66544=CARTESIAN_POINT ( 'NONE',  ( -3.061334144399999957, 1442.717432058590020, 200.6190578008389878 ) ) ;
#66547=CARTESIAN_POINT ( 'NONE',  ( 207.7471169361000136, -8387.357407334289746, -1761.517333167069864 ) ) ;
#66549=CARTESIAN_POINT ( 'NONE',  ( -1.561041872522580087, 1508.551704408389924, 220.0816520586899969 ) ) ;
#66552=CARTESIAN_POINT ( 'NONE',  ( -4.678143775780629454, 1508.611354794059935, 206.6339233318589947 ) ) ;
#66555=CARTESIAN_POINT ( 'NONE',  ( 10.82590729831830068, 1491.268289583239948, 211.1351721366039840 ) ) ;
#66556=CARTESIAN_POINT ( 'NONE',  ( -11.16717556649999921, 1414.661898229710005, 212.7267128011690147 ) ) ;
#66557=ORIENTED_EDGE ( 'NONE', *, *, #46707, .T. ) ;
#66560=ADVANCED_FACE ( 'NONE', ( #7161 ), #47394, .F. ) ;
#66562=CARTESIAN_POINT ( 'NONE',  ( 4.889439660094519802, 1508.551704408389924, 205.9425365203790079 ) ) ;
#66570=CARTESIAN_POINT ( 'NONE',  ( -9.457585828349998280, 1462.148799080189974, 206.2711936052490103 ) ) ;
#66572=CARTESIAN_POINT ( 'NONE',  ( 2.765840199879999961, 1444.819550273290133, 203.5022050372989781 ) ) ;
#66573=CARTESIAN_POINT ( 'NONE',  ( -9.088471267427010503, 1508.551704408389924, 218.6183512830809832 ) ) ;
#66577=CARTESIAN_POINT ( 'NONE',  ( 7.311196690888119853, 1433.969857655230044, 203.9080805087000101 ) ) ;
#66593=DIRECTION ( 'NONE',  ( -1.000000000000000000, 0.000000000000000000, 0.000000000000000000 ) ) ;
#66595=CARTESIAN_POINT ( 'NONE',  ( -7.969533265219999940, 1425.156681655810189, 206.0885952228989879 ) ) ;
#66600=CARTESIAN_POINT ( 'NONE',  ( 7.457299212086079265, 1425.231075921110005, 212.3345666727680054 ) ) ;
#66606=CARTESIAN_POINT ( 'NONE',  ( -6.338357687459999390, 1461.235457266589947, 207.8854984423689984 ) ) ;
#66611=EDGE_LOOP ( 'NONE', ( #7484, #107275, #94835, #33923 ) ) ;
#66615=CARTESIAN_POINT ( 'NONE',  ( 10.14394188820000053, 1461.870444916690076, 209.6790091569899914 ) ) ;
#66626=CARTESIAN_POINT ( 'NONE',  ( 3.747941686733399891, 1508.879013277289914, 213.3683127840300244 ) ) ;
#66635=CARTESIAN_POINT ( 'NONE',  ( 17.69622990075129820, 1430.679836004809886, 213.5595397380919849 ) ) ;
#66636=ORIENTED_EDGE ( 'NONE', *, *, #18001, .T. ) ;
#66641=CARTESIAN_POINT ( 'NONE',  ( 7.474305816439999361, 1422.145197690320174, 195.6519535563990075 ) ) ;
#66643=CARTESIAN_POINT ( 'NONE',  ( -5.094674989349999628, 1496.284763139690085, 199.1200413041989918 ) ) ;
#66647=CARTESIAN_POINT ( 'NONE',  ( 10.68158499005449968, 1423.994661768180094, 206.6794003566110121 ) ) ;
#66655=CARTESIAN_POINT ( 'NONE',  ( 9.784730986437239153, 1426.272936423899864, 209.3148760698660169 ) ) ;
#66656=CARTESIAN_POINT ( 'NONE',  ( 11.35995302351660108, 1425.310403992989905, 202.9730432884799995 ) ) ;
#66666=CARTESIAN_POINT ( 'NONE',  ( 5.275783403443830899, 1466.070747001820109, 217.9942205468059910 ) ) ;
#66672=CARTESIAN_POINT ( 'NONE',  ( -0.2024664826940029971, 1479.235308103189936, 229.5453557735989989 ) ) ;
#66676=CARTESIAN_POINT ( 'NONE',  ( 3.217370148928750062, 1424.184623195729955, 188.9579834054289904 ) ) ;
#66680=ORIENTED_EDGE ( 'NONE', *, *, #32316, .F. ) ;
#66683=CARTESIAN_POINT ( 'NONE',  ( -15.17700602440057622, 1445.095295946591477, 196.7536451946974410 ) ) ;
#66688=CARTESIAN_POINT ( 'NONE',  ( -0.5111327314519990006, 1484.634848108790038, 198.3940791051990118 ) ) ;
#66689=CARTESIAN_POINT ( 'NONE',  ( 9.831955598149999531, 1479.326580839289818, 204.9319913846790087 ) ) ;
#66693=FACE_OUTER_BOUND ( 'NONE', #46760, .T. ) ;
#66695=CARTESIAN_POINT ( 'NONE',  ( -16.96581893389999962, 1420.808731266319910, 208.6966097274290064 ) ) ;
#66700=CARTESIAN_POINT ( 'NONE',  ( 11.73186578479040065, 1421.919406218840095, 207.6102233476609911 ) ) ;
#66706=CARTESIAN_POINT ( 'NONE',  ( 10.51937569161310115, 1470.762630565469863, 209.9255540597749814 ) ) ;
#66711=B_SPLINE_CURVE_WITH_KNOTS ( 'NONE', 5,
 ( #11820, #15506, #7136, #14412, #31228, #20746 ),
 .UNSPECIFIED., .F., .F.,
 ( 6, 6 ),
 ( 0.000000000000000000, 3.472809815250000209 ),
 .UNSPECIFIED. ) ;
#66717=CARTESIAN_POINT ( 'NONE',  ( 9.549998141239999683, 1451.222071590189898, 207.5451647913689897 ) ) ;
#66719=ADVANCED_FACE ( 'NONE', ( #97774 ), #107285, .T. ) ;
#66722=CARTESIAN_POINT ( 'NONE',  ( -2.514213374330000139, 1455.572514118689924, 199.8771817507590072 ) ) ;
#66726=ORIENTED_EDGE ( 'NONE', *, *, #17858, .T. ) ;
#66731=EDGE_CURVE ( 'NONE', #73174, #100464, #77000, .T. ) ;
#66735=CARTESIAN_POINT ( 'NONE',  ( 12.20582139389999909, 1500.450892145889839, 208.0634134494790146 ) ) ;
#66744=B_SPLINE_CURVE_WITH_KNOTS ( 'NONE', 3,
 ( #28871, #96626, #105022, #63065, #72533, #106124, #11519, #29399, #63600, #64147, #98266, #46247, #88777, #97718, #12615, #19336, #55749, #10965, #44570 ),
 .UNSPECIFIED., .F., .F.,
 ( 4, 3, 3, 3, 3, 3, 4 ),
 ( -7.661770161623569386, -7.428136132220500620, -6.292251436735150527, -5.400505869387740354, -4.641385543154090243, -3.845608395895360410, -3.139241426659999945 ),
 .UNSPECIFIED. ) ;
#66748=CARTESIAN_POINT ( 'NONE',  ( 22.14279730899999876, 1473.984189751590065, 210.1089390466149780 ) ) ;
#66749=EDGE_CURVE ( 'NONE', #102658, #1876, #2687, .T. ) ;
#66754=CARTESIAN_POINT ( 'NONE',  ( 10.42657513622150134, 1453.119160424219899, 211.0495624056229929 ) ) ;
#66756=CARTESIAN_POINT ( 'NONE',  ( -18.43454007138939943, 1507.986789759319890, 209.4721884240840097 ) ) ;
#66768=( BOUNDED_CURVE ( )  B_SPLINE_CURVE ( 3, ( #101855, #110827, #17842, #7270 ),
 .UNSPECIFIED., .F., .T. ) 
 B_SPLINE_CURVE_WITH_KNOTS ( ( 4, 4 ),
 ( 1.007411674165658022, 2.134181044723490128 ),
 .UNSPECIFIED. ) 
 CURVE ( )  GEOMETRIC_REPRESENTATION_ITEM ( )  RATIONAL_B_SPLINE_CURVE ( ( 1.000000000000000000, 0.8969682421527426230, 0.8969682421527426230, 1.000000000000000000 ) ) 
 REPRESENTATION_ITEM ( '' )  );
#66776=CARTESIAN_POINT ( 'NONE',  ( 6.360756793238519613, 1429.512739015589887, 216.1615566237340147 ) ) ;
#66777=CARTESIAN_POINT ( 'NONE',  ( -18.44377863300000087, 1443.022878208090106, 205.4489113795289938 ) ) ;
#66786=CARTESIAN_POINT ( 'NONE',  ( 19.55988977460000200, 1474.636381753090063, 214.0184790771390055 ) ) ;
#66793=CARTESIAN_POINT ( 'NONE',  ( 2.898099067781010341, 1515.492902831140100, 213.2585957832889960 ) ) ;
#66795=CARTESIAN_POINT ( 'NONE',  ( -11.77310042539119905, 1501.438875975280098, 211.3558264699879885 ) ) ;
#66798=CARTESIAN_POINT ( 'NONE',  ( -0.9646231412680019712, 1508.481254761890114, 220.5684046465989923 ) ) ;
#66800=CARTESIAN_POINT ( 'NONE',  ( -2.916739703929999816, 1436.466740336890098, 227.4199358109989930 ) ) ;
#66801=CARTESIAN_POINT ( 'NONE',  ( -5.823377452736959725, 1441.464471037789963, 202.2443272568390000 ) ) ;
#66803=CARTESIAN_POINT ( 'NONE',  ( 20.93524908849999733, 1496.483007425989854, 206.0866933769390243 ) ) ;
#66806=CARTESIAN_POINT ( 'NONE',  ( -10.25236302078530137, 1481.942182559430194, 205.9183910829460160 ) ) ;
#66808=ORIENTED_EDGE ( 'NONE', *, *, #17166, .F. ) ;
#66815=CARTESIAN_POINT ( 'NONE',  ( 1.890874494093850000, 1454.654138192250002, 218.3350682022239937 ) ) ;
#66818=CARTESIAN_POINT ( 'NONE',  ( -16.64004004550000104, 1417.307962343580130, 206.7231940078289938 ) ) ;
#66835=CARTESIAN_POINT ( 'NONE',  ( 4.326992699989999913, 1515.158586642889986, 208.7649733894699864 ) ) ;
#66836=CARTESIAN_POINT ( 'NONE',  ( -2.244413514002144616, 1507.820143033591194, 221.0491532391985743 ) ) ;
#66844=CARTESIAN_POINT ( 'NONE',  ( -19.22849213419559788, 1445.326212981899971, 199.8420603585589959 ) ) ;
#66846=CARTESIAN_POINT ( 'NONE',  ( -8.229007828222330900, 1439.448142495530192, 228.6152152553840153 ) ) ;
#66872=CARTESIAN_POINT ( 'NONE',  ( 0.4875494646660009646, 1444.157371980789776, 200.0448216578990071 ) ) ;
#66875=CARTESIAN_POINT ( 'NONE',  ( -3.165749237226819890, 1462.941186258239895, 199.8678155363639917 ) ) ;
#66878=CARTESIAN_POINT ( 'NONE',  ( 2.564080272660000048, 1443.257105148589972, 214.7475389528890162 ) ) ;
#66891=CARTESIAN_POINT ( 'NONE',  ( -19.50318791720000178, 1467.690391532990134, 205.2505305201189856 ) ) ;
#66894=CARTESIAN_POINT ( 'NONE',  ( -12.57798105409999856, 1503.242005039890046, 208.6149048402859876 ) ) ;
#66897=ADVANCED_FACE ( 'NONE', ( #86488 ), #51801, .T. ) ;
#66898=EDGE_LOOP ( 'NONE', ( #107973, #109165, #18536, #5058 ) ) ;
#66910=FACE_OUTER_BOUND ( 'NONE', #37533, .T. ) ;
#66915=CARTESIAN_POINT ( 'NONE',  ( 2.032300221149999864, 1441.827160225690022, 218.8459470114090379 ) ) ;
#66922=EDGE_LOOP ( 'NONE', ( #26477, #107646, #56873, #66081 ) ) ;
#66927=CARTESIAN_POINT ( 'NONE',  ( 9.058637367069879431, 1472.814398557088680, 216.2138489941888508 ) ) ;
#66928=CARTESIAN_POINT ( 'NONE',  ( -15.96075179420000367, 1466.903945902690111, 196.1521398069990312 ) ) ;
#66931=B_SPLINE_CURVE_WITH_KNOTS ( 'NONE', 3,
 ( #18158, #102699, #25993, #103835, #87029, #10319, #78637, #1953, #51223, #103254, #36090, #27683, #102161, #25443, #59637, #85927, #42828, #60191, #94310, #15736, #91926, #6812 ),
 .UNSPECIFIED., .F., .F.,
 ( 4, 2, 1, 1, 2, 2, 2, 2, 1, 1, 2, 2, 4 ),
 ( 0.000000000000000000, 0.1250000000002231271, 0.1875000000003487211, 0.2187500000003965162, 0.2343750000004201361, 0.2500000000004437561, 0.5000000000003356204, 0.6250000000002815526, 0.6875000000002354783, 0.7187500000001927347, 0.7343750000001930678, 0.7500000000001934009, 1.000000000000000000 ),
 .UNSPECIFIED. ) ;
#66934=CARTESIAN_POINT ( 'NONE',  ( -9.544534124909469952, 1448.313337447510094, 209.6434600324809878 ) ) ;
#66941=CARTESIAN_POINT ( 'NONE',  ( 10.95069398041579944, 1461.279514859859773, 209.5869465053850149 ) ) ;
#66943=CARTESIAN_POINT ( 'NONE',  ( -1.003913049989999973, 1443.013031698689929, 219.0745052372589896 ) ) ;
#66955=CARTESIAN_POINT ( 'NONE',  ( -8.697262469415090180, 1440.006290268419889, 206.1600271334220054 ) ) ;
#66962=CARTESIAN_POINT ( 'NONE',  ( -3.542321145578850139, 1515.375307573260216, 213.1422533703459976 ) ) ;
#66972=ORIENTED_EDGE ( 'NONE', *, *, #3817, .F. ) ;
#66973=CARTESIAN_POINT ( 'NONE',  ( -11.61029367559999947, 1501.887990983090049, 208.8313354872300067 ) ) ;
#66977=CARTESIAN_POINT ( 'NONE',  ( -3.129785590100000015, 1444.786455221890037, 217.7016765222190031 ) ) ;
#66981=CARTESIAN_POINT ( 'NONE',  ( 7.616741216099999434, 1423.421902274779995, 213.1545376211790028 ) ) ;
#66988=ORIENTED_EDGE ( 'NONE', *, *, #19245, .F. ) ;
#66992=CARTESIAN_POINT ( 'NONE',  ( 13.52266831577220074, 1497.923527929759985, 227.8730120457710200 ) ) ;
#66994=CARTESIAN_POINT ( 'NONE',  ( 0.2136372107412991272, 1473.445861986991986, 219.3446630527206480 ) ) ;
#66998=CARTESIAN_POINT ( 'NONE',  ( -7.260870878720000476, 1480.575647549590030, 208.3277293783959863 ) ) ;
#67004=CARTESIAN_POINT ( 'NONE',  ( -8.912705131193250807, 1448.592310648610010, 211.1800892463350010 ) ) ;
#67008=CARTESIAN_POINT ( 'NONE',  ( -4.329415431089000066, 1515.066066275049934, 210.8307989536980074 ) ) ;
#67014=CARTESIAN_POINT ( 'NONE',  ( 8.586756624946868754, 1425.130607248830074, 194.8120923273959875 ) ) ;
#67031=EDGE_LOOP ( 'NONE', ( #54919, #8236, #30970, #6804 ) ) ;
#67032=CARTESIAN_POINT ( 'NONE',  ( 9.651063919191019025, 1425.440657924460083, 195.4941620015079877 ) ) ;
#67041=CARTESIAN_POINT ( 'NONE',  ( 7.097314899640720043, 1439.093628026630086, 216.1530160518380228 ) ) ;
#67047=CARTESIAN_POINT ( 'NONE',  ( -8.650219412924689877, 1438.157521317829833, 208.3097233004990017 ) ) ;
#67050=CARTESIAN_POINT ( 'NONE',  ( 19.64599270300000100, 1476.662575758389949, 214.0395835971089866 ) ) ;
#67054=CARTESIAN_POINT ( 'NONE',  ( -14.92733988109999999, 1416.530231069960109, 207.6074944693189934 ) ) ;
#67056=CARTESIAN_POINT ( 'NONE',  ( 6.223729794970000562, 1487.458568572190188, 200.0625369783790006 ) ) ;
#67060=CARTESIAN_POINT ( 'NONE',  ( -17.97880235851549457, 1445.573137004940918, 203.2555883697691286 ) ) ;
#67065=CARTESIAN_POINT ( 'NONE',  ( -17.06299074029999829, 1420.289561323179896, 203.8301379063090337 ) ) ;
#67069=CARTESIAN_POINT ( 'NONE',  ( -0.1492209459390009818, 1474.475942019490049, 219.5409241924989772 ) ) ;
#67072=CARTESIAN_POINT ( 'NONE',  ( -0.08180352518808278739, 1423.482083046089883, 191.1879846049409934 ) ) ;
#67073=CARTESIAN_POINT ( 'NONE',  ( -11.38946577428759888, 1470.924613609000062, 208.4453646624949954 ) ) ;
#67074=CARTESIAN_POINT ( 'NONE',  ( -5.309623260221089325, 1508.254033944475623, 220.3333518336809504 ) ) ;
#67076=ADVANCED_FACE ( 'NONE', ( #79768 ), #56346, .T. ) ;
#67081=CARTESIAN_POINT ( 'NONE',  ( -15.23238439385559850, 1418.498828849909842, 202.0312086372670137 ) ) ;
#67082=CARTESIAN_POINT ( 'NONE',  ( -0.8685429202199980159, 1491.841791262990000, 188.0762365942990186 ) ) ;
#67091=CARTESIAN_POINT ( 'NONE',  ( 740.1067240283520050, 11216.44053380570222, 2045.284428720447750 ) ) ;
#67098=CARTESIAN_POINT ( 'NONE',  ( 11.42677157140140132, 1491.914064927579830, 210.1973818834709959 ) ) ;
#67099=CARTESIAN_POINT ( 'NONE',  ( 1.660746386170000033, 1456.055583820689890, 218.8271601458489783 ) ) ;
#67104=CARTESIAN_POINT ( 'NONE',  ( 8.506705275679738776, 1436.886745436839874, 207.6663867986219998 ) ) ;
#67108=CARTESIAN_POINT ( 'NONE',  ( -3.644352556202699933, 1515.551704204679936, 205.8496992207700202 ) ) ;
#67111=CARTESIAN_POINT ( 'NONE',  ( -6.040927710290000086, 1463.272537550489915, 201.2370028249389975 ) ) ;
#67113=CARTESIAN_POINT ( 'NONE',  ( 2.236830499889160162, 1495.676457076940096, 221.2569898194790028 ) ) ;
#67115=CARTESIAN_POINT ( 'NONE',  ( -15.49290351828469881, 1508.551704408389924, 214.3946075353640026 ) ) ;
#67118=CARTESIAN_POINT ( 'NONE',  ( 3.256906394843720243, 1487.066025393580048, 197.6188337626330167 ) ) ;
#67128=CARTESIAN_POINT ( 'NONE',  ( -13.31089767776890120, 1503.456584347970193, 208.6977459380580058 ) ) ;
#67131=CARTESIAN_POINT ( 'NONE',  ( 2.115055685359999771, 1476.785742987490039, 198.5761133807990007 ) ) ;
#67137=CARTESIAN_POINT ( 'NONE',  ( 0.8644693283286819518, 1429.652419925939967, 217.3904187270329942 ) ) ;
#67138=CARTESIAN_POINT ( 'NONE',  ( -8.477967594009999885, 1424.852341466620146, 205.3179503978689979 ) ) ;
#67142=CARTESIAN_POINT ( 'NONE',  ( 4.329448776040000446, 1515.064792882589927, 206.7917118356089929 ) ) ;
#67143=CARTESIAN_POINT ( 'NONE',  ( 7.405955376734920215, 1426.244457028639999, 212.5578732180090071 ) ) ;
#67147=CARTESIAN_POINT ( 'NONE',  ( -11.21869170107060043, 1491.835551150570154, 206.9930840995259871 ) ) ;
#67149=CARTESIAN_POINT ( 'NONE',  ( -1.748905610829809998, 1488.269106374019884, 219.8524659745219765 ) ) ;
#67151=CARTESIAN_POINT ( 'NONE',  ( -1.640992637469999904, 1486.309234237589862, 220.9425018421990217 ) ) ;
#67156=DIRECTION ( 'NONE',  ( 0.000000000000000000, 1.000000000000000000, -1.836970198721029688E-16 ) ) ;
#67157=CARTESIAN_POINT ( 'NONE',  ( 9.728472712500000341, 1463.031710894390017, 210.0816964760090002 ) ) ;
#67180=CARTESIAN_POINT ( 'NONE',  ( -4.984765438550020633, 1508.551704408389924, 211.7339477409330186 ) ) ;
#67182=CARTESIAN_POINT ( 'NONE',  ( 7.477592609290000247, 1422.768710552009907, 195.6698503542990011 ) ) ;
#67183=CARTESIAN_POINT ( 'NONE',  ( -1.447235060822049890, 1432.423094547480105, 218.5251106399929881 ) ) ;
#67184=CARTESIAN_POINT ( 'NONE',  ( 10.70780782887229954, 1479.022113073340051, 205.9701340518660118 ) ) ;
#67188=CARTESIAN_POINT ( 'NONE',  ( 11.50132634430500111, 1426.392275987999938, 206.5139615940070144 ) ) ;
#67199=CARTESIAN_POINT ( 'NONE',  ( 11.19200130296239948, 1422.145316461549783, 210.4507779064919930 ) ) ;
#67200=CARTESIAN_POINT ( 'NONE',  ( 10.96812435474240033, 1424.188686434009924, 203.1558521378470061 ) ) ;
#67202=CARTESIAN_POINT ( 'NONE',  ( 0.7162966257659990621, 1429.709262178790141, 217.4063658874189855 ) ) ;
#67213=CARTESIAN_POINT ( 'NONE',  ( 10.13868529792319961, 1424.969151293629920, 198.0587525885179900 ) ) ;
#67214=CARTESIAN_POINT ( 'NONE',  ( 9.280010414808909758, 1463.749110535250111, 212.8038994763399785 ) ) ;
#67216=LINE ( 'NONE', #31929, #81747 ) ;
#67224=CARTESIAN_POINT ( 'NONE',  ( 2.104155298439795985, 1498.155611471770271, 198.0147149805754623 ) ) ;
#67226=ADVANCED_FACE ( 'NONE', ( #42155 ), #68479, .T. ) ;
#67227=CARTESIAN_POINT ( 'NONE',  ( -17.44763429059999993, 1419.603095734770022, 210.4313944482690033 ) ) ;
#67232=CARTESIAN_POINT ( 'NONE',  ( -17.25884833950082609, 1444.159326553692381, 200.5184012139974357 ) ) ;
#67237=CARTESIAN_POINT ( 'NONE',  ( -0.7967004023129989898, 1485.728201538589929, 197.6341324597989910 ) ) ;
#67243=CARTESIAN_POINT ( 'NONE',  ( -4.027171621128789347, 1433.589808380620070, 217.4404546235140003 ) ) ;
#67246=LINE ( 'NONE', #43134, #46804 ) ;
#67250=CARTESIAN_POINT ( 'NONE',  ( 11.75990446747050022, 1426.852756732119815, 206.8413600417420071 ) ) ;
#67252=EDGE_CURVE ( 'NONE', #108761, #36610, #16861, .T. ) ;
#67258=CARTESIAN_POINT ( 'NONE',  ( 4.808466515050000112, 1473.073685605089850, 218.2848264561289966 ) ) ;
#67260=B_SPLINE_CURVE_WITH_KNOTS ( 'NONE', 5,
 ( #92260, #41317, #75488, #32893, #37331, #95574, #88832, #2647, #18844 ),
 .UNSPECIFIED., .F., .F.,
 ( 6, 3, 6 ),
 ( 0.000000000000000000, 0.3683424536080230349, 1.000000000000000000 ),
 .UNSPECIFIED. ) ;
#67263=CARTESIAN_POINT ( 'NONE',  ( -11.24222043440000007, 1491.652723429889875, 206.9322345682190303 ) ) ;
#67271=CARTESIAN_POINT ( 'NONE',  ( -2.255841543630000334, 1456.176501937790135, 199.9086794445890121 ) ) ;
#67292=CARTESIAN_POINT ( 'NONE',  ( 12.66352736667499990, 1500.820466445309876, 210.2033082695159862 ) ) ;
#67297=CARTESIAN_POINT ( 'NONE',  ( -9.609622886946858955, 1464.248407205509920, 228.1966016402350022 ) ) ;
#67299=VERTEX_POINT ( 'NONE', #61200 ) ;
#67301=CARTESIAN_POINT ( 'NONE',  ( 10.24817655218739887, 1453.388637960930055, 211.8760523666580298 ) ) ;
#67304=CARTESIAN_POINT ( 'NONE',  ( -13.59236344883730041, 1508.248948055430219, 209.5387630291689902 ) ) ;
#67305=CARTESIAN_POINT ( 'NONE',  ( 4.325231581420000637, 1515.225841049890050, 210.2096722485289888 ) ) ;
#67306=CARTESIAN_POINT ( 'NONE',  ( -4.659350606432629327, 1455.294773417379929, 200.9200808099520259 ) ) ;
#67319=ORIENTED_EDGE ( 'NONE', *, *, #5484, .F. ) ;
#67322=CARTESIAN_POINT ( 'NONE',  ( -18.60427693160000118, 1442.816495467589903, 206.3589439838089845 ) ) ;
#67323=CARTESIAN_POINT ( 'NONE',  ( -4.138380534042295444, 1488.912756140813372, 219.2090725797449409 ) ) ;
#67326=CARTESIAN_POINT ( 'NONE',  ( 10.16156728606890169, 1469.494191575119885, 207.3232880352639711 ) ) ;
#67332=CARTESIAN_POINT ( 'NONE',  ( 6.046917389341460058, 1467.277928683999789, 199.7767350800179997 ) ) ;
#67333=CARTESIAN_POINT ( 'NONE',  ( 6.454036364709999418, 1470.375359969389820, 211.5526526928690032 ) ) ;
#67343=CARTESIAN_POINT ( 'NONE',  ( -12.22599082290759931, 1501.771664294480161, 211.5404786625699955 ) ) ;
#67350=CARTESIAN_POINT ( 'NONE',  ( 2.532296112024570167, 1445.968147867059997, 199.3366315615400026 ) ) ;
#67352=CARTESIAN_POINT ( 'NONE',  ( -6.871201816620469138, 1426.439416242710195, 202.8156393802020148 ) ) ;
#67369=CARTESIAN_POINT ( 'NONE',  ( -15.81441164190000315, 1416.657489259210024, 207.5143518867189982 ) ) ;
#67372=CARTESIAN_POINT ( 'NONE',  ( -17.64146421497870065, 1419.304501645640130, 207.1873797621490212 ) ) ;
#67373=CARTESIAN_POINT ( 'NONE',  ( -4.885870092120000230, 1496.077246227390106, 219.2393726144989898 ) ) ;
#67375=CARTESIAN_POINT ( 'NONE',  ( -2.151012986799999638, 1477.102208436890123, 201.8328325564689862 ) ) ;
#67378=CARTESIAN_POINT ( 'NONE',  ( -10.68670300233429948, 1508.551704408280102, 208.2058367971190194 ) ) ;
#67394=CARTESIAN_POINT ( 'NONE',  ( 12.49224530861089910, 1421.594377902519909, 207.3542241632320042 ) ) ;
#67395=CARTESIAN_POINT ( 'NONE',  ( 11.05809750370510081, 1479.027348187909865, 206.7510526044619894 ) ) ;
#67397=CARTESIAN_POINT ( 'NONE',  ( 5.278853968920000028, 1437.432420937689812, 228.7383191228989858 ) ) ;
#67399=CARTESIAN_POINT ( 'NONE',  ( -17.11734381175650199, 1420.830841924690048, 201.6585952501770009 ) ) ;
#67400=CARTESIAN_POINT ( 'NONE',  ( -16.88664006666689943, 1417.438760776740082, 207.9215829781489902 ) ) ;
#67405=CARTESIAN_POINT ( 'NONE',  ( 6.788622268498730072, 1448.339992550449779, 201.4086086841240331 ) ) ;
#67423=CARTESIAN_POINT ( 'NONE',  ( 2.849562163010020299, 1515.551843419029865, 205.1388868824799943 ) ) ;
#67429=CARTESIAN_POINT ( 'NONE',  ( 2.800557851600000259, 1466.634424046189906, 219.8247096032989987 ) ) ;
#67431=( NAMED_UNIT ( * ) PLANE_ANGLE_UNIT ( ) SI_UNIT ( $, .RADIAN. ) );
#67432=CARTESIAN_POINT ( 'NONE',  ( 11.31770122492290120, 1479.526177409110232, 208.6192917484059990 ) ) ;
#67446=CARTESIAN_POINT ( 'NONE',  ( -11.33291981729999875, 1502.012779296890130, 207.3104068824690103 ) ) ;
#67457=VERTEX_POINT ( 'NONE', #12944 ) ;
#67459=CARTESIAN_POINT ( 'NONE',  ( 3.346707516019999940, 1443.005054410889898, 217.3642451189890323 ) ) ;
#67462=B_SPLINE_CURVE_WITH_KNOTS ( 'NONE', 5,
 ( #82664, #39557, #56367, #40653, #66436, #14885 ),
 .UNSPECIFIED., .F., .F.,
 ( 6, 6 ),
 ( 0.000000000000000000, 1.000000000000000000 ),
 .UNSPECIFIED. ) ;
#67465=CARTESIAN_POINT ( 'NONE',  ( -3.775538771436770080, 1428.481285291019958, 200.5571954888419839 ) ) ;
#67469=CARTESIAN_POINT ( 'NONE',  ( 9.738091431092259498, 1435.054350372520048, 207.9788105490890189 ) ) ;
#67473=ORIENTED_EDGE ( 'NONE', *, *, #57841, .F. ) ;
#67477=EDGE_CURVE ( 'NONE', #70504, #52452, #105661, .T. ) ;
#67486=CARTESIAN_POINT ( 'NONE',  ( -9.310808169944788659, 1449.136903302260180, 208.8655000368800074 ) ) ;
#67488=ORIENTED_EDGE ( 'NONE', *, *, #26320, .T. ) ;
#67493=CYLINDRICAL_SURFACE ( 'NONE', #73358, 0.4999999999999449329 ) ;
#67495=CARTESIAN_POINT ( 'NONE',  ( -7.992444398102118264, 1461.756363228467990, 203.5959791406405088 ) ) ;
#67496=CARTESIAN_POINT ( 'NONE',  ( 4.789673499540000101, 1465.867933640490037, 219.0700355186390027 ) ) ;
#67506=CARTESIAN_POINT ( 'NONE',  ( 9.793647689141911528, 1463.364106758136359, 209.6829145745567757 ) ) ;
#67508=CARTESIAN_POINT ( 'NONE',  ( 5.172586535390000684, 1492.767659076290101, 188.8148697515989909 ) ) ;
#67511=CARTESIAN_POINT ( 'NONE',  ( 12.68801076269999939, 1500.413651118889902, 208.6561541774999853 ) ) ;
#67515=CARTESIAN_POINT ( 'NONE',  ( -9.361409357458470026, 1438.259538539160076, 210.6630235057149889 ) ) ;
#67516=CARTESIAN_POINT ( 'NONE',  ( 2.020654978418439995, 1495.217425279760164, 220.5028404108620066 ) ) ;
#67519=CARTESIAN_POINT ( 'NONE',  ( -5.552491127060000586, 1484.291244666589819, 199.5131677064289875 ) ) ;
#67523=ORIENTED_EDGE ( 'NONE', *, *, #98663, .F. ) ;
#67528=CARTESIAN_POINT ( 'NONE',  ( 1.477486856589759867, 1435.528368648049991, 227.5227238277980177 ) ) ;
#67529=CARTESIAN_POINT ( 'NONE',  ( -15.30308233943090102, 1416.035155480296453, 206.6202068181550828 ) ) ;
#67530=CARTESIAN_POINT ( 'NONE',  ( 1.758536932969999800, 1455.155312436190115, 218.3895007395989865 ) ) ;
#67532=CARTESIAN_POINT ( 'NONE',  ( -8.272393485109997613, 1447.204352650790042, 213.4245211968789988 ) ) ;
#67537=CARTESIAN_POINT ( 'NONE',  ( 7.377911345740000293, 1424.802628287519838, 212.4706883527589696 ) ) ;
#67542=CARTESIAN_POINT ( 'NONE',  ( -18.89431622735909855, 1483.154720315450049, 218.3089724768730093 ) ) ;
#67544=ORIENTED_EDGE ( 'NONE', *, *, #78365, .F. ) ;
#67545=ORIENTED_EDGE ( 'NONE', *, *, #27065, .T. ) ;
#67556=CARTESIAN_POINT ( 'NONE',  ( -8.992323206176040529, 1449.218714500919987, 210.9227175850809886 ) ) ;
#67560=CARTESIAN_POINT ( 'NONE',  ( -4.327051608332210364, 1515.156337024050117, 209.3139746709489941 ) ) ;
#67568=AXIS2_PLACEMENT_3D ( 'NONE', #79770, #55129, #36105 ) ;
#67572=VECTOR ( 'NONE', #69769, 1000.000000000000000 ) ;
#67584=CARTESIAN_POINT ( 'NONE',  ( 10.74646275119079952, 1460.429788200699704, 207.1630952569950068 ) ) ;
#67589=CARTESIAN_POINT ( 'NONE',  ( -4.869818399669999742, 1491.215867106689984, 188.8099941780989752 ) ) ;
#67590=CARTESIAN_POINT ( 'NONE',  ( -18.31482527320000031, 1445.278739201789904, 204.5307550449689984 ) ) ;
#67595=CARTESIAN_POINT ( 'NONE',  ( -10.30262272859999939, 1471.797637931690133, 208.8808052225769814 ) ) ;
#67601=CARTESIAN_POINT ( 'NONE',  ( -12.14128143079999944, 1416.006154796849842, 206.7539641484389961 ) ) ;
#67603=CARTESIAN_POINT ( 'NONE',  ( 5.653236855950000361, 1487.809232560990040, 198.9822455535989718 ) ) ;
#67605=CARTESIAN_POINT ( 'NONE',  ( -11.60674135321730027, 1507.508082919659955, 207.5537295141489835 ) ) ;
#67612=CARTESIAN_POINT ( 'NONE',  ( 1.582067810090000045E-15, 1508.551704408389924, 209.1218459616989946 ) ) ;
#67613=CARTESIAN_POINT ( 'NONE',  ( -17.02334047809999973, 1420.318775465339968, 203.7071964112190017 ) ) ;
#67615=CARTESIAN_POINT ( 'NONE',  ( -18.17086109458769982, 1508.551704408389924, 210.8151139196999679 ) ) ;
#67619=CARTESIAN_POINT ( 'NONE',  ( -0.4696341913122200062, 1423.394439732270030, 191.2019798439270062 ) ) ;
#67620=CARTESIAN_POINT ( 'NONE',  ( -7.756928808066270165, 1508.430203411700177, 219.4938965895260026 ) ) ;
#67627=CARTESIAN_POINT ( 'NONE',  ( -12.16253720638220059, 1419.838831633310065, 197.2883658129150035 ) ) ;
#67631=B_SPLINE_CURVE_WITH_KNOTS ( 'NONE', 3,
 ( #109143, #39154, #49787, #13388, #81700, #30758, #64939, #99053, #22332, #56533, #34625, #92869, #58732, #25655, #32958, #59305, #67147, #85561, #67699, #102372, #101808, #84476, #16686, #60964, #93970, #110224, #51431, #1052, #76628, #18356, #41382, #50883, #76086, #93419 ),
 .UNSPECIFIED., .F., .F.,
 ( 4, 3, 3, 3, 3, 3, 3, 3, 3, 3, 3, 4 ),
 ( -2.000000000000000000, -1.872087319251769966, -1.687892984705650079, -1.501460662300799997, -1.313840537329579838, -1.124757636572869979, -0.9352500492189879111, -0.7457836696873179072, -0.5568196230199600194, -0.3695388451267069829, -0.1838439808487151161, 0.000000000000000000 ),
 .UNSPECIFIED. ) ;
#67633=CARTESIAN_POINT ( 'NONE',  ( -4.318206861440000210, 1497.528676090189947, 220.7835062296990145 ) ) ;
#67635=CARTESIAN_POINT ( 'NONE',  ( -18.22821675530000007, 1443.229620277490085, 204.5519556382290034 ) ) ;
#67640=CARTESIAN_POINT ( 'NONE',  ( 10.08036567563580199, 1422.462408472209972, 212.0547761052640112 ) ) ;
#67644=CARTESIAN_POINT ( 'NONE',  ( 18.94656048379999902, 1455.761273475090093, 200.3458234316790083 ) ) ;
#67649=CARTESIAN_POINT ( 'NONE',  ( 10.54079341922740021, 1491.061758365090100, 212.2573636860299757 ) ) ;
#67650=FACE_OUTER_BOUND ( 'NONE', #81033, .T. ) ;
#67651=ORIENTED_EDGE ( 'NONE', *, *, #80204, .T. ) ;
#67656=VERTEX_POINT ( 'NONE', #86090 ) ;
#67657=CARTESIAN_POINT ( 'NONE',  ( -4.993214567250789493, 1391.653935164599716, 214.7089805434449943 ) ) ;
#67658=CARTESIAN_POINT ( 'NONE',  ( -8.170894480889998590, 1500.638869073389969, 209.8833235920569962 ) ) ;
#67662=CARTESIAN_POINT ( 'NONE',  ( -10.28857233090000101, 1463.185141274090256, 204.9217573806190273 ) ) ;
#67665=DIRECTION ( 'NONE',  ( -1.305148739725796033E-31, 1.000000000000000000, -1.836970198721029688E-16 ) ) ;
#67666=CARTESIAN_POINT ( 'NONE',  ( -11.35885305070239859, 1508.551704408389924, 217.6084463250130057 ) ) ;
#67669=CARTESIAN_POINT ( 'NONE',  ( -1.553759244419499863, 1485.745504604600001, 197.3241831226270051 ) ) ;
#67670=CARTESIAN_POINT ( 'NONE',  ( -2.130922739038390024, 1467.954349360780043, 220.0452206896550251 ) ) ;
#67676=CARTESIAN_POINT ( 'NONE',  ( 20.53971479803719902, 1476.913985495619954, 217.7491938173760104 ) ) ;
#67683=CARTESIAN_POINT ( 'NONE',  ( -11.96878399062378939, 1507.593741241288626, 208.5523078659349494 ) ) ;
#67685=CARTESIAN_POINT ( 'NONE',  ( 0.2414385729460010177, 1476.817046155289972, 198.6010158731990032 ) ) ;
#67690=CARTESIAN_POINT ( 'NONE',  ( 3.260623164134589747, 1428.697964756740021, 216.7257091047359836 ) ) ;
#67691=CARTESIAN_POINT ( 'NONE',  ( -7.885009387709999373, 1425.368775642419905, 206.6265662114490169 ) ) ;
#67695=CARTESIAN_POINT ( 'NONE',  ( 7.446545243910679623, 1426.150453638759927, 212.4588778087180003 ) ) ;
#67699=CARTESIAN_POINT ( 'NONE',  ( -11.14769255285479943, 1491.958836887719826, 207.0420635619269945 ) ) ;
#67701=CARTESIAN_POINT ( 'NONE',  ( 12.67629937430701936, 1426.478869958664063, 202.7079000866955028 ) ) ;
#67703=CARTESIAN_POINT ( 'NONE',  ( 8.935942533379998665, 1425.567594377970181, 193.3040559142989991 ) ) ;
#67709=CARTESIAN_POINT ( 'NONE',  ( 8.909790489964100502, 1434.607596429470050, 206.3238506486309802 ) ) ;
#67719=CARTESIAN_POINT ( 'NONE',  ( 4.303242241110600830, 1508.728291974460035, 212.9101315294259678 ) ) ;
#67731=CARTESIAN_POINT ( 'NONE',  ( -10.44591860737159905, 1479.590090999679887, 210.1597183799869697 ) ) ;
#67735=CARTESIAN_POINT ( 'NONE',  ( 7.573774609450000028, 1421.897575251010039, 195.7040863559990100 ) ) ;
#67736=CARTESIAN_POINT ( 'NONE',  ( -2.557552783909830207, 1432.931063180149977, 218.3108672520129971 ) ) ;
#67737=CARTESIAN_POINT ( 'NONE',  ( -4.311223378659999383, 1495.728807022490173, 198.3651121709989980 ) ) ;
#67747=CARTESIAN_POINT ( 'NONE',  ( -11.05503427808429961, 1483.026236761159907, 204.6865788484709867 ) ) ;
#67749=CARTESIAN_POINT ( 'NONE',  ( 9.104124838956808574, 1427.252791609349742, 211.0639582536120145 ) ) ;
#67750=CARTESIAN_POINT ( 'NONE',  ( 12.18334191729579885, 1421.374448972539994, 203.4336414120620020 ) ) ;
#67759=CARTESIAN_POINT ( 'NONE',  ( 4.653685083909150144, 1466.070315411240017, 218.6935422048629789 ) ) ;
#67765=CARTESIAN_POINT ( 'NONE',  ( 0.3646030894699989755, 1473.314417745290257, 216.5794721063890051 ) ) ;
#67768=CARTESIAN_POINT ( 'NONE',  ( 12.70693932329499809, 1426.829486560239957, 205.0434112651460055 ) ) ;
#67769=CARTESIAN_POINT ( 'NONE',  ( -9.838224544249689174, 1462.268909281400056, 227.9668214889109947 ) ) ;
#67771=CARTESIAN_POINT ( 'NONE',  ( -18.45566820803939834, 1419.316056982640021, 207.4717884025210139 ) ) ;
#67774=ORIENTED_EDGE ( 'NONE', *, *, #61954, .T. ) ;
#67783=CARTESIAN_POINT ( 'NONE',  ( -11.39446584399999907, 1470.674086033289996, 209.5209555135179755 ) ) ;
#67785=CARTESIAN_POINT ( 'NONE',  ( 9.146237114798470458, 1449.998848199699978, 208.1168068718100130 ) ) ;
#67788=CARTESIAN_POINT ( 'NONE',  ( -6.865221456288480795, 1434.987526699120053, 214.6275269604420259 ) ) ;
#67791=CARTESIAN_POINT ( 'NONE',  ( -15.68237649659999811, 1416.893877491339936, 210.3432287165989862 ) ) ;
#67796=CARTESIAN_POINT ( 'NONE',  ( 12.45038714344340036, 1421.619513592610019, 207.5027818182680051 ) ) ;
#67803=CARTESIAN_POINT ( 'NONE',  ( 3.028998513489999933, 1474.332429607289896, 219.7118052044990009 ) ) ;
#67804=CIRCLE ( 'NONE', #19493, 15.41143114519999990 ) ;
#67807=CARTESIAN_POINT ( 'NONE',  ( -11.38768754900000069, 1491.978877293390042, 204.2815689120989759 ) ) ;
#67815=CARTESIAN_POINT ( 'NONE',  ( -3.271538066909999820, 1454.292002242289982, 199.1638777246189989 ) ) ;
#67819=B_SPLINE_SURFACE_WITH_KNOTS ( 'NONE', 5, 1, ( 
 ( #24817, #82560 ),
 ( #14785, #48416 ),
 ( #75811, #5852 ),
 ( #14228, #15324 ),
 ( #32696, #65763 ),
 ( #108300, #50609 ),
 ( #7493, #48970 ),
 ( #84741, #23178 ),
 ( #41655, #109962 ) ),
 .UNSPECIFIED., .F., .F., .F.,
 ( 6, 3, 6 ),
 ( 2, 2 ),
 ( 0.000000000000000000, 3.215063553959999876, 6.404940046369999251 ),
 ( 0.000000000000000000, 14.00000000000000000 ),
 .UNSPECIFIED. ) ;
#67821=CARTESIAN_POINT ( 'NONE',  ( -2.699177585649999767, 1497.662919768989923, 198.1511405123989960 ) ) ;
#67823=ORIENTED_EDGE ( 'NONE', *, *, #21553, .F. ) ;
#67831=ADVANCED_FACE ( 'NONE', ( #89943 ), #77009, .T. ) ;
#67840=CARTESIAN_POINT ( 'NONE',  ( 4.714200449835320050, 1508.551704408389924, 212.7479841881830112 ) ) ;
#67844=CARTESIAN_POINT ( 'NONE',  ( 9.831033741157400030, 1461.797019875059959, 208.3422837267889918 ) ) ;
#67845=DIRECTION ( 'NONE',  ( 0.02091224828123190022, 0.9990482215818557998, 0.03827961371219716635 ) ) ;
#67846=ORIENTED_EDGE ( 'NONE', *, *, #74162, .F. ) ;
#67847=ORIENTED_EDGE ( 'NONE', *, *, #6332, .T. ) ;
#67849=CARTESIAN_POINT ( 'NONE',  ( 10.47141298996499970, 1453.021995586940193, 210.7640114736790053 ) ) ;
#67851=CARTESIAN_POINT ( 'NONE',  ( -13.58463681145030044, 1508.551704409039985, 210.0579325790299947 ) ) ;
#67852=CARTESIAN_POINT ( 'NONE',  ( 4.038581993089999322, 1515.598601291389969, 209.4983956875140052 ) ) ;
#67853=VECTOR ( 'NONE', #61004, 1000.000000000000114 ) ;
#67868=ORIENTED_EDGE ( 'NONE', *, *, #20166, .F. ) ;
#67871=CARTESIAN_POINT ( 'NONE',  ( -8.589426147275000645, 1436.798469860880004, 209.9038450004319998 ) ) ;
#67874=CARTESIAN_POINT ( 'NONE',  ( -7.145047903430882030, 1489.825692955459090, 217.4065108216325370 ) ) ;
#67876=CARTESIAN_POINT ( 'NONE',  ( 10.37416452553040003, 1469.777074456880200, 207.1978045308729861 ) ) ;
#67877=CARTESIAN_POINT ( 'NONE',  ( -9.404697644369997889, 1472.841355724789992, 204.0220805676790121 ) ) ;
#67883=CARTESIAN_POINT ( 'NONE',  ( 4.849004271086250206, 1466.839050287979944, 199.1402214942249884 ) ) ;
#67888=ADVANCED_FACE ( 'NONE', ( #32789 ), #9054, .T. ) ;
#67892=CARTESIAN_POINT ( 'NONE',  ( 5.476230074880000132, 1506.245546354389944, 219.4133339360989794 ) ) ;
#67893=CARTESIAN_POINT ( 'NONE',  ( -14.86110812849999974, 1416.023439710309958, 213.2201437424990047 ) ) ;
#67894=CARTESIAN_POINT ( 'NONE',  ( -11.31981798910900139, 1500.653229225639961, 211.0236618496560084 ) ) ;
#67895=VERTEX_POINT ( 'NONE', #42864 ) ;
#67897=CARTESIAN_POINT ( 'NONE',  ( -2.174382577350000290, 1508.375792276090124, 220.6907864031990130 ) ) ;
#67905=CARTESIAN_POINT ( 'NONE',  ( -10.17045319919999891, 1479.387637944790185, 211.9243876371689908 ) ) ;
#67911=CARTESIAN_POINT ( 'NONE',  ( 1.326713953160000070, 1454.806608698389937, 218.4390644836289823 ) ) ;
#67915=CARTESIAN_POINT ( 'NONE',  ( 1.326713953160000070, 1454.806608698389937, 218.4390644836289823 ) ) ;
#67918=CARTESIAN_POINT ( 'NONE',  ( -10.48877660729999839, 1461.381695361490074, 212.5316338973990185 ) ) ;
#67919=AXIS2_PLACEMENT_3D ( 'NONE', #82210, #81108, #6614 ) ;
#67921=CARTESIAN_POINT ( 'NONE',  ( -16.64332109206937815, 1419.610251472236087, 209.0439647319126948 ) ) ;
#67922=CARTESIAN_POINT ( 'NONE',  ( -5.269464883259999510, 1497.518825018089956, 219.5548267382990275 ) ) ;
#67928=CARTESIAN_POINT ( 'NONE',  ( 10.54494294924669973, 1481.809169021529897, 210.1168006503139907 ) ) ;
#67933=ADVANCED_FACE ( 'NONE', ( #43966 ), #105338, .T. ) ;
#67944=CARTESIAN_POINT ( 'NONE',  ( 4.474738246519999407, 1484.773668731990028, 219.2871524305990079 ) ) ;
#67945=CIRCLE ( 'NONE', #57241, 3.250000000000000000 ) ;
#67946=ADVANCED_FACE ( 'NONE', ( #50704 ), #43035, .T. ) ;
#67950=CARTESIAN_POINT ( 'NONE',  ( -19.47049107349999630, 1446.886758059190015, 200.1674925962190059 ) ) ;
#67956=DIRECTION ( 'NONE',  ( -1.000000000000000000, 0.000000000000000000, 0.000000000000000000 ) ) ;
#67964=CARTESIAN_POINT ( 'NONE',  ( 5.662343758720000508, 1504.894618425089902, 220.5557215505990314 ) ) ;
#67971=ORIENTED_EDGE ( 'NONE', *, *, #26512, .T. ) ;
#67978=CARTESIAN_POINT ( 'NONE',  ( 4.329415281104790125, 1515.068899390480283, 206.1637483033499905 ) ) ;
#67989=ORIENTED_EDGE ( 'NONE', *, *, #70801, .T. ) ;
#67996=CARTESIAN_POINT ( 'NONE',  ( -7.852484159231844174, 1474.938952242313007, 202.4682600550963514 ) ) ;
#68000=EDGE_CURVE ( 'NONE', #42483, #75452, #98401, .T. ) ;
#68001=CARTESIAN_POINT ( 'NONE',  ( 11.35450994474380160, 1422.091444931230171, 210.1627864600919793 ) ) ;
#68017=CARTESIAN_POINT ( 'NONE',  ( 1.598076626895770458, 1456.722266292764971, 199.3428600893386715 ) ) ;
#68018=LINE ( 'NONE', #18124, #14106 ) ;
#68020=EDGE_CURVE ( 'NONE', #51946, #40367, #97040, .T. ) ;
#68027=CARTESIAN_POINT ( 'NONE',  ( -11.85515813369189964, 1482.126388357829910, 208.2119403444889940 ) ) ;
#68037=CARTESIAN_POINT ( 'NONE',  ( 11.82041243239999950, 1421.864495970979760, 207.3036273995689669 ) ) ;
#68041=CARTESIAN_POINT ( 'NONE',  ( -9.183331090101370719, 1449.795978047580093, 208.6042095093999933 ) ) ;
#68045=CARTESIAN_POINT ( 'NONE',  ( -10.38930660322390054, 1508.437704431200018, 218.6021076291179952 ) ) ;
#68049=CARTESIAN_POINT ( 'NONE',  ( 10.94755632455209948, 1461.011583818969939, 208.8505059419150029 ) ) ;
#68051=CARTESIAN_POINT ( 'NONE',  ( -1.073543300500000131, 1444.993504060389796, 218.0402178135990141 ) ) ;
#68059=CARTESIAN_POINT ( 'NONE',  ( -2.699757113132419839, 1445.584394931136330, 217.7557302367460750 ) ) ;
#68060=ORIENTED_EDGE ( 'NONE', *, *, #7663, .T. ) ;
#68061=CARTESIAN_POINT ( 'NONE',  ( -9.359063114774409442, 1440.623793696270013, 205.4860248794589950 ) ) ;
#68068=CARTESIAN_POINT ( 'NONE',  ( 11.40247488079999982, 1503.020469010889883, 210.7587791148490055 ) ) ;
#68071=B_SPLINE_SURFACE_WITH_KNOTS ( 'NONE', 5, 1, ( 
 ( #68536, #51165 ),
 ( #85293, #89717 ),
 ( #4085, #46645 ),
 ( #55043, #89170 ),
 ( #72393, #62352 ),
 ( #27614, #37668 ) ),
 .UNSPECIFIED., .F., .F., .F.,
 ( 6, 6 ),
 ( 2, 2 ),
 ( 0.000000000000000000, 14.54369801220000014 ),
 ( 0.000000000000000000, 14.00000000000000000 ),
 .UNSPECIFIED. ) ;
#68073=CARTESIAN_POINT ( 'NONE',  ( -2.329957323386520063, 1515.551704201149960, 212.9510108339450198 ) ) ;
#68081=ADVANCED_FACE ( 'NONE', ( #46741 ), #17044, .T. ) ;
#68084=ORIENTED_EDGE ( 'NONE', *, *, #62431, .T. ) ;
#68086=CARTESIAN_POINT ( 'NONE',  ( -2.275164556450000042, 1500.397458187289885, 230.3260808154989832 ) ) ;
#68090=CARTESIAN_POINT ( 'NONE',  ( -6.864156050670000120, 1445.800717418090017, 215.8105125318990076 ) ) ;
#68102=ORIENTED_EDGE ( 'NONE', *, *, #104342, .T. ) ;
#68111=CARTESIAN_POINT ( 'NONE',  ( -0.8344454606485569581, 1475.590793790669977, 197.7023485705600194 ) ) ;
#68115=CARTESIAN_POINT ( 'NONE',  ( -9.521762932734290530, 1448.211015946100133, 209.8758324204249845 ) ) ;
#68119=EDGE_LOOP ( 'NONE', ( #47950, #18898, #83113, #74422, #68697, #100994, #55922, #60344, #108474, #35091, #52192, #34454 ) ) ;
#68120=CARTESIAN_POINT ( 'NONE',  ( -4.327012684985790614, 1515.157823446690145, 209.2498876927999731 ) ) ;
#68125=EDGE_CURVE ( 'NONE', #38761, #21803, #83071, .T. ) ;
#68127=CARTESIAN_POINT ( 'NONE',  ( 8.149545062026291475, 1425.007426972460053, 194.5668190883189936 ) ) ;
#68142=CARTESIAN_POINT ( 'NONE',  ( -11.39446592756109844, 1470.674086296440009, 209.5209556861319982 ) ) ;
#68154=CARTESIAN_POINT ( 'NONE',  ( 9.163876979147371316, 1436.806046061350116, 211.4130592609789971 ) ) ;
#68155=CARTESIAN_POINT ( 'NONE',  ( 4.709428332219590452, 1480.407433587830155, 228.9870284858090201 ) ) ;
#68165=CARTESIAN_POINT ( 'NONE',  ( -3.707800477540000195, 1428.659817276889953, 200.9450977677189769 ) ) ;
#68168=CARTESIAN_POINT ( 'NONE',  ( -17.71996445940000342, 1417.056829823310181, 208.8389207556330120 ) ) ;
#68170=CARTESIAN_POINT ( 'NONE',  ( 3.971087474159999520, 1486.546787240489948, 198.9371065660989757 ) ) ;
#68174=CARTESIAN_POINT ( 'NONE',  ( -4.500000000000000000, 1508.551704408389924, 209.1218459616989946 ) ) ;
#68179=CARTESIAN_POINT ( 'NONE',  ( -17.35289783740000047, 1420.153549694379990, 203.7868233213689848 ) ) ;
#68181=CARTESIAN_POINT ( 'NONE',  ( -17.18717870511359891, 1508.551704408389924, 212.3238880613659774 ) ) ;
#68183=DIRECTION ( 'NONE',  ( 0.000000000000000000, -1.836970198721029688E-16, -1.000000000000000000 ) ) ;
#68186=CARTESIAN_POINT ( 'NONE',  ( -11.27898552558059997, 1471.200097733860275, 207.3676664588759877 ) ) ;
#68187=CARTESIAN_POINT ( 'NONE',  ( -7.088902828084099994, 1508.383691274782677, 219.7372291895070759 ) ) ;
#68190=CARTESIAN_POINT ( 'NONE',  ( 9.326415766526549689, 1460.944052182000178, 206.0389247924669860 ) ) ;
#68193=CARTESIAN_POINT ( 'NONE',  ( -4.255262048852619827, 1420.457194194370004, 194.1488550391260048 ) ) ;
#68200=CARTESIAN_POINT ( 'NONE',  ( -4.226426730299999157, 1515.477082009390188, 209.1218459616989946 ) ) ;
#68207=CARTESIAN_POINT ( 'NONE',  ( -17.65532971150000208, 1419.497219977419945, 207.2321558962389929 ) ) ;
#68223=CARTESIAN_POINT ( 'NONE',  ( 11.66681882931680114, 1479.992204709489897, 210.8129482343040024 ) ) ;
#68226=AXIS2_PLACEMENT_3D ( 'NONE', #73137, #73707, #64764 ) ;
#68231=CARTESIAN_POINT ( 'NONE',  ( 6.648508775361010592, 1432.796636464459880, 201.9740405741240181 ) ) ;
#68236=CARTESIAN_POINT ( 'NONE',  ( -4.635574868235029733, 1480.378675748950172, 230.9803143308730000 ) ) ;
#68245=CARTESIAN_POINT ( 'NONE',  ( -1.952774559090199924, 1420.709932442649915, 193.8387323542239926 ) ) ;
#68247=CARTESIAN_POINT ( 'NONE',  ( 1.251899778580000122, 1477.970563818089886, 198.7571063212990055 ) ) ;
#68254=CARTESIAN_POINT ( 'NONE',  ( -7.788352316159999233, 1425.537561632160077, 206.3143906032090058 ) ) ;
#68258=CARTESIAN_POINT ( 'NONE',  ( -5.886614042649569001, 1470.748248646887305, 217.3971333049484258 ) ) ;
#68259=CARTESIAN_POINT ( 'NONE',  ( 7.418470818223539709, 1426.217778447260116, 212.5279654691829876 ) ) ;
#68268=CARTESIAN_POINT ( 'NONE',  ( -3.152270375085599596, 1474.954422185709745, 198.1306180807430053 ) ) ;
#68269=CARTESIAN_POINT ( 'NONE',  ( 8.045781271640001009, 1426.290936267859934, 211.5934327219790134 ) ) ;
#68276=CARTESIAN_POINT ( 'NONE',  ( 8.665450313672950600, 1435.069259100369891, 206.7692196636689914 ) ) ;
#68284=CARTESIAN_POINT ( 'NONE',  ( 4.487249027372319787, 1509.038643251730036, 211.6097700576100067 ) ) ;
#68287=CARTESIAN_POINT ( 'NONE',  ( -5.667996024009999800, 1427.963166378290225, 202.8006845438689822 ) ) ;
#68292=CARTESIAN_POINT ( 'NONE',  ( 1.932637921108910195, 1445.685508784159993, 199.2156413524129732 ) ) ;
#68297=CARTESIAN_POINT ( 'NONE',  ( -4.333038850355530158, 1508.551704408389924, 213.2968085732719885 ) ) ;
#68299=CARTESIAN_POINT ( 'NONE',  ( 7.405238242969999440, 1422.788992526760012, 195.6018663419989991 ) ) ;
#68300=CARTESIAN_POINT ( 'NONE',  ( -0.8336025234663499983, 1432.165250642160117, 218.5883475804189686 ) ) ;
#68308=ORIENTED_EDGE ( 'NONE', *, *, #58015, .T. ) ;
#68310=CARTESIAN_POINT ( 'NONE',  ( -9.828026979480000591, 1446.801135606790012, 212.2328361272089978 ) ) ;
#68313=CARTESIAN_POINT ( 'NONE',  ( 8.490723549529160863, 1425.167024220250141, 210.6110084034939973 ) ) ;
#68322=CARTESIAN_POINT ( 'NONE',  ( 14.07282483770000070, 1429.542793039189974, 194.9276198725990241 ) ) ;
#68323=CARTESIAN_POINT ( 'NONE',  ( 9.931914985161359510, 1420.236473162700122, 196.5017368352029905 ) ) ;
#68332=CARTESIAN_POINT ( 'NONE',  ( -1.094850995740000110, 1515.349842019790003, 204.8390133007890199 ) ) ;
#68333=CARTESIAN_POINT ( 'NONE',  ( 5.047151244050088970, 1472.875750233941744, 217.9874323986091440 ) ) ;
#68334=CARTESIAN_POINT ( 'NONE',  ( 10.37959263469830162, 1453.090484190960069, 190.0119661209870117 ) ) ;
#68336=CARTESIAN_POINT ( 'NONE',  ( -11.87156193126500092, 1422.672759239169864, 205.5660461887279951 ) ) ;
#68342=CARTESIAN_POINT ( 'NONE',  ( -8.366082161509995174, 1446.966775783084813, 191.6214408458980074 ) ) ;
#68347=CARTESIAN_POINT ( 'NONE',  ( -10.96172188900000144, 1470.923991379590007, 209.2568965565250210 ) ) ;
#68350=FACE_OUTER_BOUND ( 'NONE', #31366, .T. ) ;
#68351=CARTESIAN_POINT ( 'NONE',  ( -8.812222042580639680, 1437.453945644680061, 211.4808504019430018 ) ) ;
#68358=CARTESIAN_POINT ( 'NONE',  ( 9.729357915104159815, 1424.710738619140102, 208.6220594428340007 ) ) ;
#68364=CARTESIAN_POINT ( 'NONE',  ( 4.672259132070000653, 1473.556464307690248, 218.6750198893490165 ) ) ;
#68367=CARTESIAN_POINT ( 'NONE',  ( -10.42285073610000090, 1493.346802325689850, 205.0798751281189993 ) ) ;
#68371=FACE_OUTER_BOUND ( 'NONE', #80226, .T. ) ;
#68372=CARTESIAN_POINT ( 'NONE',  ( 12.44780699480000052, 1501.268281545989794, 211.7240718090590121 ) ) ;
#68375=CARTESIAN_POINT ( 'NONE',  ( -2.868493496300000167, 1454.499781787289976, 199.0262477489989976 ) ) ;
#68380=CARTESIAN_POINT ( 'NONE',  ( 1.554813298490000051, 1495.819410965689940, 221.3803746977989988 ) ) ;
#68385=CARTESIAN_POINT ( 'NONE',  ( 0.000000000000000000, 1414.421228241719973, 209.1218459616989946 ) ) ;
#68396=ADVANCED_FACE ( 'NONE', ( #33206 ), #93964, .T. ) ;
#68397=CARTESIAN_POINT ( 'NONE',  ( 3.507271589441150361, 1508.551704408389924, 213.8929761831950032 ) ) ;
#68398=B_SPLINE_CURVE_WITH_KNOTS ( 'NONE', 5,
 ( #87120, #105594, #104470, #62513, #52988, #28877 ),
 .UNSPECIFIED., .F., .F.,
 ( 6, 6 ),
 ( 0.000000000000000000, 1.000000000000000000 ),
 .UNSPECIFIED. ) ;
#68400=ORIENTED_EDGE ( 'NONE', *, *, #92675, .T. ) ;
#68407=CARTESIAN_POINT ( 'NONE',  ( 8.376099081319999584, 1424.325079649750023, 195.9777991686989935 ) ) ;
#68409=CARTESIAN_POINT ( 'NONE',  ( -12.18109756395920051, 1417.441079092732707, 199.6933909727965215 ) ) ;
#68410=CARTESIAN_POINT ( 'NONE',  ( 4.226426710960000221, 1515.477082012290111, 209.4928269685999851 ) ) ;
#68411=B_SPLINE_CURVE_WITH_KNOTS ( 'NONE', 5,
 ( #57389, #56261, #14795, #5862, #40003, #30496 ),
 .UNSPECIFIED., .F., .F.,
 ( 6, 6 ),
 ( 0.000000000000000000, 1.000000000000000000 ),
 .UNSPECIFIED. ) ;
#68412=CARTESIAN_POINT ( 'NONE',  ( -4.523944140811339665, 1455.378620635879997, 200.8408219016489795 ) ) ;
#68415=CARTESIAN_POINT ( 'NONE',  ( 9.718886300337560513, 1452.141959363349997, 209.5745625312270022 ) ) ;
#68427=CARTESIAN_POINT ( 'NONE',  ( -8.508749110203201127, 1436.403459463997706, 210.5997781497169399 ) ) ;
#68428=CARTESIAN_POINT ( 'NONE',  ( -9.670072478253100456, 1461.149693659710238, 208.5233768627159918 ) ) ;
#68430=CARTESIAN_POINT ( 'NONE',  ( 9.967393941860828832, 1469.042125965680043, 207.5003470271620074 ) ) ;
#68431=CARTESIAN_POINT ( 'NONE',  ( -10.56464281290000073, 1472.012291739390093, 204.5722061169090011 ) ) ;
#68432=CARTESIAN_POINT ( 'NONE',  ( 6.508711678220000074, 1494.153788970689902, 218.6819253028189962 ) ) ;
#68436=CARTESIAN_POINT ( 'NONE',  ( 3.281831459213320201, 1466.303209658950209, 198.5678429405679992 ) ) ;
#68443=CARTESIAN_POINT ( 'NONE',  ( -14.87918228200000037, 1415.865102022439942, 212.9009079454490063 ) ) ;
#68444=CARTESIAN_POINT ( 'NONE',  ( 1.475794680595370112, 1515.075282686660103, 204.7926718715959851 ) ) ;
#68450=CARTESIAN_POINT ( 'NONE',  ( -10.99821780924659897, 1462.161413399840058, 209.8874997588229974 ) ) ;
#68452=CARTESIAN_POINT ( 'NONE',  ( -6.374652409100740158, 1426.817684424950130, 202.3048622467989901 ) ) ;
#68456=CARTESIAN_POINT ( 'NONE',  ( -10.54015973009999918, 1480.209825774290039, 212.3170011562690149 ) ) ;
#68465=CARTESIAN_POINT ( 'NONE',  ( 1.777651795228360143, 1454.685074748580064, 218.3589571427669966 ) ) ;
#68468=CARTESIAN_POINT ( 'NONE',  ( -16.25046204339999889, 1416.958518179149905, 207.5324767410789946 ) ) ;
#68471=CARTESIAN_POINT ( 'NONE',  ( -2.345429900402050016, 1485.575015422800107, 197.4542373693989816 ) ) ;
#68478=CARTESIAN_POINT ( 'NONE',  ( -10.86685207181099955, 1508.551704408280102, 208.7084760166389970 ) ) ;
#68479=CYLINDRICAL_SURFACE ( 'NONE', #20534, 0.5000000000000026645 ) ;
#68488=CARTESIAN_POINT ( 'NONE',  ( 4.326992699989999913, 1515.158586642889986, 209.1218459616989946 ) ) ;
#68489=CARTESIAN_POINT ( 'NONE',  ( -2.188078410709979771, 1508.020976590390092, 220.9453026643990086 ) ) ;
#68495=CARTESIAN_POINT ( 'NONE',  ( 10.51780859130439971, 1480.734537470010082, 208.3820307640789906 ) ) ;
#68497=CARTESIAN_POINT ( 'NONE',  ( -19.50074017869999921, 1447.081821278189864, 200.2081706008290212 ) ) ;
#68500=DIRECTION ( 'NONE',  ( -0.9525506456058961957, 0.2950089284981370352, 0.07494664543641200993 ) ) ;
#68504=DIRECTION ( 'NONE',  ( -9.153092986051941045E-47, 1.000000000000000000, -1.836970198721029688E-16 ) ) ;
#68505=CARTESIAN_POINT ( 'NONE',  ( -15.16604635449859906, 1420.474734527899955, 211.5444020733049797 ) ) ;
#68520=EDGE_LOOP ( 'NONE', ( #76098, #57112, #26637, #77900, #77459, #93318 ) ) ;
#68523=CARTESIAN_POINT ( 'NONE',  ( 3.542321145568990026, 1515.375307573260216, 205.1014385530530149 ) ) ;
#68530=EDGE_CURVE ( 'NONE', #52143, #56179, #15940, .T. ) ;
#68533=CARTESIAN_POINT ( 'NONE',  ( 17.78284146230000218, 1432.724246433989947, 213.5810953123289835 ) ) ;
#68536=CARTESIAN_POINT ( 'NONE',  ( 0.4279777834130009673, 1433.008008542290099, 203.3794753978790197 ) ) ;
#68546=CARTESIAN_POINT ( 'NONE',  ( 11.19147978021466550, 1422.145535819584893, 210.4506286102420916 ) ) ;
#68549=ORIENTED_EDGE ( 'NONE', *, *, #104242, .F. ) ;
#68551=ORIENTED_EDGE ( 'NONE', *, *, #100705, .T. ) ;
#68558=CARTESIAN_POINT ( 'NONE',  ( -3.220674668504990290, 1433.265634988960073, 218.1214075394389909 ) ) ;
#68559=ORIENTED_EDGE ( 'NONE', *, *, #10326, .F. ) ;
#68561=CARTESIAN_POINT ( 'NONE',  ( -13.58041510073769942, 1508.551704408389924, 210.3416170870220014 ) ) ;
#68564=EDGE_CURVE ( 'NONE', #41801, #32360, #48810, .T. ) ;
#68568=CARTESIAN_POINT ( 'NONE',  ( 2.601664184880000175, 1468.435072065989971, 215.8528537042190010 ) ) ;
#68583=CARTESIAN_POINT ( 'NONE',  ( -9.270159725700629849, 1448.714146504459904, 209.7629294459360096 ) ) ;
#68592=CARTESIAN_POINT ( 'NONE',  ( -7.506265444784725460, 1461.911152747223696, 202.9443364886544998 ) ) ;
#68593=CARTESIAN_POINT ( 'NONE',  ( 3.604343046649999938, 1467.193817153390000, 218.5376378362390142 ) ) ;
#68595=EDGE_CURVE ( 'NONE', #78107, #27485, #66029, .T. ) ;
#68599=CARTESIAN_POINT ( 'NONE',  ( -1.879007491539999908, 1430.448079191990018, 200.8521231223890027 ) ) ;
#68601=CARTESIAN_POINT ( 'NONE',  ( 10.47063686347510014, 1481.493996793529959, 210.6398709714650010 ) ) ;
#68612=CARTESIAN_POINT ( 'NONE',  ( 12.70238417940000097, 1500.652076303089871, 209.5864169051759802 ) ) ;
#68615=FACE_OUTER_BOUND ( 'NONE', #101759, .T. ) ;
#68618=B_SPLINE_CURVE_WITH_KNOTS ( 'NONE', 3,
 ( #57057, #88976, #6077, #21745, #13350, #64355, #97921, #12820, #47000, #80589 ),
 .UNSPECIFIED., .F., .F.,
 ( 4, 2, 2, 2, 4 ),
 ( 0.000000000000000000, 0.2499999999999998335, 0.4999999999999998890, 0.7499999999999998890, 1.000000000000000000 ),
 .UNSPECIFIED. ) ;
#68621=CARTESIAN_POINT ( 'NONE',  ( -6.191729861150000680, 1483.183474162390212, 200.3799189381190047 ) ) ;
#68624=EDGE_LOOP ( 'NONE', ( #16264, #57927, #62068, #55459, #34232 ) ) ;
#68627=CARTESIAN_POINT ( 'NONE',  ( -9.399544156962228669, 1482.890756672869884, 227.8968317774389902 ) ) ;
#68628=ORIENTED_EDGE ( 'NONE', *, *, #16453, .T. ) ;
#68631=CARTESIAN_POINT ( 'NONE',  ( -15.20276107160831103, 1416.056970463632979, 206.2047736444255293 ) ) ;
#68634=CARTESIAN_POINT ( 'NONE',  ( -2.543319604096950126, 1457.772035387090000, 219.4813672542439917 ) ) ;
#68640=CARTESIAN_POINT ( 'NONE',  ( 10.37959279779999910, 1453.090483345690018, 190.0119662633989890 ) ) ;
#68645=CARTESIAN_POINT ( 'NONE',  ( -14.00462132320000030, 1415.677402202029953, 214.2425697179989754 ) ) ;
#68647=EDGE_LOOP ( 'NONE', ( #34977, #84279, #38153, #79247 ) ) ;
#68669=CARTESIAN_POINT ( 'NONE',  ( 6.812867228078430593, 1424.640977396479911, 193.9125305968219948 ) ) ;
#68697=ORIENTED_EDGE ( 'NONE', *, *, #18138, .F. ) ;
#68705=CARTESIAN_POINT ( 'NONE',  ( -3.611921233329999925, 1429.380855016690020, 201.5074060074890099 ) ) ;
#68720=B_SPLINE_SURFACE_WITH_KNOTS ( 'NONE', 5, 5, ( 
 ( #89111, #110591, #13480, #73975, #12942, #91861 ),
 ( #4028, #14597, #65582, #107010, #56069, #47123 ),
 ( #55530, #72875, #30298, #99694, #14038, #57191 ),
 ( #29750, #81250, #72336, #22420, #38699, #63938 ),
 ( #31402, #22986, #82369, #47670, #108106, #4565 ),
 ( #91315, #38156, #48787, #82911, #64491, #90196 ),
 ( #89656, #98606, #21870, #81798, #6202, #48229 ),
 ( #40354, #98051, #5100, #106466, #56623, #39253 ),
 ( #30849, #23550, #73428, #100271, #90758, #107563 ) ),
 .UNSPECIFIED., .F., .F., .F.,
 ( 6, 3, 6 ),
 ( 6, 6 ),
 ( 3.226035699099999654, 5.548136904300000616, 7.870238109499999801 ),
 ( 0.000000000000000000, 2.000000000000000000 ),
 .UNSPECIFIED. ) ;
#68722=CARTESIAN_POINT ( 'NONE',  ( -17.24072850490000164, 1420.216406558149856, 203.6744263160889830 ) ) ;
#68727=CARTESIAN_POINT ( 'NONE',  ( 3.028279354519999966, 1442.219580477389854, 217.5826834191090029 ) ) ;
#68733=CARTESIAN_POINT ( 'NONE',  ( -7.372143812753932046, 1458.228344989418474, 215.2092666101164582 ) ) ;
#68736=CARTESIAN_POINT ( 'NONE',  ( -13.93291478854189869, 1418.292988176089921, 201.4314801882400161 ) ) ;
#68737=CARTESIAN_POINT ( 'NONE',  ( -5.292247061280000331, 1391.913060387289988, 203.8075142969990168 ) ) ;
#68746=CARTESIAN_POINT ( 'NONE',  ( -10.37617513879240150, 1479.403831811299824, 210.6295454707710064 ) ) ;
#68747=B_SPLINE_SURFACE_WITH_KNOTS ( 'NONE', 5, 5, ( 
 ( #85680, #603, #58845, #67263, #35287, #86236 ),
 ( #16252, #33610, #24645, #43148, #94635, #92979 ),
 ( #33072, #68367, #26319, #34732, #84580, #67807 ),
 ( #69472, #59963, #60511, #50456, #59411, #42039 ),
 ( #76191, #110338, #101918, #8415, #42587, #103592 ),
 ( #50997, #43695, #93524, #26892, #61082, #16793 ),
 ( #76740, #51, #77848, #95197, #102474, #25764 ),
 ( #68923, #18457, #17347, #52655, #17909, #103023 ),
 ( #75654, #86792, #41494, #109793, #104695, #55412 ) ),
 .UNSPECIFIED., .F., .F., .F.,
 ( 6, 3, 6 ),
 ( 6, 6 ),
 ( 9.378668589109999232, 19.09106091769999836, 27.09462474520000086 ),
 ( 0.000000000000000000, 2.000000000000000000 ),
 .UNSPECIFIED. ) ;
#68750=CARTESIAN_POINT ( 'NONE',  ( -1.952265610894980075, 1487.388746950699897, 219.9076763016360019 ) ) ;
#68751=CARTESIAN_POINT ( 'NONE',  ( -19.86622903030000131, 1443.388330262490172, 213.1207022696590059 ) ) ;
#68756=CARTESIAN_POINT ( 'NONE',  ( 10.57208727109580160, 1452.520229422010061, 209.3749135230609966 ) ) ;
#68764=B_SPLINE_CURVE_WITH_KNOTS ( 'NONE', 3,
 ( #110336, #24103, #49896, #84578, #25205, #90775, #39831, #100287, #108124, #31418, #65600, #99713, #83470 ),
 .UNSPECIFIED., .F., .F.,
 ( 4, 3, 3, 3, 4 ),
 ( -1.703847294900000087, -0.8071511513289990614, 0.08392122703059357036, 0.9654601872785679717, 1.703847294900000087 ),
 .UNSPECIFIED. ) ;
#68771=CARTESIAN_POINT ( 'NONE',  ( 9.025697246586840805, 1436.232127817869923, 209.4982936030500014 ) ) ;
#68780=CARTESIAN_POINT ( 'NONE',  ( -16.26820474405350225, 1420.723844530150018, 203.3064050127150040 ) ) ;
#68784=ORIENTED_EDGE ( 'NONE', *, *, #107689, .T. ) ;
#68785=CARTESIAN_POINT ( 'NONE',  ( 18.28526225389999738, 1474.357479485790009, 194.7997304761989881 ) ) ;
#68789=CARTESIAN_POINT ( 'NONE',  ( -6.677286941980000279, 1473.976478301389989, 206.5095183912090135 ) ) ;
#68791=CARTESIAN_POINT ( 'NONE',  ( -12.78943302956389871, 1502.708798875820094, 209.0180534851929792 ) ) ;
#68794=CARTESIAN_POINT ( 'NONE',  ( -3.152270393760000289, 1474.954422226189990, 198.1306180379989996 ) ) ;
#68800=CARTESIAN_POINT ( 'NONE',  ( -7.713704896070000316, 1426.546663328330169, 206.3890337723190100 ) ) ;
#68805=CARTESIAN_POINT ( 'NONE',  ( 7.528229201135600235, 1425.827014894030071, 212.2334219967879960 ) ) ;
#68811=AXIS2_PLACEMENT_3D ( 'NONE', #28054, #44327, #37006 ) ;
#68812=CARTESIAN_POINT ( 'NONE',  ( 3.191256178858096426, 1486.666090685424251, 219.4504335181268289 ) ) ;
#68814=CARTESIAN_POINT ( 'NONE',  ( 7.898683012529999381, 1423.849047743189885, 212.3277966039590012 ) ) ;
#68815=CARTESIAN_POINT ( 'NONE',  ( -2.173216434189999990, 1456.191253960590075, 215.4656985532890019 ) ) ;
#68821=CARTESIAN_POINT ( 'NONE',  ( 8.062481262145620775, 1436.236301647820028, 206.1279573699050047 ) ) ;
#68837=CARTESIAN_POINT ( 'NONE',  ( 2.252366801017199993, 1445.834810329979973, 199.2768572914679908 ) ) ;
#68840=CARTESIAN_POINT ( 'NONE',  ( 4.492641941105749659, 1508.880976867409800, 206.0044425539609847 ) ) ;
#68842=CARTESIAN_POINT ( 'NONE',  ( -4.141018396419839931, 1508.551704408389924, 213.4853617037059905 ) ) ;
#68846=B_SPLINE_SURFACE_WITH_KNOTS ( 'NONE', 5, 5, ( 
 ( #70131, #84668, #110433, #7967, #61178, #16888 ),
 ( #42134, #67905, #34275, #68456, #104243, #94732 ),
 ( #85778, #26417, #102014, #10177, #44351, #9078 ),
 ( #59498, #60610, #51093, #52204, #9617, #43786 ),
 ( #69569, #35380, #103688, #26989, #95295, #88555 ),
 ( #91152, #62268, #96398, #45468, #2914, #44917 ),
 ( #105348, #65428, #97494, #105908, #20762, #40199 ),
 ( #37031, #19105, #74382, #80696, #63378, #36484 ),
 ( #46561, #79610, #28081, #80139, #99535, #54961 ) ),
 .UNSPECIFIED., .F., .F., .F.,
 ( 6, 3, 6 ),
 ( 6, 6 ),
 ( 14.15949905700000144, 24.81975873950000278, 34.67967148589999482 ),
 ( 0.000000000000000000, 2.000000000000000000 ),
 .UNSPECIFIED. ) ;
#68863=CARTESIAN_POINT ( 'NONE',  ( 8.389454068704580436, 1423.883216928779802, 211.4473611657970196 ) ) ;
#68864=CARTESIAN_POINT ( 'NONE',  ( -0.6927649375505723350, 1420.881850026484017, 193.7326374981037702 ) ) ;
#68865=CARTESIAN_POINT ( 'NONE',  ( -4.327986479516029661, 1515.120635733899917, 208.2727843191470072 ) ) ;
#68866=EDGE_CURVE ( 'NONE', #100464, #44452, #82126, .T. ) ;
#68874=CARTESIAN_POINT ( 'NONE',  ( -14.22051243745750071, 1421.364670842500118, 196.1737613524439894 ) ) ;
#68876=CARTESIAN_POINT ( 'NONE',  ( 10.03630746922679862, 1421.534750384480049, 198.5668548094549806 ) ) ;
#68881=CARTESIAN_POINT ( 'NONE',  ( -8.118430090829926726, 1425.413100047793023, 208.7305073936668691 ) ) ;
#68885=CARTESIAN_POINT ( 'NONE',  ( -1.114108910779999961, 1515.531799303389789, 205.0293305988190014 ) ) ;
#68888=CARTESIAN_POINT ( 'NONE',  ( 22.14279729195780178, 1473.984189419150198, 210.1089391048309949 ) ) ;
#68890=CARTESIAN_POINT ( 'NONE',  ( -15.99159030839580176, 1420.231971570089854, 209.2067213653590159 ) ) ;
#68899=ORIENTED_EDGE ( 'NONE', *, *, #96519, .F. ) ;
#68900=CARTESIAN_POINT ( 'NONE',  ( -11.41020920480000100, 1470.800728306390056, 208.9610728516699965 ) ) ;
#68905=CARTESIAN_POINT ( 'NONE',  ( -4.072722851587129433, 1432.588601696869773, 216.5672232244940005 ) ) ;
#68907=CARTESIAN_POINT ( 'NONE',  ( 1.842963219480119985, 1515.064792700640055, 213.4512947425059792 ) ) ;
#68908=DIRECTION ( 'NONE',  ( 0.9361323810649732069, 0.3043587179164370382, 0.1761304515121860370 ) ) ;
#68917=ORIENTED_EDGE ( 'NONE', *, *, #2209, .T. ) ;
#68921=CARTESIAN_POINT ( 'NONE',  ( -18.56563103275550120, 1441.651807245909822, 211.5798049646579955 ) ) ;
#68923=CARTESIAN_POINT ( 'NONE',  ( -6.192225852249999996, 1496.322100554489907, 199.7152199997689763 ) ) ;
#68936=CARTESIAN_POINT ( 'NONE',  ( -1.337955765360000049, 1494.783074254390158, 220.2332542844989973 ) ) ;
#68951=CARTESIAN_POINT ( 'NONE',  ( -5.236048985779999221, 1391.923671604790115, 214.6057402034190034 ) ) ;
#68955=CARTESIAN_POINT ( 'NONE',  ( 9.505847783012139729, 1461.812439321519832, 207.0696516400899725 ) ) ;
#68962=VERTEX_POINT ( 'NONE', #38585 ) ;
#68964=CARTESIAN_POINT ( 'NONE',  ( -10.34027448514628489, 1418.149532852553193, 197.7030072931336235 ) ) ;
#68965=CARTESIAN_POINT ( 'NONE',  ( -0.7790226144181949808, 1442.687261678630193, 200.2740145696140246 ) ) ;
#68969=CARTESIAN_POINT ( 'NONE',  ( 9.628418581815711974, 1451.441045534420027, 207.9857633263249852 ) ) ;
#68980=CARTESIAN_POINT ( 'NONE',  ( -7.087060292473280398, 1508.534494050320063, 219.4009365383440127 ) ) ;
#68987=CARTESIAN_POINT ( 'NONE',  ( -5.898813458170000246, 1474.065724237490031, 199.2881457417290108 ) ) ;
#68992=CARTESIAN_POINT ( 'NONE',  ( 6.726720322338469948, 1467.543326730849913, 200.2279294393160001 ) ) ;
#68994=DIRECTION ( 'NONE',  ( -0.1455443991891719746, -0.4512270418750849443, -0.8804606660977668531 ) ) ;
#68995=CARTESIAN_POINT ( 'NONE',  ( -9.789280099085180709, 1501.631186488149979, 228.6396568906859841 ) ) ;
#68998=DIRECTION ( 'NONE',  ( -9.341989762165448955E-47, 1.000000000000000000, -1.836970198721029688E-16 ) ) ;
#69001=CARTESIAN_POINT ( 'NONE',  ( 1.273031542862190113, 1515.087982642930001, 204.7930044310420215 ) ) ;
#69007=CARTESIAN_POINT ( 'NONE',  ( -10.96786518298100077, 1462.082438629349781, 210.1872772324369976 ) ) ;
#69012=CARTESIAN_POINT ( 'NONE',  ( -11.00420836870640073, 1481.586346291950122, 208.5478340898509657 ) ) ;
#69023=CARTESIAN_POINT ( 'NONE',  ( -15.15027404274539968, 1418.004900903659973, 203.1594184435460022 ) ) ;
#69032=CARTESIAN_POINT ( 'NONE',  ( -7.898270967410000232, 1498.870872765589866, 219.0971900149289979 ) ) ;
#69036=CARTESIAN_POINT ( 'NONE',  ( -12.91325991995259947, 1507.673968524629800, 209.2392918421849970 ) ) ;
#69047=CARTESIAN_POINT ( 'NONE',  ( 4.324092179320000007, 1515.269353058490196, 209.1218459616989946 ) ) ;
#69051=( BOUNDED_CURVE ( )  B_SPLINE_CURVE ( 3, ( #46441, #20102, #20634, #54294 ),
 .UNSPECIFIED., .F., .F. ) 
 B_SPLINE_CURVE_WITH_KNOTS ( ( 4, 4 ),
 ( 5.498078028609830525, 7.068189169012200068 ),
 .UNSPECIFIED. ) 
 CURVE ( )  GEOMETRIC_REPRESENTATION_ITEM ( )  RATIONAL_B_SPLINE_CURVE ( ( 1.000000000000000000, 0.8048993264383194068, 0.8048993264383194068, 1.000000000000000000 ) ) 
 REPRESENTATION_ITEM ( '' )  );
#69053=CARTESIAN_POINT ( 'NONE',  ( 4.998913908720000521, 1484.124591968289906, 219.8555354240990027 ) ) ;
#69056=CARTESIAN_POINT ( 'NONE',  ( 5.371360332529999226, 1437.823705336689954, 228.7343661627989775 ) ) ;
#69058=CARTESIAN_POINT ( 'NONE',  ( -0.3862240865043620186, 1500.063269132039977, 233.1571802061429821 ) ) ;
#69061=CARTESIAN_POINT ( 'NONE',  ( 8.481739720359620094, 1422.818663224589727, 213.7027558147750028 ) ) ;
#69062=CARTESIAN_POINT ( 'NONE',  ( 9.820661198562449457, 1435.530196802239971, 209.1647375191699894 ) ) ;
#69063=CARTESIAN_POINT ( 'NONE',  ( -11.28649141220000018, 1489.673453124989919, 212.4368142099590102 ) ) ;
#69065=CARTESIAN_POINT ( 'NONE',  ( -19.27355791249999939, 1467.813399981289876, 204.3088842694490097 ) ) ;
#69074=EDGE_LOOP ( 'NONE', ( #72702, #74586, #12816, #68628 ) ) ;
#69078=ORIENTED_EDGE ( 'NONE', *, *, #34423, .F. ) ;
#69081=CARTESIAN_POINT ( 'NONE',  ( 3.368596972436100234, 1515.551842520359969, 205.3433046317179844 ) ) ;
#69086=CARTESIAN_POINT ( 'NONE',  ( 2.770834604750000096, 1467.540123119690179, 218.8375473850189792 ) ) ;
#69094=CARTESIAN_POINT ( 'NONE',  ( -0.2691619379491070330, 1432.197445330879873, 200.7020891982060107 ) ) ;
#69095=VERTEX_POINT ( 'NONE', #15023 ) ;
#69099=CARTESIAN_POINT ( 'NONE',  ( -5.559835380637566438, 1475.920404062059333, 200.3847495419848030 ) ) ;
#69101=CARTESIAN_POINT ( 'NONE',  ( -1.991394312995570015, 1465.005291665100003, 198.2980544129180203 ) ) ;
#69103=CARTESIAN_POINT ( 'NONE',  ( 11.66548674282380027, 1421.980630269289804, 209.5620691455910105 ) ) ;
#69105=CARTESIAN_POINT ( 'NONE',  ( 2.773997830410000365, 1465.987719246390043, 198.8503135595989875 ) ) ;
#69118=CARTESIAN_POINT ( 'NONE',  ( -18.13023266204549699, 1508.551704408389924, 210.4115160111289811 ) ) ;
#69119=CARTESIAN_POINT ( 'NONE',  ( -4.038582000520636761, 1515.598601297060668, 208.8111433043314946 ) ) ;
#69122=CARTESIAN_POINT ( 'NONE',  ( -2.710325452122229972, 1429.081471984569816, 200.1517093420179947 ) ) ;
#69137=CARTESIAN_POINT ( 'NONE',  ( 7.348570800660000124, 1422.803073198840139, 195.5677875354990078 ) ) ;
#69140=CARTESIAN_POINT ( 'NONE',  ( -10.37115945647730086, 1448.032435977620025, 209.0451274022370001 ) ) ;
#69148=CARTESIAN_POINT ( 'NONE',  ( 3.432220944640000049, 1466.863758737489889, 218.8549222279790172 ) ) ;
#69153=CARTESIAN_POINT ( 'NONE',  ( -2.123092008920000051, 1429.895782721190017, 200.6928439449890220 ) ) ;
#69154=EDGE_CURVE ( 'NONE', #9541, #69447, #83901, .T. ) ;
#69155=CARTESIAN_POINT ( 'NONE',  ( 10.43348778195679927, 1481.587817364219973, 210.8845854110620053 ) ) ;
#69156=CARTESIAN_POINT ( 'NONE',  ( 3.826065771026290196, 1507.355962757600082, 220.1845845182679966 ) ) ;
#69164=CARTESIAN_POINT ( 'NONE',  ( 11.57530253989999913, 1501.342159807790040, 208.5271154974659851 ) ) ;
#69167=CARTESIAN_POINT ( 'NONE',  ( 8.214113159060000058, 1423.929736563989991, 211.6354375824689953 ) ) ;
#69172=CARTESIAN_POINT ( 'NONE',  ( -5.192564606620000411, 1483.459670744789946, 199.8090169432990137 ) ) ;
#69180=CARTESIAN_POINT ( 'NONE',  ( 0.3839115268003259751, 1435.761583004419890, 227.5864344777720021 ) ) ;
#69181=CARTESIAN_POINT ( 'NONE',  ( -14.89207660494735386, 1416.116151593460017, 205.0818956363123675 ) ) ;
#69183=CARTESIAN_POINT ( 'NONE',  ( -0.4823735185300109807, 1457.129037944750053, 219.7424419883419944 ) ) ;
#69186=EDGE_CURVE ( 'NONE', #8260, #54763, #103540, .T. ) ;
#69188=CARTESIAN_POINT ( 'NONE',  ( 7.894362808210001248, 1424.028044848189893, 212.1595859666189767 ) ) ;
#69189=CARTESIAN_POINT ( 'NONE',  ( -8.627754863869999014, 1437.492696374190018, 228.3379673428989918 ) ) ;
#69195=ORIENTED_EDGE ( 'NONE', *, *, #83, .T. ) ;
#69210=ORIENTED_EDGE ( 'NONE', *, *, #70737, .F. ) ;
#69220=ORIENTED_EDGE ( 'NONE', *, *, #94766, .F. ) ;
#69223=EDGE_CURVE ( 'NONE', #91400, #29545, #96819, .T. ) ;
#69228=EDGE_CURVE ( 'NONE', #7587, #86208, #34136, .T. ) ;
#69238=CARTESIAN_POINT ( 'NONE',  ( 19.33081166079999846, 1455.566665276290223, 210.0606673158609965 ) ) ;
#69246=CARTESIAN_POINT ( 'NONE',  ( -6.068033889650000567, 1450.398953434090117, 208.9968551374399794 ) ) ;
#69262=EDGE_CURVE ( 'NONE', #82048, #52413, #51389, .T. ) ;
#69266=CARTESIAN_POINT ( 'NONE',  ( 11.55221588404359956, 1480.217597516799970, 211.4789165460060190 ) ) ;
#69269=TOROIDAL_SURFACE ( 'NONE', #12020, 12.73448142120000171, 1.000000000000000000 ) ;
#69277=CARTESIAN_POINT ( 'NONE',  ( 2.999854733669999884, 1441.831681250090014, 217.8331532265690100 ) ) ;
#69283=CARTESIAN_POINT ( 'NONE',  ( 8.820344574085469347, 1461.063527266820074, 204.9905474934919880 ) ) ;
#69286=CARTESIAN_POINT ( 'NONE',  ( -9.141596155196140217, 1420.494364209170044, 195.3822545821539904 ) ) ;
#69295=CARTESIAN_POINT ( 'NONE',  ( 9.651066088509999474, 1425.440658930580184, 195.4941615409990163 ) ) ;
#69296=CARTESIAN_POINT ( 'NONE',  ( -10.51265743563710053, 1480.030739721740019, 208.9489006321179829 ) ) ;
#69299=EDGE_CURVE ( 'NONE', #43306, #52400, #33028, .T. ) ;
#69300=CARTESIAN_POINT ( 'NONE',  ( -3.895893481806210090, 1487.443163804099868, 219.7113992567399805 ) ) ;
#69301=CARTESIAN_POINT ( 'NONE',  ( 18.28863238269999769, 1430.119121229389975, 201.0315571599689974 ) ) ;
#69308=VERTEX_POINT ( 'NONE', #58258 ) ;
#69313=ORIENTED_EDGE ( 'NONE', *, *, #92146, .F. ) ;
#69332=DIRECTION ( 'NONE',  ( -0.9158452764874773777, 0.3011522798863591199, -0.2655837605254210976 ) ) ;
#69334=CARTESIAN_POINT ( 'NONE',  ( -3.747824384279149879, 1508.879013859839915, 213.3683195021539802 ) ) ;
#69335=CARTESIAN_POINT ( 'NONE',  ( -13.43693033329999764, 1470.316141799590014, 192.0299142216990163 ) ) ;
#69342=CARTESIAN_POINT ( 'NONE',  ( -2.131219751997940115, 1421.405227258459945, 193.6669010562050062 ) ) ;
#69350=CARTESIAN_POINT ( 'NONE',  ( -8.205225261000000714, 1424.128567649279830, 209.5451383975179738 ) ) ;
#69356=CARTESIAN_POINT ( 'NONE',  ( 7.527384429723530168, 1425.477955340190192, 212.1953674759300270 ) ) ;
#69365=CARTESIAN_POINT ( 'NONE',  ( -18.89253822837050123, 1508.457456783149837, 210.4078925326670060 ) ) ;
#69366=EDGE_CURVE ( 'NONE', #66058, #102270, #7429, .T. ) ;
#69388=CARTESIAN_POINT ( 'NONE',  ( -3.670436692600000050, 1428.951561624590113, 201.2856071730990095 ) ) ;
#69394=EDGE_LOOP ( 'NONE', ( #57127, #65320, #53251, #104878 ) ) ;
#69401=CARTESIAN_POINT ( 'NONE',  ( -4.164270815259999203, 1497.128533180889917, 198.6585142336989804 ) ) ;
#69403=CARTESIAN_POINT ( 'NONE',  ( -1.073559340110749938, 1444.993510080170154, 218.0402162255370229 ) ) ;
#69410=EDGE_CURVE ( 'NONE', #36343, #72135, #19460, .T. ) ;
#69416=CARTESIAN_POINT ( 'NONE',  ( -8.668122330615428695, 1484.012669316429992, 200.9602178716519916 ) ) ;
#69418=CARTESIAN_POINT ( 'NONE',  ( -20.05314457115955307, 1508.136158586383772, 209.6329359176547484 ) ) ;
#69419=CARTESIAN_POINT ( 'NONE',  ( 2.799112436247476854, 1421.785673600051723, 193.9260731165295226 ) ) ;
#69420=CARTESIAN_POINT ( 'NONE',  ( -10.73398234689440045, 1462.915869440839970, 206.4721582478690038 ) ) ;
#69425=CARTESIAN_POINT ( 'NONE',  ( -9.642181709647690724, 1460.678695209409852, 208.4214907479299939 ) ) ;
#69426=CARTESIAN_POINT ( 'NONE',  ( -9.198431329101820708, 1421.868764589120246, 192.2153590489439807 ) ) ;
#69427=CARTESIAN_POINT ( 'NONE',  ( 10.00923256885409884, 1425.484835869890048, 195.7305245570549914 ) ) ;
#69428=CARTESIAN_POINT ( 'NONE',  ( 10.36623042182900178, 1462.084445524129933, 211.0499476876460108 ) ) ;
#69437=CARTESIAN_POINT ( 'NONE',  ( -13.32684193225579961, 1469.522593795099965, 191.9925906374970168 ) ) ;
#69439=CARTESIAN_POINT ( 'NONE',  ( -13.19880346797889992, 1421.769212956930232, 206.7699246856669788 ) ) ;
#69445=CARTESIAN_POINT ( 'NONE',  ( -4.293363079010000583, 1475.442267412990077, 199.5995467683989943 ) ) ;
#69447=VERTEX_POINT ( 'NONE', #71798 ) ;
#69448=CARTESIAN_POINT ( 'NONE',  ( -3.406331129536729563, 1508.551704408389924, 219.9476367669959984 ) ) ;
#69458=CARTESIAN_POINT ( 'NONE',  ( -10.57308237661970018, 1471.786795378390025, 206.9537732482530146 ) ) ;
#69466=DIRECTION ( 'NONE',  ( -9.500914144214121536E-47, 1.000000000000000000, -1.836970198721029688E-16 ) ) ;
#69468=CARTESIAN_POINT ( 'NONE',  ( 6.030521501068090373, 1467.020543277260003, 217.0291475865519999 ) ) ;
#69469=EDGE_LOOP ( 'NONE', ( #73742, #23109, #37010, #9256 ) ) ;
#69470=CARTESIAN_POINT ( 'NONE',  ( 6.055110513760000757, 1450.647404142589949, 209.2214892968010247 ) ) ;
#69472=CARTESIAN_POINT ( 'NONE',  ( -10.05915832670000043, 1494.201315354589951, 204.1613691274089888 ) ) ;
#69480=CARTESIAN_POINT ( 'NONE',  ( 1.269526426719999934, 1457.689347263989930, 199.6687966702490087 ) ) ;
#69485=CARTESIAN_POINT ( 'NONE',  ( -2.021380015520000129, 1496.949193287590106, 197.9094991689989911 ) ) ;
#69502=EDGE_CURVE ( 'NONE', #109440, #23969, #56472, .T. ) ;
#69503=CARTESIAN_POINT ( 'NONE',  ( -5.093521796410000135, 1391.866579497489965, 214.5262673350590035 ) ) ;
#69505=ORIENTED_EDGE ( 'NONE', *, *, #4527, .F. ) ;
#69507=CARTESIAN_POINT ( 'NONE',  ( 9.226870674553810048, 1461.939016979510143, 206.0483255767620108 ) ) ;
#69515=ORIENTED_EDGE ( 'NONE', *, *, #27283, .T. ) ;
#69518=CARTESIAN_POINT ( 'NONE',  ( -14.73770141384289900, 1508.451171878049990, 209.7916384116149970 ) ) ;
#69523=CARTESIAN_POINT ( 'NONE',  ( 9.248740396683809095, 1450.941274981350034, 208.9745031941699835 ) ) ;
#69529=VERTEX_POINT ( 'NONE', #101193 ) ;
#69532=ORIENTED_EDGE ( 'NONE', *, *, #63153, .F. ) ;
#69536=CARTESIAN_POINT ( 'NONE',  ( -9.042214778654647844, 1490.548019693297647, 215.3561743177068308 ) ) ;
#69540=CARTESIAN_POINT ( 'NONE',  ( -6.325873692910000123, 1474.305489392889967, 200.4708573935690197 ) ) ;
#69541=CARTESIAN_POINT ( 'NONE',  ( 11.41833521740000101, 1492.743966703789738, 212.4764450907990181 ) ) ;
#69544=CARTESIAN_POINT ( 'NONE',  ( -20.79256037440000071, 1505.243615344689943, 209.5690373176560115 ) ) ;
#69545=CARTESIAN_POINT ( 'NONE',  ( 9.607386820528988736, 1468.930745809150039, 203.2606402744570175 ) ) ;
#69552=B_SPLINE_SURFACE_WITH_KNOTS ( 'NONE', 5, 5, ( 
 ( #80352, #53511, #3669, #55169, #89294, #12590 ),
 ( #4731, #98239, #45115, #46769, #80899, #64118 ),
 ( #21510, #55722, #38875, #104440, #61922, #2567 ),
 ( #70883, #104996, #96038, #19309, #28286, #15323 ),
 ( #66875, #74170, #49517, #6396, #5851, #23177 ),
 ( #47846, #100985, #107196, #99326, #41093, #108299 ),
 ( #74717, #75272, #84195, #98791, #99878, #57378 ),
 ( #83641, #39992, #32144, #31584, #32695, #109419 ),
 ( #65762, #23731, #66331, #64673, #73054, #91504 ) ),
 .UNSPECIFIED., .F., .F., .F.,
 ( 6, 3, 6 ),
 ( 6, 6 ),
 ( 13.48398407686089939, 16.53063851469999790, 19.57724985460000156 ),
 ( -9.649567376679359532E-06, 2.000042901542320006 ),
 .UNSPECIFIED. ) ;
#69557=CARTESIAN_POINT ( 'NONE',  ( 1.403832663128229852, 1515.079617817420058, 204.7927853908689997 ) ) ;
#69559=CARTESIAN_POINT ( 'NONE',  ( -15.76868314863217080, 1415.798507515539768, 209.6929715414478039 ) ) ;
#69564=LINE ( 'NONE', #43239, #41975 ) ;
#69566=CARTESIAN_POINT ( 'NONE',  ( -2.188078410709979771, 1508.020976590390092, 220.9453026643990086 ) ) ;
#69569=CARTESIAN_POINT ( 'NONE',  ( -8.131139148520000859, 1477.102955269890117, 215.8146692214089910 ) ) ;
#69592=CARTESIAN_POINT ( 'NONE',  ( -12.96253978517979988, 1508.551708299209849, 210.0000646660610073 ) ) ;
#69603=B_SPLINE_CURVE_WITH_KNOTS ( 'NONE', 3,
 ( #73919, #91256, #6697, #101840, #101279, #100210, #85049, #15077, #34104, #91799, #24023, #8339, #84507, #93447, #24575, #25134, #59337, #42503, #41962, #76116 ),
 .UNSPECIFIED., .F., .F.,
 ( 4, 2, 2, 2, 1, 1, 1, 1, 2, 2, 2, 4 ),
 ( 0.000000000000000000, 0.2500000000006933898, 0.3750000000010487722, 0.4375000000012101986, 0.4687500000012878587, 0.4843750000013154478, 0.4921875000013438695, 0.4960937500013579138, 0.4980468750013504198, 0.5000000000013429258, 0.7500000000006714629, 1.000000000000000000 ),
 .UNSPECIFIED. ) ;
#69604=CARTESIAN_POINT ( 'NONE',  ( -9.687216859550042969, 1494.456727822050880, 203.5511929442279779 ) ) ;
#69605=CARTESIAN_POINT ( 'NONE',  ( 4.091781189549999809, 1515.531881637889910, 208.0020576612490117 ) ) ;
#69609=CARTESIAN_POINT ( 'NONE',  ( 5.161034791280000533, 1485.814572579490005, 218.5690567784690188 ) ) ;
#69610=CARTESIAN_POINT ( 'NONE',  ( 10.85852436008239863, 1479.618465607619783, 207.8019171430970005 ) ) ;
#69612=CARTESIAN_POINT ( 'NONE',  ( 10.41726918004940039, 1452.895226299490105, 190.0448634872510354 ) ) ;
#69614=CARTESIAN_POINT ( 'NONE',  ( -21.51339057085170126, 1505.551704407249872, 209.1218459615049881 ) ) ;
#69617=CARTESIAN_POINT ( 'NONE',  ( -4.994992779129999505, 1391.721842640289879, 203.5951896846190152 ) ) ;
#69618=DIRECTION ( 'NONE',  ( 0.2803360189751119558, -0.4513760013199308863, -0.8471548984085587319 ) ) ;
#69619=CARTESIAN_POINT ( 'NONE',  ( -10.84352170600000242, 1490.621361297190106, 211.6123805837090117 ) ) ;
#69623=CARTESIAN_POINT ( 'NONE',  ( 0.000000000000000000, 1399.332476024090056, 209.1218459616989946 ) ) ;
#69627=CARTESIAN_POINT ( 'NONE',  ( 6.687607498646199744, 1504.526125536900054, 220.0428038810069893 ) ) ;
#69636=CARTESIAN_POINT ( 'NONE',  ( 0.7518804359284473326, 1457.963929617798613, 199.6002294408864088 ) ) ;
#69637=CARTESIAN_POINT ( 'NONE',  ( -10.23096445512489971, 1448.798712686370209, 207.3500612127919851 ) ) ;
#69644=CARTESIAN_POINT ( 'NONE',  ( 2.995626829160000337, 1468.394067435089937, 218.6771455671389788 ) ) ;
#69646=EDGE_CURVE ( 'NONE', #102504, #76431, #87526, .T. ) ;
#69650=CARTESIAN_POINT ( 'NONE',  ( -7.022715574297880181, 1424.820957301160206, 207.8595816151610336 ) ) ;
#69659=CARTESIAN_POINT ( 'NONE',  ( 21.13734888319999783, 1496.938803861589804, 209.1218459616989946 ) ) ;
#69661=CARTESIAN_POINT ( 'NONE',  ( -0.4364796396607459328, 1465.308788633660015, 198.1255561066119810 ) ) ;
#69663=CARTESIAN_POINT ( 'NONE',  ( 11.51161966288469962, 1422.036711861869890, 209.8677670191129891 ) ) ;
#69679=CARTESIAN_POINT ( 'NONE',  ( 2.727717259937589844, 1423.594114422599887, 192.7156380009489851 ) ) ;
#69680=CARTESIAN_POINT ( 'NONE',  ( 0.005666290841312040041, 1455.183973234658879, 218.5515631892139083 ) ) ;
#69683=DIRECTION ( 'NONE',  ( -0.9236849191514725499, -0.3806575521132582463, -0.04365773873301222185 ) ) ;
#69687=B_SPLINE_SURFACE_WITH_KNOTS ( 'NONE', 5, 5, ( 
 ( #52120, #86248, #16267, #94652, #51559, #59424 ),
 ( #9539, #43162, #1169, #84593, #44271, #77317 ),
 ( #67821, #35300, #101933, #25220, #93536, #615 ),
 ( #16807, #34747, #69485, #51009, #85142, #8430 ),
 ( #26907, #61096, #42600, #76756, #105264, #97950 ),
 ( #45925, #54338, #4471, #10664, #71713, #78985 ),
 ( #87933, #3934, #54880, #2288, #38599, #21218 ),
 ( #29651, #45385, #72779, #63295, #106366, #80618 ),
 ( #3381, #38061, #105831, #37509, #104707, #36946 ) ),
 .UNSPECIFIED., .F., .F., .F.,
 ( 6, 3, 6 ),
 ( 6, 6 ),
 ( 4.164915011539999767, 8.224269361119999289, 13.59025040360000069 ),
 ( 0.000000000000000000, 2.000000000000000000 ),
 .UNSPECIFIED. ) ;
#69693=CARTESIAN_POINT ( 'NONE',  ( -11.84714928711539983, 1482.159292582530043, 208.0957396826470074 ) ) ;
#69715=CARTESIAN_POINT ( 'NONE',  ( -19.80095844739999933, 1467.038543526389958, 210.3340861277090141 ) ) ;
#69721=CARTESIAN_POINT ( 'NONE',  ( 0.8853928803100010736, 1430.729413004489970, 199.7003955947189979 ) ) ;
#69722=CARTESIAN_POINT ( 'NONE',  ( 10.94008111561099916, 1480.254962643290128, 209.9041328597590166 ) ) ;
#69723=CARTESIAN_POINT ( 'NONE',  ( 2.705175745250000041, 1507.754439583389967, 220.5492045685990092 ) ) ;
#69729=CARTESIAN_POINT ( 'NONE',  ( 9.817221195247329391, 1469.134009909099859, 205.3197251424940077 ) ) ;
#69731=CARTESIAN_POINT ( 'NONE',  ( 11.47878270300000025, 1502.051335001390044, 209.2507985867119942 ) ) ;
#69733=CARTESIAN_POINT ( 'NONE',  ( 7.503281267020000200, 1424.102137712849981, 212.3377160795290024 ) ) ;
#69737=CARTESIAN_POINT ( 'NONE',  ( -10.06499266109999979, 1481.481387821690078, 205.8730048975889986 ) ) ;
#69743=ORIENTED_EDGE ( 'NONE', *, *, #103785, .T. ) ;
#69748=CARTESIAN_POINT ( 'NONE',  ( 0.5343213467924259330, 1456.848408503409928, 219.7312664301520044 ) ) ;
#69753=CARTESIAN_POINT ( 'NONE',  ( 7.724069020439999989, 1425.270033306300093, 211.8061983222289939 ) ) ;
#69754=CARTESIAN_POINT ( 'NONE',  ( 0.9103409915569969924, 1462.760008604990162, 230.5111369474990113 ) ) ;
#69755=B_SPLINE_CURVE_WITH_KNOTS ( 'NONE', 3,
 ( #44403, #85264, #52255, #76892, #43294, #202, #77442, #34325, #77985, #18603, #25348, #103739, #94217, #16936, #52803, #78545, #17492, #103163, #69062, #42181, #1291, #27040, #35431, #35994, #70184 ),
 .UNSPECIFIED., .F., .F.,
 ( 4, 3, 3, 3, 3, 3, 3, 3, 4 ),
 ( -14.84821972146360025, -14.69753164292139935, -14.02977699588210037, -13.36301733525779945, -12.71109731192579950, -12.40463753468570118, -11.81983018498929994, -11.09617899401849961, -10.57397516620000033 ),
 .UNSPECIFIED. ) ;
#69760=CARTESIAN_POINT ( 'NONE',  ( 7.333575610579999626, 1455.004670275590115, 216.8632114976190053 ) ) ;
#69769=DIRECTION ( 'NONE',  ( 9.500914144214121536E-47, -1.000000000000000000, 1.836970198721029688E-16 ) ) ;
#69782=FACE_OUTER_BOUND ( 'NONE', #103196, .T. ) ;
#69792=B_SPLINE_SURFACE_WITH_KNOTS ( 'NONE', 5, 5, ( 
 ( #68488, #69047, #41616, #109381, #60644, #6896 ),
 ( #66835, #100945, #58422, #92548, #15816, #44389 ),
 ( #19139, #3496, #1277, #61751, #54457, #103723 ),
 ( #80181, #77970, #35417, #95874, #69605, #96994 ),
 ( #35978, #86921, #27025, #62310, #62882, #104831 ),
 ( #53344, #20257, #78532, #61213, #36523, #37623 ) ),
 .UNSPECIFIED., .F., .F., .F.,
 ( 6, 6 ),
 ( 6, 6 ),
 ( 4.991132198209999871, 7.657648704760000591 ),
 ( 0.000000000000000000, 0.5000000000000000000 ),
 .UNSPECIFIED. ) ;
#69817=EDGE_LOOP ( 'NONE', ( #54577, #24078, #34708, #38619, #7499, #76207, #66377 ) ) ;
#69837=CARTESIAN_POINT ( 'NONE',  ( 4.814474515349520090, 1424.592626270299888, 191.7967880341639955 ) ) ;
#69846=CARTESIAN_POINT ( 'NONE',  ( 5.823572337359999906, 1487.975078907890065, 198.5964445195989754 ) ) ;
#69847=CARTESIAN_POINT ( 'NONE',  ( -5.007591594161714177, 1391.741091803201698, 203.5445219108341632 ) ) ;
#69851=CARTESIAN_POINT ( 'NONE',  ( -4.679791067032079255, 1508.610720099250102, 212.2979123687669869 ) ) ;
#69857=CARTESIAN_POINT ( 'NONE',  ( -10.27696724499340064, 1491.210326720090052, 213.0881471566560208 ) ) ;
#69861=ADVANCED_FACE ( 'NONE', ( #108515 ), #43511, .F. ) ;
#69870=EDGE_CURVE ( 'NONE', #41661, #75670, #51342, .T. ) ;
#69871=CARTESIAN_POINT ( 'NONE',  ( -14.81767606095329981, 1417.858166622450199, 213.3262279172620026 ) ) ;
#69879=FACE_OUTER_BOUND ( 'NONE', #101388, .T. ) ;
#69886=CARTESIAN_POINT ( 'NONE',  ( -9.147922398094991081, 1449.650533038000049, 209.9742684363969829 ) ) ;
#69887=CARTESIAN_POINT ( 'NONE',  ( -10.30332664446770075, 1423.841252421040053, 204.4542459073049940 ) ) ;
#69890=CARTESIAN_POINT ( 'NONE',  ( 2.125574643609999814, 1472.895346367389948, 219.1091941688290206 ) ) ;
#69893=CARTESIAN_POINT ( 'NONE',  ( 22.18328064218600204, 1474.773901063470021, 209.9706487204360030 ) ) ;
#69900=CARTESIAN_POINT ( 'NONE',  ( -20.59725329420000151, 1484.571939645490147, 210.1086304389179986 ) ) ;
#69903=EDGE_CURVE ( 'NONE', #93900, #22042, #59342, .T. ) ;
#69904=VECTOR ( 'NONE', #19728, 999.9999999999998863 ) ;
#69915=CARTESIAN_POINT ( 'NONE',  ( -9.041223454946500482, 1447.413830056329971, 212.1276203665690048 ) ) ;
#69916=CARTESIAN_POINT ( 'NONE',  ( -6.777304992429280084, 1470.983459794990495, 216.6342898665807297 ) ) ;
#69918=CARTESIAN_POINT ( 'NONE',  ( -2.842752294796690116, 1497.021273686229961, 221.1752333403379964 ) ) ;
#69923=CARTESIAN_POINT ( 'NONE',  ( 3.959152859930000101, 1428.396642669490120, 216.3690266601789745 ) ) ;
#69925=CARTESIAN_POINT ( 'NONE',  ( -17.26078256985329773, 1508.541932187329849, 212.5336323307500095 ) ) ;
#69927=CARTESIAN_POINT ( 'NONE',  ( -8.769340852563940913, 1438.886933218489958, 207.8278986470189977 ) ) ;
#69950=EDGE_LOOP ( 'NONE', ( #18272, #2056, #5725, #12329 ) ) ;
#69951=CARTESIAN_POINT ( 'NONE',  ( 3.892696960845567045, 1515.551704300027950, 207.5713754906064707 ) ) ;
#69957=CARTESIAN_POINT ( 'NONE',  ( -3.786785403780000170, 1495.627531097190058, 197.8060809205989869 ) ) ;
#69971=CARTESIAN_POINT ( 'NONE',  ( -8.270734047218098794, 1484.136534094920080, 200.5535876571919971 ) ) ;
#69973=CARTESIAN_POINT ( 'NONE',  ( 12.50011566148209852, 1426.394375987810236, 202.7337349580159866 ) ) ;
#69975=CARTESIAN_POINT ( 'NONE',  ( -4.327012391429009952, 1515.157834657069998, 208.9940569023019918 ) ) ;
#69982=CARTESIAN_POINT ( 'NONE',  ( -16.83566772702310033, 1418.884435451930131, 201.2565165529269962 ) ) ;
#69983=CARTESIAN_POINT ( 'NONE',  ( 0.000000000000000000, 1414.421228241719973, 209.1218459616989946 ) ) ;
#69988=CARTESIAN_POINT ( 'NONE',  ( -0.9161335898489990637, 1443.103187093389806, 200.2678566797989959 ) ) ;
#69992=CARTESIAN_POINT ( 'NONE',  ( -16.98954224973644145, 1419.974429067340452, 207.7469223126931297 ) ) ;
#69996=CARTESIAN_POINT ( 'NONE',  ( 9.738317455238711062, 1493.400073354660208, 188.2659979897460119 ) ) ;
#69998=CARTESIAN_POINT ( 'NONE',  ( 9.176228414599330918, 1450.984694443030094, 210.2421773183669984 ) ) ;
#70000=CARTESIAN_POINT ( 'NONE',  ( 5.246794622849999534, 1436.700339732089788, 207.6218553049789932 ) ) ;
#70001=EDGE_LOOP ( 'NONE', ( #53255, #39166, #50899, #63196 ) ) ;
#70005=CARTESIAN_POINT ( 'NONE',  ( -4.352858573179999802, 1475.884254538489813, 199.7486192038290085 ) ) ;
#70007=ORIENTED_EDGE ( 'NONE', *, *, #95289, .F. ) ;
#70008=CARTESIAN_POINT ( 'NONE',  ( -7.055342795364590636, 1508.551704404470001, 219.1733338826510078 ) ) ;
#70016=CARTESIAN_POINT ( 'NONE',  ( 0.9870939535439990919, 1430.542140937089926, 217.5404060487589959 ) ) ;
#70022=CARTESIAN_POINT ( 'NONE',  ( 11.34606461758039941, 1422.095439081570021, 210.1857495716350002 ) ) ;
#70026=CARTESIAN_POINT ( 'NONE',  ( 11.62672742097220002, 1491.248664925870116, 206.9181316795630039 ) ) ;
#70029=CARTESIAN_POINT ( 'NONE',  ( 8.495474403110010897, 1465.434214291670060, 214.1564210924720157 ) ) ;
#70034=CARTESIAN_POINT ( 'NONE',  ( -0.3263949288959780426, 1496.478667861620124, 196.7673131782539997 ) ) ;
#70050=CARTESIAN_POINT ( 'NONE',  ( -3.148245054199999782, 1496.969444965490084, 220.6920657697990009 ) ) ;
#70059=AXIS2_PLACEMENT_3D ( 'NONE', #82160, #13838, #5459 ) ;
#70064=CARTESIAN_POINT ( 'NONE',  ( -4.992349863779999453, 1391.620913471789891, 214.4932724168290008 ) ) ;
#70068=CARTESIAN_POINT ( 'NONE',  ( 10.41193553163299867, 1460.804056526489831, 207.7426899176469988 ) ) ;
#70071=EDGE_LOOP ( 'NONE', ( #26020, #31608, #71018, #100227 ) ) ;
#70073=CARTESIAN_POINT ( 'NONE',  ( 8.079271929000000796, 1423.284668454760094, 195.9721669254989820 ) ) ;
#70081=CARTESIAN_POINT ( 'NONE',  ( 9.922915408476299604, 1451.489621189869695, 207.3832923455570096 ) ) ;
#70082=CARTESIAN_POINT ( 'NONE',  ( 2.835697453489999909, 1501.613331751589840, 230.3199997588990016 ) ) ;
#70093=CARTESIAN_POINT ( 'NONE',  ( -7.744919283042880132, 1508.476290139939920, 219.4107736818559999 ) ) ;
#70095=CARTESIAN_POINT ( 'NONE',  ( -9.120463652338420601, 1471.255923615639858, 213.5777534691339952 ) ) ;
#70100=CARTESIAN_POINT ( 'NONE',  ( -2.465027318521849864, 1422.346290854769904, 192.7050527383619851 ) ) ;
#70103=CARTESIAN_POINT ( 'NONE',  ( -14.90880384090000099, 1503.968912916589943, 208.7967653244450048 ) ) ;
#70108=CARTESIAN_POINT ( 'NONE',  ( -6.115766451680039850, 1497.554681153639876, 215.1697308089790113 ) ) ;
#70114=CARTESIAN_POINT ( 'NONE',  ( 3.837812054080000035, 1506.875571340089891, 220.1607364553989896 ) ) ;
#70117=CARTESIAN_POINT ( 'NONE',  ( 1.364625987975899735, 1515.082030188910039, 204.7928485609430140 ) ) ;
#70119=CARTESIAN_POINT ( 'NONE',  ( -15.68073676374516445, 1415.733564152250437, 209.6599020335900150 ) ) ;
#70125=CARTESIAN_POINT ( 'NONE',  ( 0.8076263318534745439, 1444.250888050305093, 218.0378284561443820 ) ) ;
#70128=DIRECTION ( 'NONE',  ( 0.8775825618903763115, 0.000000000000000000, -0.4794255386041963996 ) ) ;
#70131=CARTESIAN_POINT ( 'NONE',  ( -10.37617513340000031, 1479.403831781789904, 210.6295454589389919 ) ) ;
#70140=CARTESIAN_POINT ( 'NONE',  ( -15.61594006588599903, 1418.240309429660101, 203.0222030835800240 ) ) ;
#70149=ORIENTED_EDGE ( 'NONE', *, *, #15321, .T. ) ;
#70154=CARTESIAN_POINT ( 'NONE',  ( 8.060344786502357195, 1436.149655876709176, 226.2159421968783022 ) ) ;
#70168=DIRECTION ( 'NONE',  ( -0.9533478951374150245, 0.2986798387784170283, 0.04379662937212339818 ) ) ;
#70173=CARTESIAN_POINT ( 'NONE',  ( 5.034012500299999360, 1484.257038904289857, 219.3935155832990063 ) ) ;
#70174=CARTESIAN_POINT ( 'NONE',  ( 10.65098579914269905, 1480.263159560079885, 208.4913410984459858 ) ) ;
#70176=CARTESIAN_POINT ( 'NONE',  ( 10.68098866639740052, 1451.528505696489901, 190.2751307916069834 ) ) ;
#70180=B_SPLINE_CURVE_WITH_KNOTS ( 'NONE', 5,
 ( #90214, #21889, #28681, #21344, #20261, #55550, #54461, #89133, #12959, #80739, #47141, #88599, #46054, #38716, #4047, #81267, #13499, #3503, #4582, #72891, #107032 ),
 .UNSPECIFIED., .F., .F.,
 ( 6, 3, 3, 3, 3, 3, 6 ),
 ( -36.02199544990000390, -35.70255572539999633, -35.38311600090000297, -30.91096027220000053, -15.58155506210000141, -15.15568292920000104, -14.73068219289999803 ),
 .UNSPECIFIED. ) ;
#70181=DIRECTION ( 'NONE',  ( 0.1751037286923191050, 0.3726097680845921745, -0.9113180810924323971 ) ) ;
#70184=CARTESIAN_POINT ( 'NONE',  ( 9.788553136239070085, 1435.243871060430138, 208.4607419252359932 ) ) ;
#70185=CARTESIAN_POINT ( 'NONE',  ( -11.32899621019999969, 1490.498838803789795, 210.5081409889190240 ) ) ;
#70195=CARTESIAN_POINT ( 'NONE',  ( 10.99927853205480055, 1502.537208110279835, 214.7972864508199962 ) ) ;
#70196=CARTESIAN_POINT ( 'NONE',  ( -9.617736285228385640, 1422.771253444837839, 210.6923910180071857 ) ) ;
#70215=CARTESIAN_POINT ( 'NONE',  ( -3.497059220858349526, 1428.107238701659981, 208.0505560005599932 ) ) ;
#70217=ORIENTED_EDGE ( 'NONE', *, *, #37814, .F. ) ;
#70227=CARTESIAN_POINT ( 'NONE',  ( -1.353007460168119902, 1465.121494863239832, 198.2016196216069943 ) ) ;
#70232=ORIENTED_EDGE ( 'NONE', *, *, #76427, .T. ) ;
#70234=ORIENTED_EDGE ( 'NONE', *, *, #24097, .F. ) ;
#70237=EDGE_LOOP ( 'NONE', ( #90118, #73304, #108836, #10395 ) ) ;
#70242=CARTESIAN_POINT ( 'NONE',  ( -3.563323249086690403, 1433.447251056540154, 218.0070131686250079 ) ) ;
#70244=CARTESIAN_POINT ( 'NONE',  ( 6.646318662569973057, 1377.913060387289988, 209.1218459647943746 ) ) ;
#70246=CARTESIAN_POINT ( 'NONE',  ( -2.188078410700000198, 1508.020976590390092, 220.9453026643990086 ) ) ;
#70249=CARTESIAN_POINT ( 'NONE',  ( -2.923984041130000211, 1463.321251604189911, 228.6078422769990084 ) ) ;
#70253=CARTESIAN_POINT ( 'NONE',  ( -11.70289210622340192, 1482.471125327160053, 206.9498061491099747 ) ) ;
#70256=ORIENTED_EDGE ( 'NONE', *, *, #3599, .F. ) ;
#70260=DIRECTION ( 'NONE',  ( 0.02616798426500960631, 0.9993150019883683122, 0.02616798426500945712 ) ) ;
#70262=CARTESIAN_POINT ( 'NONE',  ( 7.443246446248299009, 1423.092341332710021, 195.6161848952980051 ) ) ;
#70263=B_SPLINE_CURVE_WITH_KNOTS ( 'NONE', 5,
 ( #25725, #59925, #109754, #84545, #60474, #59375 ),
 .UNSPECIFIED., .F., .F.,
 ( 6, 6 ),
 ( -2.000000000000000000, -2.311399205368047660E-08 ),
 .UNSPECIFIED. ) ;
#70266=CARTESIAN_POINT ( 'NONE',  ( -9.191350345563439106, 1450.447642638940124, 208.3545562163980094 ) ) ;
#70270=CARTESIAN_POINT ( 'NONE',  ( -10.49942725105620056, 1508.438008077390123, 218.5529879601039909 ) ) ;
#70274=CARTESIAN_POINT ( 'NONE',  ( 20.89240899049999811, 1496.462831935489930, 205.9570778813589982 ) ) ;
#70281=CARTESIAN_POINT ( 'NONE',  ( 1.372954253770000133, 1432.414673090790075, 200.7998073325189807 ) ) ;
#70284=CARTESIAN_POINT ( 'NONE',  ( -0.3534431153210010335, 1507.725504649390132, 220.9869073979990048 ) ) ;
#70289=CARTESIAN_POINT ( 'NONE',  ( 4.449801743544099963, 1466.569988769939982, 199.3372086498600027 ) ) ;
#70291=FACE_OUTER_BOUND ( 'NONE', #79696, .T. ) ;
#70293=CARTESIAN_POINT ( 'NONE',  ( 9.461346545499999650, 1428.170031190390091, 212.4970399571089956 ) ) ;
#70303=CARTESIAN_POINT ( 'NONE',  ( -11.36959371680000075, 1503.847165134090119, 207.0750569533189775 ) ) ;
#70305=CARTESIAN_POINT ( 'NONE',  ( -1.642047857909999964, 1448.524332027589935, 190.1362812327990071 ) ) ;
#70307=CARTESIAN_POINT ( 'NONE',  ( -1.955601760757490037, 1457.577163455510117, 219.5947542298710005 ) ) ;
#70308=CARTESIAN_POINT ( 'NONE',  ( -2.170628023513319516, 1485.611815822959898, 197.4219878149299916 ) ) ;
#70309=CARTESIAN_POINT ( 'NONE',  ( -9.114100666540000617, 1450.438723326089985, 204.6615263125590047 ) ) ;
#70311=CARTESIAN_POINT ( 'NONE',  ( 7.389162030640000545, 1425.109552474849806, 212.4764166173689830 ) ) ;
#70312=CARTESIAN_POINT ( 'NONE',  ( 11.69992624430000028, 1435.514532378290141, 225.6365414701989778 ) ) ;
#70327=CARTESIAN_POINT ( 'NONE',  ( -3.665756888920000289, 1508.551704408389924, 214.1089243971590008 ) ) ;
#70340=CARTESIAN_POINT ( 'NONE',  ( -4.023353920839999986, 1454.320588500490203, 200.2248028819489889 ) ) ;
#70344=B_SPLINE_SURFACE_WITH_KNOTS ( 'NONE', 5, 5, ( 
 ( #20641, #1681, #71108, #27966, #79486, #88967 ),
 ( #43670, #2793, #35260, #77822, #96841, #44790 ),
 ( #78942, #95722, #28521, #1130, #70553, #52630 ),
 ( #26864, #70005, #69445, #62720, #35822, #104119 ),
 ( #104672, #27406, #62150, #96277, #65452, #13897 ),
 ( #5521, #55390, #23413, #99560, #46448, #57050 ),
 ( #38558, #98467, #89520, #97909, #21180, #4432 ),
 ( #12258, #12812, #107418, #22285, #72204, #46992 ),
 ( #64900, #81115, #106327, #73281, #66008, #72737 ) ),
 .UNSPECIFIED., .F., .F., .F.,
 ( 6, 3, 6 ),
 ( 6, 6 ),
 ( 20.66572445029999727, 22.33923004749999919, 24.01273564469999755 ),
 ( 0.000000000000000000, 2.000000000000000000 ),
 .UNSPECIFIED. ) ;
#70366=CARTESIAN_POINT ( 'NONE',  ( 24.04366655069240366, 1494.655546942339924, 207.1744041867209773 ) ) ;
#70379=CARTESIAN_POINT ( 'NONE',  ( 3.511588562210000042, 1485.920069248189975, 198.9399334953989751 ) ) ;
#70391=CARTESIAN_POINT ( 'NONE',  ( 4.865303301610000908, 1425.588844564269948, 210.1313439721089935 ) ) ;
#70394=CARTESIAN_POINT ( 'NONE',  ( 2.735388290130000399, 1441.676293522389869, 218.2628663559290203 ) ) ;
#70396=CARTESIAN_POINT ( 'NONE',  ( -3.129590240750207641, 1508.089762839850664, 220.8354442735884788 ) ) ;
#70402=CARTESIAN_POINT ( 'NONE',  ( 4.253777714910000007, 1442.471859903390168, 216.9083338397390150 ) ) ;
#70409=CARTESIAN_POINT ( 'NONE',  ( -2.461679514290000537, 1485.354438815590129, 197.8976887413989800 ) ) ;
#70410=CARTESIAN_POINT ( 'NONE',  ( -4.646147325060000277, 1378.399971913189802, 203.6922293430689876 ) ) ;
#70411=CARTESIAN_POINT ( 'NONE',  ( -10.47307406344970104, 1479.706635250730187, 209.8500660232109851 ) ) ;
#70413=CARTESIAN_POINT ( 'NONE',  ( -11.37556622210709811, 1470.595267410999895, 209.8768689712920263 ) ) ;
#70414=CARTESIAN_POINT ( 'NONE',  ( -8.150407651345240367, 1489.695318043820180, 216.4961765964640108 ) ) ;
#70415=CARTESIAN_POINT ( 'NONE',  ( -19.58883746862870012, 1465.811302608600045, 204.1485295717249926 ) ) ;
#70422=CARTESIAN_POINT ( 'NONE',  ( 10.57119421182350116, 1452.454795556669978, 209.2037162487509931 ) ) ;
#70423=ORIENTED_EDGE ( 'NONE', *, *, #106847, .T. ) ;
#70427=ADVANCED_FACE ( 'NONE', ( #94063 ), #44642, .T. ) ;
#70432=CARTESIAN_POINT ( 'NONE',  ( 6.824596843277944913, 1424.786834349993342, 213.4892281956427098 ) ) ;
#70435=CARTESIAN_POINT ( 'NONE',  ( -4.214198108440539770, 1495.305865917009896, 197.5356767487029970 ) ) ;
#70441=CARTESIAN_POINT ( 'NONE',  ( -1.768532852147479906, 1515.064792882589927, 213.4512947377390049 ) ) ;
#70447=CARTESIAN_POINT ( 'NONE',  ( -2.487924076119420125, 1508.884228858900087, 213.6131300271670170 ) ) ;
#70448=CARTESIAN_POINT ( 'NONE',  ( -17.60826646697100273, 1487.424402488250053, 195.0120373652249839 ) ) ;
#70457=CARTESIAN_POINT ( 'NONE',  ( -9.659668702359999415, 1460.930246203189881, 210.9154259863990148 ) ) ;
#70462=CARTESIAN_POINT ( 'NONE',  ( -8.769605281700000532, 1423.161328079120040, 210.3743386932289923 ) ) ;
#70463=ORIENTED_EDGE ( 'NONE', *, *, #19919, .F. ) ;
#70467=CARTESIAN_POINT ( 'NONE',  ( 7.112947187247390168, 1426.630951286630079, 213.1637636118960017 ) ) ;
#70469=CARTESIAN_POINT ( 'NONE',  ( 1.553494589745609833, 1495.825222316409963, 221.3635534445299982 ) ) ;
#70476=CARTESIAN_POINT ( 'NONE',  ( -16.93034130587640007, 1508.454808519469907, 213.3837835212590051 ) ) ;
#70478=CARTESIAN_POINT ( 'NONE',  ( -8.588755023577968828, 1437.818823225090000, 207.9413749079909906 ) ) ;
#70484=CARTESIAN_POINT ( 'NONE',  ( 8.435534112686301711, 1435.555565619180015, 206.9221676573980062 ) ) ;
#70504=VERTEX_POINT ( 'NONE', #18996 ) ;
#70505=CARTESIAN_POINT ( 'NONE',  ( 2.487924076119540029, 1508.884228858900087, 204.6305618962310007 ) ) ;
#70506=EDGE_CURVE ( 'NONE', #2790, #41237, #17831, .T. ) ;
#70513=CARTESIAN_POINT ( 'NONE',  ( -3.403509591720000227, 1496.471358393389892, 198.2852398950990107 ) ) ;
#70517=DIRECTION ( 'NONE',  ( 0.4794255386042031719, 0.000000000000000000, 0.8775825618903726477 ) ) ;
#70524=CARTESIAN_POINT ( 'NONE',  ( -8.061508288203871331, 1484.198171600520254, 200.3613286617199947 ) ) ;
#70531=DIRECTION ( 'NONE',  ( -9.439841191556039654E-47, 1.000000000000000000, -1.836970198721029688E-16 ) ) ;
#70533=CARTESIAN_POINT ( 'NONE',  ( 3.122055633242120098, 1424.574844735749821, 188.9232701594920059 ) ) ;
#70537=CARTESIAN_POINT ( 'NONE',  ( 10.78168260516119936, 1461.896513113439823, 211.1674540152700104 ) ) ;
#70542=CARTESIAN_POINT ( 'NONE',  ( -16.08688390367190379, 1420.213695813531103, 209.4851459447380080 ) ) ;
#70549=CARTESIAN_POINT ( 'NONE',  ( 3.074703527060000052, 1441.333178254290033, 218.5515148082390056 ) ) ;
#70553=CARTESIAN_POINT ( 'NONE',  ( -4.557053783849999817, 1474.667304043090098, 199.0764274286989917 ) ) ;
#70557=CARTESIAN_POINT ( 'NONE',  ( -6.059217065147319836, 1508.551704408389924, 219.4267866760630170 ) ) ;
#70559=B_SPLINE_SURFACE_WITH_KNOTS ( 'NONE', 5, 5, ( 
 ( #611, #84040, #76748, #51005, #7338, #67815 ),
 ( #16261, #50464, #60, #49353, #59971, #68375 ),
 ( #83481, #42048, #66722, #94086, #84588, #51553 ),
 ( #17356, #67271, #85688, #41502, #8985, #75116 ),
 ( #24114, #34741, #76200, #6775, #25216, #75661 ),
 ( #59420, #109803, #109263, #43157, #100297, #58305 ),
 ( #92427, #33082, #35295, #38467, #72644, #26902 ),
 ( #1165, #61624, #103602, #81027, #52114, #44266 ),
 ( #95756, #69480, #64251, #61091, #95206, #94645 ) ),
 .UNSPECIFIED., .F., .F., .F.,
 ( 6, 3, 6 ),
 ( 6, 6 ),
 ( 3.966463181890000023, 7.853302612130000249, 13.00030988960000045 ),
 ( 0.000000000000000000, 2.000000000000000000 ),
 .UNSPECIFIED. ) ;
#70563=CARTESIAN_POINT ( 'NONE',  ( -2.265697975220000160, 1431.525679395089810, 217.2185296630090079 ) ) ;
#70564=CARTESIAN_POINT ( 'NONE',  ( -10.24672469099380123, 1472.256837706050192, 207.1292450579819899 ) ) ;
#70569=CARTESIAN_POINT ( 'NONE',  ( 9.612801490498689816, 1424.761641057829820, 208.8539646045889810 ) ) ;
#70575=CARTESIAN_POINT ( 'NONE',  ( 7.443246446248299009, 1423.092341332710021, 195.6161848952980051 ) ) ;
#70578=CARTESIAN_POINT ( 'NONE',  ( -0.9569096709085479491, 1496.314324137450058, 196.8078323967840220 ) ) ;
#70581=CARTESIAN_POINT ( 'NONE',  ( -14.55278341820000065, 1420.461940006850000, 213.8336615198890058 ) ) ;
#70583=CARTESIAN_POINT ( 'NONE',  ( 4.353674023710000007, 1446.914190579090018, 199.8745573264090183 ) ) ;
#70593=CARTESIAN_POINT ( 'NONE',  ( -2.667618532240000118, 1496.805265767590072, 220.8079931561990179 ) ) ;
#70601=CARTESIAN_POINT ( 'NONE',  ( 16.83374205149999980, 1433.582731286290027, 217.5197046195389987 ) ) ;
#70606=CARTESIAN_POINT ( 'NONE',  ( -5.032977198260000229, 1391.805267112089950, 214.4361776263990009 ) ) ;
#70609=CARTESIAN_POINT ( 'NONE',  ( 7.793403662019999345, 1494.414358568890066, 218.7662867540790046 ) ) ;
#70615=CARTESIAN_POINT ( 'NONE',  ( 8.972797426533400511, 1452.010477424879809, 211.5435742291749932 ) ) ;
#70619=CARTESIAN_POINT ( 'NONE',  ( -6.488391801617740207, 1419.348173448909165, 195.1544855266193395 ) ) ;
#70625=EDGE_CURVE ( 'NONE', #106056, #98544, #95425, .T. ) ;
#70626=CARTESIAN_POINT ( 'NONE',  ( 9.370963865242019963, 1451.172249539200038, 208.3746166689639949 ) ) ;
#70627=EDGE_CURVE ( 'NONE', #70893, #66058, #52589, .T. ) ;
#70633=VERTEX_POINT ( 'NONE', #13908 ) ;
#70640=CARTESIAN_POINT ( 'NONE',  ( -7.679361995703810173, 1508.551704408399928, 219.1247835820369971 ) ) ;
#70641=CARTESIAN_POINT ( 'NONE',  ( -17.06003757377249741, 1420.270326980760046, 204.0766453804359912 ) ) ;
#70643=CARTESIAN_POINT ( 'NONE',  ( -2.130647964720339793, 1467.954295551920040, 220.0452685800179893 ) ) ;
#70648=CARTESIAN_POINT ( 'NONE',  ( 7.882820024130000824, 1493.775712921889863, 217.5949005480990195 ) ) ;
#70652=CARTESIAN_POINT ( 'NONE',  ( -18.26060618049999817, 1504.473730909189953, 209.2482098315410042 ) ) ;
#70653=DIRECTION ( 'NONE',  ( 1.000000000000000000, 2.249639673992789970E-32, 1.224646799147350002E-16 ) ) ;
#70656=CARTESIAN_POINT ( 'NONE',  ( -9.920924821321568388, 1439.719005343529943, 207.8524026893080077 ) ) ;
#70658=EDGE_LOOP ( 'NONE', ( #34378, #85515, #47603, #74568, #42337 ) ) ;
#70662=B_SPLINE_CURVE_WITH_KNOTS ( 'NONE', 5,
 ( #108796, #32087, #89241, #12537, #46716, #80846, #98184, #4150, #38277, #106590, #59510, #91989, #33726, #67918, #24218 ),
 .UNSPECIFIED., .F., .F.,
 ( 6, 3, 3, 3, 6 ),
 ( 0.000000000000000000, 0.1200153949226330508, 0.2400307898452661015, 0.4800615796854195150, 1.000000000000000000 ),
 .UNSPECIFIED. ) ;
#70665=CARTESIAN_POINT ( 'NONE',  ( 3.725765543819999692, 1506.045642329989960, 220.5640007132990092 ) ) ;
#70666=CARTESIAN_POINT ( 'NONE',  ( -15.10310828839999964, 1416.172775391969935, 212.2626019875489760 ) ) ;
#70668=CARTESIAN_POINT ( 'NONE',  ( 1.621556534070299982, 1515.068963820189992, 204.7925064057230031 ) ) ;
#70670=CARTESIAN_POINT ( 'NONE',  ( -17.16683859837399950, 1418.026022597180145, 204.8288321923220110 ) ) ;
#70671=DIRECTION ( 'NONE',  ( 0.000000000000000000, 1.000000000000000000, -1.836970198721029688E-16 ) ) ;
#70672=CARTESIAN_POINT ( 'NONE',  ( -15.85592065860000055, 1415.880107938199899, 209.4912318213870037 ) ) ;
#70679=ADVANCED_FACE ( 'NONE', ( #93382 ), #34745, .T. ) ;
#70681=CARTESIAN_POINT ( 'NONE',  ( -4.772433264290000032, 1461.586210710390105, 228.1254610687989839 ) ) ;
#70704=CARTESIAN_POINT ( 'NONE',  ( -13.27281985135759967, 1508.551708237569983, 210.0518082456389948 ) ) ;
#70720=CARTESIAN_POINT ( 'NONE',  ( -3.657993755839999750, 1474.872004365689918, 218.7367895275489786 ) ) ;
#70724=CARTESIAN_POINT ( 'NONE',  ( 1.918627788879999851, 1422.032892955219950, 193.7879044333990066 ) ) ;
#70728=CARTESIAN_POINT ( 'NONE',  ( 8.204285602689999735, 1462.106119291689993, 228.8664411563990200 ) ) ;
#70734=CARTESIAN_POINT ( 'NONE',  ( -12.21915924449999835, 1490.155271298389835, 209.9311082064550078 ) ) ;
#70737=EDGE_CURVE ( 'NONE', #345, #25915, #16110, .T. ) ;
#70739=B_SPLINE_CURVE_WITH_KNOTS ( 'NONE', 5,
 ( #56627, #21874, #65586, #30854, #82374, #21331 ),
 .UNSPECIFIED., .F., .F.,
 ( 6, 6 ),
 ( 0.000000000000000000, 1.000000000000000000 ),
 .UNSPECIFIED. ) ;
#70744=ORIENTED_EDGE ( 'NONE', *, *, #16871, .T. ) ;
#70745=ORIENTED_EDGE ( 'NONE', *, *, #99362, .F. ) ;
#70748=ORIENTED_EDGE ( 'NONE', *, *, #29551, .T. ) ;
#70750=CARTESIAN_POINT ( 'NONE',  ( 11.16012950169999840, 1500.726265256889974, 206.0864327037589874 ) ) ;
#70762=CARTESIAN_POINT ( 'NONE',  ( -4.993214567250789493, 1391.653935164599716, 214.7089805434449943 ) ) ;
#70764=ORIENTED_EDGE ( 'NONE', *, *, #10421, .F. ) ;
#70775=CARTESIAN_POINT ( 'NONE',  ( 10.14286467640000033, 1461.576202403990010, 208.9373515736710090 ) ) ;
#70791=FACE_OUTER_BOUND ( 'NONE', #78214, .T. ) ;
#70792=CARTESIAN_POINT ( 'NONE',  ( -1.673997294314879980, 1422.546829072329956, 192.5753128275750043 ) ) ;
#70794=CARTESIAN_POINT ( 'NONE',  ( 10.79528402730720060, 1489.628194868570063, 207.4012257063180016 ) ) ;
#70796=CARTESIAN_POINT ( 'NONE',  ( -2.360319324340000247, 1507.471933479789868, 221.3436898553990204 ) ) ;
#70797=ADVANCED_FACE ( 'NONE', ( #81395 ), #58903, .T. ) ;
#70799=CARTESIAN_POINT ( 'NONE',  ( 0.4156989469490010025, 1498.844189599989932, 200.5557808060589764 ) ) ;
#70801=EDGE_CURVE ( 'NONE', #3002, #79909, #83977, .T. ) ;
#70803=ADVANCED_FACE ( 'NONE', ( #4707 ), #84775, .T. ) ;
#70814=CARTESIAN_POINT ( 'NONE',  ( -11.71397076299980000, 1489.483175994190105, 212.5377881273170146 ) ) ;
#70815=CARTESIAN_POINT ( 'NONE',  ( -15.29584542989999996, 1415.909343553620147, 206.6854934211490047 ) ) ;
#70823=ORIENTED_EDGE ( 'NONE', *, *, #87834, .T. ) ;
#70827=CARTESIAN_POINT ( 'NONE',  ( 1.842963895390000273, 1515.551704166990021, 213.1059277586890062 ) ) ;
#70831=CARTESIAN_POINT ( 'NONE',  ( 3.159263275979999896, 1466.676511794390080, 219.3004963912989922 ) ) ;
#70835=CARTESIAN_POINT ( 'NONE',  ( 1.180525396009999950, 1431.432006926090253, 200.4326319868589792 ) ) ;
#70836=CARTESIAN_POINT ( 'NONE',  ( -15.92610956699463642, 1415.966321813838249, 209.5991204954336524 ) ) ;
#70838=CARTESIAN_POINT ( 'NONE',  ( -18.75625549219999755, 1442.404531551690070, 208.2016858895329960 ) ) ;
#70839=AXIS2_PLACEMENT_3D ( 'NONE', #74491, #57694, #109723 ) ;
#70843=CARTESIAN_POINT ( 'NONE',  ( 3.415182420970000354, 1486.712733516890239, 198.4695609272989998 ) ) ;
#70858=CARTESIAN_POINT ( 'NONE',  ( -11.34054827985558944, 1501.996627661553475, 207.3924314934697293 ) ) ;
#70862=CARTESIAN_POINT ( 'NONE',  ( -9.881667340448540671, 1438.678908226070007, 210.2323064812840130 ) ) ;
#70864=CARTESIAN_POINT ( 'NONE',  ( -9.173748801299998590, 1450.559996510189876, 208.1432996479669839 ) ) ;
#70866=CARTESIAN_POINT ( 'NONE',  ( 7.601709514279999524, 1425.061887899960084, 212.0249446704789875 ) ) ;
#70867=CARTESIAN_POINT ( 'NONE',  ( 5.140094423509999011, 1436.845494339190054, 228.7442485628990028 ) ) ;
#70872=CARTESIAN_POINT ( 'NONE',  ( 8.401749989260000717, 1454.595346029489974, 215.7321778818789824 ) ) ;
#70883=CARTESIAN_POINT ( 'NONE',  ( -2.528233502088980345, 1463.070495996789987, 199.6737502978820089 ) ) ;
#70890=ORIENTED_EDGE ( 'NONE', *, *, #42452, .T. ) ;
#70893=VERTEX_POINT ( 'NONE', #63554 ) ;
#70895=CARTESIAN_POINT ( 'NONE',  ( -3.589036755729999584, 1455.442922379190122, 200.3873980026590118 ) ) ;
#70900=CARTESIAN_POINT ( 'NONE',  ( 5.440512190109999757, 1424.738065781850082, 191.9794586101990319 ) ) ;
#70923=ADVANCED_FACE ( 'NONE', ( #47272 ), #93717, .F. ) ;
#70926=CARTESIAN_POINT ( 'NONE',  ( -17.84104788077500103, 1489.004184077329910, 195.1797443787960162 ) ) ;
#70928=EDGE_LOOP ( 'NONE', ( #5447, #71542, #75007, #50090 ) ) ;
#70929=DIRECTION ( 'NONE',  ( -1.000000000000000000, 0.000000000000000000, 0.000000000000000000 ) ) ;
#70942=CARTESIAN_POINT ( 'NONE',  ( 9.957762540578798394, 1469.139097590099936, 207.8491545737729780 ) ) ;
#70948=ORIENTED_EDGE ( 'NONE', *, *, #83, .F. ) ;
#70949=FACE_OUTER_BOUND ( 'NONE', #60823, .T. ) ;
#70950=CARTESIAN_POINT ( 'NONE',  ( 18.06315781999999714, 1430.297107959589766, 211.8007709855490077 ) ) ;
#70951=EDGE_CURVE ( 'NONE', #10343, #88662, #42177, .T. ) ;
#70953=CARTESIAN_POINT ( 'NONE',  ( 4.497572334437839103, 1424.519692532310046, 191.7182092258769899 ) ) ;
#70955=CARTESIAN_POINT ( 'NONE',  ( -207.7471169361000136, -8387.357407334289746, 2179.761025090469957 ) ) ;
#70956=DIRECTION ( 'NONE',  ( 0.2768460956572699194, -0.4521313779474797068, -0.8478994376661886934 ) ) ;
#70959=CARTESIAN_POINT ( 'NONE',  ( -2.031883580139580037, 1464.998375551469962, 198.3053770173009980 ) ) ;
#70963=CARTESIAN_POINT ( 'NONE',  ( -10.05392054895050080, 1472.343305534860065, 210.7099757364429706 ) ) ;
#70964=ORIENTED_EDGE ( 'NONE', *, *, #68020, .T. ) ;
#70971=LINE ( 'NONE', #37335, #3081 ) ;
#70973=CARTESIAN_POINT ( 'NONE',  ( -10.97127478134579981, 1470.155385822019980, 212.1066267448319991 ) ) ;
#70974=CARTESIAN_POINT ( 'NONE',  ( -8.552474816142620284, 1488.818340932279852, 216.6102650812369745 ) ) ;
#70976=CARTESIAN_POINT ( 'NONE',  ( -13.90060862545290021, 1502.276468621130107, 227.4029620636050026 ) ) ;
#70987=ORIENTED_EDGE ( 'NONE', *, *, #82208, .T. ) ;
#70993=CARTESIAN_POINT ( 'NONE',  ( 8.559827946524409370, 1437.030862833870060, 207.9841999479689889 ) ) ;
#70995=CARTESIAN_POINT ( 'NONE',  ( -0.2421828111940010075, 1488.147221623489941, 217.2451007367390048 ) ) ;
#70999=CARTESIAN_POINT ( 'NONE',  ( -1.621556533595490013, 1515.068963820210001, 213.4511855176750146 ) ) ;
#71001=CARTESIAN_POINT ( 'NONE',  ( -15.44414269670690132, 1421.125735695469757, 203.4397924531029958 ) ) ;
#71005=CARTESIAN_POINT ( 'NONE',  ( -3.273042392791920108, 1508.551704408389924, 214.1089285546999861 ) ) ;
#71006=CARTESIAN_POINT ( 'NONE',  ( -21.35037659171259961, 1486.708548635719808, 201.9023949429700053 ) ) ;
#71008=DIRECTION ( 'NONE',  ( 0.4794255386042031719, 0.000000000000000000, 0.8775825618903726477 ) ) ;
#71011=CARTESIAN_POINT ( 'NONE',  ( 4.328907235665639952, 1515.085473475149911, 210.4350698618210060 ) ) ;
#71014=CARTESIAN_POINT ( 'NONE',  ( -10.04630323299999972, 1461.008343231690105, 213.6807241916089879 ) ) ;
#71018=ORIENTED_EDGE ( 'NONE', *, *, #50747, .F. ) ;
#71019=CARTESIAN_POINT ( 'NONE',  ( -8.080215484499998269, 1424.584971138479887, 209.6516123241690082 ) ) ;
#71026=CARTESIAN_POINT ( 'NONE',  ( -1.737201087752100026, 1496.680566212609847, 221.3643383344579831 ) ) ;
#71029=( BOUNDED_CURVE ( )  B_SPLINE_CURVE ( 3, ( #105688, #28970, #82672, #12708 ),
 .UNSPECIFIED., .F., .T. ) 
 B_SPLINE_CURVE_WITH_KNOTS ( ( 4, 4 ),
 ( 1.009769430403854029, 2.131822871348764803 ),
 .UNSPECIFIED. ) 
 CURVE ( )  GEOMETRIC_REPRESENTATION_ITEM ( )  RATIONAL_B_SPLINE_CURVE ( ( 1.000000000000000000, 0.8978061898640717908, 0.8978061898640717908, 1.000000000000000000 ) ) 
 REPRESENTATION_ITEM ( '' )  );
#71031=CARTESIAN_POINT ( 'NONE',  ( 2.276078898794865690, 1487.012333271777834, 219.6970559366252189 ) ) ;
#71032=CARTESIAN_POINT ( 'NONE',  ( 8.910663374729999475, 1471.585705475490158, 214.3446098367489867 ) ) ;
#71033=CARTESIAN_POINT ( 'NONE',  ( -9.954813569522620753, 1439.582591239990052, 208.1867998061339904 ) ) ;
#71040=ORIENTED_EDGE ( 'NONE', *, *, #61177, .F. ) ;
#71043=CARTESIAN_POINT ( 'NONE',  ( 0.7923714640039719592, 1467.258159185920022, 220.1721432627789738 ) ) ;
#71052=CARTESIAN_POINT ( 'NONE',  ( -10.33299300126450149, 1447.717326489380184, 209.8084994042759774 ) ) ;
#71058=CARTESIAN_POINT ( 'NONE',  ( 4.678976733710090485, 1508.551704408389924, 205.0635106934799978 ) ) ;
#71061=CARTESIAN_POINT ( 'NONE',  ( -4.987078438843339789, 1508.551704408389924, 211.6718637777229901 ) ) ;
#71069=CIRCLE ( 'NONE', #103139, 14.91144628110000170 ) ;
#71074=CARTESIAN_POINT ( 'NONE',  ( -16.70831018089999986, 1417.149231790749809, 207.3570869115089863 ) ) ;
#71075=CARTESIAN_POINT ( 'NONE',  ( 4.637787270109999582, 1462.124489585889933, 228.1829287868989979 ) ) ;
#71076=CARTESIAN_POINT ( 'NONE',  ( -7.416192941597599564, 1484.381854404939986, 199.8094865323589886 ) ) ;
#71077=CARTESIAN_POINT ( 'NONE',  ( -20.09781860883127536, 1508.119603360660221, 209.6220754275047113 ) ) ;
#71080=CARTESIAN_POINT ( 'NONE',  ( -4.329448776040000446, 1515.064792882589927, 207.2788837304390199 ) ) ;
#71088=VERTEX_POINT ( 'NONE', #19724 ) ;
#71100=CARTESIAN_POINT ( 'NONE',  ( -3.137380515432329986, 1508.729448924109874, 204.5649393178340176 ) ) ;
#71102=CARTESIAN_POINT ( 'NONE',  ( -1732.234191736389675, 11221.53578756870047, -1992.291823225089274 ) ) ;
#71103=CARTESIAN_POINT ( 'NONE',  ( -2.330134126090000368, 1515.551704408389924, 205.2922258481490303 ) ) ;
#71104=CARTESIAN_POINT ( 'NONE',  ( 3.440131352139999876, 1441.985517479789905, 217.4173380492889862 ) ) ;
#71108=CARTESIAN_POINT ( 'NONE',  ( -4.794939693159999905, 1475.260167711990107, 199.8527928283789947 ) ) ;
#71111=CARTESIAN_POINT ( 'NONE',  ( -3.612392877355159904, 1508.551704408389924, 219.9195952245149783 ) ) ;
#71115=CARTESIAN_POINT ( 'NONE',  ( 3.269916730896537338, 1485.110870265661788, 219.7892682990461424 ) ) ;
#71118=CARTESIAN_POINT ( 'NONE',  ( -14.82545538847084110, 1420.108256178820739, 213.3440734001790418 ) ) ;
#71125=CARTESIAN_POINT ( 'NONE',  ( -3.378249781281797759, 1476.214897016527402, 219.3461772814387984 ) ) ;
#71126=CARTESIAN_POINT ( 'NONE',  ( 10.81577661162920023, 1490.127638817409888, 207.3825687807529903 ) ) ;
#71133=CARTESIAN_POINT ( 'NONE',  ( 12.45662817246929954, 1427.088122696140090, 206.6493147128259977 ) ) ;
#71145=CARTESIAN_POINT ( 'NONE',  ( -7.732430556567909896, 1493.472238524849899, 207.1384183514769859 ) ) ;
#71155=CARTESIAN_POINT ( 'NONE',  ( 2.265886247949999710, 1487.020940553290075, 219.7147332017989925 ) ) ;
#71165=CARTESIAN_POINT ( 'NONE',  ( 10.44089720877999916, 1453.109204862920024, 211.0141701243190084 ) ) ;
#71166=CARTESIAN_POINT ( 'NONE',  ( 5.522475241700000481, 1424.154859417280022, 193.8631810266990101 ) ) ;
#71169=CARTESIAN_POINT ( 'NONE',  ( -9.642223397419670050, 1460.679120766980077, 208.4218084076549928 ) ) ;
#71177=CARTESIAN_POINT ( 'NONE',  ( -2.419927497189999777, 1502.444211376990097, 230.3922731312990209 ) ) ;
#71189=CARTESIAN_POINT ( 'NONE',  ( -9.842736051686820531, 1471.074784007589869, 212.0439963695450274 ) ) ;
#71193=CARTESIAN_POINT ( 'NONE',  ( -12.77139216734400051, 1502.534344327860026, 209.6059914789669847 ) ) ;
#71194=CARTESIAN_POINT ( 'NONE',  ( -2.402424516307810176, 1422.211108107479959, 192.9590038495489921 ) ) ;
#71195=CARTESIAN_POINT ( 'NONE',  ( 11.26937486967429969, 1478.652699849539886, 205.8601904136019982 ) ) ;
#71196=CARTESIAN_POINT ( 'NONE',  ( 8.343648446271952679, 1424.442999199686028, 195.7429581655293873 ) ) ;
#71197=CARTESIAN_POINT ( 'NONE',  ( -14.27911803519999978, 1503.311367094989919, 208.8533501441869760 ) ) ;
#71198=CARTESIAN_POINT ( 'NONE',  ( 10.26782831285779984, 1469.378476928209921, 204.4240403020939993 ) ) ;
#71199=CARTESIAN_POINT ( 'NONE',  ( 11.93531355930769955, 1421.883139682599904, 207.3300720177520020 ) ) ;
#71201=CARTESIAN_POINT ( 'NONE',  ( -9.962284032283351465, 1439.515202336300035, 208.3475260488820027 ) ) ;
#71205=B_SPLINE_CURVE_WITH_KNOTS ( 'NONE', 5,
 ( #21113, #31738, #3825, #48567, #22761, #56410 ),
 .UNSPECIFIED., .F., .F.,
 ( 6, 6 ),
 ( 0.000000000000000000, 1.000000000000000000 ),
 .UNSPECIFIED. ) ;
#71210=CARTESIAN_POINT ( 'NONE',  ( 3.554299223149999687, 1505.806595534090093, 220.9721875483989777 ) ) ;
#71212=CARTESIAN_POINT ( 'NONE',  ( -17.81215992105380153, 1419.248216703719891, 206.8919694010189687 ) ) ;
#71214=CARTESIAN_POINT ( 'NONE',  ( -17.38240445386849942, 1417.772954075339840, 205.8675793474119757 ) ) ;
#71217=CARTESIAN_POINT ( 'NONE',  ( -19.74523735960000081, 1465.054873128789950, 210.0762488071430028 ) ) ;
#71221=DIRECTION ( 'NONE',  ( 0.000000000000000000, 1.000000000000000000, -1.836970198721029688E-16 ) ) ;
#71225=CARTESIAN_POINT ( 'NONE',  ( 9.708743359033459086, 1469.923152700759829, 211.7994329600670085 ) ) ;
#71246=CARTESIAN_POINT ( 'NONE',  ( -3.827053565004849833, 1515.145425758850251, 209.1218459619010162 ) ) ;
#71250=CARTESIAN_POINT ( 'NONE',  ( -19.27355791249999939, 1467.813399981289876, 204.3088842694490097 ) ) ;
#71257=VECTOR ( 'NONE', #105952, 1000.000000000000114 ) ;
#71261=B_SPLINE_SURFACE_WITH_KNOTS ( 'NONE', 5, 5, ( 
 ( #35985, #26456, #60650, #95334, #52246, #18595 ),
 ( #52792, #34315, #86926, #102594, #10217, #79103 ),
 ( #93645, #17483, #44395, #78537, #51129, #27574 ),
 ( #61757, #19144, #87496, #10784, #44956, #2411 ),
 ( #36528, #70724, #47143, #88601, #37630, #105392 ),
 ( #37076, #54463, #11884, #62316, #62890, #46608 ),
 ( #11340, #28684, #53921, #4049, #20263, #45513 ),
 ( #5121, #97000, #81819, #38176, #63421, #79654 ),
 ( #2959, #29232, #46056, #39277, #107034, #38718 ) ),
 .UNSPECIFIED., .F., .F., .F.,
 ( 6, 3, 6 ),
 ( 6, 6 ),
 ( 4.410666364559999941, 8.626592454029999857, 14.48744219459999982 ),
 ( 0.000000000000000000, 2.000000000000000000 ),
 .UNSPECIFIED. ) ;
#71267=CARTESIAN_POINT ( 'NONE',  ( -10.83190899079038161, 1493.268439024361669, 206.6147278250968213 ) ) ;
#71270=CIRCLE ( 'NONE', #35498, 15.40132948099999943 ) ;
#71283=CARTESIAN_POINT ( 'NONE',  ( -2.515588616550900269, 1448.349620516269852, 188.5842437137009995 ) ) ;
#71289=CARTESIAN_POINT ( 'NONE',  ( 1766.069695707609526, -8382.262153571264207, 2383.103299250912187 ) ) ;
#71295=CARTESIAN_POINT ( 'NONE',  ( 11.46366843843170003, 1502.128415927390051, 212.5217899936770323 ) ) ;
#71296=CARTESIAN_POINT ( 'NONE',  ( -14.98674809609716263, 1420.597066439330092, 210.5912578852586989 ) ) ;
#71302=CARTESIAN_POINT ( 'NONE',  ( 0.02352154200225501854, 1457.675724657883848, 199.5853667110562242 ) ) ;
#71308=B_SPLINE_CURVE_WITH_KNOTS ( 'NONE', 3,
 ( #61861, #43384, #95981, #19242, #77532, #33856 ),
 .UNSPECIFIED., .F., .F.,
 ( 4, 2, 4 ),
 ( 0.000000000000000000, 0.5000000000000000000, 1.000000000000000000 ),
 .UNSPECIFIED. ) ;
#71310=CARTESIAN_POINT ( 'NONE',  ( -0.7443733913810010039, 1468.219489664089906, 219.4953987198990148 ) ) ;
#71315=CARTESIAN_POINT ( 'NONE',  ( -10.78881813950000002, 1422.299201281090063, 210.6311831754890136 ) ) ;
#71318=CARTESIAN_POINT ( 'NONE',  ( -13.97985296220000073, 1420.196174967039951, 195.9955836506989897 ) ) ;
#71319=CARTESIAN_POINT ( 'NONE',  ( -1.417680259639110041, 1431.646251614470202, 200.8417364822699938 ) ) ;
#71320=EDGE_LOOP ( 'NONE', ( #76400, #32382, #3951 ) ) ;
#71322=ADVANCED_FACE ( 'NONE', ( #78402 ), #12503, .T. ) ;
#71329=CARTESIAN_POINT ( 'NONE',  ( 2.340033977622370198, 1466.009485822560009, 198.3389262314019845 ) ) ;
#71336=ORIENTED_EDGE ( 'NONE', *, *, #30765, .F. ) ;
#71338=CARTESIAN_POINT ( 'NONE',  ( 11.76014171143800091, 1479.338753478690023, 208.6264959333659874 ) ) ;
#71344=CARTESIAN_POINT ( 'NONE',  ( 6.826689052339999897, 1469.354294130389917, 209.2233868860279813 ) ) ;
#71346=CARTESIAN_POINT ( 'NONE',  ( -3.286480964850000408, 1456.341185808290220, 218.0120306903490075 ) ) ;
#71351=CARTESIAN_POINT ( 'NONE',  ( -16.32163040922650055, 1507.551697810010182, 213.4489835936819873 ) ) ;
#71352=B_SPLINE_CURVE_WITH_KNOTS ( 'NONE', 3,
 ( #1669, #95710, #45334, #18976, #53173, #87883, #44779, #71663, #96828, #54831, #10045, #19542, #105221, #70542, #61039, #11706, #72194, #87315, #37461, #29066, #10610, #36350, #62139, #80016, #35810, #104659, #95162, #18419, #62709, #52619, #69992, #20097, #27956, #78929, #44218, #78361 ),
 .UNSPECIFIED., .F., .F.,
 ( 4, 2, 2, 1, 1, 1, 1, 2, 2, 2, 2, 1, 1, 2, 2, 2, 2, 1, 1, 2, 2, 4 ),
 ( 0.000000000000000000, 0.1249999999996103950, 0.1874999999994146627, 0.2187499999993167688, 0.2343749999992800759, 0.2421874999992680855, 0.2460937499992680855, 0.2480468749992686128, 0.2499999999992691957, 0.3749999999996406208, 0.4374999999998094857, 0.4687499999998851474, 0.4843749999999223399, 0.4921874999999306666, 0.4999999999999389377, 0.6249999999998843148, 0.6874999999998553379, 0.7187499999998425704, 0.7343749999998377964, 0.7421874999998345768, 0.7499999999998312461, 1.000000000000000000 ),
 .UNSPECIFIED. ) ;
#71363=CARTESIAN_POINT ( 'NONE',  ( 7.622520388263168911, 1452.679533476516099, 191.4523119007226910 ) ) ;
#71365=ORIENTED_EDGE ( 'NONE', *, *, #4346, .T. ) ;
#71368=CARTESIAN_POINT ( 'NONE',  ( -9.202353836351246485, 1488.302798331107169, 217.0664070768366969 ) ) ;
#71369=CARTESIAN_POINT ( 'NONE',  ( -20.11385680769999951, 1487.601373209189887, 204.1067431612489997 ) ) ;
#71375=CARTESIAN_POINT ( 'NONE',  ( -8.972902429201688790, 1449.183751661920041, 211.0003755984220106 ) ) ;
#71382=CARTESIAN_POINT ( 'NONE',  ( -0.008738962350170510068, 1515.558522550590169, 213.2765912358790104 ) ) ;
#71385=CARTESIAN_POINT ( 'NONE',  ( 20.54534055259999903, 1497.714303034489831, 214.2326470396490095 ) ) ;
#71393=CARTESIAN_POINT ( 'NONE',  ( -4.138993644310000164, 1515.551749209589843, 209.4962531541799819 ) ) ;
#71396=CARTESIAN_POINT ( 'NONE',  ( 10.70401247158669911, 1470.123045870449914, 207.0335124537880063 ) ) ;
#71400=CARTESIAN_POINT ( 'NONE',  ( -4.487249772970000272, 1509.038615934189920, 209.1218459608020055 ) ) ;
#71402=B_SPLINE_SURFACE_WITH_KNOTS ( 'NONE', 5, 1, ( 
 ( #91973, #50540 ),
 ( #41016, #6319 ),
 ( #41584, #66803 ),
 ( #92513, #7964 ),
 ( #76836, #51090 ),
 ( #49982, #33708 ) ),
 .UNSPECIFIED., .F., .F., .F.,
 ( 6, 6 ),
 ( 2, 2 ),
 ( 0.000000000000000000, 3.920049511110000218 ),
 ( 0.000000000000000000, 14.00000000000000000 ),
 .UNSPECIFIED. ) ;
#71404=B_SPLINE_CURVE_WITH_KNOTS ( 'NONE', 3,
 ( #68436, #33689, #25830, #75720, #42660, #34804, #84099, #85753, #67883, #76815, #109866, #33143, #49963, #67332, #101430, #93590, #68992, #8486, #59479, #60031, #24721, #15227, #93049, #16866, #51069, #50523, #94149, #51618, #103093, #6837, #86862, #95814, #9595, #69545, #43765, #104217, #26964, #80114, #71198, #2888, #78471, #10720, #104770, #44891, #18532, #96370, #52727, #103666, #53285 ),
 .UNSPECIFIED., .F., .F.,
 ( 4, 3, 3, 3, 3, 3, 3, 3, 3, 3, 3, 3, 3, 3, 3, 3, 4 ),
 ( -28.88939375100000007, -28.35496397148130043, -26.99855305397730021, -25.63863431757279798, -24.27724806815169956, -22.91518329866390147, -21.55400513323160183, -20.19477292252609857, -18.83849860325140213, -17.48889295550879908, -16.74086542361019880, -15.46648022024419866, -14.14486414810110126, -12.80329080502029981, -11.46594563996600158, -10.15626214476240108, -8.883338167809998964 ),
 .UNSPECIFIED. ) ;
#71405=CARTESIAN_POINT ( 'NONE',  ( -10.91430100039999829, 1483.114603242489920, 204.3199828216889955 ) ) ;
#71410=VECTOR ( 'NONE', #76148, 1000.000000000000227 ) ;
#71415=CARTESIAN_POINT ( 'NONE',  ( -1.022619748562719977, 1436.061388905930016, 227.5769040188990004 ) ) ;
#71421=CARTESIAN_POINT ( 'NONE',  ( -10.22077960920000095, 1448.827726244289806, 207.2905429624990177 ) ) ;
#71424=CARTESIAN_POINT ( 'NONE',  ( 7.553999303160000345, 1425.256314220230024, 212.1065527620190210 ) ) ;
#71427=DIRECTION ( 'NONE',  ( 0.07512831052118132402, 0.9801898970463382987, 0.1832580221614370231 ) ) ;
#71429=AXIS2_PLACEMENT_3D ( 'NONE', #109196, #59901, #58784 ) ;
#71432=CARTESIAN_POINT ( 'NONE',  ( 6.163562822530000318, 1453.283431879389809, 216.1943447892690244 ) ) ;
#71439=CARTESIAN_POINT ( 'NONE',  ( 4.304841658572250651, 1499.458000153912508, 198.5863174272942899 ) ) ;
#71454=ADVANCED_FACE ( 'NONE', ( #24530 ), #71533, .T. ) ;
#71456=CARTESIAN_POINT ( 'NONE',  ( -3.617198352219999968, 1454.554796268290147, 200.0420705370489998 ) ) ;
#71463=CARTESIAN_POINT ( 'NONE',  ( 7.904651180169999236, 1423.075284537190100, 213.5785853047590024 ) ) ;
#71471=ORIENTED_EDGE ( 'NONE', *, *, #3817, .T. ) ;
#71482=CARTESIAN_POINT ( 'NONE',  ( -21.59687499341919903, 1507.523464219199923, 209.4572686751589856 ) ) ;
#71484=ORIENTED_EDGE ( 'NONE', *, *, #3509, .T. ) ;
#71494=( BOUNDED_CURVE ( )  B_SPLINE_CURVE ( 3, ( #90624, #81661, #22293, #6075 ),
 .UNSPECIFIED., .F., .F. ) 
 B_SPLINE_CURVE_WITH_KNOTS ( ( 4, 4 ),
 ( 4.143391436656575166, 5.281615214968810257 ),
 .UNSPECIFIED. ) 
 CURVE ( )  GEOMETRIC_REPRESENTATION_ITEM ( )  RATIONAL_B_SPLINE_CURVE ( ( 1.000000000000000000, 0.8949199307684150284, 0.8949199307684150284, 1.000000000000000000 ) ) 
 REPRESENTATION_ITEM ( '' )  );
#71503=CARTESIAN_POINT ( 'NONE',  ( 10.54077562621580100, 1470.446268097909751, 208.9023493837970022 ) ) ;
#71508=TOROIDAL_SURFACE ( 'NONE', #94714, 12.73448142120000171, 1.000000000000000000 ) ;
#71510=CARTESIAN_POINT ( 'NONE',  ( 18.20258715539999983, 1429.723789929190161, 209.1218459616989946 ) ) ;
#71512=CARTESIAN_POINT ( 'NONE',  ( 2.026941135499999991, 1442.331840242090038, 218.1303087973689969 ) ) ;
#71522=CARTESIAN_POINT ( 'NONE',  ( -10.13169652023110068, 1472.475396586130046, 210.1560152870009688 ) ) ;
#71525=CARTESIAN_POINT ( 'NONE',  ( -8.256084004110000762, 1508.551704433089981, 218.9904985306490062 ) ) ;
#71528=CARTESIAN_POINT ( 'NONE',  ( -2.979329921729999775, 1485.440599754389950, 197.5893634892990178 ) ) ;
#71529=AXIS2_PLACEMENT_3D ( 'NONE', #32257, #4842, #83758 ) ;
#71533=B_SPLINE_SURFACE_WITH_KNOTS ( 'NONE', 5, 5, ( 
 ( #76067, #41913, #32941, #59286, #110210, #68794 ),
 ( #7748, #84996, #15569, #101793, #102355, #26193 ),
 ( #58718, #485, #93951, #76613, #50867, #51413 ),
 ( #85545, #33483, #93404, #25083, #77182, #60381 ),
 ( #8291, #8841, #43024, #16669, #92299, #110765 ),
 ( #25638, #50335, #67685, #102894, #42454, #34608 ),
 ( #17218, #84461, #34055, #23976, #92853, #49771 ),
 ( #68247, #59830, #58170, #83902, #16129, #7208 ),
 ( #41364, #75531, #109666, #67131, #101230, #108371 ) ),
 .UNSPECIFIED., .F., .F., .F.,
 ( 6, 3, 6 ),
 ( 6, 6 ),
 ( 3.959746331690000343, 7.829449941020000026, 12.95412177010000043 ),
 ( 0.000000000000000000, 2.000000000000000000 ),
 .UNSPECIFIED. ) ;
#71534=DIRECTION ( 'NONE',  ( 0.000000000000000000, 1.000000000000000000, 0.000000000000000000 ) ) ;
#71536=CARTESIAN_POINT ( 'NONE',  ( -7.889194276409699391, 1488.589073438359947, 217.2869014410679824 ) ) ;
#71537=CARTESIAN_POINT ( 'NONE',  ( 4.803837674189999518, 1471.771474222590086, 187.6888395837989947 ) ) ;
#71540=CARTESIAN_POINT ( 'NONE',  ( 7.671689734580000142, 1427.928541111089999, 213.1259205237190031 ) ) ;
#71541=CARTESIAN_POINT ( 'NONE',  ( -18.35946451589240169, 1443.345020097670158, 213.1741786437940220 ) ) ;
#71542=ORIENTED_EDGE ( 'NONE', *, *, #39288, .F. ) ;
#71547=ORIENTED_EDGE ( 'NONE', *, *, #88592, .F. ) ;
#71554=ADVANCED_FACE ( 'NONE', ( #103251 ), #67493, .T. ) ;
#71565=ADVANCED_FACE ( 'NONE', ( #16416 ), #67819, .T. ) ;
#71570=CARTESIAN_POINT ( 'NONE',  ( -12.97219746350000058, 1506.894675433090015, 209.2202028069119990 ) ) ;
#71571=CARTESIAN_POINT ( 'NONE',  ( 16.63319105031239786, 1492.894349348930064, 193.2649508192429835 ) ) ;
#71576=CIRCLE ( 'NONE', #23228, 15.09021984820000029 ) ;
#71577=CARTESIAN_POINT ( 'NONE',  ( 4.328404850859260300, 1515.104658776890119, 210.1767891407040167 ) ) ;
#71587=CARTESIAN_POINT ( 'NONE',  ( -9.299128358382350967, 1447.143969702200138, 212.1393002196799955 ) ) ;
#71590=CARTESIAN_POINT ( 'NONE',  ( 7.133777758825489812, 1426.611815516710067, 213.1249336043190112 ) ) ;
#71598=CARTESIAN_POINT ( 'NONE',  ( -8.584430616891150834, 1438.454652122179823, 207.6921544452859791 ) ) ;
#71603=CARTESIAN_POINT ( 'NONE',  ( 9.313029624468448731, 1435.254921036249925, 208.0259770765709959 ) ) ;
#71608=CARTESIAN_POINT ( 'NONE',  ( 3.235048515759559873, 1466.472015849239824, 219.6884157167970102 ) ) ;
#71611=CARTESIAN_POINT ( 'NONE',  ( 4.989246313819999834, 1471.909539260290103, 189.7082128665990126 ) ) ;
#71620=CARTESIAN_POINT ( 'NONE',  ( 0.2521604941109990006, 1444.846786543190092, 215.4142079403889909 ) ) ;
#71625=CARTESIAN_POINT ( 'NONE',  ( -9.173749095941850840, 1450.559996438570124, 208.1432995907519796 ) ) ;
#71628=CARTESIAN_POINT ( 'NONE',  ( -6.416973687110000490, 1415.004829294899992, 206.0388214070289905 ) ) ;
#71633=DIRECTION ( 'NONE',  ( 0.3790982213344173957, 0.2704758103281632020, 0.8849448426926984634 ) ) ;
#71638=CARTESIAN_POINT ( 'NONE',  ( -16.98677577339999800, 1417.365056119239853, 206.8931061268690144 ) ) ;
#71641=B_SPLINE_CURVE_WITH_KNOTS ( 'NONE', 5,
 ( #110156, #102836, #26130, #17158, #103387, #77124 ),
 .UNSPECIFIED., .F., .F.,
 ( 6, 6 ),
 ( -2.000000000000000000, 0.000000000000000000 ),
 .UNSPECIFIED. ) ;
#71646=VECTOR ( 'NONE', #105119, 1000.000000000000000 ) ;
#71649=DIRECTION ( 'NONE',  ( -1.000000000000000000, 0.000000000000000000, 0.000000000000000000 ) ) ;
#71651=CARTESIAN_POINT ( 'NONE',  ( -9.704836608734391135, 1461.007466806910088, 210.6916309006689971 ) ) ;
#71654=ORIENTED_EDGE ( 'NONE', *, *, #26981, .F. ) ;
#71658=CARTESIAN_POINT ( 'NONE',  ( 10.95515571501579899, 1480.001721184990174, 209.1067782184190094 ) ) ;
#71660=CARTESIAN_POINT ( 'NONE',  ( -1.637338503800000122, 1444.255706267190135, 199.2007328904890073 ) ) ;
#71663=CARTESIAN_POINT ( 'NONE',  ( -15.95079730031611831, 1420.249988525623849, 209.7644246339181677 ) ) ;
#71671=CARTESIAN_POINT ( 'NONE',  ( 9.181100887863649973, 1450.964097471789955, 210.1935140534000084 ) ) ;
#71678=ORIENTED_EDGE ( 'NONE', *, *, #31765, .F. ) ;
#71679=CARTESIAN_POINT ( 'NONE',  ( 18.46111558074320058, 1471.785967886609797, 195.2229703376199836 ) ) ;
#71682=CARTESIAN_POINT ( 'NONE',  ( -0.9541980877279990780, 1483.985701638789806, 201.2944014693789825 ) ) ;
#71683=CARTESIAN_POINT ( 'NONE',  ( 3.584503077415259753, 1486.500511906220027, 219.3043361390229791 ) ) ;
#71686=CARTESIAN_POINT ( 'NONE',  ( -2.492462743589999974, 1432.101689878689967, 217.3048426501089807 ) ) ;
#71690=CARTESIAN_POINT ( 'NONE',  ( 5.650554639980001070, 1452.063337922390019, 211.4905752170589892 ) ) ;
#71694=CARTESIAN_POINT ( 'NONE',  ( 11.43665885888289857, 1491.402434470230219, 208.3916377791149728 ) ) ;
#71701=EDGE_CURVE ( 'NONE', #105896, #21322, #65873, .T. ) ;
#71708=LINE ( 'NONE', #88463, #107295 ) ;
#71713=CARTESIAN_POINT ( 'NONE',  ( 0.3681096306540009855, 1496.876227892089901, 197.1249798701990130 ) ) ;
#71716=EDGE_LOOP ( 'NONE', ( #88870, #80562, #6051, #1473 ) ) ;
#71732=EDGE_LOOP ( 'NONE', ( #30360, #109704, #60253, #16530, #41311, #11557, #16288, #78712 ) ) ;
#71733=CARTESIAN_POINT ( 'NONE',  ( 10.06014724255809867, 1452.783669392659931, 210.4777447332699865 ) ) ;
#71734=CARTESIAN_POINT ( 'NONE',  ( 7.495582065179999809, 1424.824266038629958, 194.2083062206990007 ) ) ;
#71737=CARTESIAN_POINT ( 'NONE',  ( -4.447876660801433069, 1419.909382011105208, 194.3620334553881150 ) ) ;
#71751=ORIENTED_EDGE ( 'NONE', *, *, #62384, .T. ) ;
#71755=CARTESIAN_POINT ( 'NONE',  ( 2.045518813257909851, 1498.492502908489996, 197.9893470804480273 ) ) ;
#71756=VECTOR ( 'NONE', #49584, 1000.000000000000000 ) ;
#71757=CARTESIAN_POINT ( 'NONE',  ( -7.630521968176440240, 1469.354043036800022, 216.8955778692430272 ) ) ;
#71760=CARTESIAN_POINT ( 'NONE',  ( 1.548774059501979883, 1474.902113389930037, 220.4354346946340115 ) ) ;
#71763=CARTESIAN_POINT ( 'NONE',  ( -14.15252861969999820, 1503.726965476990017, 208.7499539689279970 ) ) ;
#71765=CARTESIAN_POINT ( 'NONE',  ( 11.55990587695049854, 1422.181602173609917, 207.1874422316890048 ) ) ;
#71766=VECTOR ( 'NONE', #91837, 999.9999999999997726 ) ;
#71774=CARTESIAN_POINT ( 'NONE',  ( 3.775314268589999855, 1507.374707634990045, 220.2027404231990033 ) ) ;
#71776=CARTESIAN_POINT ( 'NONE',  ( -16.16618494246800353, 1419.872609311620181, 210.0412365793670233 ) ) ;
#71777=ORIENTED_EDGE ( 'NONE', *, *, #81687, .T. ) ;
#71778=CARTESIAN_POINT ( 'NONE',  ( -15.88421513919616146, 1415.958925770876931, 209.7365058685432189 ) ) ;
#71780=CARTESIAN_POINT ( 'NONE',  ( 20.02377564230000218, 1475.402829072889972, 206.2263482165890025 ) ) ;
#71782=CARTESIAN_POINT ( 'NONE',  ( -0.6427045307039329636, 1430.099853101789904, 199.7385159216829891 ) ) ;
#71784=CARTESIAN_POINT ( 'NONE',  ( -3.829620113550000315, 1515.051704408389924, 209.0973262533439936 ) ) ;
#71786=CARTESIAN_POINT ( 'NONE',  ( 7.744112962519119847, 1460.365312253459933, 203.2200444182140018 ) ) ;
#71798=CARTESIAN_POINT ( 'NONE',  ( -3.829620113550000315, 1515.551704408389924, 211.4519800877889963 ) ) ;
#71800=CARTESIAN_POINT ( 'NONE',  ( 12.61325660393820058, 1426.953648319100012, 205.8283967020159935 ) ) ;
#71810=ORIENTED_EDGE ( 'NONE', *, *, #20778, .T. ) ;
#71814=CARTESIAN_POINT ( 'NONE',  ( -5.077887651979027694, 1463.916885366726319, 200.2638546281883123 ) ) ;
#71839=CARTESIAN_POINT ( 'NONE',  ( 19.05639497150000139, 1459.894456182490103, 220.3270700572990108 ) ) ;
#71846=CARTESIAN_POINT ( 'NONE',  ( 2173.981453289206911, -8382.262153571264207, -1556.947849745907888 ) ) ;
#71853=CARTESIAN_POINT ( 'NONE',  ( 8787.386475773348138, -2339.246371527899555, -2767.671033105199513 ) ) ;
#71854=CARTESIAN_POINT ( 'NONE',  ( -11.17519453696281140, 1422.142527340527977, 210.6369239073095798 ) ) ;
#71857=ORIENTED_EDGE ( 'NONE', *, *, #61177, .T. ) ;
#71860=DIRECTION ( 'NONE',  ( 0.9746209764380640017, 5.558287066451319365E-07, 0.2238614577961240137 ) ) ;
#71867=CARTESIAN_POINT ( 'NONE',  ( -1.636741585329999804, 1469.777368439289830, 219.0527109404189900 ) ) ;
#71869=CARTESIAN_POINT ( 'NONE',  ( 12.53490346717240023, 1501.124165648190001, 211.2564677464939962 ) ) ;
#71873=CARTESIAN_POINT ( 'NONE',  ( -7.110895733399999585, 1481.050959687990144, 207.2709231533789875 ) ) ;
#71876=CARTESIAN_POINT ( 'NONE',  ( -1.219629049478790028, 1431.745899841950177, 200.8064624575089852 ) ) ;
#71883=CARTESIAN_POINT ( 'NONE',  ( -3.116134553580160560, 1509.034509793703819, 204.6344886145632529 ) ) ;
#71884=CARTESIAN_POINT ( 'NONE',  ( 9.742642355230000106, 1463.575582522990089, 210.1498719498890182 ) ) ;
#71888=CARTESIAN_POINT ( 'NONE',  ( 0.1600667122320010294, 1463.646925499989948, 199.3014139421989910 ) ) ;
#71892=ORIENTED_EDGE ( 'NONE', *, *, #2155, .F. ) ;
#71894=CARTESIAN_POINT ( 'NONE',  ( 11.54563913674000020, 1478.900881724800001, 206.9376360146720231 ) ) ;
#71895=ORIENTED_EDGE ( 'NONE', *, *, #15100, .F. ) ;
#71898=CARTESIAN_POINT ( 'NONE',  ( -17.69340222479375058, 1508.456513906287682, 212.3435705202165025 ) ) ;
#71899=CARTESIAN_POINT ( 'NONE',  ( 8.249561420100000930, 1502.931132867190172, 210.0140376356389993 ) ) ;
#71905=CARTESIAN_POINT ( 'NONE',  ( -4.297012669169999910, 1508.497024723489858, 220.4589697836989899 ) ) ;
#71907=CARTESIAN_POINT ( 'NONE',  ( -0.004106634418278950170, 1498.706732373090063, 200.5431806547190092 ) ) ;
#71914=CARTESIAN_POINT ( 'NONE',  ( -11.44339780954279995, 1482.754209377100096, 205.8243739520100064 ) ) ;
#71922=CARTESIAN_POINT ( 'NONE',  ( -14.86532350809999947, 1415.677402202029953, 206.7896748190889866 ) ) ;
#71925=CARTESIAN_POINT ( 'NONE',  ( -15.46337563405010052, 1415.677402202039957, 209.5778891453549875 ) ) ;
#71934=CARTESIAN_POINT ( 'NONE',  ( -0.7620301703830010265, 1515.588179473189939, 213.1365024013990137 ) ) ;
#71938=CARTESIAN_POINT ( 'NONE',  ( -10.10200468158650011, 1447.143925580010091, 211.2823309413680022 ) ) ;
#71943=EDGE_CURVE ( 'NONE', #92278, #105852, #103188, .T. ) ;
#71946=CARTESIAN_POINT ( 'NONE',  ( 9.501613403289589144, 1467.857654184219882, 205.8614462207000031 ) ) ;
#71948=CARTESIAN_POINT ( 'NONE',  ( 19.38392212389999969, 1495.496321584190127, 199.6762541507190178 ) ) ;
#71953=CARTESIAN_POINT ( 'NONE',  ( 12.32716646574370145, 1492.190914138330072, 209.5898718627249764 ) ) ;
#71954=CARTESIAN_POINT ( 'NONE',  ( -10.49359245019999953, 1482.960578323189793, 204.4802844074689858 ) ) ;
#71966=CARTESIAN_POINT ( 'NONE',  ( -18.39846574424100112, 1508.551704408389924, 210.4158962701780240 ) ) ;
#71969=CARTESIAN_POINT ( 'NONE',  ( 7.278733183479999980, 1426.463158066219876, 212.8449153079989742 ) ) ;
#71970=CARTESIAN_POINT ( 'NONE',  ( -17.55008888309999904, 1487.029577685089862, 194.9701234138989889 ) ) ;
#71992=ORIENTED_EDGE ( 'NONE', *, *, #110291, .T. ) ;
#72017=ADVANCED_FACE ( 'NONE', ( #31450 ), #60837, .T. ) ;
#72024=CARTESIAN_POINT ( 'NONE',  ( 14.76737052841249920, 1427.310067236570148, 198.6611131540680049 ) ) ;
#72025=CARTESIAN_POINT ( 'NONE',  ( -0.03314418650357400103, 1502.038643116309913, 233.2541165707570201 ) ) ;
#72026=EDGE_CURVE ( 'NONE', #69447, #106884, #97782, .T. ) ;
#72032=EDGE_CURVE ( 'NONE', #78921, #328, #24386, .T. ) ;
#72035=CARTESIAN_POINT ( 'NONE',  ( -2.940135782350000060, 1428.954742266889980, 200.2247184200489869 ) ) ;
#72037=CARTESIAN_POINT ( 'NONE',  ( -0.6157698266020030786, 1500.133018751690088, 230.4529138410990186 ) ) ;
#72044=CARTESIAN_POINT ( 'NONE',  ( 10.08381526586729926, 1469.545492192299889, 207.5775108819740069 ) ) ;
#72048=ORIENTED_EDGE ( 'NONE', *, *, #80775, .T. ) ;
#72052=CARTESIAN_POINT ( 'NONE',  ( 9.044573916982399098, 1425.064980843364992, 195.6694192215943815 ) ) ;
#72054=CARTESIAN_POINT ( 'NONE',  ( -0.4938125538340010778, 1443.407940923189926, 218.3972833972489980 ) ) ;
#72058=CARTESIAN_POINT ( 'NONE',  ( -19.75056259240000145, 1465.177823603190063, 209.1218459616989946 ) ) ;
#72066=CARTESIAN_POINT ( 'NONE',  ( -16.52648624529999921, 1508.522148411690068, 213.6168893376890026 ) ) ;
#72074=CARTESIAN_POINT ( 'NONE',  ( 5.755594507168209084, 1494.343245214239914, 219.1208262999909948 ) ) ;
#72076=CARTESIAN_POINT ( 'NONE',  ( -8.494709194219998594, 1488.072329416189859, 217.7903042847989923 ) ) ;
#72077=CARTESIAN_POINT ( 'NONE',  ( -18.47517498779149747, 1466.235640218240178, 200.8822797504410005 ) ) ;
#72080=CARTESIAN_POINT ( 'NONE',  ( 5.773132394310000137, 1428.572103629089952, 215.3275095299590021 ) ) ;
#72081=CARTESIAN_POINT ( 'NONE',  ( -8.799999999999998934, 1412.913060387329779, 209.1218459616989946 ) ) ;
#72088=CARTESIAN_POINT ( 'NONE',  ( 2.475018581880529922, 1497.111080376900190, 196.9667223532030107 ) ) ;
#72094=CARTESIAN_POINT ( 'NONE',  ( -5.100957845159999948, 1482.122785942490054, 228.9672709512990139 ) ) ;
#72096=CARTESIAN_POINT ( 'NONE',  ( 6.413454494903159997, 1466.819085582309981, 216.7143828116000179 ) ) ;
#72101=CARTESIAN_POINT ( 'NONE',  ( -7.281830411814069315, 1478.108126808140014, 218.1541311745150153 ) ) ;
#72105=EDGE_LOOP ( 'NONE', ( #44501, #14326, #62209, #86413 ) ) ;
#72109=CARTESIAN_POINT ( 'NONE',  ( -11.69896337610000181, 1483.759246082390064, 228.3345905838990291 ) ) ;
#72115=CARTESIAN_POINT ( 'NONE',  ( 3.495214741176849937, 1484.713663407669856, 220.4421414041750040 ) ) ;
#72121=CARTESIAN_POINT ( 'NONE',  ( -7.800000000000001599, 1392.213060387289943, 209.1218459616989946 ) ) ;
#72129=CARTESIAN_POINT ( 'NONE',  ( -3.289314091018219699, 1497.168725298330173, 221.0708042131589934 ) ) ;
#72132=ADVANCED_FACE ( 'NONE', ( #72248 ), #17729, .T. ) ;
#72133=CARTESIAN_POINT ( 'NONE',  ( 6.024188629869999367, 1473.161425684690130, 217.8957855105489898 ) ) ;
#72135=VERTEX_POINT ( 'NONE', #108579 ) ;
#72144=CARTESIAN_POINT ( 'NONE',  ( 11.34298750825909963, 1471.339403186539812, 210.4402065159420090 ) ) ;
#72168=EDGE_CURVE ( 'NONE', #7001, #75598, #49800, .T. ) ;
#72175=CARTESIAN_POINT ( 'NONE',  ( -3.467940602053699806, 1495.562067921990092, 197.2905559617530002 ) ) ;
#72177=CARTESIAN_POINT ( 'NONE',  ( -13.54981492583890024, 1508.446256337960222, 216.7328168714189758 ) ) ;
#72186=CARTESIAN_POINT ( 'NONE',  ( 10.47998729271419904, 1499.735940323320165, 203.4895150079940151 ) ) ;
#72192=CARTESIAN_POINT ( 'NONE',  ( 12.01579051976940171, 1501.533415298749787, 211.5805978092899977 ) ) ;
#72193=EDGE_CURVE ( 'NONE', #31705, #42338, #67945, .T. ) ;
#72194=CARTESIAN_POINT ( 'NONE',  ( -16.33084092821613709, 1420.150255326767819, 208.9983406252053726 ) ) ;
#72201=ORIENTED_EDGE ( 'NONE', *, *, #42824, .T. ) ;
#72204=CARTESIAN_POINT ( 'NONE',  ( -3.265595362850000072, 1475.097840200290193, 198.5785976524989849 ) ) ;
#72207=CARTESIAN_POINT ( 'NONE',  ( -3.005266857462870256, 1450.300088869250203, 188.5532293206870236 ) ) ;
#72208=ORIENTED_EDGE ( 'NONE', *, *, #39971, .F. ) ;
#72214=CARTESIAN_POINT ( 'NONE',  ( -15.03789156734744381, 1420.076630009843029, 212.7487531976570097 ) ) ;
#72221=CARTESIAN_POINT ( 'NONE',  ( 11.15330175375659927, 1491.129753307649935, 208.9113124793660177 ) ) ;
#72240=FACE_OUTER_BOUND ( 'NONE', #39185, .T. ) ;
#72248=FACE_OUTER_BOUND ( 'NONE', #86543, .T. ) ;
#72251=ORIENTED_EDGE ( 'NONE', *, *, #56340, .F. ) ;
#72256=ORIENTED_EDGE ( 'NONE', *, *, #40299, .F. ) ;
#72257=CARTESIAN_POINT ( 'NONE',  ( 10.11443659974309917, 1452.508654505240202, 209.7494611922460024 ) ) ;
#72270=CARTESIAN_POINT ( 'NONE',  ( 5.436197771951739810, 1483.947504832600089, 219.6404701149249945 ) ) ;
#72271=EDGE_CURVE ( 'NONE', #86829, #46077, #91019, .T. ) ;
#72279=CARTESIAN_POINT ( 'NONE',  ( -8.451373773768418474, 1470.993491901630023, 214.7957158758800063 ) ) ;
#72281=CARTESIAN_POINT ( 'NONE',  ( 8.743785848119999926, 1420.947065512389827, 196.4302455952989703 ) ) ;
#72283=CARTESIAN_POINT ( 'NONE',  ( -4.633397090840619903, 1377.913060387289988, 204.3568503472270095 ) ) ;
#72286=CARTESIAN_POINT ( 'NONE',  ( -16.32500455070000100, 1504.098762924189941, 208.8919858110830035 ) ) ;
#72289=CARTESIAN_POINT ( 'NONE',  ( -9.526128307108560733, 1440.436522615020067, 205.9995050262249947 ) ) ;
#72296=ADVANCED_FACE ( 'NONE', ( #36706 ), #50820, .T. ) ;
#72297=B_SPLINE_SURFACE_WITH_KNOTS ( 'NONE', 5, 1, ( 
 ( #11056, #54732 ),
 ( #79365, #79917 ),
 ( #105677, #55280 ),
 ( #54184, #2679 ),
 ( #96155, #10496 ),
 ( #36249, #88860 ),
 ( #70995, #87775 ),
 ( #36804, #28404 ),
 ( #81007, #72094 ) ),
 .UNSPECIFIED., .F., .F., .F.,
 ( 6, 3, 6 ),
 ( 2, 2 ),
 ( 0.000000000000000000, 3.871851108280000009, 7.729255844190000779 ),
 ( 0.000000000000000000, 14.00000000000000000 ),
 .UNSPECIFIED. ) ;
#72298=CARTESIAN_POINT ( 'NONE',  ( 5.423172162180000200, 1506.748560102689908, 219.4673452336990067 ) ) ;
#72300=CARTESIAN_POINT ( 'NONE',  ( -15.28618265780000129, 1416.164270469039820, 211.6194353647389903 ) ) ;
#72301=CARTESIAN_POINT ( 'NONE',  ( -17.84478100760759745, 1419.380458095060021, 206.8875292346940000 ) ) ;
#72302=ORIENTED_EDGE ( 'NONE', *, *, #37770, .T. ) ;
#72303=CARTESIAN_POINT ( 'NONE',  ( 3.355048246850000471, 1428.659755942190031, 216.6919371868989970 ) ) ;
#72305=CARTESIAN_POINT ( 'NONE',  ( -16.48345269260000023, 1416.839564662629982, 208.3476362942829780 ) ) ;
#72306=CARTESIAN_POINT ( 'NONE',  ( 1.419401350206249912, 1430.917749770590035, 199.7704084515799821 ) ) ;
#72317=EDGE_CURVE ( 'NONE', #86947, #89851, #71576, .T. ) ;
#72322=CARTESIAN_POINT ( 'NONE',  ( 12.46349861749770049, 1427.083103380439752, 206.6193291359699913 ) ) ;
#72334=CARTESIAN_POINT ( 'NONE',  ( 2.961801441480000019, 1478.312073041489839, 199.0497942763989840 ) ) ;
#72336=CARTESIAN_POINT ( 'NONE',  ( -11.16049073669999991, 1491.416285126389994, 208.9675611111450166 ) ) ;
#72338=CARTESIAN_POINT ( 'NONE',  ( -8.590093507847479160, 1437.218756716850066, 210.0971559123210000 ) ) ;
#72341=CARTESIAN_POINT ( 'NONE',  ( -11.60954088560589881, 1481.114764782069869, 211.3792897891370046 ) ) ;
#72346=CARTESIAN_POINT ( 'NONE',  ( -8.770356860863364190, 1423.116964779634145, 210.6628905271092265 ) ) ;
#72352=CARTESIAN_POINT ( 'NONE',  ( -9.442895466421070694, 1461.069229439506216, 206.8582801283209847 ) ) ;
#72354=CARTESIAN_POINT ( 'NONE',  ( 3.375977092230000309, 1446.395221922789915, 199.5681764357789802 ) ) ;
#72359=CARTESIAN_POINT ( 'NONE',  ( -19.58883600250999635, 1465.811282985779826, 204.1485273088549945 ) ) ;
#72366=CARTESIAN_POINT ( 'NONE',  ( 203.9558787908000284, -8382.262153571269664, -1760.903728536709878 ) ) ;
#72373=CARTESIAN_POINT ( 'NONE',  ( 11.41987517966060039, 1502.185978170540011, 211.2996822900650216 ) ) ;
#72374=CARTESIAN_POINT ( 'NONE',  ( -12.46225008516609556, 1421.619546445686638, 210.6462345555370916 ) ) ;
#72378=ORIENTED_EDGE ( 'NONE', *, *, #53610, .F. ) ;
#72381=CARTESIAN_POINT ( 'NONE',  ( 0.9962946536900849637, 1485.568703864239978, 220.9525874579420019 ) ) ;
#72389=CARTESIAN_POINT ( 'NONE',  ( 7.628187097038660269, 1483.025225563630102, 218.3251324470150223 ) ) ;
#72393=CARTESIAN_POINT ( 'NONE',  ( 4.554071316310000839, 1435.609063005990038, 205.7950640489989951 ) ) ;
#72397=ORIENTED_EDGE ( 'NONE', *, *, #95886, .T. ) ;
#72405=DIRECTION ( 'NONE',  ( 0.7616194158028416483, 1.190401854521374756E-16, 0.6480245870892076265 ) ) ;
#72419=CARTESIAN_POINT ( 'NONE',  ( -18.14127185173783019, 1508.457047458428633, 211.6720055858629337 ) ) ;
#72421=CARTESIAN_POINT ( 'NONE',  ( -6.806372913706649541, 1435.357145811779901, 216.0422613199140187 ) ) ;
#72442=CARTESIAN_POINT ( 'NONE',  ( -4.238023215140263034, 1486.921097696548031, 220.3845390032697367 ) ) ;
#72443=CARTESIAN_POINT ( 'NONE',  ( -14.68843015960000109, 1416.151303865629870, 204.4183550279689712 ) ) ;
#72445=CARTESIAN_POINT ( 'NONE',  ( 11.78588353789999843, 1420.143588805510035, 199.1665921514089916 ) ) ;
#72446=AXIS2_PLACEMENT_3D ( 'NONE', #90680, #73347, #89582 ) ;
#72455=CARTESIAN_POINT ( 'NONE',  ( 1.842963900900000063, 1515.551704191689851, 212.9514661349190021 ) ) ;
#72457=CARTESIAN_POINT ( 'NONE',  ( 1.150023946295242183, 1463.916996383109336, 199.3782771554538442 ) ) ;
#72458=CARTESIAN_POINT ( 'NONE',  ( 13.72029690906714805, 1499.818747152161222, 226.3681697707128251 ) ) ;
#72459=FACE_OUTER_BOUND ( 'NONE', #78440, .T. ) ;
#72461=CARTESIAN_POINT ( 'NONE',  ( -7.604289863101939773, 1426.735970264149955, 206.0920986175900111 ) ) ;
#72464=CARTESIAN_POINT ( 'NONE',  ( -4.138543415650000057, 1515.492058123790002, 210.9648098330690118 ) ) ;
#72478=CARTESIAN_POINT ( 'NONE',  ( -2.487934962309999776, 1508.551704408389924, 204.1347675205190058 ) ) ;
#72480=ORIENTED_EDGE ( 'NONE', *, *, #80775, .F. ) ;
#72481=CARTESIAN_POINT ( 'NONE',  ( -11.33349574978999819, 1502.222612973462901, 207.2846957396286598 ) ) ;
#72482=CARTESIAN_POINT ( 'NONE',  ( -13.58135394501369930, 1508.550209656430070, 210.2785163480139943 ) ) ;
#72484=CARTESIAN_POINT ( 'NONE',  ( -6.509625120830000000, 1510.892449458290002, 215.5197494809989962 ) ) ;
#72488=CARTESIAN_POINT ( 'NONE',  ( -9.066559479250001274, 1450.410201457089897, 206.4479026976190141 ) ) ;
#72490=CARTESIAN_POINT ( 'NONE',  ( 7.958039864590000789, 1426.668732447519915, 211.8424160901890048 ) ) ;
#72496=CARTESIAN_POINT ( 'NONE',  ( 8.572313988419999475, 1452.460948930489849, 212.8151060300189954 ) ) ;
#72498=VERTEX_POINT ( 'NONE', #12610 ) ;
#72526=CARTESIAN_POINT ( 'NONE',  ( -18.72256362461450152, 1508.551704408389924, 209.8107881426000176 ) ) ;
#72529=CIRCLE ( 'NONE', #8078, 4.250000000000000000 ) ;
#72533=CARTESIAN_POINT ( 'NONE',  ( -12.20950249781779995, 1490.126853475539974, 210.0346353896779874 ) ) ;
#72538=ORIENTED_EDGE ( 'NONE', *, *, #72632, .F. ) ;
#72539=CARTESIAN_POINT ( 'NONE',  ( -3.677613769069999778E-16, 1378.399971913189802, 209.1218459616989946 ) ) ;
#72542=CARTESIAN_POINT ( 'NONE',  ( 10.95098205620359977, 1471.837422849929908, 212.3987392730099657 ) ) ;
#72548=CARTESIAN_POINT ( 'NONE',  ( 5.440512190109999757, 1424.738065781850082, 191.9794586101990319 ) ) ;
#72555=ORIENTED_EDGE ( 'NONE', *, *, #72168, .F. ) ;
#72562=CARTESIAN_POINT ( 'NONE',  ( 11.52804851922353890, 1414.677402202029953, 211.3132271615170623 ) ) ;
#72564=CARTESIAN_POINT ( 'NONE',  ( 11.34922769319999958, 1426.257359350699971, 206.1386472418390099 ) ) ;
#72565=CARTESIAN_POINT ( 'NONE',  ( -2.240533496870801944, 1497.807162272345067, 198.0577364717022419 ) ) ;
#72567=CARTESIAN_POINT ( 'NONE',  ( -16.18244964864798163, 1416.494914503025257, 208.5996723762598037 ) ) ;
#72568=CARTESIAN_POINT ( 'NONE',  ( 9.529616025180215999, 1459.343410991622932, 203.7689766306496040 ) ) ;
#72569=CARTESIAN_POINT ( 'NONE',  ( 11.41166285218010046, 1470.995102172900033, 209.2012249493139961 ) ) ;
#72574=DIRECTION ( 'NONE',  ( -1.224646799147353207E-16, -1.836970198721029688E-16, -1.000000000000000000 ) ) ;
#72575=B_SPLINE_CURVE_WITH_KNOTS ( 'NONE', 5,
 ( #100681, #107433, #6083, #73858, #22859, #22300 ),
 .UNSPECIFIED., .F., .F.,
 ( 6, 6 ),
 ( 0.000000000000000000, 1.000000000000000000 ),
 .UNSPECIFIED. ) ;
#72577=CARTESIAN_POINT ( 'NONE',  ( 9.651063919191019025, 1425.440657924460083, 195.4941620015079877 ) ) ;
#72578=CARTESIAN_POINT ( 'NONE',  ( 1.042629999269999885, 1442.250188905790083, 219.0243665098589929 ) ) ;
#72582=CARTESIAN_POINT ( 'NONE',  ( 9.947665014826124974, 1488.618077319816621, 204.6704152026359793 ) ) ;
#72589=CARTESIAN_POINT ( 'NONE',  ( -9.549500093889998098, 1508.435385506690182, 218.9685490284190053 ) ) ;
#72590=DIRECTION ( 'NONE',  ( -9.152776640618289361E-47, 1.000000000000000000, -1.836970198721029688E-16 ) ) ;
#72592=CARTESIAN_POINT ( 'NONE',  ( 10.62769165429999951, 1422.391598617170075, 210.1052261204159777 ) ) ;
#72593=CARTESIAN_POINT ( 'NONE',  ( -2.936010229900000379, 1484.512606866390115, 198.6791449311989766 ) ) ;
#72598=CARTESIAN_POINT ( 'NONE',  ( 4.028444003397729567, 1493.864063547320029, 219.5261911965480124 ) ) ;
#72599=CARTESIAN_POINT ( 'NONE',  ( -4.705750868621540128, 1479.984690096089935, 230.9466464819849989 ) ) ;
#72601=CARTESIAN_POINT ( 'NONE',  ( -15.44962914106915441, 1415.677402202029953, 209.5155034275957746 ) ) ;
#72602=DIRECTION ( 'NONE',  ( -9.138167445698339565E-47, 1.000000000000000000, -1.836970198721029688E-16 ) ) ;
#72603=CARTESIAN_POINT ( 'NONE',  ( 5.311406560260000020, 1429.286496272289924, 216.0669640761489916 ) ) ;
#72604=CARTESIAN_POINT ( 'NONE',  ( 4.900006679340000559, 1499.255191946190052, 229.7873568473989963 ) ) ;
#72605=ORIENTED_EDGE ( 'NONE', *, *, #55698, .T. ) ;
#72608=ORIENTED_EDGE ( 'NONE', *, *, #76582, .T. ) ;
#72621=CARTESIAN_POINT ( 'NONE',  ( 0.1783569641990820354, 1515.156623775960043, 213.4488900611540032 ) ) ;
#72632=EDGE_CURVE ( 'NONE', #89343, #73491, #51867, .T. ) ;
#72633=CARTESIAN_POINT ( 'NONE',  ( 9.636843969170000079, 1494.191090576590113, 188.1746674836989826 ) ) ;
#72635=CARTESIAN_POINT ( 'NONE',  ( 7.439417113980000273, 1422.547532122410075, 195.6475770543989938 ) ) ;
#72641=CARTESIAN_POINT ( 'NONE',  ( 4.327495487223619541, 1515.139385973049912, 209.7044482359050050 ) ) ;
#72643=LINE ( 'NONE', #3803, #87295 ) ;
#72644=CARTESIAN_POINT ( 'NONE',  ( 0.5257072283710009231, 1456.163790123490116, 198.9387035231989955 ) ) ;
#72651=ORIENTED_EDGE ( 'NONE', *, *, #86358, .F. ) ;
#72653=CARTESIAN_POINT ( 'NONE',  ( -8.728534304065659555, 1447.922708812389828, 212.1734976818020186 ) ) ;
#72667=CARTESIAN_POINT ( 'NONE',  ( 9.744580062524020647, 1435.065973224739992, 208.0102391462599769 ) ) ;
#72673=CARTESIAN_POINT ( 'NONE',  ( 10.99606214793050007, 1471.801637878359998, 212.2474561802740141 ) ) ;
#72684=ORIENTED_EDGE ( 'NONE', *, *, #97074, .T. ) ;
#72693=CARTESIAN_POINT ( 'NONE',  ( -11.80614671260000037, 1416.487503907969767, 205.3428939757990008 ) ) ;
#72702=ORIENTED_EDGE ( 'NONE', *, *, #9660, .T. ) ;
#72711=CARTESIAN_POINT ( 'NONE',  ( -1.430539248151910137, 1444.328264662749916, 199.1703804428329931 ) ) ;
#72718=CARTESIAN_POINT ( 'NONE',  ( 10.92768932611909882, 1501.618341437669869, 205.6861941585989939 ) ) ;
#72720=CARTESIAN_POINT ( 'NONE',  ( 11.33311166264400072, 1479.605569753980035, 208.8962439930940036 ) ) ;
#72723=CARTESIAN_POINT ( 'NONE',  ( -3.648559762950000174, 1443.531551953690041, 199.7293442341890000 ) ) ;
#72725=FACE_OUTER_BOUND ( 'NONE', #54788, .T. ) ;
#72728=CARTESIAN_POINT ( 'NONE',  ( -4.544862314595019548, 1508.551704408290107, 205.1599765735010124 ) ) ;
#72737=CARTESIAN_POINT ( 'NONE',  ( -3.152270363119999974, 1474.954422145789977, 198.1306181043989909 ) ) ;
#72739=EDGE_LOOP ( 'NONE', ( #105374, #18292, #2558, #86164 ) ) ;
#72740=CARTESIAN_POINT ( 'NONE',  ( -19.34950756859469934, 1446.106588470199995, 200.0047979462570140 ) ) ;
#72746=CARTESIAN_POINT ( 'NONE',  ( 3.554051323329999956, 1466.352086058089981, 219.5854740514990056 ) ) ;
#72747=CARTESIAN_POINT ( 'NONE',  ( -10.06682062296219904, 1472.945273473310181, 207.3391469858899825 ) ) ;
#72751=FACE_OUTER_BOUND ( 'NONE', #83307, .T. ) ;
#72765=CARTESIAN_POINT ( 'NONE',  ( -15.58093640500000099, 1419.947093784519893, 211.3491018407289914 ) ) ;
#72771=EDGE_CURVE ( 'NONE', #97433, #53857, #96394, .T. ) ;
#72773=CARTESIAN_POINT ( 'NONE',  ( -2.664535259099999805E-15, 1424.786834349990158, 209.1218459616989946 ) ) ;
#72779=CARTESIAN_POINT ( 'NONE',  ( 1.502806645429999977, 1497.907953363189790, 197.7820368093990169 ) ) ;
#72784=CARTESIAN_POINT ( 'NONE',  ( -12.99775963039999915, 1420.302662752830201, 196.1023006302990268 ) ) ;
#72789=CARTESIAN_POINT ( 'NONE',  ( -0.6032294603500010233, 1487.495129746489965, 219.9704429636989857 ) ) ;
#72794=CARTESIAN_POINT ( 'NONE',  ( -19.75056259240000145, 1465.177823603190063, 209.1218459616989946 ) ) ;
#72796=EDGE_LOOP ( 'NONE', ( #26861, #81172, #70217, #68549 ) ) ;
#72798=EDGE_CURVE ( 'NONE', #43776, #34771, #44764, .T. ) ;
#72813=CARTESIAN_POINT ( 'NONE',  ( -3.430374836980000008, 1431.708658569990121, 216.7924588047190184 ) ) ;
#72814=CARTESIAN_POINT ( 'NONE',  ( 10.02421119480000122, 1480.534221758890226, 205.8829018067289951 ) ) ;
#72822=CARTESIAN_POINT ( 'NONE',  ( 12.57118999910000134, 1420.461935673439939, 200.4069075869790026 ) ) ;
#72823=CARTESIAN_POINT ( 'NONE',  ( -1.360835085989610116, 1475.742324412110065, 220.4819849918339969 ) ) ;
#72831=CARTESIAN_POINT ( 'NONE',  ( -9.860305081645158509, 1439.899766047359890, 207.4024662252320184 ) ) ;
#72833=EDGE_LOOP ( 'NONE', ( #21246, #79264, #50168, #65730 ) ) ;
#72840=CARTESIAN_POINT ( 'NONE',  ( -17.11352124978379763, 1419.945169622900039, 207.4943747003180192 ) ) ;
#72842=FACE_OUTER_BOUND ( 'NONE', #62717, .T. ) ;
#72845=FACE_OUTER_BOUND ( 'NONE', #28986, .T. ) ;
#72848=CARTESIAN_POINT ( 'NONE',  ( 5.062170296090039656, 1457.731097799089866, 200.0536533579299885 ) ) ;
#72854=CARTESIAN_POINT ( 'NONE',  ( 2.281064403174069888, 1474.722235171090006, 220.3124694468160101 ) ) ;
#72871=VERTEX_POINT ( 'NONE', #40282 ) ;
#72875=CARTESIAN_POINT ( 'NONE',  ( -11.02929229669999955, 1491.798645198889972, 209.3597145180599739 ) ) ;
#72883=CARTESIAN_POINT ( 'NONE',  ( -12.02742519731079973, 1491.141813116759977, 206.6978330293360102 ) ) ;
#72884=CARTESIAN_POINT ( 'NONE',  ( -4.626713179916450258, 1508.551704408389924, 205.3420549087489917 ) ) ;
#72891=CARTESIAN_POINT ( 'NONE',  ( -11.25082884059999877, 1500.153667613989910, 210.9046300046090039 ) ) ;
#72897=CARTESIAN_POINT ( 'NONE',  ( -20.42726709853700129, 1466.741775361090049, 211.1910253039249881 ) ) ;
#72903=CARTESIAN_POINT ( 'NONE',  ( -2173.981453289206911, -8382.262153571264207, 1975.191541669308435 ) ) ;
#72905=CONICAL_SURFACE ( 'NONE', #78329, 6.911399307709998219, 0.04363323129990067523 ) ;
#72911=CARTESIAN_POINT ( 'NONE',  ( -4.378216884482949212, 1453.707746088449994, 199.6107954155660025 ) ) ;
#72912=CARTESIAN_POINT ( 'NONE',  ( -10.44405160111380759, 1422.438935318351241, 210.6442778920145429 ) ) ;
#72915=EDGE_LOOP ( 'NONE', ( #20304, #85863 ) ) ;
#72920=CARTESIAN_POINT ( 'NONE',  ( -1.888943442820300023, 1486.364918105139850, 220.8936722016070178 ) ) ;
#72921=CARTESIAN_POINT ( 'NONE',  ( 12.34024189100000157, 1499.852123274089990, 206.2429094169490043 ) ) ;
#72932=CARTESIAN_POINT ( 'NONE',  ( -17.66147422859999949, 1440.150478811289986, 218.7822781203190061 ) ) ;
#72935=ORIENTED_EDGE ( 'NONE', *, *, #16095, .T. ) ;
#72937=FACE_OUTER_BOUND ( 'NONE', #64902, .T. ) ;
#72951=CARTESIAN_POINT ( 'NONE',  ( 9.688817234588901428, 1462.677202180080030, 207.9888309564389886 ) ) ;
#72953=ORIENTED_EDGE ( 'NONE', *, *, #61441, .T. ) ;
#72958=CARTESIAN_POINT ( 'NONE',  ( 8.303833566477019090, 1428.472849154070218, 213.7034505198590182 ) ) ;
#72959=CARTESIAN_POINT ( 'NONE',  ( -17.40244824282851255, 1508.456020371283103, 212.7521859866272678 ) ) ;
#72960=CARTESIAN_POINT ( 'NONE',  ( 21.08771820830000010, 1497.249269049990062, 211.1908499358290214 ) ) ;
#72961=CARTESIAN_POINT ( 'NONE',  ( -7.845903147674250455, 1436.115355770489941, 214.9328208583779940 ) ) ;
#72971=CARTESIAN_POINT ( 'NONE',  ( -10.23881579017958643, 1480.796270772398884, 206.5571936345679376 ) ) ;
#72976=CARTESIAN_POINT ( 'NONE',  ( -4.501970322318059381, 1483.174855501109960, 199.4671179167419837 ) ) ;
#72982=CARTESIAN_POINT ( 'NONE',  ( -20.69918688649430294, 1486.905067481629885, 208.2779964567390039 ) ) ;
#72983=CARTESIAN_POINT ( 'NONE',  ( -6.985287221996019369, 1440.244100505809911, 203.7176696286690287 ) ) ;
#72990=CARTESIAN_POINT ( 'NONE',  ( 19.09822630769999918, 1458.162647406989890, 212.8926528854489959 ) ) ;
#72993=CIRCLE ( 'NONE', #10389, 15.40132948099999943 ) ;
#72995=CARTESIAN_POINT ( 'NONE',  ( 0.7331377668379990276, 1515.470556211590065, 213.3402424911989783 ) ) ;
#73002=DIRECTION ( 'NONE',  ( -1.000000000000000000, 0.000000000000000000, 0.000000000000000000 ) ) ;
#73013=CARTESIAN_POINT ( 'NONE',  ( 8.784743044050069116, 1452.237884045540113, 212.1741271052380000 ) ) ;
#73017=CARTESIAN_POINT ( 'NONE',  ( 3.744429477602492895, 1509.032014137963188, 213.3627840903013180 ) ) ;
#73018=CARTESIAN_POINT ( 'NONE',  ( 12.32485495299399858, 1492.010170158399887, 208.9028815630869929 ) ) ;
#73029=DIRECTION ( 'NONE',  ( -8.555280247707230573E-26, -1.000000000000000000, 1.836970198721029688E-16 ) ) ;
#73033=CARTESIAN_POINT ( 'NONE',  ( -4.378216172770000192, 1453.707746473490033, 199.6107950798590025 ) ) ;
#73035=CARTESIAN_POINT ( 'NONE',  ( 12.24365541422369930, 1500.600794001439908, 208.6479367469619888 ) ) ;
#73036=CARTESIAN_POINT ( 'NONE',  ( -5.586162938070000195, 1491.245995699590139, 185.8699225748990216 ) ) ;
#73044=ADVANCED_FACE ( 'NONE', ( #79966 ), #16174, .T. ) ;
#73054=CARTESIAN_POINT ( 'NONE',  ( -5.302730571406519822, 1464.205385412599981, 199.9536530435450175 ) ) ;
#73061=EDGE_LOOP ( 'NONE', ( #99890, #14114, #29655, #5065, #9800, #95064 ) ) ;
#73065=VERTEX_POINT ( 'NONE', #44730 ) ;
#73067=CARTESIAN_POINT ( 'NONE',  ( 20.69709747799999988, 1495.539518117790067, 213.2340985757189742 ) ) ;
#73074=ORIENTED_EDGE ( 'NONE', *, *, #74106, .T. ) ;
#73075=CARTESIAN_POINT ( 'NONE',  ( -18.67382096187029816, 1508.542127769639819, 210.2892683469680151 ) ) ;
#73078=EDGE_CURVE ( 'NONE', #52143, #77481, #20579, .T. ) ;
#73081=VERTEX_POINT ( 'NONE', #107910 ) ;
#73082=CARTESIAN_POINT ( 'NONE',  ( -8.099792069101098946, 1452.596710452009802, 204.5152729218939669 ) ) ;
#73097=CARTESIAN_POINT ( 'NONE',  ( 14.05303364027069968, 1427.055417490390028, 197.7369918085530003 ) ) ;
#73109=CARTESIAN_POINT ( 'NONE',  ( 12.11317892429999965, 1426.372560516109843, 203.9710410313989826 ) ) ;
#73112=CARTESIAN_POINT ( 'NONE',  ( 9.788554748827010599, 1435.243870499410150, 208.4607419128279844 ) ) ;
#73114=CARTESIAN_POINT ( 'NONE',  ( 10.06361417826360061, 1469.502718807920019, 207.4652888198990013 ) ) ;
#73123=CARTESIAN_POINT ( 'NONE',  ( 1.569168191259999956, 1442.549728379589851, 218.2360776051089886 ) ) ;
#73127=CARTESIAN_POINT ( 'NONE',  ( 4.431405375871572794, 1485.802552508792360, 199.2752504294042524 ) ) ;
#73132=CARTESIAN_POINT ( 'NONE',  ( -9.699660872752350116, 1472.030908259890111, 212.1562907213800031 ) ) ;
#73135=CARTESIAN_POINT ( 'NONE',  ( -15.59348407829999950, 1508.491154456789900, 214.8963640716490033 ) ) ;
#73137=CARTESIAN_POINT ( 'NONE',  ( -5.292247061280000331, 1391.613060387290034, 209.1218459616989946 ) ) ;
#73149=CARTESIAN_POINT ( 'NONE',  ( 5.009886284249999377, 1430.069699660889910, 217.1776678749689893 ) ) ;
#73150=CARTESIAN_POINT ( 'NONE',  ( 7.359652241210000057, 1491.427741320190080, 211.7193137660989919 ) ) ;
#73151=ORIENTED_EDGE ( 'NONE', *, *, #56832, .F. ) ;
#73163=CARTESIAN_POINT ( 'NONE',  ( 3.250000000000000444, 1524.551704408390151, 209.1218459616989946 ) ) ;
#73170=CARTESIAN_POINT ( 'NONE',  ( -8.143105617842628874, 1478.527044422649851, 217.4342497289609923 ) ) ;
#73174=VERTEX_POINT ( 'NONE', #101147 ) ;
#73176=CARTESIAN_POINT ( 'NONE',  ( -12.81343579419999834, 1504.349109748190131, 208.8281390619199840 ) ) ;
#73177=CARTESIAN_POINT ( 'NONE',  ( 24.05733473906539999, 1495.051195187770190, 207.1050250271510151 ) ) ;
#73183=CARTESIAN_POINT ( 'NONE',  ( 5.170554601400000116, 1484.055082523290139, 219.7711189574989703 ) ) ;
#73185=CARTESIAN_POINT ( 'NONE',  ( -5.208772481359999595, 1458.757019672090109, 218.5248626948989852 ) ) ;
#73194=CARTESIAN_POINT ( 'NONE',  ( -8.673948557444399299, 1448.059622049680002, 212.1973933741120106 ) ) ;
#73201=ORIENTED_EDGE ( 'NONE', *, *, #41183, .F. ) ;
#73204=AXIS2_PLACEMENT_3D ( 'NONE', #87630, #37771, #38850 ) ;
#73208=CARTESIAN_POINT ( 'NONE',  ( -5.889293977349999487, 1482.137417484389971, 204.3352348937889928 ) ) ;
#73219=DIRECTION ( 'NONE',  ( -9.341989762165448955E-47, 1.000000000000000000, -1.836970198721029688E-16 ) ) ;
#73222=CARTESIAN_POINT ( 'NONE',  ( 6.844748814533139658, 1439.290426551219753, 215.8329238270310100 ) ) ;
#73236=B_SPLINE_CURVE_WITH_KNOTS ( 'NONE', 5,
 ( #58282, #100804, #15142, #15679, #49883, #101342 ),
 .UNSPECIFIED., .F., .F.,
 ( 6, 6 ),
 ( 0.000000000000000000, 1.000000000000000000 ),
 .UNSPECIFIED. ) ;
#73247=EDGE_CURVE ( 'NONE', #29545, #26775, #109589, .T. ) ;
#73255=CARTESIAN_POINT ( 'NONE',  ( -3.047096304819949975, 1454.406456363820098, 199.0892365841679919 ) ) ;
#73262=VERTEX_POINT ( 'NONE', #95266 ) ;
#73263=CARTESIAN_POINT ( 'NONE',  ( 11.33998819790270041, 1479.686981350909946, 209.1734062345460075 ) ) ;
#73265=CARTESIAN_POINT ( 'NONE',  ( -2.349897617149999896, 1443.007235233090114, 200.3879200387590060 ) ) ;
#73267=DIRECTION ( 'NONE',  ( -3.697785493223495027E-32, -1.000000000000000000, 1.836970198721029688E-16 ) ) ;
#73273=CARTESIAN_POINT ( 'NONE',  ( -11.43788434358669903, 1501.179491375600037, 208.6405304903099989 ) ) ;
#73281=CARTESIAN_POINT ( 'NONE',  ( -3.046862472289999513, 1475.471993788190048, 198.8673669194990339 ) ) ;
#73284=CARTESIAN_POINT ( 'NONE',  ( -20.43379687057499794, 1466.940231432759902, 211.2182850803170027 ) ) ;
#73289=CARTESIAN_POINT ( 'NONE',  ( -3.912777227685780179, 1515.493283046529996, 205.6567642959410023 ) ) ;
#73293=CARTESIAN_POINT ( 'NONE',  ( -5.534112078819999780, 1464.371868428389917, 199.5915707823590139 ) ) ;
#73295=CARTESIAN_POINT ( 'NONE',  ( 20.97480781879999867, 1494.611541218489947, 207.0969001841590114 ) ) ;
#73304=ORIENTED_EDGE ( 'NONE', *, *, #50153, .T. ) ;
#73310=CARTESIAN_POINT ( 'NONE',  ( -14.57096372540000040, 1420.584117712579882, 213.1076017662689992 ) ) ;
#73314=CARTESIAN_POINT ( 'NONE',  ( 9.374720191569998917, 1498.531797635389921, 228.6938383677990316 ) ) ;
#73317=CARTESIAN_POINT ( 'NONE',  ( -9.983087554349619808, 1446.969730184950095, 211.7543459487629889 ) ) ;
#73323=CARTESIAN_POINT ( 'NONE',  ( 7.366488175266259653, 1425.086169979620081, 212.5226571148190260 ) ) ;
#73327=FACE_OUTER_BOUND ( 'NONE', #39886, .T. ) ;
#73337=CARTESIAN_POINT ( 'NONE',  ( -3.286480964850000408, 1456.341185808290220, 218.0120306903490075 ) ) ;
#73347=DIRECTION ( 'NONE',  ( 0.000000000000000000, 1.000000000000000000, -1.836970198721029688E-16 ) ) ;
#73348=EDGE_CURVE ( 'NONE', #51048, #14195, #97465, .T. ) ;
#73354=CARTESIAN_POINT ( 'NONE',  ( -7.096551626949999303, 1426.600319239269993, 204.6398483329990086 ) ) ;
#73357=CARTESIAN_POINT ( 'NONE',  ( 9.855039225750559240, 1481.788109175460022, 215.6330005400349705 ) ) ;
#73358=AXIS2_PLACEMENT_3D ( 'NONE', #76418, #60755, #94879 ) ;
#73362=VERTEX_POINT ( 'NONE', #72283 ) ;
#73363=CARTESIAN_POINT ( 'NONE',  ( -11.00403485397939995, 1481.586315828709985, 208.5475605672099846 ) ) ;
#73367=CARTESIAN_POINT ( 'NONE',  ( 11.32581438617719982, 1502.327464439309779, 214.9380970868279803 ) ) ;
#73369=CARTESIAN_POINT ( 'NONE',  ( 8.768419210700001187, 1421.106171289960002, 196.5082349784990186 ) ) ;
#73370=CARTESIAN_POINT ( 'NONE',  ( 0.6402605648741300781, 1475.143224049549872, 220.5254527812860204 ) ) ;
#73376=CARTESIAN_POINT ( 'NONE',  ( 11.07919842396059984, 1425.821831854960010, 206.4952777197320017 ) ) ;
#73380=ORIENTED_EDGE ( 'NONE', *, *, #73348, .F. ) ;
#73383=CARTESIAN_POINT ( 'NONE',  ( -17.00293377828755581, 1417.375270068509735, 206.8726622690845431 ) ) ;
#73388=CARTESIAN_POINT ( 'NONE',  ( -15.57735599724670017, 1420.358456224219935, 210.5575541888260034 ) ) ;
#73390=EDGE_CURVE ( 'NONE', #78921, #67457, #50888, .T. ) ;
#73391=CARTESIAN_POINT ( 'NONE',  ( 3.075808390909999801, 1430.545926202089959, 217.6856249740289968 ) ) ;
#73397=CARTESIAN_POINT ( 'NONE',  ( 1.145281290628310078, 1458.110497838100173, 199.6352755006269888 ) ) ;
#73398=CARTESIAN_POINT ( 'NONE',  ( 8.539235273727440401, 1425.244712013389972, 194.2347455539940029 ) ) ;
#73400=EDGE_CURVE ( 'NONE', #56950, #63442, #58773, .T. ) ;
#73402=AXIS2_PLACEMENT_3D ( 'NONE', #18589, #19712, #9649 ) ;
#73403=CARTESIAN_POINT ( 'NONE',  ( 12.17073567488309926, 1499.730396444349708, 205.6506566649260321 ) ) ;
#73407=ADVANCED_FACE ( 'NONE', ( #15084 ), #16805, .T. ) ;
#73411=CARTESIAN_POINT ( 'NONE',  ( 1.125259334100000119, 1515.531689041389882, 205.0307428966389978 ) ) ;
#73413=CARTESIAN_POINT ( 'NONE',  ( -9.771923697420890065, 1448.872169750079820, 190.8346798121849872 ) ) ;
#73423=EDGE_LOOP ( 'NONE', ( #17430, #60674, #12027 ) ) ;
#73425=EDGE_CURVE ( 'NONE', #53764, #50471, #102950, .T. ) ;
#73426=CARTESIAN_POINT ( 'NONE',  ( 2.008229241910000074, 1477.194275679390103, 198.7982270564990017 ) ) ;
#73428=CARTESIAN_POINT ( 'NONE',  ( -10.99857149249999999, 1492.065342166190021, 207.0970266674490006 ) ) ;
#73430=CARTESIAN_POINT ( 'NONE',  ( 4.967684365510000255, 1469.890599266690060, 189.7939106698990201 ) ) ;
#73437=CARTESIAN_POINT ( 'NONE',  ( -12.10212147083699996, 1491.001746246500034, 207.1149663066109952 ) ) ;
#73438=CARTESIAN_POINT ( 'NONE',  ( -4.105525334182019925, 1508.551704408389924, 204.7297663225739939 ) ) ;
#73443=CARTESIAN_POINT ( 'NONE',  ( -0.03690140138640260470, 1502.066352419989926, 230.5451525067989849 ) ) ;
#73445=CARTESIAN_POINT ( 'NONE',  ( -9.642223397419670050, 1460.679120766980077, 208.4218084076549928 ) ) ;
#73446=CARTESIAN_POINT ( 'NONE',  ( 10.24713651180139884, 1471.272112719760116, 211.7185712946420040 ) ) ;
#73456=CARTESIAN_POINT ( 'NONE',  ( -18.27900023279999786, 1466.853294321590283, 217.8669514379789973 ) ) ;
#73460=CARTESIAN_POINT ( 'NONE',  ( 20.02429320899999965, 1475.403248319589693, 206.2289784283690040 ) ) ;
#73463=CARTESIAN_POINT ( 'NONE',  ( -16.36753375360000007, 1504.434416204990157, 208.8870069452450196 ) ) ;
#73467=CARTESIAN_POINT ( 'NONE',  ( 9578.491711904032854, -2339.246371527899555, -432.3565737843579768 ) ) ;
#73474=EDGE_LOOP ( 'NONE', ( #76009, #68102, #88771, #4604 ) ) ;
#73475=CARTESIAN_POINT ( 'NONE',  ( -0.7745270672630399922, 1486.078395409020004, 220.9964989435360110 ) ) ;
#73483=CARTESIAN_POINT ( 'NONE',  ( 10.33351940753939857, 1481.839770964269974, 211.5429078627209947 ) ) ;
#73488=ORIENTED_EDGE ( 'NONE', *, *, #1758, .T. ) ;
#73489=CARTESIAN_POINT ( 'NONE',  ( 11.27339694790000024, 1433.557990534789951, 225.8166789514989716 ) ) ;
#73491=VERTEX_POINT ( 'NONE', #20595 ) ;
#73497=CARTESIAN_POINT ( 'NONE',  ( 12.66527585539470024, 1500.313660553920045, 208.2538028397970038 ) ) ;
#73498=CARTESIAN_POINT ( 'NONE',  ( -19.39187281942849950, 1508.251301914079932, 209.6313561747230096 ) ) ;
#73503=CARTESIAN_POINT ( 'NONE',  ( -1.255931481480000000, 1464.641271298989977, 198.9598639639989983 ) ) ;
#73520=CARTESIAN_POINT ( 'NONE',  ( -6.988050048983349249, 1435.480056246220101, 215.8758039753799949 ) ) ;
#73531=CARTESIAN_POINT ( 'NONE',  ( -10.38518064779726657, 1480.556690206445182, 207.3434171914812225 ) ) ;
#73532=CARTESIAN_POINT ( 'NONE',  ( 3.401541474470889614, 1468.225229937070026, 218.5224292273400124 ) ) ;
#73543=CARTESIAN_POINT ( 'NONE',  ( -7.195143960150679696, 1440.674916713600169, 203.7359215401640142 ) ) ;
#73546=CARTESIAN_POINT ( 'NONE',  ( 7.524255332260000095, 1421.856213011689988, 195.6731416337989913 ) ) ;
#73547=CARTESIAN_POINT ( 'NONE',  ( -2.823233910641499644, 1474.899251128670130, 216.0777834340740071 ) ) ;
#73560=CARTESIAN_POINT ( 'NONE',  ( 0.5244545025614146816, 1463.744894996491666, 199.3254876305578307 ) ) ;
#73563=CARTESIAN_POINT ( 'NONE',  ( -7.228518429932707434, 1439.534556209132461, 204.1938366727016501 ) ) ;
#73567=CARTESIAN_POINT ( 'NONE',  ( -2.469737515570000319, 1507.227429580189892, 221.7265305201989918 ) ) ;
#73568=CARTESIAN_POINT ( 'NONE',  ( -4.325231544520000249, 1515.225845272990000, 210.2100514189989724 ) ) ;
#73582=CARTESIAN_POINT ( 'NONE',  ( 12.10692502261549919, 1491.460737533769816, 207.0028281992289863 ) ) ;
#73587=CARTESIAN_POINT ( 'NONE',  ( 12.77583168044349904, 1421.377537522909961, 206.0195167871399917 ) ) ;
#73592=CARTESIAN_POINT ( 'NONE',  ( -19.73708035071419786, 1467.795414648790029, 204.3773339574159991 ) ) ;
#73593=AXIS2_PLACEMENT_3D ( 'NONE', #39784, #48196, #98020 ) ;
#73599=CARTESIAN_POINT ( 'NONE',  ( 7.527441479340000186, 1427.147074679829984, 212.6188437181790221 ) ) ;
#73600=CARTESIAN_POINT ( 'NONE',  ( -17.84103545810000213, 1489.004099770289940, 195.1797354288989936 ) ) ;
#73602=CARTESIAN_POINT ( 'NONE',  ( -21.33855393657290023, 1418.051173837530087, 208.5953683876979881 ) ) ;
#73608=VERTEX_POINT ( 'NONE', #105560 ) ;
#73616=CARTESIAN_POINT ( 'NONE',  ( 1.668731198869999988, 1443.775019653990057, 200.3211300381289846 ) ) ;
#73637=CARTESIAN_POINT ( 'NONE',  ( -11.42155100230000109, 1501.800602108690100, 208.0855181463290080 ) ) ;
#73642=VERTEX_POINT ( 'NONE', #63042 ) ;
#73652=CARTESIAN_POINT ( 'NONE',  ( -14.25094185831662230, 1415.731847238539103, 214.3326356602875649 ) ) ;
#73660=CARTESIAN_POINT ( 'NONE',  ( 12.27064591350710110, 1492.413804220679822, 210.4788641801989684 ) ) ;
#73673=ADVANCED_FACE ( 'NONE', ( #97694 ), #20501, .T. ) ;
#73675=CARTESIAN_POINT ( 'NONE',  ( 4.987078442593329441, 1508.551704408389924, 206.6339108768089829 ) ) ;
#73676=CARTESIAN_POINT ( 'NONE',  ( -2.673720665360000304, 1500.461465227589997, 230.2728548803989952 ) ) ;
#73677=CARTESIAN_POINT ( 'NONE',  ( 12.07937513949999975, 1426.251990374380057, 203.1934598926790159 ) ) ;
#73680=LINE ( 'NONE', #73112, #81913 ) ;
#73681=CARTESIAN_POINT ( 'NONE',  ( 4.617353517619999792, 1460.098150474590057, 228.0971968620989969 ) ) ;
#73686=EDGE_LOOP ( 'NONE', ( #75977, #11680, #65814, #101820 ) ) ;
#73691=CARTESIAN_POINT ( 'NONE',  ( 10.85236227365940032, 1461.719670514279869, 210.7330291806389937 ) ) ;
#73692=CARTESIAN_POINT ( 'NONE',  ( 8.436619542363665403, 1424.469057821296929, 195.8194399936322725 ) ) ;
#73694=CARTESIAN_POINT ( 'NONE',  ( 2.942575405789999987, 1443.229435617889749, 217.5275331713689866 ) ) ;
#73705=CARTESIAN_POINT ( 'NONE',  ( -14.30687469689999958, 1508.551704411289847, 215.7932974708489837 ) ) ;
#73707=DIRECTION ( 'NONE',  ( 1.224646799147350002E-16, -1.836970198721029688E-16, -1.000000000000000000 ) ) ;
#73711=EDGE_CURVE ( 'NONE', #24288, #26097, #29117, .T. ) ;
#73712=CARTESIAN_POINT ( 'NONE',  ( -8.628345599877569327, 1437.012300105949862, 209.5206063237490071 ) ) ;
#73716=CARTESIAN_POINT ( 'NONE',  ( -9.642223397419670050, 1460.679120766980077, 208.4218084076549928 ) ) ;
#73717=CARTESIAN_POINT ( 'NONE',  ( -15.15772398740000071, 1439.441663529990137, 221.0618115286989962 ) ) ;
#73720=ORIENTED_EDGE ( 'NONE', *, *, #110273, .F. ) ;
#73725=CARTESIAN_POINT ( 'NONE',  ( -11.38916142969999967, 1500.505134835889976, 209.9622123134469973 ) ) ;
#73727=CARTESIAN_POINT ( 'NONE',  ( 1.423785136650000060, 1455.243703889889957, 218.4445183310089931 ) ) ;
#73729=CARTESIAN_POINT ( 'NONE',  ( 9.309724285312150016, 1436.355445090830017, 210.5148441957229863 ) ) ;
#73732=CARTESIAN_POINT ( 'NONE',  ( 8.778595366665010502, 1422.758389621050128, 213.4479264546969830 ) ) ;
#73735=CARTESIAN_POINT ( 'NONE',  ( 1.107569330185070200, 1515.100382602269974, 213.4503627880180261 ) ) ;
#73742=ORIENTED_EDGE ( 'NONE', *, *, #14410, .T. ) ;
#73744=CARTESIAN_POINT ( 'NONE',  ( 19.23094364312690274, 1497.625611886179968, 221.9534124282759819 ) ) ;
#73750=CARTESIAN_POINT ( 'NONE',  ( 4.327725855061919980, 1515.130588580249878, 209.8370891087949985 ) ) ;
#73752=CARTESIAN_POINT ( 'NONE',  ( 10.03054928460160156, 1469.026556028670029, 208.9478250291980146 ) ) ;
#73753=CARTESIAN_POINT ( 'NONE',  ( -4.665462402540000220, 1457.845415160889843, 217.6027515947390327 ) ) ;
#73758=ORIENTED_EDGE ( 'NONE', *, *, #245, .T. ) ;
#73761=CARTESIAN_POINT ( 'NONE',  ( -8.570364584155420573, 1448.478232341050216, 212.2952113106709930 ) ) ;
#73764=CARTESIAN_POINT ( 'NONE',  ( -17.64794458902535723, 1419.546587406255867, 207.1439701417919252 ) ) ;
#73774=CARTESIAN_POINT ( 'NONE',  ( -3.392503662839999823, 1483.205550810290106, 202.1035814847290055 ) ) ;
#73793=CARTESIAN_POINT ( 'NONE',  ( -10.17628962590000086, 1472.218688241290238, 207.3995869476289897 ) ) ;
#73799=DIRECTION ( 'NONE',  ( -0.06124624279912479347, -0.4472592145003609354, -0.8923049326253389424 ) ) ;
#73804=CARTESIAN_POINT ( 'NONE',  ( -4.240726796310859470, 1476.401387198489829, 199.6760741912259789 ) ) ;
#73809=ORIENTED_EDGE ( 'NONE', *, *, #101923, .T. ) ;
#73815=CARTESIAN_POINT ( 'NONE',  ( -2.279616087740000019, 1474.769975645390105, 219.1638168117989949 ) ) ;
#73825=DIRECTION ( 'NONE',  ( 0.1454373636825659899, -0.4507558898458529084, 0.8807196494993957403 ) ) ;
#73831=CARTESIAN_POINT ( 'NONE',  ( 11.43088729239800116, 1502.411350489410097, 211.2362053281570127 ) ) ;
#73838=CARTESIAN_POINT ( 'NONE',  ( -11.41402561306639996, 1500.969831351809944, 208.5831151434670119 ) ) ;
#73840=CARTESIAN_POINT ( 'NONE',  ( 0.7098482576299989244, 1456.796867040289953, 219.7430208676990162 ) ) ;
#73841=EDGE_LOOP ( 'NONE', ( #42685, #72397, #50699, #46240 ) ) ;
#73844=CARTESIAN_POINT ( 'NONE',  ( 3.545811734658929737, 1508.551704408389924, 204.3700499762609866 ) ) ;
#73847=CARTESIAN_POINT ( 'NONE',  ( 19.03958733774129897, 1453.804075884379927, 200.7927936193499932 ) ) ;
#73850=CARTESIAN_POINT ( 'NONE',  ( -2.936817763033160222, 1515.374151778960140, 204.8620682627120004 ) ) ;
#73858=CARTESIAN_POINT ( 'NONE',  ( 12.55979069370000012, 1458.679714032590027, 224.9161459441990019 ) ) ;
#73866=CARTESIAN_POINT ( 'NONE',  ( 12.68557844200520002, 1420.747169022329899, 201.7075646973950143 ) ) ;
#73868=CARTESIAN_POINT ( 'NONE',  ( -14.86383190760000161, 1420.231781918219895, 213.2204302019290196 ) ) ;
#73876=CARTESIAN_POINT ( 'NONE',  ( -8.894458315472089538, 1449.037666247089874, 211.3340079007809891 ) ) ;
#73881=CARTESIAN_POINT ( 'NONE',  ( 7.417280415950580519, 1425.156060753129850, 212.4179085937329887 ) ) ;
#73894=ORIENTED_EDGE ( 'NONE', *, *, #26859, .F. ) ;
#73905=FACE_OUTER_BOUND ( 'NONE', #17613, .T. ) ;
#73907=CARTESIAN_POINT ( 'NONE',  ( 2.487923051973920163, 1508.611354625609920, 213.7999901942370116 ) ) ;
#73913=CARTESIAN_POINT ( 'NONE',  ( 11.44787351428849931, 1480.383220438659919, 211.9499576844269768 ) ) ;
#73919=CARTESIAN_POINT ( 'NONE',  ( 8.062587302181759341, 1436.235894220949831, 206.1282943059349861 ) ) ;
#73921=CARTESIAN_POINT ( 'NONE',  ( 6.713174362274499707, 1504.508803738159941, 219.9706393884620184 ) ) ;
#73922=CARTESIAN_POINT ( 'NONE',  ( 12.10433974340000063, 1420.521815624170131, 199.8646142222890205 ) ) ;
#73923=CARTESIAN_POINT ( 'NONE',  ( 19.17520749770000066, 1455.940066015489947, 211.9422318690290012 ) ) ;
#73925=CARTESIAN_POINT ( 'NONE',  ( 10.55201363404730230, 1479.182026721460034, 205.9886858934539760 ) ) ;
#73929=CARTESIAN_POINT ( 'NONE',  ( 10.93408409447810037, 1423.050204788569999, 206.8916427814799874 ) ) ;
#73937=CARTESIAN_POINT ( 'NONE',  ( 10.82744550939999861, 1427.328225570349787, 209.3701112376719777 ) ) ;
#73939=CARTESIAN_POINT ( 'NONE',  ( 11.13844977941739778, 1424.861034171799929, 203.0515873249630090 ) ) ;
#73941=CARTESIAN_POINT ( 'NONE',  ( 2.191891361270000171, 1430.523720098889953, 217.5805868065489790 ) ) ;
#73943=CARTESIAN_POINT ( 'NONE',  ( -3.657993755839999750, 1474.872004365689918, 218.7367895275489786 ) ) ;
#73946=CARTESIAN_POINT ( 'NONE',  ( 8.562340737000068813, 1433.778957528687442, 204.3790743423090248 ) ) ;
#73947=FACE_OUTER_BOUND ( 'NONE', #23747, .T. ) ;
#73948=CARTESIAN_POINT ( 'NONE',  ( 3.974701152529080073, 1457.344300949599983, 199.5572480904559995 ) ) ;
#73956=CARTESIAN_POINT ( 'NONE',  ( -20.30852359509999872, 1486.101457756589753, 213.0654537167889657 ) ) ;
#73957=B_SPLINE_CURVE_WITH_KNOTS ( 'NONE', 3,
 ( #70762, #61799, #52286, #53385 ),
 .UNSPECIFIED., .F., .F.,
 ( 4, 4 ),
 ( -19.44060205079999903, -0.6888856060759991351 ),
 .UNSPECIFIED. ) ;
#73958=CARTESIAN_POINT ( 'NONE',  ( 4.781276783620000081, 1452.020048942890071, 190.5513815401990030 ) ) ;
#73960=CARTESIAN_POINT ( 'NONE',  ( 1.454938208119999965, 1515.064792882589927, 204.7923971856590128 ) ) ;
#73972=CARTESIAN_POINT ( 'NONE',  ( -1.835774698489999857, 1484.769563356690014, 198.4308759197990071 ) ) ;
#73975=CARTESIAN_POINT ( 'NONE',  ( -11.40503445839999941, 1490.739836597089834, 209.6941760096060250 ) ) ;
#73992=CARTESIAN_POINT ( 'NONE',  ( 10.01012151112310100, 1469.368595336919952, 209.9818033434729898 ) ) ;
#74000=CARTESIAN_POINT ( 'NONE',  ( -19.67777960560400174, 1467.001721752909816, 204.2858066586710208 ) ) ;
#74008=CARTESIAN_POINT ( 'NONE',  ( -17.55491153119999836, 1504.812299793789862, 208.9605407232590153 ) ) ;
#74015=ORIENTED_EDGE ( 'NONE', *, *, #74452, .F. ) ;
#74021=CARTESIAN_POINT ( 'NONE',  ( 12.53292608669999986, 1500.050071955789917, 207.1420395195890194 ) ) ;
#74029=EDGE_CURVE ( 'NONE', #28705, #96418, #2715, .T. ) ;
#74030=CARTESIAN_POINT ( 'NONE',  ( 12.45931607057640100, 1501.250537210039965, 211.6676667882360050 ) ) ;
#74031=EDGE_CURVE ( 'NONE', #54902, #36343, #60365, .T. ) ;
#74035=CARTESIAN_POINT ( 'NONE',  ( -4.705736654490000781, 1479.984769897790102, 230.9466533013989817 ) ) ;
#74044=CARTESIAN_POINT ( 'NONE',  ( -18.42382187532859916, 1508.551704391109979, 210.1329842148610112 ) ) ;
#74048=CARTESIAN_POINT ( 'NONE',  ( -8.986359071028783063, 1482.816979524136059, 227.9996318485843005 ) ) ;
#74056=ORIENTED_EDGE ( 'NONE', *, *, #110696, .T. ) ;
#74062=CARTESIAN_POINT ( 'NONE',  ( 8.060623735539611090, 1428.631035214050144, 214.1143366338490068 ) ) ;
#74085=CARTESIAN_POINT ( 'NONE',  ( -12.16530128034490055, 1501.737063442450108, 211.5189884477989892 ) ) ;
#74086=EDGE_LOOP ( 'NONE', ( #57187, #9991, #107336, #62353 ) ) ;
#74090=CARTESIAN_POINT ( 'NONE',  ( -15.80167951410000171, 1415.804990609770130, 209.5032351745619792 ) ) ;
#74093=CARTESIAN_POINT ( 'NONE',  ( 7.758184319229999737, 1421.576654411539948, 195.8091089427989857 ) ) ;
#74106=EDGE_CURVE ( 'NONE', #24288, #100109, #89546, .T. ) ;
#74107=CARTESIAN_POINT ( 'NONE',  ( 1.989421934769288303, 1464.165607546044384, 199.5054174974058299 ) ) ;
#74109=DIRECTION ( 'NONE',  ( -0.2907001422290489967, -0.4501984363202189976, 0.8442835988237840095 ) ) ;
#74114=CARTESIAN_POINT ( 'NONE',  ( -10.92081006369999940, 1499.922668861390093, 212.8248374489089940 ) ) ;
#74128=B_SPLINE_SURFACE_WITH_KNOTS ( 'NONE', 5, 5, ( 
 ( #108927, #75877, #32217, #83175, #24350, #67496 ),
 ( #40065, #5919, #58536, #31656, #92661, #6465 ),
 ( #15936, #109483, #40614, #74785, #42271, #92120 ),
 ( #50139, #24884, #84266, #41716, #110025, #33301 ),
 ( #101600, #17024, #110575, #33860, #102160, #51222 ),
 ( #10318, #85355, #68593, #94881, #78077, #60190 ),
 ( #840, #17588, #25992, #69148, #1380, #94309 ),
 ( #28231, #102698, #35522, #61320, #51787, #43932 ),
 ( #53456, #103253, #76988, #36635, #70831, #27682 ) ),
 .UNSPECIFIED., .F., .F., .F.,
 ( 6, 3, 6 ),
 ( 6, 6 ),
 ( 0.000000000000000000, 1.406546626929999988, 2.813093253849999975 ),
 ( 0.000000000000000000, 2.000000000000000000 ),
 .UNSPECIFIED. ) ;
#74129=CARTESIAN_POINT ( 'NONE',  ( 12.30756928984159870, 1491.905514282249896, 208.5176378714709813 ) ) ;
#74132=CARTESIAN_POINT ( 'NONE',  ( 4.900006679340000559, 1499.255191946190052, 229.7873568473989963 ) ) ;
#74133=CARTESIAN_POINT ( 'NONE',  ( 12.86007276073260108, 1421.274266495399843, 205.3533571373839948 ) ) ;
#74137=B_SPLINE_SURFACE_WITH_KNOTS ( 'NONE', 5, 1, ( 
 ( #106195, #72604 ),
 ( #29477, #105663 ),
 ( #64215, #63672 ),
 ( #13212, #47402 ),
 ( #4825, #38971 ),
 ( #73150, #107293 ) ),
 .UNSPECIFIED., .F., .F., .F.,
 ( 6, 6 ),
 ( 2, 2 ),
 ( 0.000000000000000000, 17.81543997039999994 ),
 ( 0.000000000000000000, 14.00000000000000000 ),
 .UNSPECIFIED. ) ;
#74139=CARTESIAN_POINT ( 'NONE',  ( -13.59453042928210031, 1507.871302099940067, 209.3931762073830214 ) ) ;
#74140=CARTESIAN_POINT ( 'NONE',  ( 20.81805263692159969, 1457.016373647149976, 206.8941932428749908 ) ) ;
#74146=CARTESIAN_POINT ( 'NONE',  ( -4.686874221129999185, 1454.311615498590072, 200.8248795411589924 ) ) ;
#74148=CARTESIAN_POINT ( 'NONE',  ( 7.647272590590000974, 1426.541769689450120, 212.1576498646190032 ) ) ;
#74157=ORIENTED_EDGE ( 'NONE', *, *, #41416, .T. ) ;
#74162=EDGE_CURVE ( 'NONE', #345, #30629, #39914, .T. ) ;
#74165=CARTESIAN_POINT ( 'NONE',  ( 2.989015302459999912, 1446.190165938789960, 199.4457794469589942 ) ) ;
#74170=CARTESIAN_POINT ( 'NONE',  ( -3.240770211191819961, 1463.391176810840079, 199.8726916786840206 ) ) ;
#74180=ORIENTED_EDGE ( 'NONE', *, *, #66456, .T. ) ;
#74188=B_SPLINE_CURVE_WITH_KNOTS ( 'NONE', 5,
 ( #34430, #42279, #8659, #51795, #33868, #26002 ),
 .UNSPECIFIED., .F., .F.,
 ( 6, 6 ),
 ( -1.999999981381699987, 0.000000000000000000 ),
 .UNSPECIFIED. ) ;
#74190=CARTESIAN_POINT ( 'NONE',  ( -11.44093224520000085, 1503.454049389589727, 207.5539012139990120 ) ) ;
#74194=VERTEX_POINT ( 'NONE', #39426 ) ;
#74196=CARTESIAN_POINT ( 'NONE',  ( -9.126765308707120994, 1450.806276981840028, 207.6833491750169856 ) ) ;
#74215=CARTESIAN_POINT ( 'NONE',  ( 2.395822483399999925, 1441.661856669790041, 218.7568551047190226 ) ) ;
#74227=CARTESIAN_POINT ( 'NONE',  ( -2.079673249558308346, 1495.029477387638508, 220.0949141771806126 ) ) ;
#74229=CARTESIAN_POINT ( 'NONE',  ( 12.74373164180000018, 1426.782509952399778, 204.7461156749990039 ) ) ;
#74243=CARTESIAN_POINT ( 'NONE',  ( 9.367332565670180244, 1425.287430459912912, 195.5756684483055494 ) ) ;
#74244=CARTESIAN_POINT ( 'NONE',  ( -1.009278519650000039, 1444.031905486989899, 218.1361756941589931 ) ) ;
#74255=LINE ( 'NONE', #108386, #15705 ) ;
#74257=CARTESIAN_POINT ( 'NONE',  ( 11.26824400833899986, 1470.496689712369971, 207.5795241769199890 ) ) ;
#74262=CARTESIAN_POINT ( 'NONE',  ( -9.978843980182551476, 1439.175531641559928, 209.1458737907410068 ) ) ;
#74263=CARTESIAN_POINT ( 'NONE',  ( 2.947604512712040048, 1495.328382756780002, 220.7041825259470045 ) ) ;
#74265=CARTESIAN_POINT ( 'NONE',  ( -14.43789412238549907, 1415.677402204810051, 205.2933806555749925 ) ) ;
#74268=CARTESIAN_POINT ( 'NONE',  ( -18.17365796220000007, 1441.208305948289762, 213.5442559039389891 ) ) ;
#74271=EDGE_CURVE ( 'NONE', #328, #26746, #109252, .T. ) ;
#74274=ORIENTED_EDGE ( 'NONE', *, *, #53075, .T. ) ;
#74276=CARTESIAN_POINT ( 'NONE',  ( -12.69354645500000167, 1502.230858064689983, 210.5965602401589933 ) ) ;
#74278=CARTESIAN_POINT ( 'NONE',  ( 5.456719627610000067, 1455.595244131089885, 218.2350948550090095 ) ) ;
#74283=CARTESIAN_POINT ( 'NONE',  ( 9.285715353111019255, 1464.591735933340033, 212.3819174308400193 ) ) ;
#74286=CARTESIAN_POINT ( 'NONE',  ( -3.707546501630690106, 1454.065007432690209, 199.3225983413989866 ) ) ;
#74295=CARTESIAN_POINT ( 'NONE',  ( 19.36069530197559985, 1498.614194606489946, 221.8424376627909851 ) ) ;
#74300=CARTESIAN_POINT ( 'NONE',  ( 4.327853128026699636, 1515.125728221819827, 209.9038229511910174 ) ) ;
#74302=CARTESIAN_POINT ( 'NONE',  ( -7.279378368329999738, 1479.856447813089972, 209.7098936948849826 ) ) ;
#74304=CARTESIAN_POINT ( 'NONE',  ( 18.25317160297629826, 1431.535582262299840, 208.0285350045080008 ) ) ;
#74305=CARTESIAN_POINT ( 'NONE',  ( -3.620275138579999830, 1456.955153447490147, 217.9164953791890014 ) ) ;
#74310=CARTESIAN_POINT ( 'NONE',  ( -4.327152622306649654, 1515.152479455989806, 209.4468724884619917 ) ) ;
#74318=CARTESIAN_POINT ( 'NONE',  ( -17.64167022720579681, 1419.649359460465575, 207.0478719141029273 ) ) ;
#74322=ORIENTED_EDGE ( 'NONE', *, *, #78179, .T. ) ;
#74337=CARTESIAN_POINT ( 'NONE',  ( 10.81529792403469870, 1460.553129422620032, 207.5316501181210072 ) ) ;
#74344=CARTESIAN_POINT ( 'NONE',  ( 5.039568361674230168, 1440.423861375179968, 217.2666807852390036 ) ) ;
#74357=CARTESIAN_POINT ( 'NONE',  ( -17.48895720149999988, 1417.651609471990014, 206.3668144019989938 ) ) ;
#74360=CARTESIAN_POINT ( 'NONE',  ( 7.340611670529999522, 1487.529895563990067, 201.1154889873190257 ) ) ;
#74367=CARTESIAN_POINT ( 'NONE',  ( -17.63541786559999736, 1417.743836435179901, 206.3821828179090119 ) ) ;
#74370=CARTESIAN_POINT ( 'NONE',  ( -14.35866385045889970, 1508.448434989210000, 216.0828215529409988 ) ) ;
#74372=CARTESIAN_POINT ( 'NONE',  ( -3.410173980340000188, 1476.067642529390241, 219.2827969570990092 ) ) ;
#74375=CARTESIAN_POINT ( 'NONE',  ( -3.924179544107323281, 1508.147948383610583, 220.6842618796573845 ) ) ;
#74377=CARTESIAN_POINT ( 'NONE',  ( -1.465977870436109942, 1455.136833094290068, 198.7136623775919873 ) ) ;
#74379=B_SPLINE_SURFACE_WITH_KNOTS ( 'NONE', 5, 1, ( 
 ( #50541, #24202 ),
 ( #694, #41017 ),
 ( #60052, #34272 ),
 ( #100905, #52203 ),
 ( #41585, #7965 ),
 ( #32628, #60608 ) ),
 .UNSPECIFIED., .F., .F., .F.,
 ( 6, 6 ),
 ( 2, 2 ),
 ( 0.000000000000000000, 16.62916768389999689 ),
 ( 0.000000000000000000, 14.00000000000000000 ),
 .UNSPECIFIED. ) ;
#74382=CARTESIAN_POINT ( 'NONE',  ( -4.455702694979999379, 1476.149614445790121, 218.6586916280889739 ) ) ;
#74385=ORIENTED_EDGE ( 'NONE', *, *, #19277, .F. ) ;
#74386=CARTESIAN_POINT ( 'NONE',  ( 6.680902021104210498, 1440.813589410888653, 214.8934479320009245 ) ) ;
#74388=CARTESIAN_POINT ( 'NONE',  ( -1.927340254199999769, 1443.937843298589996, 199.6634601012389965 ) ) ;
#74389=CARTESIAN_POINT ( 'NONE',  ( 7.871286969770000752, 1423.706537194029806, 195.8927146150989813 ) ) ;
#74390=CARTESIAN_POINT ( 'NONE',  ( -0.8775825618903739800, 1380.371560387289946, 209.6012715003031985 ) ) ;
#74392=CARTESIAN_POINT ( 'NONE',  ( 0.7436733002139179760, 1508.551704408389924, 219.9150180538129860 ) ) ;
#74395=CARTESIAN_POINT ( 'NONE',  ( -4.987078422688609791, 1508.551704408389924, 206.6339250122549913 ) ) ;
#74398=CARTESIAN_POINT ( 'NONE',  ( 10.65708661477679975, 1491.469129873149996, 211.9150438862110093 ) ) ;
#74399=CARTESIAN_POINT ( 'NONE',  ( 0.1234260537299990135, 1456.953841043490229, 219.7696534638990045 ) ) ;
#74403=CARTESIAN_POINT ( 'NONE',  ( 4.733838391792250633, 1508.551704408389924, 205.5349709131090208 ) ) ;
#74404=VERTEX_POINT ( 'NONE', #66039 ) ;
#74408=DIRECTION ( 'NONE',  ( -0.2673318221160059793, 0.3729039878434610156, -0.8885247957905170191 ) ) ;
#74409=CARTESIAN_POINT ( 'NONE',  ( -3.983717799494409295, 1515.551844914359890, 206.7919068544310051 ) ) ;
#74412=CARTESIAN_POINT ( 'NONE',  ( -5.976488786809999176, 1464.287555164190053, 199.8460616603990161 ) ) ;
#74415=CARTESIAN_POINT ( 'NONE',  ( -14.58361734293779932, 1508.551704408389924, 215.2898793084600015 ) ) ;
#74419=CARTESIAN_POINT ( 'NONE',  ( 7.823841191072109069, 1434.286212867250015, 204.6742520563170160 ) ) ;
#74422=ORIENTED_EDGE ( 'NONE', *, *, #56997, .F. ) ;
#74430=CARTESIAN_POINT ( 'NONE',  ( -14.99991866480000091, 1420.433500232019924, 212.5351666037989844 ) ) ;
#74441=CARTESIAN_POINT ( 'NONE',  ( 6.864181478733449637, 1424.874072653679832, 213.4309032859040087 ) ) ;
#74443=ORIENTED_EDGE ( 'NONE', *, *, #44566, .T. ) ;
#74452=EDGE_CURVE ( 'NONE', #94689, #73642, #91336, .T. ) ;
#74464=ORIENTED_EDGE ( 'NONE', *, *, #881, .T. ) ;
#74468=CARTESIAN_POINT ( 'NONE',  ( 4.492641946539720266, 1508.880976916049804, 212.2392405230349937 ) ) ;
#74470=AXIS2_PLACEMENT_3D ( 'NONE', #99566, #30722, #13349 ) ;
#74473=CARTESIAN_POINT ( 'NONE',  ( -6.730034279650000784, 1426.619567491610042, 203.0656631102989991 ) ) ;
#74481=CARTESIAN_POINT ( 'NONE',  ( -437.6900670641260263, 1424.998713256100018, 209.1045946275809797 ) ) ;
#74485=CARTESIAN_POINT ( 'NONE',  ( 9.564368764730000194, 1420.652513758999930, 197.0358326467990082 ) ) ;
#74487=CARTESIAN_POINT ( 'NONE',  ( -9.442246275039069658, 1493.175626386839895, 201.2440496806180192 ) ) ;
#74488=CARTESIAN_POINT ( 'NONE',  ( -4.748472660380000043, 1496.422918367389912, 198.9435340602989868 ) ) ;
#74491=CARTESIAN_POINT ( 'NONE',  ( 6.646318662569999702, 1378.413060387289988, 209.1218459647943746 ) ) ;
#74492=CARTESIAN_POINT ( 'NONE',  ( 10.77287936046479899, 1425.076563501110058, 206.5335355432609958 ) ) ;
#74500=CARTESIAN_POINT ( 'NONE',  ( 10.63130018098530094, 1427.874628198720075, 210.9979093251330085 ) ) ;
#74501=CARTESIAN_POINT ( 'NONE',  ( 11.26113244141030023, 1425.135562406779854, 203.0046430561289981 ) ) ;
#74503=CARTESIAN_POINT ( 'NONE',  ( 1.057929922660000077, 1429.578271572490166, 217.3710875290090030 ) ) ;
#74505=CARTESIAN_POINT ( 'NONE',  ( -17.00797328670000397, 1417.537217351680056, 207.7155449971589860 ) ) ;
#74509=CARTESIAN_POINT ( 'NONE',  ( -1.693092047772239983, 1443.235800395060096, 218.9922115469449864 ) ) ;
#74514=CARTESIAN_POINT ( 'NONE',  ( 5.587699803720799885, 1473.877678908759890, 219.0867832512670077 ) ) ;
#74516=CARTESIAN_POINT ( 'NONE',  ( -20.69303424980000372, 1486.764600954290017, 209.1218459616989946 ) ) ;
#74517=CARTESIAN_POINT ( 'NONE',  ( -2.497138374290000407, 1474.686822087490100, 216.2214433156790108 ) ) ;
#74521=CARTESIAN_POINT ( 'NONE',  ( 11.69992642896390045, 1435.514533225360083, 225.6365413922099776 ) ) ;
#74536=CARTESIAN_POINT ( 'NONE',  ( 9.146237114798470458, 1449.998848199699978, 208.1168068718100130 ) ) ;
#74542=CARTESIAN_POINT ( 'NONE',  ( 1.338019653377509943, 1431.361302561429966, 218.5179672105229827 ) ) ;
#74547=CARTESIAN_POINT ( 'NONE',  ( 4.061051490899999727, 1501.418159739390148, 230.0899566632990059 ) ) ;
#74549=CARTESIAN_POINT ( 'NONE',  ( 4.873735476160000246, 1472.089320948289924, 218.0431589096889695 ) ) ;
#74550=CARTESIAN_POINT ( 'NONE',  ( 11.39904368536729962, 1471.112668423910009, 209.6179614837379859 ) ) ;
#74553=CARTESIAN_POINT ( 'NONE',  ( -11.05399937894872409, 1492.687025461389339, 208.1826818617392121 ) ) ;
#74559=CARTESIAN_POINT ( 'NONE',  ( 7.184742850290000149, 1480.879511957389923, 207.6765937235290096 ) ) ;
#74565=ORIENTED_EDGE ( 'NONE', *, *, #47494, .F. ) ;
#74568=ORIENTED_EDGE ( 'NONE', *, *, #107818, .F. ) ;
#74574=B_SPLINE_CURVE_WITH_KNOTS ( 'NONE', 5,
 ( #59558, #84186, #16407, #93672, #41646, #50058 ),
 .UNSPECIFIED., .F., .F.,
 ( 6, 6 ),
 ( 0.000000000000000000, 1.000000000000000000 ),
 .UNSPECIFIED. ) ;
#74580=DIRECTION ( 'NONE',  ( 0.6480245870892075155, -1.644245901462725924E-32, -0.7616194158028418704 ) ) ;
#74583=AXIS2_PLACEMENT_3D ( 'NONE', #68174, #91134, #25562 ) ;
#74586=ORIENTED_EDGE ( 'NONE', *, *, #87815, .F. ) ;
#74587=CARTESIAN_POINT ( 'NONE',  ( 20.33643750519999926, 1475.138452888789971, 218.0161091832190152 ) ) ;
#74593=CARTESIAN_POINT ( 'NONE',  ( 12.64235333510859860, 1500.251838740290168, 207.9986088160900124 ) ) ;
#74596=CARTESIAN_POINT ( 'NONE',  ( 2.330134126090002145, 1515.193466806515744, 204.7957666309817455 ) ) ;
#74601=CARTESIAN_POINT ( 'NONE',  ( -5.510910596163090542E-16, 1508.551704408389924, 213.6218459616989946 ) ) ;
#74615=CARTESIAN_POINT ( 'NONE',  ( -9.276727106389110133, 1461.679952532089828, 206.2486811414470083 ) ) ;
#74621=EDGE_CURVE ( 'NONE', #84259, #79128, #36018, .T. ) ;
#74636=CARTESIAN_POINT ( 'NONE',  ( 3.376777021050000105, 1508.158926475389762, 220.2301072607990022 ) ) ;
#74639=CARTESIAN_POINT ( 'NONE',  ( -4.792927608962380681, 1442.435446138249972, 201.1994192484410178 ) ) ;
#74641=CARTESIAN_POINT ( 'NONE',  ( -7.326027882650599565, 1426.061615434360192, 203.3611598758510013 ) ) ;
#74647=CARTESIAN_POINT ( 'NONE',  ( 18.87853829029999986, 1458.344553362990155, 213.8102309971890236 ) ) ;
#74652=CARTESIAN_POINT ( 'NONE',  ( 10.95672663321720108, 1490.269269208220067, 209.3699634639930025 ) ) ;
#74655=ADVANCED_FACE ( 'NONE', ( #102361 ), #3582, .F. ) ;
#74659=CARTESIAN_POINT ( 'NONE',  ( -3.677613769069999778E-16, 1378.399971913189802, 209.1218459616989946 ) ) ;
#74666=CARTESIAN_POINT ( 'NONE',  ( -4.324478665330000027, 1515.254593745989951, 209.8453557593589949 ) ) ;
#74678=CARTESIAN_POINT ( 'NONE',  ( -21.48851227519999796, 1507.175870272490101, 211.5129893581290048 ) ) ;
#74688=CARTESIAN_POINT ( 'NONE',  ( -13.59199629040490009, 1508.179429147699921, 209.5634456311599934 ) ) ;
#74693=CARTESIAN_POINT ( 'NONE',  ( 9.905242068095489572, 1468.560492227489931, 207.6656469818879884 ) ) ;
#74697=CARTESIAN_POINT ( 'NONE',  ( -6.681506626574450713, 1488.898881121549948, 189.3483665020969795 ) ) ;
#74699=CYLINDRICAL_SURFACE ( 'NONE', #102965, 7.799999999999999822 ) ;
#74701=CARTESIAN_POINT ( 'NONE',  ( -20.41709936247310253, 1418.495400755769879, 207.2248099484089892 ) ) ;
#74706=VERTEX_POINT ( 'NONE', #72121 ) ;
#74717=CARTESIAN_POINT ( 'NONE',  ( -4.087663179609560160, 1462.748586608149935, 200.2519740037880069 ) ) ;
#74718=CARTESIAN_POINT ( 'NONE',  ( -17.39983170771839838, 1417.829866268649994, 207.0843391556029758 ) ) ;
#74733=EDGE_LOOP ( 'NONE', ( #18660, #34749, #44810, #42059 ) ) ;
#74734=CARTESIAN_POINT ( 'NONE',  ( -11.44024719100000098, 1501.432053922590057, 208.7106206354860092 ) ) ;
#74743=ORIENTED_EDGE ( 'NONE', *, *, #101364, .T. ) ;
#74748=CARTESIAN_POINT ( 'NONE',  ( 20.95983796500000196, 1494.619252927089747, 207.1496602654190156 ) ) ;
#74755=CARTESIAN_POINT ( 'NONE',  ( 12.32716646574370145, 1492.190914138330072, 209.5898718627249764 ) ) ;
#74759=CARTESIAN_POINT ( 'NONE',  ( 9.545106316202870644, 1434.678111609370035, 206.9724244943959945 ) ) ;
#74769=CARTESIAN_POINT ( 'NONE',  ( 5.161016356839920327, 1485.814728700380101, 218.5690746218629954 ) ) ;
#74770=CARTESIAN_POINT ( 'NONE',  ( 12.01083267770000162, 1421.737728622410032, 206.5830778804790100 ) ) ;
#74783=CARTESIAN_POINT ( 'NONE',  ( 10.94775415561070098, 1461.310702779670009, 209.6708789985609940 ) ) ;
#74785=CARTESIAN_POINT ( 'NONE',  ( 4.297841960619999568, 1466.500008501689990, 218.4916883454490062 ) ) ;
#74790=CARTESIAN_POINT ( 'NONE',  ( 10.68615365387295846, 1489.405825820419523, 206.7782173583013616 ) ) ;
#74795=ORIENTED_EDGE ( 'NONE', *, *, #46404, .F. ) ;
#74801=CARTESIAN_POINT ( 'NONE',  ( 0.000000000000000000, 1414.421228241719973, 209.1218459616989946 ) ) ;
#74804=CARTESIAN_POINT ( 'NONE',  ( -9.405025281284439487, 1438.375388356170106, 210.4453402788009839 ) ) ;
#74806=EDGE_CURVE ( 'NONE', #94930, #56950, #101415, .T. ) ;
#74808=CARTESIAN_POINT ( 'NONE',  ( -14.91790798717360111, 1415.677402202029953, 207.0650159394080276 ) ) ;
#74809=CARTESIAN_POINT ( 'NONE',  ( -9.650684282758110299, 1460.400330742749929, 209.4245232134740036 ) ) ;
#74819=CARTESIAN_POINT ( 'NONE',  ( 3.592245589920000093, 1454.165506685890023, 217.7999889770889865 ) ) ;
#74821=CARTESIAN_POINT ( 'NONE',  ( -7.173910393199999902, 1445.489765703290232, 216.0073357348389891 ) ) ;
#74822=EDGE_CURVE ( 'NONE', #91400, #97154, #108997, .T. ) ;
#74836=ORIENTED_EDGE ( 'NONE', *, *, #44618, .T. ) ;
#74837=ORIENTED_EDGE ( 'NONE', *, *, #57715, .T. ) ;
#74840=CARTESIAN_POINT ( 'NONE',  ( -21.43898449730000166, 1507.201558673590171, 216.1670088357489874 ) ) ;
#74845=CARTESIAN_POINT ( 'NONE',  ( -9.878129727571689500, 1422.666951092116960, 210.6716409553268079 ) ) ;
#74849=CARTESIAN_POINT ( 'NONE',  ( -3.300861552920000275, 1457.646899589489976, 218.4769539783190169 ) ) ;
#74852=ORIENTED_EDGE ( 'NONE', *, *, #21709, .T. ) ;
#74853=CARTESIAN_POINT ( 'NONE',  ( -4.328003007221890464, 1515.120004566319949, 209.9804044844569830 ) ) ;
#74860=VECTOR ( 'NONE', #33901, 1000.000000000000227 ) ;
#74864=DIRECTION ( 'NONE',  ( 9.156846217086110244E-47, -1.000000000000000000, 1.836970198721029688E-16 ) ) ;
#74865=EDGE_LOOP ( 'NONE', ( #105976, #74464, #59317, #77335 ) ) ;
#74871=CARTESIAN_POINT ( 'NONE',  ( 5.161277996873639751, 1424.205379132380131, 193.2953224460849810 ) ) ;
#74878=CARTESIAN_POINT ( 'NONE',  ( 1.581629459946789940, 1425.904611509570032, 191.1542090707819739 ) ) ;
#74886=CARTESIAN_POINT ( 'NONE',  ( 8.580955436158870242, 1438.351440300460126, 210.6486608506509981 ) ) ;
#74891=CARTESIAN_POINT ( 'NONE',  ( -8.588688654723730664, 1437.818490182359938, 207.9409985343149856 ) ) ;
#74893=ORIENTED_EDGE ( 'NONE', *, *, #52190, .F. ) ;
#74895=EDGE_CURVE ( 'NONE', #53103, #14695, #62832, .T. ) ;
#74897=B_SPLINE_SURFACE_WITH_KNOTS ( 'NONE', 5, 5, ( 
 ( #50917, #108608, #101838, #25133, #100738, #85048 ),
 ( #24022, #103506, #26808, #53136, #68840, #52582 ),
 ( #71058, #85593, #95121, #1082, #45292, #52025 ),
 ( #86716, #17269, #10008, #60433, #60995, #86165 ),
 ( #78890, #2196, #96225, #95672, #104065, #36865 ),
 ( #9457, #2744, #59878, #18385, #70505, #44179 ) ),
 .UNSPECIFIED., .F., .F., .F.,
 ( 6, 6 ),
 ( 6, 6 ),
 ( 7.548656686150499340, 12.57640183258060063 ),
 ( 0.000000000000000000, 0.5000176499934450014 ),
 .UNSPECIFIED. ) ;
#74903=CARTESIAN_POINT ( 'NONE',  ( 6.910350421100000418, 1487.761360645689820, 200.5560116829490198 ) ) ;
#74904=CARTESIAN_POINT ( 'NONE',  ( -3.344817776469899862, 1476.714814503689922, 199.3081550772679975 ) ) ;
#74906=CARTESIAN_POINT ( 'NONE',  ( -3.805396659119999914, 1495.647976226690162, 219.6495707272989932 ) ) ;
#74911=DIRECTION ( 'NONE',  ( -1.000000000000000000, 0.000000000000000000, 0.000000000000000000 ) ) ;
#74912=CARTESIAN_POINT ( 'NONE',  ( -16.87197715709999812, 1420.411836349220039, 203.4718720851689966 ) ) ;
#74916=CARTESIAN_POINT ( 'NONE',  ( -1.402942795860000036, 1473.972991866589837, 219.3058795016989961 ) ) ;
#74918=CARTESIAN_POINT ( 'NONE',  ( 1.914156658600000060, 1431.087920121590059, 199.8421650995689731 ) ) ;
#74919=CARTESIAN_POINT ( 'NONE',  ( -6.400436228969967445, 1508.335654507707204, 219.9811977713085582 ) ) ;
#74921=CARTESIAN_POINT ( 'NONE',  ( -1.966553775129000314, 1454.917737290639934, 198.8051624357930223 ) ) ;
#74922=EDGE_CURVE ( 'NONE', #96418, #63858, #2, .T. ) ;
#74925=CARTESIAN_POINT ( 'NONE',  ( -10.93154302307010006, 1470.132843826959970, 212.2379041850950046 ) ) ;
#74927=LINE ( 'NONE', #22820, #36730 ) ;
#74931=CARTESIAN_POINT ( 'NONE',  ( 5.262016255162093259, 1441.844739931066215, 216.2609436936466238 ) ) ;
#74934=CARTESIAN_POINT ( 'NONE',  ( -1.435439190950000166, 1443.368777369690179, 200.1970386830489872 ) ) ;
#74938=B_SPLINE_CURVE_WITH_KNOTS ( 'NONE', 3,
 ( #32040, #82455, #38782, #5752, #72958, #39894, #74062, #64575, #48871, #6288, #55070, #100875, #60019, #9039, #32599, #76250, #662, #66776, #91943, #40987, #33133, #93038, #101982, #93579, #51058 ),
 .UNSPECIFIED., .F., .F.,
 ( 4, 3, 3, 3, 3, 3, 3, 3, 4 ),
 ( -9.314730572460000246, -9.152340534729230370, -7.863899930683609263, -6.569977427668559855, -5.272424565628810456, -3.924989230018409714, -2.618936221757099503, -1.310405461081899148, 0.000000000000000000 ),
 .UNSPECIFIED. ) ;
#74940=CARTESIAN_POINT ( 'NONE',  ( -0.2978291352960920069, 1508.551704408389924, 220.0371209971259816 ) ) ;
#74945=CARTESIAN_POINT ( 'NONE',  ( -11.91268647012529946, 1502.145580229700045, 208.8923034686130222 ) ) ;
#74946=CARTESIAN_POINT ( 'NONE',  ( 10.90310790672270080, 1491.867556085790056, 211.5980998715699855 ) ) ;
#74947=CARTESIAN_POINT ( 'NONE',  ( -2.705951369970000187, 1457.026427619289962, 218.3778972485089866 ) ) ;
#74951=CARTESIAN_POINT ( 'NONE',  ( -0.7593982673170009967, 1430.316802068590050, 217.4503154216889982 ) ) ;
#74962=CARTESIAN_POINT ( 'NONE',  ( -10.19854404760319966, 1508.551704408389924, 218.1794582448719950 ) ) ;
#74965=CARTESIAN_POINT ( 'NONE',  ( 18.87853829029999986, 1458.344553362990155, 213.8102309971890236 ) ) ;
#74967=CARTESIAN_POINT ( 'NONE',  ( 3.974452695383380085, 1433.901817095809974, 201.5205318130460341 ) ) ;
#74978=CARTESIAN_POINT ( 'NONE',  ( 0.3106507903294934980, 1515.598599846736306, 213.1604233196099756 ) ) ;
#74983=CARTESIAN_POINT ( 'NONE',  ( 4.900006679340000559, 1499.255191946190052, 229.7873568473989963 ) ) ;
#74984=CARTESIAN_POINT ( 'NONE',  ( 2.029027972364500165, 1429.198891036370014, 217.1629461471520131 ) ) ;
#74985=CARTESIAN_POINT ( 'NONE',  ( -7.675048655830000399, 1425.718923958530013, 206.0025236838089882 ) ) ;
#74989=CARTESIAN_POINT ( 'NONE',  ( 7.324673508793529741, 1425.042193375519901, 212.6072707562309745 ) ) ;
#74992=VECTOR ( 'NONE', #70168, 1000.000000000000114 ) ;
#74996=CARTESIAN_POINT ( 'NONE',  ( -6.119584387729999797, 1461.516739551189858, 206.9548909377989787 ) ) ;
#74997=CARTESIAN_POINT ( 'NONE',  ( -4.329448776040000446, 1515.064792882589927, 207.2788837304390199 ) ) ;
#75005=CARTESIAN_POINT ( 'NONE',  ( 11.40660427760000140, 1502.131503807389890, 207.7526879073789985 ) ) ;
#75007=ORIENTED_EDGE ( 'NONE', *, *, #95918, .F. ) ;
#75012=CARTESIAN_POINT ( 'NONE',  ( 7.626975074059999748, 1491.048095285289946, 210.5944414621689873 ) ) ;
#75014=CARTESIAN_POINT ( 'NONE',  ( 4.544868981635990401, 1508.551704407889929, 213.0836524628859934 ) ) ;
#75023=CARTESIAN_POINT ( 'NONE',  ( 9.809383389668809627, 1433.663778845850175, 224.8559793928490080 ) ) ;
#75025=CARTESIAN_POINT ( 'NONE',  ( -11.87165566641069958, 1481.759760406750047, 209.4550520684960020 ) ) ;
#75029=CARTESIAN_POINT ( 'NONE',  ( 8.621399425004019790, 1503.742512659089925, 218.5082872257249846 ) ) ;
#75030=CARTESIAN_POINT ( 'NONE',  ( 7.424966210989999205, 1422.119254455250029, 195.6160877161989902 ) ) ;
#75031=CARTESIAN_POINT ( 'NONE',  ( 1.066132977100159973, 1431.451844506829730, 218.5524226113819850 ) ) ;
#75032=B_SPLINE_SURFACE_WITH_KNOTS ( 'NONE', 5, 5, ( 
 ( #57849, #91977, #66806, #15252, #65694, #23106 ),
 ( #30968, #92516, #100907, #99812, #83566, #24205 ),
 ( #22535, #90872, #49985, #6859, #56736, #14160 ),
 ( #48346, #58391, #82485, #15784, #18556, #1243 ),
 ( #77394, #43245, #76284, #17442, #78494, #42682 ),
 ( #696, #86331, #25853, #27533, #25297, #93609 ),
 ( #60054, #85218, #93071, #103117, #35945, #16345 ),
 ( #34825, #1808, #52750, #102560, #76840, #77936 ),
 ( #33712, #18011, #50543, #69012, #8509, #94172 ) ),
 .UNSPECIFIED., .F., .F., .F.,
 ( 6, 3, 6 ),
 ( 6, 6 ),
 ( 3.171312204904120247, 5.447745999499999492, 7.724179794085880069 ),
 ( -2.050297588106100003E-05, 2.000000000000000000 ),
 .UNSPECIFIED. ) ;
#75033=CARTESIAN_POINT ( 'NONE',  ( 10.25673954719900038, 1479.616108303600186, 205.9965886202919876 ) ) ;
#75037=CARTESIAN_POINT ( 'NONE',  ( 11.79199745574979907, 1426.669443530059880, 206.5449107423220028 ) ) ;
#75045=B_SPLINE_SURFACE_WITH_KNOTS ( 'NONE', 5, 5, ( 
 ( #19170, #12984, #36553, #47167, #28150, #81295 ),
 ( #53376, #87522, #70750, #96465, #19745, #82419 ),
 ( #83493, #100838, #107060, #99188, #40950, #72921 ),
 ( #56668, #81844, #14645, #84051, #30893, #56112 ),
 ( #15178, #5713, #22468, #92440, #39858, #74021 ),
 ( #6789, #32559, #21916, #75127, #109275, #65072 ),
 ( #108155, #31445, #91901, #65628, #66735, #30344 ),
 ( #99742, #23033, #64535, #48831, #90804, #57783 ),
 ( #15716, #48275, #108710, #14085, #49917, #24127 ) ),
 .UNSPECIFIED., .F., .F., .F.,
 ( 6, 3, 6 ),
 ( 6, 6 ),
 ( 3.182123501530000009, 5.472533560919999651, 7.762943620309999737 ),
 ( 0.000000000000000000, 2.000000000000000000 ),
 .UNSPECIFIED. ) ;
#75047=CARTESIAN_POINT ( 'NONE',  ( 9.844913728421918364, 1422.934237187859935, 210.2671035938940065 ) ) ;
#75048=CARTESIAN_POINT ( 'NONE',  ( 11.17620620616699867, 1424.953917489370269, 203.0360129599930303 ) ) ;
#75062=DIRECTION ( 'NONE',  ( 0.7600087925167849923, -0.4999999999970537456, -0.4151946956550922052 ) ) ;
#75070=CARTESIAN_POINT ( 'NONE',  ( 1.129779230730000084, 1515.569191395689813, 205.1526891147690037 ) ) ;
#75083=CARTESIAN_POINT ( 'NONE',  ( -2.170627950300000109, 1485.611815725089855, 197.4219880479989797 ) ) ;
#75084=CARTESIAN_POINT ( 'NONE',  ( 10.89260962470000038, 1478.390639884389884, 204.6475587744990037 ) ) ;
#75087=CARTESIAN_POINT ( 'NONE',  ( -8.817122548632680079, 1437.178451963229918, 212.6735601864489809 ) ) ;
#75096=CARTESIAN_POINT ( 'NONE',  ( 11.49495574083080029, 1422.044481766739864, 209.9123749212659789 ) ) ;
#75100=CARTESIAN_POINT ( 'NONE',  ( 2.673427297959769966, 1437.319176057519826, 227.4663404305809706 ) ) ;
#75102=CARTESIAN_POINT ( 'NONE',  ( 5.133103592700000384, 1472.975266187489979, 218.0948351415289892 ) ) ;
#75103=CARTESIAN_POINT ( 'NONE',  ( 10.50142226597180084, 1470.839680593169987, 210.1830287100939927 ) ) ;
#75113=CARTESIAN_POINT ( 'NONE',  ( 4.288117823509999482, 1445.747328214890103, 201.1375687007889894 ) ) ;
#75116=CARTESIAN_POINT ( 'NONE',  ( -2.031588052790000098, 1454.893423854089860, 198.8069212169990010 ) ) ;
#75127=CARTESIAN_POINT ( 'NONE',  ( 11.78257430589999899, 1500.696465547190201, 207.7593786822990012 ) ) ;
#75133=B_SPLINE_SURFACE_WITH_KNOTS ( 'NONE', 5, 1, ( 
 ( #66998, #49095 ),
 ( #23309, #6521 ),
 ( #40673, #32276 ),
 ( #109540, #49643 ),
 ( #74302, #65900 ),
 ( #90520, #82119 ) ),
 .UNSPECIFIED., .F., .F., .F.,
 ( 6, 6 ),
 ( 2, 2 ),
 ( 0.000000000000000000, 3.803024431209999889 ),
 ( 0.000000000000000000, 14.00000000000000000 ),
 .UNSPECIFIED. ) ;
#75139=ORIENTED_EDGE ( 'NONE', *, *, #94937, .F. ) ;
#75140=CARTESIAN_POINT ( 'NONE',  ( -19.58884347349999899, 1465.811382978989968, 204.1485388398990040 ) ) ;
#75142=CARTESIAN_POINT ( 'NONE',  ( 3.629220049600000220, 1485.493215689190038, 199.0019176958990101 ) ) ;
#75146=CARTESIAN_POINT ( 'NONE',  ( 10.56407631929999980, 1452.658139941989930, 209.7432180256290053 ) ) ;
#75148=CARTESIAN_POINT ( 'NONE',  ( -20.36206003818799815, 1507.989860361909905, 209.5068170956690210 ) ) ;
#75151=B_SPLINE_CURVE_WITH_KNOTS ( 'NONE', 3,
 ( #13368, #4456, #49220, #56514, #29637, #39700, #21761, #99034, #73866, #55962, #21204, #30740, #15022 ),
 .UNSPECIFIED., .F., .F.,
 ( 4, 3, 3, 3, 4 ),
 ( -19.77813379760699775, -19.44850676187209970, -18.33858777542890195, -17.22488228015659928, -16.10949595319999972 ),
 .UNSPECIFIED. ) ;
#75158=VERTEX_POINT ( 'NONE', #56122 ) ;
#75161=ORIENTED_EDGE ( 'NONE', *, *, #9616, .F. ) ;
#75164=VERTEX_POINT ( 'NONE', #96478 ) ;
#75167=CARTESIAN_POINT ( 'NONE',  ( -17.45421023344330180, 1419.943788952030218, 205.7215592404089932 ) ) ;
#75168=CARTESIAN_POINT ( 'NONE',  ( -9.903018300453069855, 1462.461387641800002, 206.7225876591880080 ) ) ;
#75170=CARTESIAN_POINT ( 'NONE',  ( 10.06269975749759915, 1469.306610116130059, 207.3997075874580105 ) ) ;
#75171=CARTESIAN_POINT ( 'NONE',  ( -4.824413881312672459, 1468.483554383926275, 219.2781897695970201 ) ) ;
#75172=CARTESIAN_POINT ( 'NONE',  ( 7.501852740990000434, 1494.251036354090274, 218.4424164909689807 ) ) ;
#75177=B_SPLINE_SURFACE_WITH_KNOTS ( 'NONE', 5, 1, ( 
 ( #17798, #101814 ),
 ( #101251, #24550 ),
 ( #58738, #92877 ),
 ( #16154, #41936 ),
 ( #45269, #97296 ),
 ( #20031, #10539 ) ),
 .UNSPECIFIED., .F., .F., .F.,
 ( 6, 6 ),
 ( 2, 2 ),
 ( 0.000000000000000000, 3.199138346760000307 ),
 ( 0.000000000000000000, 14.00000000000000000 ),
 .UNSPECIFIED. ) ;
#75179=ORIENTED_EDGE ( 'NONE', *, *, #104342, .F. ) ;
#75184=CARTESIAN_POINT ( 'NONE',  ( 3.586321559907979850, 1515.071394777460000, 213.2046241622850005 ) ) ;
#75186=CARTESIAN_POINT ( 'NONE',  ( -4.329448776040000446, 1515.064792882589927, 211.4519800877889963 ) ) ;
#75192=CARTESIAN_POINT ( 'NONE',  ( -15.46336752740000087, 1415.677402202029953, 209.5779191499580065 ) ) ;
#75193=FACE_OUTER_BOUND ( 'NONE', #91195, .T. ) ;
#75195=CARTESIAN_POINT ( 'NONE',  ( -5.460803535712269507, 1427.449714376620022, 201.5391232999229771 ) ) ;
#75204=ADVANCED_FACE ( 'NONE', ( #88642 ), #102664, .F. ) ;
#75206=CARTESIAN_POINT ( 'NONE',  ( 3.965334566925400761, 1454.048335879079787, 217.6203598810320159 ) ) ;
#75208=DIRECTION ( 'NONE',  ( 1.000000000000000000, 0.000000000000000000, 0.000000000000000000 ) ) ;
#75210=CARTESIAN_POINT ( 'NONE',  ( -15.08324830079999934, 1416.126940580989867, 205.9268786477289837 ) ) ;
#75214=B_SPLINE_SURFACE_WITH_KNOTS ( 'NONE', 5, 5, ( 
 ( #2408, #83468, #30317, #40925, #91879, #22438 ),
 ( #39273, #48244, #99158, #31974, #25622, #57760 ),
 ( #6763, #30866, #56087, #73446, #98622, #48804 ),
 ( #90213, #13497, #31417, #82387, #23566, #56639 ),
 ( #47687, #107580, #81815, #99711, #5117, #90774 ),
 ( #108683, #8823, #65042, #6218, #108122, #43008 ),
 ( #40370, #49343, #14617, #75103, #14056, #15152 ),
 ( #109251, #64505, #32535, #66706, #5686, #39830 ),
 ( #73992, #65599, #66165, #59814, #100815, #74550 ) ),
 .UNSPECIFIED., .F., .F., .F.,
 ( 6, 3, 6 ),
 ( 6, 6 ),
 ( 3.122008137489260093, 5.367142198119999819, 7.612276258760739545 ),
 ( -0.0004406524307360239786, 2.000000000000000000 ),
 .UNSPECIFIED. ) ;
#75215=CARTESIAN_POINT ( 'NONE',  ( -16.21759533281229082, 1419.733967092127386, 209.9202815302434146 ) ) ;
#75216=CARTESIAN_POINT ( 'NONE',  ( -5.294961033159999886, 1496.721944649390025, 219.0642768234689868 ) ) ;
#75217=CARTESIAN_POINT ( 'NONE',  ( 0.01122475199670090046, 1477.924429480590106, 201.4578446915589893 ) ) ;
#75231=CARTESIAN_POINT ( 'NONE',  ( -2.416613126592233485, 1507.334987533291041, 221.5267771657985918 ) ) ;
#75239=CARTESIAN_POINT ( 'NONE',  ( 20.31210344360099995, 1432.638797527460156, 214.7986899441419837 ) ) ;
#75241=CARTESIAN_POINT ( 'NONE',  ( 20.33509335567159937, 1432.834523802549938, 214.7556744266179862 ) ) ;
#75243=VECTOR ( 'NONE', #69618, 1000.000000000000114 ) ;
#75254=CARTESIAN_POINT ( 'NONE',  ( -16.34717785500199838, 1420.685724369499894, 203.2930982450899933 ) ) ;
#75267=CARTESIAN_POINT ( 'NONE',  ( 2.593334035529999859, 1445.992680618890063, 199.3398764938089869 ) ) ;
#75272=CARTESIAN_POINT ( 'NONE',  ( -4.161829183451589920, 1463.201391561070068, 200.2643698894640067 ) ) ;
#75289=CARTESIAN_POINT ( 'NONE',  ( -12.35076168520000017, 1502.691457114289960, 208.7665132982610032 ) ) ;
#75300=EDGE_CURVE ( 'NONE', #27470, #110516, #50800, .T. ) ;
#75334=CARTESIAN_POINT ( 'NONE',  ( 1.842962231260000028, 1515.551704408389924, 205.2922258481490303 ) ) ;
#75341=CARTESIAN_POINT ( 'NONE',  ( -3.179033946939999744, 1457.997354113189886, 219.3203918502989893 ) ) ;
#75342=CARTESIAN_POINT ( 'NONE',  ( -0.8729764147290010046, 1444.456550671890000, 218.0453103216389934 ) ) ;
#75349=CARTESIAN_POINT ( 'NONE',  ( -1.540849967930000064, 1430.630043029990020, 200.7745420285490070 ) ) ;
#75352=AXIS2_PLACEMENT_3D ( 'NONE', #53750, #2782, #36902 ) ;
#75355=CARTESIAN_POINT ( 'NONE',  ( -8.106555239546928249, 1438.741219031890068, 205.9368975051609993 ) ) ;
#75358=CARTESIAN_POINT ( 'NONE',  ( 9.966104638080198086, 1428.054312288505116, 211.9051864186514820 ) ) ;
#75374=CARTESIAN_POINT ( 'NONE',  ( -11.44024737950000059, 1501.432054422089777, 208.7106195065049974 ) ) ;
#75376=CARTESIAN_POINT ( 'NONE',  ( 4.788126387470001077, 1455.785790442590041, 218.6153184129890121 ) ) ;
#75378=CARTESIAN_POINT ( 'NONE',  ( -4.819998716129999750, 1445.927381020789880, 216.9237746421490272 ) ) ;
#75391=ORIENTED_EDGE ( 'NONE', *, *, #93122, .T. ) ;
#75394=CARTESIAN_POINT ( 'NONE',  ( 19.46449505960000081, 1499.405048825090034, 221.7536591926989900 ) ) ;
#75396=CARTESIAN_POINT ( 'NONE',  ( 12.45662817246929954, 1427.088122696140090, 206.6493147128259977 ) ) ;
#75399=CARTESIAN_POINT ( 'NONE',  ( -14.65275159090117185, 1420.238444720549978, 213.8660283808354166 ) ) ;
#75400=B_SPLINE_CURVE_WITH_KNOTS ( 'NONE', 3,
 ( #8303, #94513, #50878, #16142, #495, #43036, #34620, #76623, #16681, #69916, #59299, #101802, #42465, #110775, #76080, #68258, #26204, #104028, #102906, #26771 ),
 .UNSPECIFIED., .F., .F.,
 ( 4, 2, 2, 2, 1, 1, 1, 1, 2, 2, 2, 4 ),
 ( 0.000000000000000000, 0.2499999999997821742, 0.3749999999996731503, 0.4374999999996273536, 0.4687499999995982658, 0.4843749999995810573, 0.4921874999995723976, 0.4960937499995769495, 0.4980468749995792810, 0.4999999999995815569, 0.7499999999997908340, 1.000000000000000000 ),
 .UNSPECIFIED. ) ;
#75407=ORIENTED_EDGE ( 'NONE', *, *, #43441, .F. ) ;
#75408=CARTESIAN_POINT ( 'NONE',  ( -4.327308595631589760, 1515.146523075020013, 209.5795434418390073 ) ) ;
#75414=CARTESIAN_POINT ( 'NONE',  ( 5.169811769132760304, 1424.207592462389812, 193.2980118299309993 ) ) ;
#75417=CARTESIAN_POINT ( 'NONE',  ( 2.175409717514719593E-31, 1397.551704408390151, 209.1218459616989946 ) ) ;
#75423=EDGE_CURVE ( 'NONE', #108598, #94471, #101352, .T. ) ;
#75443=CARTESIAN_POINT ( 'NONE',  ( 6.754813038153810290, 1440.797395171449807, 214.9116427326270014 ) ) ;
#75448=CARTESIAN_POINT ( 'NONE',  ( -9.119231684200059362, 1439.059512825920137, 208.3665791233769937 ) ) ;
#75452=VERTEX_POINT ( 'NONE', #60266 ) ;
#75453=CARTESIAN_POINT ( 'NONE',  ( 20.22421167039999901, 1476.021596313489908, 210.1180608805510133 ) ) ;
#75457=CARTESIAN_POINT ( 'NONE',  ( -4.251676037229999316, 1413.133656259280087, 207.7220070843589781 ) ) ;
#75459=CARTESIAN_POINT ( 'NONE',  ( 9.904447724410001541, 1489.619655155790042, 203.3666065851589906 ) ) ;
#75461=CARTESIAN_POINT ( 'NONE',  ( 4.210705291133630013, 1430.371004163770067, 217.6270284791030178 ) ) ;
#75475=CARTESIAN_POINT ( 'NONE',  ( -11.37137302997330046, 1470.992257629510050, 208.1706243720159932 ) ) ;
#75476=CARTESIAN_POINT ( 'NONE',  ( -6.470239033145795737, 1508.340629334880305, 219.9570550858604179 ) ) ;
#75481=CARTESIAN_POINT ( 'NONE',  ( -9.898190092519600469, 1471.698199896249889, 211.3831928317650295 ) ) ;
#75487=VECTOR ( 'NONE', #26464, 999.9999999999998863 ) ;
#75488=CARTESIAN_POINT ( 'NONE',  ( -14.74403395979999942, 1507.703932417990245, 209.3705301297690085 ) ) ;
#75489=CARTESIAN_POINT ( 'NONE',  ( 7.526684039890001010, 1423.047588554429922, 195.6744588065990058 ) ) ;
#75494=CARTESIAN_POINT ( 'NONE',  ( -3.906031934150000051, 1515.551704408389924, 207.6332190043490016 ) ) ;
#75498=CARTESIAN_POINT ( 'NONE',  ( 12.02265620508110189, 1492.768319540230095, 211.9938273525619934 ) ) ;
#75499=CARTESIAN_POINT ( 'NONE',  ( -2.341977691500000347, 1457.699844493290129, 219.5360100213989938 ) ) ;
#75504=CARTESIAN_POINT ( 'NONE',  ( -0.2725765502280009800, 1430.103961438589977, 217.4715266419189845 ) ) ;
#75511=CARTESIAN_POINT ( 'NONE',  ( 11.74542637677500068, 1479.756186535490087, 210.0649862889210056 ) ) ;
#75514=CARTESIAN_POINT ( 'NONE',  ( 3.868582513889999852, 1449.766611533390005, 190.4179587020989857 ) ) ;
#75516=CARTESIAN_POINT ( 'NONE',  ( -12.46763692646640109, 1508.551704408389924, 216.9465170557990064 ) ) ;
#75517=CARTESIAN_POINT ( 'NONE',  ( 0.4463512173630010405, 1458.283482072889910, 202.2977778284289911 ) ) ;
#75520=CARTESIAN_POINT ( 'NONE',  ( 7.544839107842309822, 1434.691991358320138, 204.7085460358119917 ) ) ;
#75529=CARTESIAN_POINT ( 'NONE',  ( 2.330134126678752526, 1515.492058413687573, 213.2603893528570893 ) ) ;
#75531=CARTESIAN_POINT ( 'NONE',  ( 1.916663648440000145, 1477.644687901090037, 198.8912423860989804 ) ) ;
#75538=CARTESIAN_POINT ( 'NONE',  ( -8.145910945669999847, 1424.779583588550167, 207.8601695130389828 ) ) ;
#75541=CARTESIAN_POINT ( 'NONE',  ( 2.330134126767420266, 1515.064792882699976, 204.7923971855439902 ) ) ;
#75542=CARTESIAN_POINT ( 'NONE',  ( 7.524442094865539943, 1425.458146191759852, 212.2002832223970188 ) ) ;
#75555=VERTEX_POINT ( 'NONE', #81259 ) ;
#75556=CARTESIAN_POINT ( 'NONE',  ( 10.92766316885620093, 1501.618323021010156, 205.6861136770480130 ) ) ;
#75579=CARTESIAN_POINT ( 'NONE',  ( 0.8500299760647389569, 1445.209765166890065, 199.0867373374109945 ) ) ;
#75584=CARTESIAN_POINT ( 'NONE',  ( -4.804127539825289617, 1508.551704408389924, 212.5477707811770074 ) ) ;
#75585=CARTESIAN_POINT ( 'NONE',  ( 8.400707445830571274, 1503.837797309470034, 218.7125449626740021 ) ) ;
#75586=CARTESIAN_POINT ( 'NONE',  ( 7.595989987639999441, 1421.918083777009997, 195.7234947746989917 ) ) ;
#75587=EDGE_CURVE ( 'NONE', #91119, #92844, #41487, .T. ) ;
#75589=CARTESIAN_POINT ( 'NONE',  ( -5.202919524220000369, 1495.777348644990070, 199.0561099548990001 ) ) ;
#75593=CARTESIAN_POINT ( 'NONE',  ( 10.69099011935269949, 1423.897063905130153, 206.6970677081539804 ) ) ;
#75594=B_SPLINE_CURVE_WITH_KNOTS ( 'NONE', 3,
 ( #84975, #46336, #105113, #62603 ),
 .UNSPECIFIED., .F., .F.,
 ( 4, 4 ),
 ( 0.000000000000000000, 1.000000000000000000 ),
 .UNSPECIFIED. ) ;
#75598=VERTEX_POINT ( 'NONE', #99848 ) ;
#75604=CARTESIAN_POINT ( 'NONE',  ( 12.08651861739819999, 1426.128252729390169, 202.8034848243579802 ) ) ;
#75605=CARTESIAN_POINT ( 'NONE',  ( -10.98588173227549980, 1462.620677329530054, 207.9438354903729760 ) ) ;
#75610=CARTESIAN_POINT ( 'NONE',  ( -11.03823282802460071, 1462.321972888460095, 209.2524123285700171 ) ) ;
#75612=CARTESIAN_POINT ( 'NONE',  ( 11.86347265473209944, 1425.940497895709996, 201.1513796338190048 ) ) ;
#75613=CARTESIAN_POINT ( 'NONE',  ( 8.832652841333949567, 1464.232421199639930, 213.8219978802969763 ) ) ;
#75620=CARTESIAN_POINT ( 'NONE',  ( 1.466212339980000001, 1515.204044912790096, 204.7960436283990191 ) ) ;
#75621=CARTESIAN_POINT ( 'NONE',  ( 12.67165775215690005, 1426.886500604199910, 205.4076336300960008 ) ) ;
#75622=CARTESIAN_POINT ( 'NONE',  ( -14.38096573875979978, 1422.143734374870064, 196.2925565939719945 ) ) ;
#75624=CARTESIAN_POINT ( 'NONE',  ( -19.16657957493040243, 1419.018181932309972, 207.3808575570400023 ) ) ;
#75638=CARTESIAN_POINT ( 'NONE',  ( -7.199110364057590417, 1435.605555164340103, 215.2453670761979936 ) ) ;
#75645=CARTESIAN_POINT ( 'NONE',  ( 12.30985188076150116, 1427.199944344410142, 207.2898684024129921 ) ) ;
#75651=CARTESIAN_POINT ( 'NONE',  ( 2.122693458210000106, 1474.244506326290093, 219.5571033596989992 ) ) ;
#75654=CARTESIAN_POINT ( 'NONE',  ( -5.387811863060000483, 1496.648312753189884, 199.2595355468089906 ) ) ;
#75661=CARTESIAN_POINT ( 'NONE',  ( -1.030872721199999953, 1455.330695093189888, 198.6237620522990142 ) ) ;
#75670=VERTEX_POINT ( 'NONE', #100416 ) ;
#75671=DIRECTION ( 'NONE',  ( 9.341989762165448955E-47, -1.000000000000000000, 1.836970198721029688E-16 ) ) ;
#75680=CARTESIAN_POINT ( 'NONE',  ( 12.58697395272539943, 1501.023083793659907, 210.9163362933149983 ) ) ;
#75681=EDGE_CURVE ( 'NONE', #93538, #18777, #5382, .T. ) ;
#75683=CARTESIAN_POINT ( 'NONE',  ( 4.940370962924140130, 1508.551704408389924, 212.0905280059049858 ) ) ;
#75685=ORIENTED_EDGE ( 'NONE', *, *, #23261, .F. ) ;
#75686=CARTESIAN_POINT ( 'NONE',  ( -13.67844991905460006, 1504.250345474479900, 227.6838247662160200 ) ) ;
#75688=VERTEX_POINT ( 'NONE', #35984 ) ;
#75689=ORIENTED_EDGE ( 'NONE', *, *, #7705, .T. ) ;
#75691=CARTESIAN_POINT ( 'NONE',  ( 10.31264293309589952, 1453.306623136699955, 211.6178708374930011 ) ) ;
#75692=CARTESIAN_POINT ( 'NONE',  ( -7.015915899421429458, 1508.242408774839987, 219.9931816339760076 ) ) ;
#75693=CARTESIAN_POINT ( 'NONE',  ( -13.58041482308779990, 1508.551704408389924, 210.3416170982540052 ) ) ;
#75696=ADVANCED_FACE ( 'NONE', ( #18051 ), #62577, .T. ) ;
#75701=ORIENTED_EDGE ( 'NONE', *, *, #78179, .F. ) ;
#75710=CARTESIAN_POINT ( 'NONE',  ( -6.593958911874039153, 1433.916835198372837, 214.5366901220844511 ) ) ;
#75711=( BOUNDED_CURVE ( )  B_SPLINE_CURVE ( 3, ( #13030, #106027, #39358, #73532 ),
 .UNSPECIFIED., .F., .F. ) 
 B_SPLINE_CURVE_WITH_KNOTS ( ( 4, 4 ),
 ( 1.013003765281151880, 2.128589034411239922 ),
 .UNSPECIFIED. ) 
 CURVE ( )  GEOMETRIC_REPRESENTATION_ITEM ( )  RATIONAL_B_SPLINE_CURVE ( ( 1.000000000000000000, 0.8989503786704379218, 0.8989503786704379218, 1.000000000000000000 ) ) 
 REPRESENTATION_ITEM ( '' )  );
#75714=CARTESIAN_POINT ( 'NONE',  ( 11.00530662964919948, 1470.220588418350189, 206.9530455906469797 ) ) ;
#75715=CARTESIAN_POINT ( 'NONE',  ( -9.853806547159999596, 1472.519282585889869, 204.9780994919989894 ) ) ;
#75716=CARTESIAN_POINT ( 'NONE',  ( -11.71397076299980000, 1489.483175994190105, 212.5377881273170146 ) ) ;
#75719=CARTESIAN_POINT ( 'NONE',  ( -20.79406209140000072, 1505.269740423389976, 209.4146929180660095 ) ) ;
#75720=CARTESIAN_POINT ( 'NONE',  ( 3.587095331290290012, 1466.405175726029938, 198.6593342341859909 ) ) ;
#75730=CARTESIAN_POINT ( 'NONE',  ( -2.319252365495519719, 1483.729198182639948, 198.7017601680090024 ) ) ;
#75731=CARTESIAN_POINT ( 'NONE',  ( -11.67852220755739800, 1501.333649510869918, 211.3056319267720085 ) ) ;
#75734=CARTESIAN_POINT ( 'NONE',  ( -1.567668168089999980, 1508.358814145789893, 220.7516519924990064 ) ) ;
#75742=CARTESIAN_POINT ( 'NONE',  ( -20.67632449137469663, 1505.206979486720002, 209.5612231824529772 ) ) ;
#75753=CARTESIAN_POINT ( 'NONE',  ( -15.94926467029999984, 1417.442432002970236, 205.6519267168989984 ) ) ;
#75756=CARTESIAN_POINT ( 'NONE',  ( -8.637984804879090817, 1437.135132880460105, 209.2914201311819795 ) ) ;
#75757=CARTESIAN_POINT ( 'NONE',  ( -7.661470012249999684, 1498.708137977089791, 218.7331922414889789 ) ) ;
#75777=CARTESIAN_POINT ( 'NONE',  ( -17.60265120761850000, 1440.931801637090075, 218.9608602370630024 ) ) ;
#75779=CARTESIAN_POINT ( 'NONE',  ( -16.61337445554759995, 1463.629612650639956, 220.4655171656389996 ) ) ;
#75785=CARTESIAN_POINT ( 'NONE',  ( 10.34950188612880062, 1451.639534178259964, 207.2650128704659949 ) ) ;
#75808=B_SPLINE_CURVE_WITH_KNOTS ( 'NONE', 3,
 ( #73445, #12957, #72352, #48803 ),
 .UNSPECIFIED., .F., .F.,
 ( 4, 4 ),
 ( 0.000000000000000000, 1.000000000000000000 ),
 .UNSPECIFIED. ) ;
#75811=CARTESIAN_POINT ( 'NONE',  ( 2.345547646620000037, 1419.146311973829825, 204.4639097625889974 ) ) ;
#75813=CARTESIAN_POINT ( 'NONE',  ( 3.716253841760000398, 1442.231740553789905, 214.0742819844890050 ) ) ;
#75819=B_SPLINE_CURVE_WITH_KNOTS ( 'NONE', 5,
 ( #87207, #63152, #108275, #97252, #46339, #37916, #63688, #10499, #2127 ),
 .UNSPECIFIED., .F., .F.,
 ( 6, 3, 6 ),
 ( 0.000000000000000000, 0.6923720093109234641, 1.000000000000000000 ),
 .UNSPECIFIED. ) ;
#75844=CARTESIAN_POINT ( 'NONE',  ( -15.13199540178550073, 1508.551704408389924, 210.3648847345600075 ) ) ;
#75853=CARTESIAN_POINT ( 'NONE',  ( -20.86254339170000094, 1504.682062816289999, 214.2159060785090219 ) ) ;
#75862=CARTESIAN_POINT ( 'NONE',  ( -4.932889665030000259, 1462.240114355689911, 204.2595497230389867 ) ) ;
#75867=CARTESIAN_POINT ( 'NONE',  ( -9.568540505426021525, 1448.523985602899984, 209.1776060292260127 ) ) ;
#75877=CARTESIAN_POINT ( 'NONE',  ( 4.647692645760000296, 1467.200465493689990, 217.9234193686490073 ) ) ;
#75894=CARTESIAN_POINT ( 'NONE',  ( -9.982373020641928107, 1439.278825435209910, 208.9079553162600007 ) ) ;
#75895=CARTESIAN_POINT ( 'NONE',  ( -3.983717799079939503, 1515.551844914359890, 211.4517850765819844 ) ) ;
#75898=CARTESIAN_POINT ( 'NONE',  ( 3.829620113920000346, 1515.551704408389924, 211.4519800804890224 ) ) ;
#75908=CARTESIAN_POINT ( 'NONE',  ( 3.001031723810000162, 1456.247125019289797, 219.3218834261989798 ) ) ;
#75910=CARTESIAN_POINT ( 'NONE',  ( -8.051936654369999502, 1448.101386734190100, 213.6171964053189924 ) ) ;
#75914=CARTESIAN_POINT ( 'NONE',  ( 7.005078520870000602, 1424.882473908839984, 213.2032269817289887 ) ) ;
#75919=FACE_OUTER_BOUND ( 'NONE', #8150, .T. ) ;
#75933=CARTESIAN_POINT ( 'NONE',  ( -9.103497831145899610, 1449.500276181969866, 210.3008157486750065 ) ) ;
#75939=VECTOR ( 'NONE', #107370, 1000.000000000000000 ) ;
#75949=B_SPLINE_SURFACE_WITH_KNOTS ( 'NONE', 5, 1, ( 
 ( #33036, #31387 ),
 ( #49862, #22970 ),
 ( #32506, #75622 ),
 ( #57727, #84547 ),
 ( #66676, #92385 ),
 ( #100255, #100781 ),
 ( #39238, #91299 ),
 ( #24072, #14582 ),
 ( #40340, #74521 ),
 ( #108652, #58264 ),
 ( #83996, #7296 ),
 ( #101322, #31939 ),
 ( #24612, #66133 ),
 ( #23535, #58807 ),
 ( #92947, #73413 ),
 ( #107549, #30836 ),
 ( #94046, #68334 ),
 ( #1672, #15 ),
 ( #95714, #102989 ),
 ( #61581, #33577 ),
 ( #95166, #86760 ),
 ( #18422, #77813 ),
 ( #67769, #34696 ),
 ( #9494, #86203 ),
 ( #77272, #35252 ),
 ( #110301, #101882 ),
 ( #1122, #51507 ),
 ( #60476, #16759 ),
 ( #59377, #69437 ),
 ( #25173, #570 ),
 ( #85639, #52070 ),
 ( #18979, #61042 ),
 ( #68888, #10048 ),
 ( #102441, #93489 ),
 ( #8382, #52622 ),
 ( #94594, #50963 ),
 ( #25727, #53176 ),
 ( #42550, #44221 ),
 ( #42005, #34149 ),
 ( #7837, #76154 ),
 ( #85090, #17872 ),
 ( #76702, #69996 ),
 ( #78364, #8939 ),
 ( #59928, #17312 ),
 ( #35813, #43113 ),
 ( #26287, #103552 ),
 ( #26855, #43661 ),
 ( #104110, #27398 ),
 ( #21728, #80571 ),
 ( #29600, #63786 ),
 ( #63252, #88958 ) ),
 .UNSPECIFIED., .F., .F., .F.,
 ( 6, 3, 3, 3, 3, 3, 3, 3, 3, 3, 3, 3, 3, 3, 3, 3, 6 ),
 ( 2, 2 ),
 ( 0.000000000000000000, 28.69702819429999963, 61.04778752440000034, 93.62768910810000023, 123.7336603250000024, 156.1762685979999787, 187.3272846180000215, 220.4669312460000015, 237.3878297990000021, 254.2938300590000154, 289.2398204710000300, 325.3030936050000150, 360.8626869010000178, 395.8828220460000011, 432.6128460950000090, 468.8934854820000169, 502.1482307969999965 ),
 ( -3.370352201716179583E-07, 2.001701706146989945 ),
 .UNSPECIFIED. ) ;
#75964=CARTESIAN_POINT ( 'NONE',  ( 10.45057174002269917, 1460.060802511540032, 206.0227405347829972 ) ) ;
#75973=VERTEX_POINT ( 'NONE', #19143 ) ;
#75975=CARTESIAN_POINT ( 'NONE',  ( -11.37631282269999922, 1471.001977454990083, 208.1230460654030026 ) ) ;
#75977=ORIENTED_EDGE ( 'NONE', *, *, #20324, .T. ) ;
#75982=CARTESIAN_POINT ( 'NONE',  ( -4.284542764180000241, 1413.032915330810056, 207.8185126793489985 ) ) ;
#75984=CARTESIAN_POINT ( 'NONE',  ( 4.037057355369999101, 1486.123908481589979, 199.1211976137989836 ) ) ;
#75994=CARTESIAN_POINT ( 'NONE',  ( -16.79954545500000052, 1420.446322000240116, 203.4828821667790066 ) ) ;
#75995=CARTESIAN_POINT ( 'NONE',  ( -17.60942431520539841, 1508.551704408389924, 211.7095227962340118 ) ) ;
#75998=B_SPLINE_CURVE_WITH_KNOTS ( 'NONE', 5,
 ( #28015, #37523, #55443, #64397, #53810, #106377 ),
 .UNSPECIFIED., .F., .F.,
 ( 6, 6 ),
 ( 297.6813684100000046, 302.5784080160000258 ),
 .UNSPECIFIED. ) ;
#76001=CARTESIAN_POINT ( 'NONE',  ( -6.821413868843755779, 1508.365261329358646, 219.8335085021152224 ) ) ;
#76006=CARTESIAN_POINT ( 'NONE',  ( -13.10445383010389975, 1418.121923837399891, 200.6546514748530115 ) ) ;
#76009=ORIENTED_EDGE ( 'NONE', *, *, #23098, .F. ) ;
#76017=CARTESIAN_POINT ( 'NONE',  ( -1.840383241931389913, 1487.831799196779912, 219.8181463656999881 ) ) ;
#76018=CARTESIAN_POINT ( 'NONE',  ( -4.324092172210000307, 1515.269353063089966, 208.7601266040480255 ) ) ;
#76021=EDGE_CURVE ( 'NONE', #8596, #4497, #64647, .T. ) ;
#76023=ADVANCED_FACE ( 'NONE', ( #57763 ), #44695, .F. ) ;
#76025=CARTESIAN_POINT ( 'NONE',  ( 4.780307568339999591, 1467.625956517089890, 217.8721402715589761 ) ) ;
#76026=CARTESIAN_POINT ( 'NONE',  ( 11.10832711078520063, 1491.515140723940021, 210.2565573149119871 ) ) ;
#76028=CARTESIAN_POINT ( 'NONE',  ( -2.695638927469999668, 1457.674280517889883, 219.0325817157390134 ) ) ;
#76034=CARTESIAN_POINT ( 'NONE',  ( 8.120708804965499183, 1436.294995401849974, 206.2774205879739782 ) ) ;
#76037=B_SPLINE_CURVE_WITH_KNOTS ( 'NONE', 5,
 ( #28315, #79833, #55194, #46795, #96064, #104461 ),
 .UNSPECIFIED., .F., .F.,
 ( 6, 6 ),
 ( -2.000000000000000000, 0.000000000000000000 ),
 .UNSPECIFIED. ) ;
#76040=CARTESIAN_POINT ( 'NONE',  ( -8.200764929360001787, 1500.840159096690059, 209.4951459900700286 ) ) ;
#76044=CARTESIAN_POINT ( 'NONE',  ( 11.77666586973660046, 1479.544451823169993, 209.3554088579860206 ) ) ;
#76047=CYLINDRICAL_SURFACE ( 'NONE', #91032, 2.458500000000005237 ) ;
#76049=FACE_OUTER_BOUND ( 'NONE', #86107, .T. ) ;
#76051=CARTESIAN_POINT ( 'NONE',  ( 2.968366584736970015, 1486.970885391709999, 197.5475828882330234 ) ) ;
#76052=CARTESIAN_POINT ( 'NONE',  ( 7.040216406195790810, 1434.373471180939987, 203.9688476978490144 ) ) ;
#76055=ORIENTED_EDGE ( 'NONE', *, *, #34423, .T. ) ;
#76056=VECTOR ( 'NONE', #56463, 1000.000000000000000 ) ;
#76057=CARTESIAN_POINT ( 'NONE',  ( -18.28539703770000102, 1466.456797679889860, 217.8105514170289894 ) ) ;
#76060=DIRECTION ( 'NONE',  ( 0.000000000000000000, -1.836970198721029688E-16, -1.000000000000000000 ) ) ;
#76067=CARTESIAN_POINT ( 'NONE',  ( -3.269259737370000085, 1476.740802117289832, 199.2818558395189825 ) ) ;
#76069=ADVANCED_FACE ( 'NONE', ( #94078 ), #68747, .T. ) ;
#76075=CARTESIAN_POINT ( 'NONE',  ( -8.180909276350000425, 1424.652263318880159, 208.1606179922690103 ) ) ;
#76076=EDGE_CURVE ( 'NONE', #37425, #104484, #47383, .T. ) ;
#76080=CARTESIAN_POINT ( 'NONE',  ( -6.643844541757576216, 1470.948041183543182, 216.7502065885994682 ) ) ;
#76081=CARTESIAN_POINT ( 'NONE',  ( 7.517250621253449339, 1425.897439506280080, 212.2678162509879769 ) ) ;
#76086=CARTESIAN_POINT ( 'NONE',  ( -10.93570548119130059, 1492.910398145819954, 207.3716705518500021 ) ) ;
#76089=CARTESIAN_POINT ( 'NONE',  ( -3.061551880244241186, 1475.979329965256511, 199.2479746720524076 ) ) ;
#76093=ORIENTED_EDGE ( 'NONE', *, *, #82208, .F. ) ;
#76098=ORIENTED_EDGE ( 'NONE', *, *, #110273, .T. ) ;
#76104=CARTESIAN_POINT ( 'NONE',  ( 3.788406704206539910, 1508.728291632010041, 213.4250813669160038 ) ) ;
#76115=CARTESIAN_POINT ( 'NONE',  ( -11.83501748325819847, 1481.582715289189991, 210.0201637637719898 ) ) ;
#76116=CARTESIAN_POINT ( 'NONE',  ( 1.248319867352440049, 1432.832940376729994, 200.7627304351539976 ) ) ;
#76117=CARTESIAN_POINT ( 'NONE',  ( -3.246944597254960208, 1508.551704408389924, 213.9909153047919972 ) ) ;
#76119=CARTESIAN_POINT ( 'NONE',  ( 8.175629841830000188, 1421.338625457219905, 196.0692449803989916 ) ) ;
#76120=CARTESIAN_POINT ( 'NONE',  ( -0.9950319637076819879, 1432.231308707049948, 218.5764185903129828 ) ) ;
#76121=CARTESIAN_POINT ( 'NONE',  ( 10.22475231824599895, 1479.684064890109994, 205.9930891779119975 ) ) ;
#76131=CARTESIAN_POINT ( 'NONE',  ( -10.82927499412819650, 1508.551704408370824, 209.2608739639107682 ) ) ;
#76134=CARTESIAN_POINT ( 'NONE',  ( 9.748898013885689551, 1427.681173174970127, 211.1332189737210001 ) ) ;
#76135=CARTESIAN_POINT ( 'NONE',  ( 12.33008173652610040, 1426.296687997340086, 202.7608368823210299 ) ) ;
#76136=CARTESIAN_POINT ( 'NONE',  ( 1.335254395760000046, 1430.413233478789834, 217.4945813416789804 ) ) ;
#76142=CARTESIAN_POINT ( 'NONE',  ( -10.57973492554160089, 1462.173887409690224, 209.2258057589959890 ) ) ;
#76144=CARTESIAN_POINT ( 'NONE',  ( 8.790767757275109062, 1424.094608705360088, 196.7971378858789819 ) ) ;
#76145=CARTESIAN_POINT ( 'NONE',  ( 6.263504934518880241, 1465.252758315099982, 218.2608339057509852 ) ) ;
#76146=CARTESIAN_POINT ( 'NONE',  ( -10.56986511919999927, 1482.340628623390103, 205.9074532915990119 ) ) ;
#76148=DIRECTION ( 'NONE',  ( 0.02091224828123190022, 0.9990482215818557998, 0.03827961371219716635 ) ) ;
#76149=CARTESIAN_POINT ( 'NONE',  ( -8.097026068654489706, 1425.580256812905645, 208.3196847037820021 ) ) ;
#76154=CARTESIAN_POINT ( 'NONE',  ( -17.84103558406399870, 1489.004100625149931, 195.1797355196500234 ) ) ;
#76156=CARTESIAN_POINT ( 'NONE',  ( -22.20130412889999860, 1417.681004048810109, 209.9662649635100138 ) ) ;
#76162=CARTESIAN_POINT ( 'NONE',  ( -18.22821675530000007, 1443.229620277490085, 204.5519556382290034 ) ) ;
#76169=CARTESIAN_POINT ( 'NONE',  ( 8.849375732825370378, 1449.202560831883147, 206.6011072519091272 ) ) ;
#76171=CARTESIAN_POINT ( 'NONE',  ( -3.117088932150390068, 1432.832834640699957, 217.3706902353420105 ) ) ;
#76179=CARTESIAN_POINT ( 'NONE',  ( 10.70122832801980017, 1423.012206936599796, 207.4581769705870329 ) ) ;
#76187=CARTESIAN_POINT ( 'NONE',  ( 1.864351022469999730, 1473.433313301389944, 219.1822183682990044 ) ) ;
#76191=CARTESIAN_POINT ( 'NONE',  ( -9.041914599929999241, 1494.936448903489918, 202.3768923597089895 ) ) ;
#76195=CARTESIAN_POINT ( 'NONE',  ( 7302.760118613915438, 5181.793945261120825, 11064.62217173819772 ) ) ;
#76196=CARTESIAN_POINT ( 'NONE',  ( 9.167612539120000292, 1450.047499010689990, 204.0226639485589999 ) ) ;
#76197=CARTESIAN_POINT ( 'NONE',  ( -21.59687142900000012, 1507.523380033690046, 209.4572543540780032 ) ) ;
#76199=EDGE_CURVE ( 'NONE', #59685, #108309, #76807, .T. ) ;
#76200=CARTESIAN_POINT ( 'NONE',  ( -1.202320767300000037, 1456.214200931789946, 199.5726487006490117 ) ) ;
#76203=ADVANCED_FACE ( 'NONE', ( #109663 ), #94650, .T. ) ;
#76207=ORIENTED_EDGE ( 'NONE', *, *, #44750, .T. ) ;
#76219=B_SPLINE_CURVE_WITH_KNOTS ( 'NONE', 3,
 ( #87123, #10413, #66363, #73652, #13145, #14263 ),
 .UNSPECIFIED., .F., .F.,
 ( 4, 2, 4 ),
 ( 0.000000000000000000, 0.5000000000000000000, 1.000000000000000000 ),
 .UNSPECIFIED. ) ;
#76222=CARTESIAN_POINT ( 'NONE',  ( 12.67146871665720020, 1500.791398092430200, 210.0979814907519767 ) ) ;
#76223=CARTESIAN_POINT ( 'NONE',  ( 3.818684287277759992, 1508.551704408389924, 213.7264380181929937 ) ) ;
#76234=CARTESIAN_POINT ( 'NONE',  ( -12.26971806897292261, 1417.403025294029476, 199.8085102575429062 ) ) ;
#76235=FACE_OUTER_BOUND ( 'NONE', #63568, .T. ) ;
#76236=CARTESIAN_POINT ( 'NONE',  ( -6.487838854381950071, 1454.049012225269962, 202.3499870543650161 ) ) ;
#76245=ORIENTED_EDGE ( 'NONE', *, *, #308, .T. ) ;
#76250=CARTESIAN_POINT ( 'NONE',  ( 6.708192185693589771, 1429.353568409279887, 215.8261836254480102 ) ) ;
#76251=CARTESIAN_POINT ( 'NONE',  ( -17.15734414464520086, 1420.193758488640015, 204.4307800783660127 ) ) ;
#76252=CARTESIAN_POINT ( 'NONE',  ( -9.639755125763619148, 1461.269863503290026, 208.0610523092789776 ) ) ;
#76255=CARTESIAN_POINT ( 'NONE',  ( -9.574683806340001269, 1473.399577885589906, 205.3280175804189867 ) ) ;
#76259=CARTESIAN_POINT ( 'NONE',  ( -5.099055259868809920, 1496.765404324240080, 199.0959566236750220 ) ) ;
#76263=B_SPLINE_CURVE_WITH_KNOTS ( 'NONE', 5,
 ( #89238, #46711, #29873, #64061, #4682, #64614 ),
 .UNSPECIFIED., .F., .F.,
 ( 6, 6 ),
 ( 266.2319129360000147, 276.0458535200000370 ),
 .UNSPECIFIED. ) ;
#76270=CARTESIAN_POINT ( 'NONE',  ( -14.53003990559999892, 1415.677402202029953, 213.1288439181290073 ) ) ;
#76274=CARTESIAN_POINT ( 'NONE',  ( -1.569490127089999909, 1507.974949271890182, 221.0030736986989837 ) ) ;
#76278=CARTESIAN_POINT ( 'NONE',  ( 19.55988977460000200, 1474.636381753090063, 214.0184790771390055 ) ) ;
#76284=CARTESIAN_POINT ( 'NONE',  ( -10.55795760898930169, 1481.591005463860029, 207.1796093610390130 ) ) ;
#76289=CARTESIAN_POINT ( 'NONE',  ( 1.875671004969999833, 1456.514200624189925, 219.5762891113990065 ) ) ;
#76296=CARTESIAN_POINT ( 'NONE',  ( -15.20766188370000194, 1415.439842373489910, 206.5207236011790144 ) ) ;
#76300=CARTESIAN_POINT ( 'NONE',  ( -8.607248916523710491, 1436.893216450120008, 209.7353648425139738 ) ) ;
#76303=CARTESIAN_POINT ( 'NONE',  ( -2.725379146709999922, 1470.857295113890132, 189.2740040492990090 ) ) ;
#76305=CARTESIAN_POINT ( 'NONE',  ( -10.93665447375030020, 1508.551709316179995, 207.6442539328949977 ) ) ;
#76315=B_SPLINE_CURVE_WITH_KNOTS ( 'NONE', 5,
 ( #89854, #47857, #4209, #5299, #39457, #20978 ),
 .UNSPECIFIED., .F., .F.,
 ( 6, 6 ),
 ( -2.000000000000000000, 0.000000000000000000 ),
 .UNSPECIFIED. ) ;
#76318=CARTESIAN_POINT ( 'NONE',  ( -5.534100668969379910, 1464.371862158079921, 199.5915835189479992 ) ) ;
#76322=CARTESIAN_POINT ( 'NONE',  ( 4.856733042310000137, 1485.951405104490050, 218.7380990343689859 ) ) ;
#76323=CARTESIAN_POINT ( 'NONE',  ( 10.49503676954149967, 1479.901654632730242, 207.2485989259390067 ) ) ;
#76325=CARTESIAN_POINT ( 'NONE',  ( 20.42700490659999701, 1433.617019421789792, 214.5837023497890073 ) ) ;
#76329=CARTESIAN_POINT ( 'NONE',  ( -2.487935012184434136, 1508.551704408389924, 204.2892291574235628 ) ) ;
#76352=CARTESIAN_POINT ( 'NONE',  ( 3.465081665767860031, 1515.493283046529996, 205.2090687340129875 ) ) ;
#76374=CARTESIAN_POINT ( 'NONE',  ( 11.19986414605820002, 1422.142818617800003, 210.4362617274329921 ) ) ;
#76384=CARTESIAN_POINT ( 'NONE',  ( -2.206960501559600107, 1422.422356592760025, 192.6328859643259932 ) ) ;
#76385=EDGE_LOOP ( 'NONE', ( #104025, #99946, #34160, #92767 ) ) ;
#76392=CARTESIAN_POINT ( 'NONE',  ( 2.281297470570000208, 1468.629604151690046, 216.0053196740190060 ) ) ;
#76400=ORIENTED_EDGE ( 'NONE', *, *, #60562, .T. ) ;
#76404=CARTESIAN_POINT ( 'NONE',  ( 0.3248848659079795476, 1494.310064355425538, 220.2531037086061758 ) ) ;
#76405=CARTESIAN_POINT ( 'NONE',  ( -3.777475378889999735, 1462.602678821090194, 203.1963512104490235 ) ) ;
#76406=CARTESIAN_POINT ( 'NONE',  ( 0.4160887415541561496, 1444.416418669234645, 218.0718905750308352 ) ) ;
#76408=CARTESIAN_POINT ( 'NONE',  ( 7.868158389100000427, 1422.937290482379922, 214.1570520181289794 ) ) ;
#76410=CARTESIAN_POINT ( 'NONE',  ( -10.36656297781870073, 1447.925473656809800, 209.2996031035340252 ) ) ;
#76415=CARTESIAN_POINT ( 'NONE',  ( -13.27214107118760111, 1508.445510704319986, 216.9337900148879896 ) ) ;
#76418=CARTESIAN_POINT ( 'NONE',  ( -1.541238598094009972E-13, 1515.051704408389924, 212.9514660752490158 ) ) ;
#76426=CARTESIAN_POINT ( 'NONE',  ( -2.532955078589999687, 1430.062185629989926, 201.0558263785989652 ) ) ;
#76427=EDGE_CURVE ( 'NONE', #52452, #72871, #91625, .T. ) ;
#76430=CARTESIAN_POINT ( 'NONE',  ( -6.852639342928195099, 1447.389009270719498, 215.1469147219418403 ) ) ;
#76431=VERTEX_POINT ( 'NONE', #39004 ) ;
#76437=CARTESIAN_POINT ( 'NONE',  ( 11.50779367390000019, 1502.003025289490097, 210.7563750071790025 ) ) ;
#76440=CARTESIAN_POINT ( 'NONE',  ( 8.758614224470001375, 1427.348506402559906, 211.4846174044990050 ) ) ;
#76454=CARTESIAN_POINT ( 'NONE',  ( -11.33871459559999906, 1500.797327991989960, 210.5565315030190163 ) ) ;
#76455=CARTESIAN_POINT ( 'NONE',  ( -15.01426432124087285, 1416.094347576616428, 205.4938507932126868 ) ) ;
#76458=CARTESIAN_POINT ( 'NONE',  ( -2.861397284679999764, 1445.646508516890208, 217.6990959301490136 ) ) ;
#76463=CARTESIAN_POINT ( 'NONE',  ( 7.910841848800000520, 1423.398885000399787, 212.8692358303489982 ) ) ;
#76466=CARTESIAN_POINT ( 'NONE',  ( -3.320856779727160202, 1454.266511067670081, 199.1807039058840019 ) ) ;
#76474=CARTESIAN_POINT ( 'NONE',  ( -21.58852250170129849, 1507.326192596420015, 209.4237101338769946 ) ) ;
#76483=CARTESIAN_POINT ( 'NONE',  ( -10.25042859964420039, 1447.425305017889968, 210.5414048152140083 ) ) ;
#76511=CARTESIAN_POINT ( 'NONE',  ( -10.37387122812170048, 1479.853456459100244, 210.7819233421560057 ) ) ;
#76526=CARTESIAN_POINT ( 'NONE',  ( -8.633016166312110329, 1493.573642282540050, 200.3527115318569827 ) ) ;
#76529=CARTESIAN_POINT ( 'NONE',  ( -17.26522478369999902, 1417.948008348349958, 205.1437062577190034 ) ) ;
#76530=CARTESIAN_POINT ( 'NONE',  ( -2.157536728406358684, 1378.913060387289988, 210.3005136483567981 ) ) ;
#76531=CARTESIAN_POINT ( 'NONE',  ( 5.537689631040000116, 1487.530061922989944, 199.3434706563589884 ) ) ;
#76536=FACE_OUTER_BOUND ( 'NONE', #9722, .T. ) ;
#76541=CARTESIAN_POINT ( 'NONE',  ( -2.480175250669919951, 1429.207669930499833, 200.0830571243679969 ) ) ;
#76547=CARTESIAN_POINT ( 'NONE',  ( -11.36767047984990064, 1471.003751822059940, 208.1245920186299827 ) ) ;
#76548=CARTESIAN_POINT ( 'NONE',  ( -4.166056713077788132, 1508.165813601425270, 220.6324487379284562 ) ) ;
#76551=CARTESIAN_POINT ( 'NONE',  ( 8.983202878996561225, 1460.605128901860098, 205.0537694474210184 ) ) ;
#76554=CARTESIAN_POINT ( 'NONE',  ( -6.433661733563849516, 1419.885808465230184, 194.8545971097019844 ) ) ;
#76559=CARTESIAN_POINT ( 'NONE',  ( -5.512326787969999309, 1497.963565169690128, 220.3136703888989985 ) ) ;
#76563=CARTESIAN_POINT ( 'NONE',  ( 8.873274052869998485, 1425.079924521729936, 195.6592732233990262 ) ) ;
#76566=CARTESIAN_POINT ( 'NONE',  ( 10.50320544853759941, 1422.350872714849856, 211.5057683799360007 ) ) ;
#76567=AXIS2_PLACEMENT_3D ( 'NONE', #49869, #7844, #17880 ) ;
#76568=CARTESIAN_POINT ( 'NONE',  ( -4.635490668534062664, 1377.970142912541405, 204.0379736860714956 ) ) ;
#76575=CARTESIAN_POINT ( 'NONE',  ( 11.12768290801760074, 1491.440051377930104, 209.9868098767680067 ) ) ;
#76581=CARTESIAN_POINT ( 'NONE',  ( 0.7162863658319988946, 1429.709265593189912, 217.4063670190490143 ) ) ;
#76582=EDGE_CURVE ( 'NONE', #2790, #43895, #35266, .T. ) ;
#76590=CARTESIAN_POINT ( 'NONE',  ( 11.56134810898769949, 1480.201629797219994, 211.4332244987409979 ) ) ;
#76594=CARTESIAN_POINT ( 'NONE',  ( -16.08708462094059755, 1508.551704408389924, 213.7294159091019878 ) ) ;
#76597=CARTESIAN_POINT ( 'NONE',  ( 2.819396220834549993, 1486.922886763410133, 197.5136065300459904 ) ) ;
#76598=CARTESIAN_POINT ( 'NONE',  ( 5.628941412700790181, 1434.147628282120195, 202.5779479739449869 ) ) ;
#76603=CARTESIAN_POINT ( 'NONE',  ( 22.16303642491469716, 1474.378995651259856, 210.0398025965960187 ) ) ;
#76605=CARTESIAN_POINT ( 'NONE',  ( 3.066583199566000534E-32, 1507.508085020990166, 209.1218459616989946 ) ) ;
#76607=CARTESIAN_POINT ( 'NONE',  ( -5.657316317590000310, 1475.078194850989803, 204.3863535599990087 ) ) ;
#76608=B_SPLINE_CURVE_WITH_KNOTS ( 'NONE', 3,
 ( #8222, #42388, #67615, #100630, #23376, #83291, #75995, #40187, #25569, #108497, #84929, #68181, #83841, #31782, #101728, #100096, #102288, #16600, #6589, #14966, #91689, #41840 ),
 .UNSPECIFIED., .F., .F.,
 ( 4, 3, 3, 3, 3, 3, 3, 4 ),
 ( -9.467922507749999994, -8.528615746326670077, -7.393658045039350313, -7.008072864428970483, -6.043576188583889675, -5.200792916686279632, -4.480935144650000090, -4.388980137787560132 ),
 .UNSPECIFIED. ) ;
#76610=CARTESIAN_POINT ( 'NONE',  ( 0.6219649428874711727, 1515.589553501007686, 213.1416252726859852 ) ) ;
#76613=CARTESIAN_POINT ( 'NONE',  ( -2.194372809809999936, 1475.747898641790016, 198.6287671099989893 ) ) ;
#76619=CARTESIAN_POINT ( 'NONE',  ( -7.634073948139999288, 1426.135584679400154, 206.2171369772389653 ) ) ;
#76620=ORIENTED_EDGE ( 'NONE', *, *, #109531, .F. ) ;
#76623=CARTESIAN_POINT ( 'NONE',  ( -7.032901808474493421, 1471.052634343683849, 216.4002283616353566 ) ) ;
#76624=CARTESIAN_POINT ( 'NONE',  ( 7.530331464701590427, 1425.809918452410102, 212.2263711254659881 ) ) ;
#76628=CARTESIAN_POINT ( 'NONE',  ( -10.94188635223400041, 1492.630926138539962, 207.2829489295590122 ) ) ;
#76630=CARTESIAN_POINT ( 'NONE',  ( -6.281421547999999966, 1461.340667028890039, 207.5740607322589995 ) ) ;
#76631=CARTESIAN_POINT ( 'NONE',  ( -4.138543392800874798, 1515.492058412108918, 207.2788837464903509 ) ) ;
#76632=CARTESIAN_POINT ( 'NONE',  ( 7.223461847829999449, 1425.153791230060051, 192.5261047659990084 ) ) ;
#76633=CARTESIAN_POINT ( 'NONE',  ( 3.873898975603070394, 1468.026799752889929, 218.3319420452740189 ) ) ;
#76638=CARTESIAN_POINT ( 'NONE',  ( 8.222217444529830388, 1435.932500431779999, 206.6299244032960019 ) ) ;
#76640=VERTEX_POINT ( 'NONE', #77453 ) ;
#76642=B_SPLINE_CURVE_WITH_KNOTS ( 'NONE', 3,
 ( #58621, #35057, #8188, #32839, #52436, #67032 ),
 .UNSPECIFIED., .F., .F.,
 ( 4, 2, 4 ),
 ( 0.000000000000000000, 0.5000000000000000000, 1.000000000000000000 ),
 .UNSPECIFIED. ) ;
#76643=CARTESIAN_POINT ( 'NONE',  ( -11.00421634129999937, 1481.586355903290041, 208.5478235484490028 ) ) ;
#76648=CARTESIAN_POINT ( 'NONE',  ( 4.678985465398590726, 1508.551704408389924, 213.1800342119370271 ) ) ;
#76649=EDGE_CURVE ( 'NONE', #40367, #32267, #583, .T. ) ;
#76651=EDGE_CURVE ( 'NONE', #56028, #13558, #84639, .T. ) ;
#76653=CARTESIAN_POINT ( 'NONE',  ( -5.842412022809999605, 1427.301855271020258, 202.1826430572290008 ) ) ;
#76657=CARTESIAN_POINT ( 'NONE',  ( 1.501528787941759813, 1445.491189390299951, 199.1508277339860058 ) ) ;
#76664=CARTESIAN_POINT ( 'NONE',  ( -2.968682043993700059, 1508.551704408389924, 214.0622169246639714 ) ) ;
#76666=CARTESIAN_POINT ( 'NONE',  ( 7.431286581940000247, 1422.782057261100135, 195.6224716579989718 ) ) ;
#76667=CARTESIAN_POINT ( 'NONE',  ( -3.114972218757349864, 1433.209950781340012, 218.1554066274329955 ) ) ;
#76680=CARTESIAN_POINT ( 'NONE',  ( 9.440304233305520043, 1422.746543296229902, 211.8015284199159964 ) ) ;
#76682=DIRECTION ( 'NONE',  ( -1.000000000000000000, 0.000000000000000000, 0.000000000000000000 ) ) ;
#76683=CARTESIAN_POINT ( 'NONE',  ( 1.245016291430000033, 1431.187216657390081, 218.1259619513589882 ) ) ;
#76688=CARTESIAN_POINT ( 'NONE',  ( -9.655872537241959819, 1460.619437666070098, 208.6456940018040029 ) ) ;
#76691=CARTESIAN_POINT ( 'NONE',  ( -1.842962215417937033, 1515.551704407335137, 213.1059277167897505 ) ) ;
#76696=CARTESIAN_POINT ( 'NONE',  ( -8.105593519943804282, 1425.120261978882354, 209.5236776171163910 ) ) ;
#76699=B_SPLINE_CURVE_WITH_KNOTS ( 'NONE', 5,
 ( #7944, #91953, #109325, #42113, #101992, #40996 ),
 .UNSPECIFIED., .F., .F.,
 ( 6, 6 ),
 ( 0.000000000000000000, 1.000000000000000000 ),
 .UNSPECIFIED. ) ;
#76702=CARTESIAN_POINT ( 'NONE',  ( 9.992001597533901602, 1491.422526970020044, 188.4943246393440006 ) ) ;
#76704=CARTESIAN_POINT ( 'NONE',  ( -16.16672696929999731, 1420.120271228960064, 210.5293282507990114 ) ) ;
#76707=VERTEX_POINT ( 'NONE', #100302 ) ;
#76715=VERTEX_POINT ( 'NONE', #49911 ) ;
#76716=B_SPLINE_SURFACE_WITH_KNOTS ( 'NONE', 5, 5, ( 
 ( #70993, #9389, #11053, #79363, #27292, #102872 ),
 ( #44108, #60923, #45224, #79915, #77701, #103427 ),
 ( #61473, #96151, #86095, #105110, #62601, #2677 ),
 ( #95600, #43552, #36247, #96717, #11602, #18320 ),
 ( #19987, #10494, #34585, #68771, #18868, #44666 ),
 ( #94478, #17751, #51954, #2121, #26735, #95052 ),
 ( #52511, #86641, #78243, #1556, #39555, #21623 ),
 ( #29489, #107306, #30033, #5397, #73729, #3778 ),
 ( #28958, #38440, #55278, #99436, #106206, #89949 ) ),
 .UNSPECIFIED., .F., .F., .F.,
 ( 6, 3, 6 ),
 ( 6, 6 ),
 ( 10.57355459961640065, 12.71109754730000141, 14.84862610992340137 ),
 ( -0.0004205665836232139773, 2.000000000000000000 ),
 .UNSPECIFIED. ) ;
#76721=CARTESIAN_POINT ( 'NONE',  ( -7.485129992997699766, 1435.765762796630042, 215.5585987123639882 ) ) ;
#76728=CARTESIAN_POINT ( 'NONE',  ( 10.15095921180179950, 1426.119696681420010, 208.5876670455920134 ) ) ;
#76736=CARTESIAN_POINT ( 'NONE',  ( 1.762362329279999917, 1472.996463562990130, 219.1807010226990258 ) ) ;
#76740=CARTESIAN_POINT ( 'NONE',  ( -6.949448346310000524, 1495.994811745590141, 200.2534193484290199 ) ) ;
#76745=CARTESIAN_POINT ( 'NONE',  ( 5.845440260250000186, 1447.515577236790023, 201.5716352439589798 ) ) ;
#76748=CARTESIAN_POINT ( 'NONE',  ( -3.264929865090000050, 1455.156803674389948, 200.1463034570790001 ) ) ;
#76756=CARTESIAN_POINT ( 'NONE',  ( -0.8447098492589989460, 1496.888790194590001, 197.4916273440990153 ) ) ;
#76757=CARTESIAN_POINT ( 'NONE',  ( 1.474632190929999975, 1495.646359947390010, 220.9745027109989906 ) ) ;
#76758=VERTEX_POINT ( 'NONE', #18472 ) ;
#76771=CARTESIAN_POINT ( 'NONE',  ( -4.992905592350000532, 1391.642135889690053, 214.6650328897389954 ) ) ;
#76772=CARTESIAN_POINT ( 'NONE',  ( -11.21638122688047368, 1413.913060387330006, 208.4170904300009397 ) ) ;
#76773=ORIENTED_EDGE ( 'NONE', *, *, #25335, .F. ) ;
#76775=CARTESIAN_POINT ( 'NONE',  ( 9.321518847882098058, 1461.563338749869899, 206.3986575956980118 ) ) ;
#76778=ORIENTED_EDGE ( 'NONE', *, *, #49993, .F. ) ;
#76779=CARTESIAN_POINT ( 'NONE',  ( -0.4039940643739989845, 1432.524637096890046, 203.3438492792190004 ) ) ;
#76782=CARTESIAN_POINT ( 'NONE',  ( -12.62024803869436340, 1417.247709474677322, 200.2862650437438674 ) ) ;
#76783=ADVANCED_FACE ( 'NONE', ( #110350 ), #69687, .T. ) ;
#76784=CARTESIAN_POINT ( 'NONE',  ( 4.290508133339999475, 1515.379316001789903, 209.4884471522930198 ) ) ;
#76790=CARTESIAN_POINT ( 'NONE',  ( 9.201685189691980682, 1450.874596308319951, 209.9835013892320035 ) ) ;
#76793=EDGE_LOOP ( 'NONE', ( #24551, #5312, #2703, #36790 ) ) ;
#76796=ORIENTED_EDGE ( 'NONE', *, *, #106350, .F. ) ;
#76805=CARTESIAN_POINT ( 'NONE',  ( -10.15849568003170056, 1462.015375114950075, 208.6822598999149818 ) ) ;
#76807=CIRCLE ( 'NONE', #41068, 11.71219856409999949 ) ;
#76809=CARTESIAN_POINT ( 'NONE',  ( -9.636570100870001099, 1473.857455401490142, 205.4329981810490153 ) ) ;
#76810=FACE_OUTER_BOUND ( 'NONE', #2670, .T. ) ;
#76815=CARTESIAN_POINT ( 'NONE',  ( 5.092807830394789903, 1466.926502071939922, 199.2585311702579816 ) ) ;
#76826=CARTESIAN_POINT ( 'NONE',  ( 0.8481724230196159287, 1515.120541028469916, 204.7938570022450051 ) ) ;
#76830=CARTESIAN_POINT ( 'NONE',  ( 0.6547232732189989246, 1508.551704408389924, 219.9513850608990140 ) ) ;
#76833=CARTESIAN_POINT ( 'NONE',  ( 3.035844568486590234, 1446.218552265309881, 199.4665232611309875 ) ) ;
#76836=CARTESIAN_POINT ( 'NONE',  ( 8.165488601299999871, 1502.104785131989956, 208.0160615438289824 ) ) ;
#76840=CARTESIAN_POINT ( 'NONE',  ( -11.40823118469380049, 1481.949762775670024, 208.3180590605030034 ) ) ;
#76842=CIRCLE ( 'NONE', #39353, 3.750000000000000000 ) ;
#76853=LINE ( 'NONE', #58951, #103351 ) ;
#76854=CARTESIAN_POINT ( 'NONE',  ( -15.62861107659999860, 1418.244676480490170, 203.0179540571090229 ) ) ;
#76857=CARTESIAN_POINT ( 'NONE',  ( -2.692717788947200486, 1485.501216450119955, 197.5304516791929927 ) ) ;
#76858=CARTESIAN_POINT ( 'NONE',  ( -16.64746823025755518, 1419.609048024772392, 209.0357172696779458 ) ) ;
#76861=CARTESIAN_POINT ( 'NONE',  ( 2.124170329769999643, 1471.509589720390068, 189.1723552809990281 ) ) ;
#76863=B_SPLINE_SURFACE_WITH_KNOTS ( 'NONE', 5, 1, ( 
 ( #21443, #46702 ),
 ( #6323, #5222 ),
 ( #32074, #40472 ),
 ( #48347, #99813 ),
 ( #97634, #72990 ),
 ( #80832, #74647 ) ),
 .UNSPECIFIED., .F., .F., .F.,
 ( 6, 6 ),
 ( 2, 2 ),
 ( 0.000000000000000000, 3.671445137310000106 ),
 ( 0.000000000000000000, 14.00000000000000000 ),
 .UNSPECIFIED. ) ;
#76864=CARTESIAN_POINT ( 'NONE',  ( -11.65521739879129903, 1507.535655379640275, 207.9035470749859940 ) ) ;
#76872=EDGE_CURVE ( 'NONE', #5037, #2310, #102099, .T. ) ;
#76876=DIRECTION ( 'NONE',  ( -1.000000000000000000, 0.000000000000000000, 0.000000000000000000 ) ) ;
#76883=CARTESIAN_POINT ( 'NONE',  ( 10.60758307464649874, 1480.113492495000173, 207.9930903275029834 ) ) ;
#76886=CARTESIAN_POINT ( 'NONE',  ( -17.66148164096410156, 1440.150380355800053, 218.7822556169580253 ) ) ;
#76892=CARTESIAN_POINT ( 'NONE',  ( 9.696539317786241341, 1436.240278671050191, 210.7713209817480049 ) ) ;
#76895=CARTESIAN_POINT ( 'NONE',  ( 5.529292985537660243, 1447.580617647699910, 200.5261424873660019 ) ) ;
#76896=DIRECTION ( 'NONE',  ( -0.07512831052118132402, 0.9801898970463382987, -0.1832580221614370231 ) ) ;
#76904=CARTESIAN_POINT ( 'NONE',  ( 7.365750702793119942, 1505.956296822819922, 218.2324441051819974 ) ) ;
#76906=ORIENTED_EDGE ( 'NONE', *, *, #100700, .F. ) ;
#76913=CARTESIAN_POINT ( 'NONE',  ( -4.487249775048080203, 1509.038615934839981, 211.6097811040130239 ) ) ;
#76928=ORIENTED_EDGE ( 'NONE', *, *, #56286, .F. ) ;
#76934=CARTESIAN_POINT ( 'NONE',  ( -19.67539872490000263, 1467.567198463789964, 206.2061548292190025 ) ) ;
#76935=CARTESIAN_POINT ( 'NONE',  ( 11.40789371488579995, 1422.073302846210026, 210.0656248370559922 ) ) ;
#76948=CARTESIAN_POINT ( 'NONE',  ( 1.370146406885849988, 1423.265678981450037, 192.5490732762039841 ) ) ;
#76951=CARTESIAN_POINT ( 'NONE',  ( -18.26458976723020200, 1508.551704408389924, 210.4136963709630095 ) ) ;
#76958=CARTESIAN_POINT ( 'NONE',  ( -2.930595334879239733, 1428.959675587809897, 200.2235252233409994 ) ) ;
#76987=B_SPLINE_CURVE_WITH_KNOTS ( 'NONE', 3,
 ( #7020, #69156, #101607, #59099, #101061, #24358, #33309, #59644, #15947, #85934, #60765, #15404, #302 ),
 .UNSPECIFIED., .F., .F.,
 ( 4, 3, 3, 3, 4 ),
 ( -3.420209351472869752, -3.144711398279999681, -1.710104561635330089, -1.461849369231190021, 0.000000000000000000 ),
 .UNSPECIFIED. ) ;
#76988=CARTESIAN_POINT ( 'NONE',  ( 3.172884302710000437, 1467.373997971989866, 218.6974001167089909 ) ) ;
#76993=CARTESIAN_POINT ( 'NONE',  ( -2.188303739500000233, 1431.240665291890082, 201.0188168257489849 ) ) ;
#76995=CARTESIAN_POINT ( 'NONE',  ( 10.58112656791359996, 1481.600201880140048, 209.5141384132439839 ) ) ;
#77000=B_SPLINE_CURVE_WITH_KNOTS ( 'NONE', 3,
 ( #40078, #75358, #82069, #40629, #109498, #49053 ),
 .UNSPECIFIED., .F., .F.,
 ( 4, 2, 4 ),
 ( 0.000000000000000000, 0.5000000000000000000, 1.000000000000000000 ),
 .UNSPECIFIED. ) ;
#77001=CARTESIAN_POINT ( 'NONE',  ( 4.777537831619650177, 1455.786797201459876, 218.6089316382710024 ) ) ;
#77002=CARTESIAN_POINT ( 'NONE',  ( -671.9628848459639130, -8383.748406600810995, -1657.040904779356197 ) ) ;
#77006=CARTESIAN_POINT ( 'NONE',  ( 11.58814563159999977, 1501.742621387089912, 209.9262120703820074 ) ) ;
#77009=B_SPLINE_SURFACE_WITH_KNOTS ( 'NONE', 5, 1, ( 
 ( #12137, #62024 ),
 ( #55272, #80459 ),
 ( #96712, #45219 ),
 ( #30028, #28953 ),
 ( #79357, #97790 ),
 ( #88853, #12691 ) ),
 .UNSPECIFIED., .F., .F., .F.,
 ( 6, 6 ),
 ( 2, 2 ),
 ( 0.000000000000000000, 3.930294876060000053 ),
 ( 0.000000000000000000, 14.00000000000000000 ),
 .UNSPECIFIED. ) ;
#77010=CARTESIAN_POINT ( 'NONE',  ( 7.481288447059999847, 1426.924569037480069, 212.2063472014090166 ) ) ;
#77014=FACE_OUTER_BOUND ( 'NONE', #95742, .T. ) ;
#77023=CARTESIAN_POINT ( 'NONE',  ( -11.77155278529999904, 1501.635673497090011, 210.8734570959489929 ) ) ;
#77026=CARTESIAN_POINT ( 'NONE',  ( 0.06756312569560819770, 1456.974508360119898, 219.7477876681689963 ) ) ;
#77028=CARTESIAN_POINT ( 'NONE',  ( 9.682511080499990541, 1436.279831232390052, 210.8541354582289955 ) ) ;
#77031=CARTESIAN_POINT ( 'NONE',  ( -9.771923492860000948, 1448.872168905890021, 190.8346797514990101 ) ) ;
#77037=ORIENTED_EDGE ( 'NONE', *, *, #93831, .F. ) ;
#77054=ORIENTED_EDGE ( 'NONE', *, *, #68125, .F. ) ;
#77069=ADVANCED_FACE ( 'NONE', ( #81997 ), #1724, .T. ) ;
#77075=AXIS2_PLACEMENT_3D ( 'NONE', #88837, #11582, #71534 ) ;
#77089=CARTESIAN_POINT ( 'NONE',  ( 6.686050678956539706, 1483.907811585419950, 213.3532383466159956 ) ) ;
#77098=CARTESIAN_POINT ( 'NONE',  ( -9.468502320038240327, 1493.161931906950031, 201.2760261155009971 ) ) ;
#77112=EDGE_CURVE ( 'NONE', #106272, #26067, #87446, .T. ) ;
#77113=CARTESIAN_POINT ( 'NONE',  ( -17.09580434209999922, 1420.284596455289829, 203.6963249145289865 ) ) ;
#77116=CARTESIAN_POINT ( 'NONE',  ( 6.813366145865759727, 1488.144601911519885, 204.7706368192809805 ) ) ;
#77118=ADVANCED_FACE ( 'NONE', ( #45561 ), #29470, .T. ) ;
#77122=CARTESIAN_POINT ( 'NONE',  ( -2.659206587534440835, 1508.055408576787386, 220.9016337176575178 ) ) ;
#77124=CARTESIAN_POINT ( 'NONE',  ( 10.79528402730720060, 1489.628194868570063, 207.4012257063180016 ) ) ;
#77125=CARTESIAN_POINT ( 'NONE',  ( -3.286480964850000408, 1456.341185808290220, 218.0120306903490075 ) ) ;
#77128=CARTESIAN_POINT ( 'NONE',  ( -11.81062501566809964, 1419.674596867499986, 197.5957448953309950 ) ) ;
#77129=CARTESIAN_POINT ( 'NONE',  ( 4.327152622306750018, 1515.152479455989806, 208.7968194348430018 ) ) ;
#77131=VERTEX_POINT ( 'NONE', #7233 ) ;
#77139=FACE_OUTER_BOUND ( 'NONE', #17527, .T. ) ;
#77140=CARTESIAN_POINT ( 'NONE',  ( 3.217389378496539720, 1424.184544469090042, 188.9579904087769933 ) ) ;
#77146=CARTESIAN_POINT ( 'NONE',  ( 10.42932300190150130, 1451.825531649119966, 207.6750499181110001 ) ) ;
#77154=CARTESIAN_POINT ( 'NONE',  ( -5.714377949607280627, 1458.767755790989895, 212.7178556816730008 ) ) ;
#77165=CARTESIAN_POINT ( 'NONE',  ( -1.080437161831740100, 1485.854186192430234, 197.2704867795639814 ) ) ;
#77171=ORIENTED_EDGE ( 'NONE', *, *, #28567, .T. ) ;
#77172=CARTESIAN_POINT ( 'NONE',  ( 22.23389067522870022, 1475.761154642579868, 209.7977657726480061 ) ) ;
#77182=CARTESIAN_POINT ( 'NONE',  ( -1.749524734880000043, 1475.561370704890123, 198.2000993585989761 ) ) ;
#77188=CARTESIAN_POINT ( 'NONE',  ( -5.303285988883490454, 1442.879254652209966, 200.5943008362860098 ) ) ;
#77193=CARTESIAN_POINT ( 'NONE',  ( 7.532490811327241076, 1425.518623867940050, 212.1875454003960044 ) ) ;
#77201=CARTESIAN_POINT ( 'NONE',  ( -0.4074389651556699632, 1487.893877509609638, 219.9700315476485457 ) ) ;
#77203=CARTESIAN_POINT ( 'NONE',  ( 7.890413475299999924, 1422.993678601120109, 213.8680409669790095 ) ) ;
#77204=CARTESIAN_POINT ( 'NONE',  ( -0.9496117000910009320, 1455.546544636789804, 215.7787860308390009 ) ) ;
#77227=CARTESIAN_POINT ( 'NONE',  ( -0.3874239798002959700, 1444.710807817890100, 199.0717356154370066 ) ) ;
#77230=CARTESIAN_POINT ( 'NONE',  ( 4.038582018629999659, 1515.598601288590089, 209.1218459616989946 ) ) ;
#77232=EDGE_CURVE ( 'NONE', #37845, #64533, #56706, .T. ) ;
#77233=CARTESIAN_POINT ( 'NONE',  ( -3.301717782203759999, 1508.551704408389924, 213.9725500436610162 ) ) ;
#77235=CARTESIAN_POINT ( 'NONE',  ( 8.003593684729999325, 1421.506473294969965, 195.9720126397990043 ) ) ;
#77251=CARTESIAN_POINT ( 'NONE',  ( 9.722118187324769067, 1428.114093149220025, 212.2006445887890038 ) ) ;
#77253=CARTESIAN_POINT ( 'NONE',  ( -11.02639390884469961, 1462.494802824179942, 208.5122157637580074 ) ) ;
#77259=CARTESIAN_POINT ( 'NONE',  ( -10.15934713503659914, 1461.826274973950149, 209.4099054465810070 ) ) ;
#77260=CARTESIAN_POINT ( 'NONE',  ( 18.26072392659999721, 1430.705547050490168, 200.8927042014090034 ) ) ;
#77261=CARTESIAN_POINT ( 'NONE',  ( 11.10393296898399917, 1422.031618569310012, 201.8322731501689873 ) ) ;
#77262=CARTESIAN_POINT ( 'NONE',  ( 4.577373674521229674, 1466.377811852470131, 218.3518963470609719 ) ) ;
#77266=CIRCLE ( 'NONE', #9398, 15.41143114519999990 ) ;
#77268=CARTESIAN_POINT ( 'NONE',  ( 1.847634001515719993, 1478.089546411300262, 198.8590795898780073 ) ) ;
#77270=CARTESIAN_POINT ( 'NONE',  ( -1.070047859720000050, 1515.100834970490041, 204.7933409809490115 ) ) ;
#77272=CARTESIAN_POINT ( 'NONE',  ( -18.32377787238529976, 1464.077817495989848, 217.4721512438379989 ) ) ;
#77274=CARTESIAN_POINT ( 'NONE',  ( -17.92363191590630223, 1419.539427151339851, 207.5409190893379900 ) ) ;
#77276=CARTESIAN_POINT ( 'NONE',  ( -2.330134126718832466, 1515.372048949687496, 204.8601094097913062 ) ) ;
#77277=CARTESIAN_POINT ( 'NONE',  ( 3.007039907259999811, 1441.535623192690082, 218.1727213951389786 ) ) ;
#77279=DIRECTION ( 'NONE',  ( -1.000000000000000000, 0.000000000000000000, 0.000000000000000000 ) ) ;
#77287=CARTESIAN_POINT ( 'NONE',  ( 7.034933902804894501, 1447.215032318710655, 203.3807619420004471 ) ) ;
#77288=CARTESIAN_POINT ( 'NONE',  ( 5.058911271898960393, 1501.257153743159961, 229.8391433438629861 ) ) ;
#77289=CARTESIAN_POINT ( 'NONE',  ( -4.221863112604749446, 1432.192955440190190, 216.4616610906159906 ) ) ;
#77291=CARTESIAN_POINT ( 'NONE',  ( -17.06449333799999835, 1423.205374796969863, 209.2384713359739976 ) ) ;
#77296=CARTESIAN_POINT ( 'NONE',  ( 11.41385934714260131, 1427.071059820410028, 208.0189296849380014 ) ) ;
#77298=CARTESIAN_POINT ( 'NONE',  ( 19.64599270300000100, 1476.662575758389949, 214.0395835971089866 ) ) ;
#77301=CARTESIAN_POINT ( 'NONE',  ( 5.204738269408170304, 1467.429567479219941, 217.6200523410610117 ) ) ;
#77303=CARTESIAN_POINT ( 'NONE',  ( 18.95676294599999778, 1454.627617991990064, 205.4346706876590076 ) ) ;
#77310=CARTESIAN_POINT ( 'NONE',  ( 4.195509702449999878, 1446.137837910890084, 200.9285957949090005 ) ) ;
#77317=CARTESIAN_POINT ( 'NONE',  ( -2.982626223070000027, 1495.726940333489893, 197.1455590585989910 ) ) ;
#77318=CARTESIAN_POINT ( 'NONE',  ( 0.07386333743999859425, 1495.692473857890036, 220.7224845649989788 ) ) ;
#77319=ORIENTED_EDGE ( 'NONE', *, *, #45529, .T. ) ;
#77321=VERTEX_POINT ( 'NONE', #82284 ) ;
#77333=CARTESIAN_POINT ( 'NONE',  ( -5.156155033729999282, 1391.908488887390149, 214.6091172688990127 ) ) ;
#77335=ORIENTED_EDGE ( 'NONE', *, *, #101724, .F. ) ;
#77337=CARTESIAN_POINT ( 'NONE',  ( -19.72124761859999964, 1465.041912645589946, 210.1751448674889673 ) ) ;
#77341=CARTESIAN_POINT ( 'NONE',  ( 9.146446762356999827, 1451.678219335869926, 210.6876116052179952 ) ) ;
#77344=CARTESIAN_POINT ( 'NONE',  ( -12.72547068037749973, 1417.199233372673916, 200.4382052065058417 ) ) ;
#77345=AXIS2_PLACEMENT_3D ( 'NONE', #45868, #4408, #105769 ) ;
#77349=CARTESIAN_POINT ( 'NONE',  ( 9.221327038241270202, 1450.741336465750237, 208.5540976675539753 ) ) ;
#77350=CARTESIAN_POINT ( 'NONE',  ( -12.48995958559999941, 1501.883328862989856, 211.6213070104490157 ) ) ;
#77363=CARTESIAN_POINT ( 'NONE',  ( -8.728492600723082973, 1490.412091298440828, 215.7830027718222823 ) ) ;
#77367=CARTESIAN_POINT ( 'NONE',  ( -8.299659899499999938, 1474.751288659789907, 202.8760590113290050 ) ) ;
#77368=CARTESIAN_POINT ( 'NONE',  ( 6.734164940669999488, 1492.669934513789940, 217.9607762184490127 ) ) ;
#77371=CARTESIAN_POINT ( 'NONE',  ( -3.753366994719999905, 1497.283149898290048, 198.4996119181990082 ) ) ;
#77374=LINE ( 'NONE', #99924, #91448 ) ;
#77380=CARTESIAN_POINT ( 'NONE',  ( -14.68341694679999954, 1416.023439710309958, 213.8223955244490071 ) ) ;
#77381=CARTESIAN_POINT ( 'NONE',  ( 0.2472019594487090133, 1515.155075545669888, 204.7947613204019888 ) ) ;
#77384=DIRECTION ( 'NONE',  ( -9.056288633775531119E-47, 1.000000000000000000, -1.836970198721029688E-16 ) ) ;
#77387=DIRECTION ( 'NONE',  ( -1.000000000000000000, -2.249639673992789970E-32, -1.224646799147350002E-16 ) ) ;
#77388=CARTESIAN_POINT ( 'NONE',  ( -2.579296836780000213, 1448.314969905590033, 190.1938323369989803 ) ) ;
#77394=CARTESIAN_POINT ( 'NONE',  ( -10.32965322753309856, 1480.667151729589932, 206.9880687129259798 ) ) ;
#77403=CARTESIAN_POINT ( 'NONE',  ( -14.89294192899999913, 1417.697066551509806, 203.6067385514490127 ) ) ;
#77406=CARTESIAN_POINT ( 'NONE',  ( -8.589426147275000645, 1436.798469860880004, 209.9038450004319998 ) ) ;
#77407=CARTESIAN_POINT ( 'NONE',  ( -7.395375191670000348, 1498.053836090689856, 218.0873371574190003 ) ) ;
#77412=CARTESIAN_POINT ( 'NONE',  ( -11.95044407570070000, 1508.551708580389914, 209.5547805494060185 ) ) ;
#77419=B_SPLINE_SURFACE_WITH_KNOTS ( 'NONE', 5, 1, ( 
 ( #47651, #73958 ),
 ( #5081, #65008 ),
 ( #48211, #82349 ),
 ( #31382, #57722 ),
 ( #6730, #65564 ),
 ( #22966, #99674 ) ),
 .UNSPECIFIED., .F., .F., .F.,
 ( 6, 6 ),
 ( 2, 2 ),
 ( 0.000000000000000000, 16.14237680569999966 ),
 ( 0.000000000000000000, 14.00000000000000000 ),
 .UNSPECIFIED. ) ;
#77423=CARTESIAN_POINT ( 'NONE',  ( 2.487935142314050108, 1509.038615934839981, 213.6090957367470082 ) ) ;
#77426=EDGE_CURVE ( 'NONE', #58087, #59861, #86144, .T. ) ;
#77428=EDGE_CURVE ( 'NONE', #5861, #63089, #104045, .T. ) ;
#77431=CARTESIAN_POINT ( 'NONE',  ( 4.533751981029999989, 1484.466359252490065, 219.6316280533989982 ) ) ;
#77436=CARTESIAN_POINT ( 'NONE',  ( 11.65726901512490166, 1435.318858471669955, 225.6545570341099847 ) ) ;
#77438=CARTESIAN_POINT ( 'NONE',  ( -5.586175246986850418, 1491.246062496780041, 185.8699218406250111 ) ) ;
#77442=CARTESIAN_POINT ( 'NONE',  ( 9.749723431585490374, 1436.068361671160119, 210.4025069022860066 ) ) ;
#77443=CARTESIAN_POINT ( 'NONE',  ( -15.06617558477470098, 1420.498972720419943, 211.7929360720449949 ) ) ;
#77444=CARTESIAN_POINT ( 'NONE',  ( 5.079734284382990239, 1447.323964650199969, 200.2742450949660054 ) ) ;
#77453=CARTESIAN_POINT ( 'NONE',  ( -0.7790226144181949808, 1442.687261678630193, 200.2740145696140246 ) ) ;
#77456=ORIENTED_EDGE ( 'NONE', *, *, #87774, .F. ) ;
#77459=ORIENTED_EDGE ( 'NONE', *, *, #27407, .T. ) ;
#77461=CARTESIAN_POINT ( 'NONE',  ( -10.36637489306960092, 1448.036064164660047, 209.0396054626149862 ) ) ;
#77462=CARTESIAN_POINT ( 'NONE',  ( 2.956826570602010040, 1515.222544082249897, 204.7977243905010027 ) ) ;
#77479=ORIENTED_EDGE ( 'NONE', *, *, #60374, .T. ) ;
#77480=ADVANCED_FACE ( 'NONE', ( #61523 ), #95577, .T. ) ;
#77481=VERTEX_POINT ( 'NONE', #79412 ) ;
#77484=CARTESIAN_POINT ( 'NONE',  ( -12.75668250589355068, 1503.496714303483031, 208.6968331601771069 ) ) ;
#77495=CARTESIAN_POINT ( 'NONE',  ( 2.409034624560000282, 1511.999350511789999, 206.7128113371389873 ) ) ;
#77502=CARTESIAN_POINT ( 'NONE',  ( -16.94284628566209960, 1508.551704408389924, 210.3926682970049740 ) ) ;
#77503=CARTESIAN_POINT ( 'NONE',  ( -12.02051106306990036, 1491.153688555679992, 206.6632162730240054 ) ) ;
#77507=B_SPLINE_CURVE_WITH_KNOTS ( 'NONE', 5,
 ( #86384, #10798, #86938, #19732, #88067, #45525 ),
 .UNSPECIFIED., .F., .F.,
 ( 6, 6 ),
 ( -2.000000000000000000, 0.000000000000000000 ),
 .UNSPECIFIED. ) ;
#77508=CARTESIAN_POINT ( 'NONE',  ( -2.678371528919849975, 1429.099047671080143, 200.1418393138040130 ) ) ;
#77520=CARTESIAN_POINT ( 'NONE',  ( 10.90828758974610047, 1490.545376044769910, 210.3161421217920122 ) ) ;
#77527=CARTESIAN_POINT ( 'NONE',  ( -9.203111897236890826, 1450.336789552200116, 208.5678280199140033 ) ) ;
#77531=CARTESIAN_POINT ( 'NONE',  ( -8.056653238513129978, 1508.431094367349942, 219.4233643241270215 ) ) ;
#77532=CARTESIAN_POINT ( 'NONE',  ( 4.858360387713474893, 1508.551704413348716, 211.6097810847319920 ) ) ;
#77543=CARTESIAN_POINT ( 'NONE',  ( 10.63508560284700089, 1480.849370521759965, 210.2894055373469939 ) ) ;
#77545=CARTESIAN_POINT ( 'NONE',  ( -4.954768278013866656, 1446.481062136786022, 216.7370039512331914 ) ) ;
#77546=EDGE_LOOP ( 'NONE', ( #72608, #81176, #32969, #107881 ) ) ;
#77549=CARTESIAN_POINT ( 'NONE',  ( 4.124008068921309444, 1455.961819920020162, 218.9107260925210028 ) ) ;
#77551=CARTESIAN_POINT ( 'NONE',  ( 0.9642394209830019713, 1486.365851861090050, 197.2124130950990093 ) ) ;
#77554=CARTESIAN_POINT ( 'NONE',  ( 11.87587340029999972, 1501.155101168290003, 209.4695087910589848 ) ) ;
#77561=CARTESIAN_POINT ( 'NONE',  ( -8.114589821750000098, 1483.072352354889972, 201.8754299783889792 ) ) ;
#77568=CARTESIAN_POINT ( 'NONE',  ( 3.035119290295853034, 1377.913060387289988, 207.4637527364374705 ) ) ;
#77573=CARTESIAN_POINT ( 'NONE',  ( 1.520272259658780101, 1456.597953077289958, 219.6336397091319839 ) ) ;
#77576=CARTESIAN_POINT ( 'NONE',  ( 7.230170464569999567, 1423.528413094569942, 213.4846319112089930 ) ) ;
#77577=CARTESIAN_POINT ( 'NONE',  ( -2.775555821850000271, 1468.867611631090085, 187.4507004057990116 ) ) ;
#77581=EDGE_CURVE ( 'NONE', #9164, #92866, #93955, .T. ) ;
#77584=VERTEX_POINT ( 'NONE', #50641 ) ;
#77589=CARTESIAN_POINT ( 'NONE',  ( 7.712506219943952246, 1500.328028434782254, 200.7279699965547763 ) ) ;
#77592=CARTESIAN_POINT ( 'NONE',  ( -1.658825910028130179, 1475.382055513630121, 197.7986645737999822 ) ) ;
#77599=EDGE_LOOP ( 'NONE', ( #56717, #34598, #103930 ) ) ;
#77620=ORIENTED_EDGE ( 'NONE', *, *, #35393, .F. ) ;
#77633=PLANE ( 'NONE',  #93817 ) ;
#77638=CARTESIAN_POINT ( 'NONE',  ( -3.464428872329999631, 1429.082167021389978, 201.1863187793390182 ) ) ;
#77644=CARTESIAN_POINT ( 'NONE',  ( 1.599187595592249878, 1431.274712152729990, 218.4776966100959896 ) ) ;
#77658=CARTESIAN_POINT ( 'NONE',  ( 3.039942922830000338, 1441.350710123290128, 218.5632362648489959 ) ) ;
#77665=CARTESIAN_POINT ( 'NONE',  ( -9277.894383878754525, -2339.359351152912041, 136.3368685514004710 ) ) ;
#77667=CARTESIAN_POINT ( 'NONE',  ( -9.417893745694790653, 1420.662742013269963, 195.0156044709679861 ) ) ;
#77668=CARTESIAN_POINT ( 'NONE',  ( -5.216843437400244810, 1391.913060387290216, 203.7324240256280916 ) ) ;
#77672=FACE_OUTER_BOUND ( 'NONE', #41180, .T. ) ;
#77680=CARTESIAN_POINT ( 'NONE',  ( 11.27337966920289958, 1433.557911275300057, 225.8166862488670006 ) ) ;
#77685=CARTESIAN_POINT ( 'NONE',  ( 10.55224117611160217, 1452.267020623229882, 208.7256732491289881 ) ) ;
#77692=VERTEX_POINT ( 'NONE', #109448 ) ;
#77694=B_SPLINE_CURVE_WITH_KNOTS ( 'NONE', 3,
 ( #82496, #48356, #4684, #90326, #73563, #5798, #106589, #65705, #89240, #107696, #80845, #56749, #30980, #99826, #47793, #12535, #38276, #90886, #38823, #29875 ),
 .UNSPECIFIED., .F., .F.,
 ( 4, 2, 2, 2, 1, 1, 1, 1, 2, 2, 2, 4 ),
 ( 0.000000000000000000, 0.2500000000009953149, 0.3750000000014879764, 0.4375000000017343904, 0.4687500000018708368, 0.4843750000019390045, 0.4921875000019731439, 0.4960937500019942381, 0.4980468750019917956, 0.5000000000019892976, 0.7500000000009947598, 1.000000000000000000 ),
 .UNSPECIFIED. ) ;
#77701=CARTESIAN_POINT ( 'NONE',  ( 9.377531398314840061, 1435.528482238679999, 208.6857172028140042 ) ) ;
#77703=EDGE_CURVE ( 'NONE', #88887, #87290, #7100, .T. ) ;
#77710=CARTESIAN_POINT ( 'NONE',  ( -14.89996083112460035, 1421.394563697389913, 203.5315014676550049 ) ) ;
#77715=ORIENTED_EDGE ( 'NONE', *, *, #34447, .F. ) ;
#77716=CARTESIAN_POINT ( 'NONE',  ( -4.565395397388770427, 1480.772680885790123, 231.0139838447539944 ) ) ;
#77719=CARTESIAN_POINT ( 'NONE',  ( -18.75679884100000194, 1468.090218040589889, 202.1898047414589996 ) ) ;
#77721=CARTESIAN_POINT ( 'NONE',  ( -20.22132488579999787, 1484.073267153790084, 213.0491124005889958 ) ) ;
#77722=CARTESIAN_POINT ( 'NONE',  ( -1.920602012799999869, 1420.567466289690174, 193.8392733480989989 ) ) ;
#77730=CARTESIAN_POINT ( 'NONE',  ( -9.215151402819998339, 1422.993424535609847, 210.2744618676390189 ) ) ;
#77735=CARTESIAN_POINT ( 'NONE',  ( 7.537620219123420284, 1425.580748762979965, 212.1821311706370068 ) ) ;
#77743=B_SPLINE_CURVE_WITH_KNOTS ( 'NONE', 3,
 ( #82661, #40097, #49620, #83753, #41207, #77573, #52932, #9264, #85390, #35553, #78110, #86509, #69748, #27167, #1412, #77026, #60225, #17621, #69183, #332, #103289, #26596, #94343, #60793, #34458, #43970, #87066, #70307, #95471, #27713, #78670, #68634, #51825, #42867, #103867, #43423, #102735 ),
 .UNSPECIFIED., .F., .F.,
 ( 4, 3, 3, 3, 3, 3, 3, 3, 3, 3, 3, 3, 4 ),
 ( -12.69765133870000007, -12.53569613955949968, -11.85572679381469996, -11.13826790116400112, -10.38487189775069908, -9.582453197718731275, -8.635551395450828949, -7.667863743602329585, -6.997493992233709825, -6.072779624993440706, -5.268273530587539000, -4.554978577956211083, -3.881604426910000072 ),
 .UNSPECIFIED. ) ;
#77745=CARTESIAN_POINT ( 'NONE',  ( -18.23402007437789862, 1508.542070153930126, 211.0639760601119974 ) ) ;
#77752=CARTESIAN_POINT ( 'NONE',  ( 9.327571024978329461, 1434.415488575019936, 206.2241823136789947 ) ) ;
#77773=CARTESIAN_POINT ( 'NONE',  ( -4.692464771771249765, 1508.551704408389924, 212.7861425959310111 ) ) ;
#77775=CARTESIAN_POINT ( 'NONE',  ( 7.443246446249998982, 1423.092341332720025, 195.6161848952989999 ) ) ;
#77777=B_SPLINE_SURFACE_WITH_KNOTS ( 'NONE', 5, 1, ( 
 ( #103000, #86770 ),
 ( #10626, #52082 ),
 ( #2797, #37475 ),
 ( #2253, #44793 ),
 ( #10060, #28524 ),
 ( #44233, #78945 ),
 ( #36365, #36917 ),
 ( #45894, #9506 ),
 ( #80030, #26297 ),
 ( #94607, #17883 ),
 ( #86213, #88971 ),
 ( #81657, #54846 ),
 ( #82222, #107974 ),
 ( #20644, #72740 ),
 ( #80583, #5524 ),
 ( #12815, #72207 ),
 ( #106866, #39680 ),
 ( #73847, #64349 ),
 ( #106330, #4963 ),
 ( #46995, #98470 ),
 ( #13900, #47536 ),
 ( #21740, #55942 ),
 ( #63798, #4435 ),
 ( #90063, #13344 ),
 ( #39107, #97912 ),
 ( #22288, #73284 ),
 ( #30157, #29613 ),
 ( #38561, #21184 ),
 ( #107421, #30718 ),
 ( #56489, #55393 ),
 ( #64903, #90620 ),
 ( #71679, #81118 ),
 ( #3899, #48087 ),
 ( #63263, #99011 ),
 ( #12261, #105798 ),
 ( #89523, #29079 ),
 ( #97373, #46451 ),
 ( #38028, #52997 ),
 ( #52446, #79295 ),
 ( #97181, #70926 ),
 ( #86574, #103928 ),
 ( #12074, #36731 ),
 ( #37290, #28886 ),
 ( #70366, #78735 ),
 ( #105042, #105603 ),
 ( #87701, #9867 ),
 ( #54115, #72025 ),
 ( #28331, #61965 ),
 ( #1483, #106141 ),
 ( #2050, #62523 ),
 ( #35615, #71482 ) ),
 .UNSPECIFIED., .F., .F., .F.,
 ( 6, 3, 3, 3, 3, 3, 3, 3, 3, 3, 3, 3, 3, 3, 3, 3, 6 ),
 ( 2, 2 ),
 ( 0.000000000000000000, 28.69702819429999963, 61.04778752440000034, 93.62768910810000023, 123.7336603250000024, 156.1762685979999787, 187.3272846180000215, 220.4669312460000015, 237.3878297990000021, 254.2938300590000154, 289.2398204710000300, 325.3030936050000150, 360.8626869010000178, 395.8828220460000011, 432.6128460950000090, 468.8934854820000169, 502.1482307969999965 ),
 ( -0.0001548847310923010001, 2.001786307029170153 ),
 .UNSPECIFIED. ) ;
#77793=CARTESIAN_POINT ( 'NONE',  ( 1.381433737519002669, 1421.416365592073362, 193.7767222259685411 ) ) ;
#77800=B_SPLINE_SURFACE_WITH_KNOTS ( 'NONE', 5, 5, ( 
 ( #49685, #107913, #23890, #65391, #66502, #39041 ),
 ( #13284, #14940, #41269, #65940, #74344, #40714 ),
 ( #56427, #14391, #99496, #92216, #101149, #81598 ),
 ( #75443, #98955, #22778, #47475, #73222, #67041 ),
 ( #56984, #107365, #90557, #48585, #57542, #13837 ),
 ( #49135, #109579, #82719, #6009, #30661, #58083 ),
 ( #91665, #64846, #31755, #83268, #32319, #6564 ),
 ( #74886, #100607, #103926, #85449, #68154, #86572 ),
 ( #27225, #51313, #42930, #110122, #9864, #92762 ) ),
 .UNSPECIFIED., .F., .F., .F.,
 ( 6, 3, 6 ),
 ( 6, 6 ),
 ( -0.0002510112223089640293, 10.92808819610000093, 17.46068133292229874 ),
 ( -0.0002510112223103900262, 2.000000000000000000 ),
 .UNSPECIFIED. ) ;
#77801=CARTESIAN_POINT ( 'NONE',  ( -10.16625295280419827, 1461.954337890570059, 208.9248117568549787 ) ) ;
#77802=CARTESIAN_POINT ( 'NONE',  ( 2.502367656480000147, 1427.111872751849887, 188.6975817531990174 ) ) ;
#77803=CARTESIAN_POINT ( 'NONE',  ( -1.842962231260000028, 1515.551704408389924, 212.9514660752490158 ) ) ;
#77813=CARTESIAN_POINT ( 'NONE',  ( 0.9103411385305409942, 1462.760009460389938, 230.5111369873399951 ) ) ;
#77815=CARTESIAN_POINT ( 'NONE',  ( -15.23895844625580054, 1421.038471381979889, 204.9739905745400108 ) ) ;
#77817=CARTESIAN_POINT ( 'NONE',  ( 3.368607595359999873, 1442.498527986489989, 217.3357187138090296 ) ) ;
#77822=CARTESIAN_POINT ( 'NONE',  ( -4.647810563630000225, 1474.919191006789788, 199.5028939205090239 ) ) ;
#77824=VERTEX_POINT ( 'NONE', #70794 ) ;
#77825=CARTESIAN_POINT ( 'NONE',  ( -5.842433632679150612, 1508.551704408389924, 219.4797894617979921 ) ) ;
#77826=VERTEX_POINT ( 'NONE', #62381 ) ;
#77830=CARTESIAN_POINT ( 'NONE',  ( 2.516232163441119773, 1464.674062513380022, 202.5523638050540001 ) ) ;
#77833=CARTESIAN_POINT ( 'NONE',  ( 1.875671004969999833, 1456.514200624189925, 219.5762891113990065 ) ) ;
#77841=CARTESIAN_POINT ( 'NONE',  ( -1.420557929969340050, 1438.189677974030019, 227.6394655603620265 ) ) ;
#77846=FACE_OUTER_BOUND ( 'NONE', #37673, .T. ) ;
#77848=CARTESIAN_POINT ( 'NONE',  ( -6.797648946129999814, 1495.115797578489946, 200.0173552654389937 ) ) ;
#77854=CARTESIAN_POINT ( 'NONE',  ( -8.437512126890000630, 1512.337580101790081, 211.2823750686789879 ) ) ;
#77861=CARTESIAN_POINT ( 'NONE',  ( 0.5197867694969990904, 1494.713114127890094, 220.2910688317990093 ) ) ;
#77864=VERTEX_POINT ( 'NONE', #86992 ) ;
#77877=CARTESIAN_POINT ( 'NONE',  ( -5.166418613160000284, 1391.906183525989718, 214.5657459001290022 ) ) ;
#77879=ORIENTED_EDGE ( 'NONE', *, *, #94808, .T. ) ;
#77881=CARTESIAN_POINT ( 'NONE',  ( 10.32735688926459794, 1460.628046964450050, 207.2416929514699859 ) ) ;
#77886=CARTESIAN_POINT ( 'NONE',  ( 9.651067907589998995, 1425.440654964710120, 195.4941613134990064 ) ) ;
#77889=CARTESIAN_POINT ( 'NONE',  ( -12.45534669159577135, 1417.321673587058740, 200.0573570912646915 ) ) ;
#77894=CARTESIAN_POINT ( 'NONE',  ( 9.209674294604401013, 1450.304425456110039, 208.7276454369840053 ) ) ;
#77895=CARTESIAN_POINT ( 'NONE',  ( 4.082704913390428736, 1515.071394844000451, 212.7082235457387185 ) ) ;
#77897=EDGE_LOOP ( 'NONE', ( #3310, #23028, #23414, #95482 ) ) ;
#77900=ORIENTED_EDGE ( 'NONE', *, *, #60243, .F. ) ;
#77903=VERTEX_POINT ( 'NONE', #27102 ) ;
#77905=CARTESIAN_POINT ( 'NONE',  ( -3.700607310100329617, 1508.505817376630148, 220.3043853933179719 ) ) ;
#77908=CARTESIAN_POINT ( 'NONE',  ( -11.03352987879990010, 1462.446752253709974, 208.7216463217210105 ) ) ;
#77913=CARTESIAN_POINT ( 'NONE',  ( 10.44002158900000055, 1492.834359288489850, 214.0636917351490069 ) ) ;
#77915=CARTESIAN_POINT ( 'NONE',  ( -21.25276517840000068, 1505.388537598189941, 209.6001788282910070 ) ) ;
#77924=CARTESIAN_POINT ( 'NONE',  ( -14.52535627939999863, 1415.865102022439942, 214.1001117942190035 ) ) ;
#77925=CARTESIAN_POINT ( 'NONE',  ( -0.3731951686936089696, 1515.150224411150020, 204.7946342890899984 ) ) ;
#77926=ORIENTED_EDGE ( 'NONE', *, *, #24163, .F. ) ;
#77930=CARTESIAN_POINT ( 'NONE',  ( 20.13562578519999846, 1473.995721266390092, 210.1107519762580012 ) ) ;
#77931=CARTESIAN_POINT ( 'NONE',  ( 3.263471513352690145, 1446.335603773660068, 199.5325906368949802 ) ) ;
#77932=CARTESIAN_POINT ( 'NONE',  ( -4.992640509747255706, 1391.632012793324975, 203.6213856293937283 ) ) ;
#77936=CARTESIAN_POINT ( 'NONE',  ( -11.86476110198860034, 1482.098049815899913, 208.3139255992990115 ) ) ;
#77947=CARTESIAN_POINT ( 'NONE',  ( 5.699301886687036856, 1480.231621539390062, 228.7443292491632860 ) ) ;
#77955=VERTEX_POINT ( 'NONE', #70244 ) ;
#77958=CARTESIAN_POINT ( 'NONE',  ( 10.57600485288619829, 1481.555237149170125, 209.3766040892330125 ) ) ;
#77960=CARTESIAN_POINT ( 'NONE',  ( -5.851400963819999745, 1449.323580990290111, 210.4453412175489859 ) ) ;
#77970=CARTESIAN_POINT ( 'NONE',  ( 4.325231544520000249, 1515.225845272990000, 208.0336405044189974 ) ) ;
#77975=CARTESIAN_POINT ( 'NONE',  ( 4.486170154879999927, 1485.164793332289946, 219.0208057013190057 ) ) ;
#77978=CARTESIAN_POINT ( 'NONE',  ( 7.979825105375810246, 1460.922446521970187, 228.8885227319260025 ) ) ;
#77980=CARTESIAN_POINT ( 'NONE',  ( -21.47380247972409961, 1487.892794807240080, 202.0847358610229776 ) ) ;
#77984=CARTESIAN_POINT ( 'NONE',  ( -4.994804046730000557, 1391.714634656189901, 203.6484225187790287 ) ) ;
#77985=CARTESIAN_POINT ( 'NONE',  ( 9.777811368307929740, 1435.956396579579859, 210.1555867559330295 ) ) ;
#77986=CARTESIAN_POINT ( 'NONE',  ( -11.07998396640000038, 1490.998932559390141, 210.3063338810989933 ) ) ;
#77987=CARTESIAN_POINT ( 'NONE',  ( 10.01154216381359952, 1451.059416430699912, 206.0422016317240264 ) ) ;
#77994=CARTESIAN_POINT ( 'NONE',  ( 8.040667369584340918, 1505.155755465120137, 217.5954850267839902 ) ) ;
#77995=CARTESIAN_POINT ( 'NONE',  ( -11.60674135321730027, 1507.508082919659955, 207.5537295141489835 ) ) ;
#77998=ORIENTED_EDGE ( 'NONE', *, *, #63669, .F. ) ;
#78006=CARTESIAN_POINT ( 'NONE',  ( -21.59687142900000012, 1507.523380033690046, 209.4572543540780032 ) ) ;
#78009=DIRECTION ( 'NONE',  ( 0.2843490923843689511, 0.3717034639898259551, 0.8837319324988487379 ) ) ;
#78012=CARTESIAN_POINT ( 'NONE',  ( -13.40911912816510032, 1421.283099727030049, 209.4572124756780056 ) ) ;
#78017=ORIENTED_EDGE ( 'NONE', *, *, #91494, .T. ) ;
#78024=CARTESIAN_POINT ( 'NONE',  ( 10.51154376439999893, 1461.171203229189814, 208.7546265782200123 ) ) ;
#78028=CARTESIAN_POINT ( 'NONE',  ( 8.641620394141629191, 1437.949431946680079, 209.8872740218120043 ) ) ;
#78034=ORIENTED_EDGE ( 'NONE', *, *, #2138, .T. ) ;
#78038=CARTESIAN_POINT ( 'NONE',  ( 3.185905804640090100, 1423.706610472649800, 192.7960985019370241 ) ) ;
#78042=CARTESIAN_POINT ( 'NONE',  ( 4.492546581380000958, 1453.878649273890005, 217.3453973181289882 ) ) ;
#78046=CARTESIAN_POINT ( 'NONE',  ( -2.505509636816239727, 1429.193828627990115, 200.0902972570239911 ) ) ;
#78050=EDGE_CURVE ( 'NONE', #52413, #22689, #19109, .T. ) ;
#78061=DIRECTION ( 'NONE',  ( 6.505213034913001952E-16, 0.02617694830786544691, -0.9996573249755575929 ) ) ;
#78070=VERTEX_POINT ( 'NONE', #15222 ) ;
#78076=EDGE_CURVE ( 'NONE', #59861, #10365, #51612, .T. ) ;
#78077=CARTESIAN_POINT ( 'NONE',  ( 3.618068937029999876, 1466.495810770989920, 219.1439048061990036 ) ) ;
#78083=CARTESIAN_POINT ( 'NONE',  ( 10.82177570574990000, 1480.619340521260028, 210.9524986334820085 ) ) ;
#78084=FACE_OUTER_BOUND ( 'NONE', #64125, .T. ) ;
#78085=EDGE_CURVE ( 'NONE', #36047, #73608, #108638, .T. ) ;
#78086=CARTESIAN_POINT ( 'NONE',  ( -6.265666849954051543, 1447.085106900710343, 215.7369580074560815 ) ) ;
#78094=CARTESIAN_POINT ( 'NONE',  ( 11.32069328670000097, 1502.651227823090039, 211.1497760302390247 ) ) ;
#78095=CARTESIAN_POINT ( 'NONE',  ( 8.289978012700000676, 1427.452913477950005, 211.9970543031389809 ) ) ;
#78107=VERTEX_POINT ( 'NONE', #23641 ) ;
#78108=CARTESIAN_POINT ( 'NONE',  ( -14.93566798913168903, 1416.108416094674567, 205.2278682516571280 ) ) ;
#78109=CARTESIAN_POINT ( 'NONE',  ( 1.538503540740000286, 1455.675331449789837, 218.5739177642490176 ) ) ;
#78110=CARTESIAN_POINT ( 'NONE',  ( 0.8264992237066920433, 1456.771628818370118, 219.7120364133879775 ) ) ;
#78114=CARTESIAN_POINT ( 'NONE',  ( 7.478662903260000050, 1425.010047449799913, 212.2620327022589777 ) ) ;
#78115=CARTESIAN_POINT ( 'NONE',  ( -17.51543818720000090, 1417.552356044260023, 206.7803260803289902 ) ) ;
#78119=CARTESIAN_POINT ( 'NONE',  ( 6.749186742440000053, 1455.205488045889979, 217.3783194977189908 ) ) ;
#78125=CARTESIAN_POINT ( 'NONE',  ( 7.522275854169816256, 1500.273529863827207, 200.5607867249156868 ) ) ;
#78128=LINE ( 'NONE', #61370, #67572 ) ;
#78143=CARTESIAN_POINT ( 'NONE',  ( -3.943364034450000499, 1453.941432717190082, 199.4131967690690033 ) ) ;
#78149=ORIENTED_EDGE ( 'NONE', *, *, #91698, .F. ) ;
#78153=ADVANCED_FACE ( 'NONE', ( #24715 ), #33021, .T. ) ;
#78170=CARTESIAN_POINT ( 'NONE',  ( 20.49831092009999978, 1496.178973653789853, 204.1013708937389879 ) ) ;
#78175=CARTESIAN_POINT ( 'NONE',  ( 0.000000000000000000, 1420.584111001019892, 209.1218459616989946 ) ) ;
#78179=EDGE_CURVE ( 'NONE', #35149, #8260, #41798, .T. ) ;
#78180=ORIENTED_EDGE ( 'NONE', *, *, #27154, .T. ) ;
#78182=FACE_OUTER_BOUND ( 'NONE', #66922, .T. ) ;
#78202=UNCERTAINTY_MEASURE_WITH_UNIT (LENGTH_MEASURE( 1.000000000000000082E-05 ), #35457, 'distance_accuracy_value', 'NONE');
#78203=CARTESIAN_POINT ( 'NONE',  ( 4.123426501090060370, 1424.433584402349879, 191.6254363278619905 ) ) ;
#78205=CARTESIAN_POINT ( 'NONE',  ( -740.1067050525047080, 11216.44053380569312, -1627.040744445698465 ) ) ;
#78208=CARTESIAN_POINT ( 'NONE',  ( 9.142604584464409712, 1459.538234665719983, 203.9517274866290109 ) ) ;
#78211=CARTESIAN_POINT ( 'NONE',  ( 11.72865777870000059, 1490.920838208090117, 205.3345067772989978 ) ) ;
#78212=CARTESIAN_POINT ( 'NONE',  ( -5.050863578716279001, 1391.819074324308986, 203.5808726994333426 ) ) ;
#78214=EDGE_LOOP ( 'NONE', ( #52843, #27325, #97704, #42387 ) ) ;
#78216=CARTESIAN_POINT ( 'NONE',  ( -4.987082680427599612, 1508.551704408389924, 212.3948994024580088 ) ) ;
#78224=CARTESIAN_POINT ( 'NONE',  ( -11.00840296587000111, 1470.178642279830001, 211.9751469970929918 ) ) ;
#78225=CARTESIAN_POINT ( 'NONE',  ( -2.298652125478059638, 1486.462338610419920, 220.8290092987670050 ) ) ;
#78229=CARTESIAN_POINT ( 'NONE',  ( -5.085463042024069402, 1391.851494597096007, 214.6322330144460864 ) ) ;
#78231=CARTESIAN_POINT ( 'NONE',  ( 10.56298886728909991, 1452.344034128999965, 208.9192460544000198 ) ) ;
#78232=ORIENTED_EDGE ( 'NONE', *, *, #40406, .F. ) ;
#78243=CARTESIAN_POINT ( 'NONE',  ( 8.736406163737710173, 1436.941576091229763, 209.9790183900369982 ) ) ;
#78251=CARTESIAN_POINT ( 'NONE',  ( 8.909955910623979847, 1434.607648340320111, 206.3240839377490090 ) ) ;
#78252=CARTESIAN_POINT ( 'NONE',  ( -15.68969716385069901, 1421.005191948239826, 203.3991960173040070 ) ) ;
#78257=CARTESIAN_POINT ( 'NONE',  ( -11.53818992870000137, 1506.400027429489910, 207.4085574012289896 ) ) ;
#78258=CARTESIAN_POINT ( 'NONE',  ( 22.28449968809999859, 1476.748388319289916, 209.6248863100890105 ) ) ;
#78275=ADVANCED_FACE ( 'NONE', ( #22931 ), #69269, .F. ) ;
#78280=CARTESIAN_POINT ( 'NONE',  ( 1.879472310086659936, 1495.752734514360100, 221.3175895178520136 ) ) ;
#78283=CARTESIAN_POINT ( 'NONE',  ( 5.268140179660000477, 1505.035622830590000, 220.7476737412989962 ) ) ;
#78288=CARTESIAN_POINT ( 'NONE',  ( -1.876581345759999797, 1456.020558252990213, 215.5707636483290059 ) ) ;
#78289=CARTESIAN_POINT ( 'NONE',  ( -8.305912316622009683, 1438.481564584539910, 206.5261465373520195 ) ) ;
#78307=B_SPLINE_CURVE_WITH_KNOTS ( 'NONE', 5,
 ( #18647, #77484, #85870, #60701, #25942, #52296 ),
 .UNSPECIFIED., .F., .F.,
 ( 6, 6 ),
 ( 0.000000000000000000, 1.000000000000000000 ),
 .UNSPECIFIED. ) ;
#78311=VERTEX_POINT ( 'NONE', #106957 ) ;
#78312=CARTESIAN_POINT ( 'NONE',  ( -0.3646785421350010048, 1445.165625539289977, 215.3775912058289919 ) ) ;
#78315=ORIENTED_EDGE ( 'NONE', *, *, #41387, .T. ) ;
#78321=EDGE_CURVE ( 'NONE', #83093, #508, #92563, .T. ) ;
#78322=B_SPLINE_CURVE_WITH_KNOTS ( 'NONE', 5,
 ( #87813, #12180, #97291, #45815, #46371, #9977, #78283, #103850, #102715 ),
 .UNSPECIFIED., .F., .F.,
 ( 6, 3, 6 ),
 ( -3.420211715829999832, -1.710105857910000138, 0.000000000000000000 ),
 .UNSPECIFIED. ) ;
#78323=DIRECTION ( 'NONE',  ( -1.224646799147350002E-16, 1.836970198721029688E-16, 1.000000000000000000 ) ) ;
#78325=CARTESIAN_POINT ( 'NONE',  ( -3.874459836649999822, 1495.423322680889896, 197.4164389294989803 ) ) ;
#78329=AXIS2_PLACEMENT_3D ( 'NONE', #14592, #22415, #65020 ) ;
#78334=CIRCLE ( 'NONE', #33622, 2.458500000000000352 ) ;
#78338=CARTESIAN_POINT ( 'NONE',  ( -17.14339296960000070, 1417.642190471430013, 207.4869690162090023 ) ) ;
#78344=CARTESIAN_POINT ( 'NONE',  ( -19.09790268268400126, 1508.458003811930212, 210.0050661408479868 ) ) ;
#78346=CARTESIAN_POINT ( 'NONE',  ( -4.328991615394409465, 1515.082251143310032, 207.7602669075220092 ) ) ;
#78352=CARTESIAN_POINT ( 'NONE',  ( -14.34085026152870057, 1421.948958043559969, 196.2628561903719913 ) ) ;
#78353=ADVANCED_FACE ( 'NONE', ( #78182 ), #108077, .T. ) ;
#78354=DIRECTION ( 'NONE',  ( -9.152776640618289361E-47, 1.000000000000000000, -1.836970198721029688E-16 ) ) ;
#78355=CARTESIAN_POINT ( 'NONE',  ( 10.22342693278199910, 1462.397256940530042, 211.7726961121359750 ) ) ;
#78361=CARTESIAN_POINT ( 'NONE',  ( -17.59976141832330043, 1419.797097700060021, 206.6695233765389901 ) ) ;
#78364=CARTESIAN_POINT ( 'NONE',  ( 16.66442746070229930, 1492.498864031070070, 193.3249227824980210 ) ) ;
#78365=EDGE_CURVE ( 'NONE', #69308, #91119, #81856, .T. ) ;
#78376=ORIENTED_EDGE ( 'NONE', *, *, #1758, .F. ) ;
#78377=CARTESIAN_POINT ( 'NONE',  ( -5.593318843000940177, 1508.551704408389924, 219.5394102594769947 ) ) ;
#78384=CARTESIAN_POINT ( 'NONE',  ( 0.2700213805099990205, 1431.728054808090064, 218.6309394840390041 ) ) ;
#78390=CARTESIAN_POINT ( 'NONE',  ( 9.799815244658731217, 1423.431771991869937, 209.4823171178350094 ) ) ;
#78392=CARTESIAN_POINT ( 'NONE',  ( 10.81586312699060137, 1489.669647427700056, 207.5188354526409853 ) ) ;
#78397=CARTESIAN_POINT ( 'NONE',  ( 6.039844978529999686, 1450.200509822089998, 208.6657062937080127 ) ) ;
#78402=FACE_OUTER_BOUND ( 'NONE', #77546, .T. ) ;
#78415=CARTESIAN_POINT ( 'NONE',  ( -2.719997508650000118, 1496.976443727390006, 221.2163582191989804 ) ) ;
#78419=VECTOR ( 'NONE', #88128, 1000.000000000000227 ) ;
#78430=CARTESIAN_POINT ( 'NONE',  ( 4.475991544341880513, 1508.551704408389924, 213.1231739162390113 ) ) ;
#78434=CARTESIAN_POINT ( 'NONE',  ( 9.301629471904078628, 1462.018477543640074, 206.2660014330650142 ) ) ;
#78440=EDGE_LOOP ( 'NONE', ( #82127, #101152, #48575, #100668, #100813 ) ) ;
#78447=CARTESIAN_POINT ( 'NONE',  ( 9.721563988697850434, 1451.950384167230141, 209.1155634365840115 ) ) ;
#78448=CARTESIAN_POINT ( 'NONE',  ( 19.41157449629999832, 1457.417846740989944, 209.1218459616989946 ) ) ;
#78453=ORIENTED_EDGE ( 'NONE', *, *, #77428, .T. ) ;
#78460=CARTESIAN_POINT ( 'NONE',  ( -4.835422890569469168, 1508.443244997879901, 220.2371915919370053 ) ) ;
#78467=CARTESIAN_POINT ( 'NONE',  ( 11.24566101859999812, 1493.273975466890079, 214.3640310562390141 ) ) ;
#78470=CARTESIAN_POINT ( 'NONE',  ( -20.22175671919999829, 1505.497798682489929, 209.1006163569459773 ) ) ;
#78471=CARTESIAN_POINT ( 'NONE',  ( 10.49331861557109846, 1469.560031205900032, 204.9147316216790102 ) ) ;
#78473=CARTESIAN_POINT ( 'NONE',  ( -9.963890954553210833, 1439.503587905810036, 208.3753853002669985 ) ) ;
#78475=ORIENTED_EDGE ( 'NONE', *, *, #50763, .F. ) ;
#78480=CARTESIAN_POINT ( 'NONE',  ( 5.246441130820000076, 1506.817910960390009, 219.5624344324990034 ) ) ;
#78482=CARTESIAN_POINT ( 'NONE',  ( -0.1783569643517119996, 1515.156623775960043, 204.7948018622450093 ) ) ;
#78483=ORIENTED_EDGE ( 'NONE', *, *, #96543, .T. ) ;
#78484=CARTESIAN_POINT ( 'NONE',  ( -15.62663836450985855, 1415.708812752953463, 209.6394265537848582 ) ) ;
#78485=CARTESIAN_POINT ( 'NONE',  ( 11.26937486967429969, 1478.652699849539886, 205.8601904136019982 ) ) ;
#78486=CARTESIAN_POINT ( 'NONE',  ( -16.22969151800000276, 1416.527220236440144, 208.6990027614089911 ) ) ;
#78494=CARTESIAN_POINT ( 'NONE',  ( -11.29380069599010028, 1482.268690959019978, 207.2091524315400193 ) ) ;
#78508=CARTESIAN_POINT ( 'NONE',  ( 7.629404627771598335, 1479.880594065073410, 228.0747595323517771 ) ) ;
#78519=CARTESIAN_POINT ( 'NONE',  ( -13.23573713899709858, 1508.551704408300111, 210.3365014446919758 ) ) ;
#78522=CARTESIAN_POINT ( 'NONE',  ( -11.82810778686869924, 1481.586904978749999, 209.9993492298939941 ) ) ;
#78532=CARTESIAN_POINT ( 'NONE',  ( 4.261736558349999981, 1515.372048625790057, 207.2788822659889831 ) ) ;
#78536=CARTESIAN_POINT ( 'NONE',  ( 3.476014316090000111, 1485.192983848789936, 219.6841126116989926 ) ) ;
#78537=CARTESIAN_POINT ( 'NONE',  ( 3.825556360259999789, 1423.414717582890034, 193.7421645440990119 ) ) ;
#78539=CARTESIAN_POINT ( 'NONE',  ( 20.83586984089999916, 1457.604279698989785, 206.7633391697789875 ) ) ;
#78541=CARTESIAN_POINT ( 'NONE',  ( 24.04367183766050076, 1494.655699982339911, 207.1743773502899728 ) ) ;
#78544=CARTESIAN_POINT ( 'NONE',  ( -5.236048287610000074, 1391.923671795290147, 203.6379494214189947 ) ) ;
#78545=CARTESIAN_POINT ( 'NONE',  ( 9.817701725550250558, 1435.668645397809996, 209.4942759991459980 ) ) ;
#78546=CARTESIAN_POINT ( 'NONE',  ( -15.46160582433359920, 1420.394257567060095, 210.8293740474650235 ) ) ;
#78551=CARTESIAN_POINT ( 'NONE',  ( 10.46238070710109902, 1503.718831861420085, 214.1759217846949923 ) ) ;
#78562=CARTESIAN_POINT ( 'NONE',  ( -10.33201215501379977, 1448.420692391850025, 208.1592603127500070 ) ) ;
#78565=CARTESIAN_POINT ( 'NONE',  ( 12.61234839950090070, 1460.710915196400038, 224.9907160281699987 ) ) ;
#78573=CARTESIAN_POINT ( 'NONE',  ( -2.854778372953739929, 1430.015594105409718, 207.6316838851879822 ) ) ;
#78579=ORIENTED_EDGE ( 'NONE', *, *, #9026, .F. ) ;
#78582=CARTESIAN_POINT ( 'NONE',  ( 12.68313602754479952, 1500.389166761179922, 208.5581353062109997 ) ) ;
#78584=CARTESIAN_POINT ( 'NONE',  ( -1.061334967899610016, 1465.179010130149891, 198.1705584392809953 ) ) ;
#78586=CARTESIAN_POINT ( 'NONE',  ( 12.20373648401209898, 1421.751843755290110, 208.2739721469480116 ) ) ;
#78590=CARTESIAN_POINT ( 'NONE',  ( 8.661166186259681155, 1437.607905750159944, 209.2119232992200182 ) ) ;
#78601=CARTESIAN_POINT ( 'NONE',  ( -0.8109757519344622523, 1455.440442885683069, 218.5281743464129534 ) ) ;
#78604=CARTESIAN_POINT ( 'NONE',  ( -4.372755355000000677, 1508.294786316789896, 220.5537717656990253 ) ) ;
#78605=CARTESIAN_POINT ( 'NONE',  ( -11.16643434163729864, 1471.372555858320084, 206.7508257846899937 ) ) ;
#78606=CARTESIAN_POINT ( 'NONE',  ( 8.534313171132479781, 1434.919546690739935, 206.3689509244539693 ) ) ;
#78637=CARTESIAN_POINT ( 'NONE',  ( -0.4530963034073862139, 1469.489877109852841, 219.1639567478746642 ) ) ;
#78642=CARTESIAN_POINT ( 'NONE',  ( 0.08548078369580100477, 1431.416326821289886, 200.5909471841690106 ) ) ;
#78644=CARTESIAN_POINT ( 'NONE',  ( 3.648450305909999525, 1506.945872735989951, 220.2261833973989837 ) ) ;
#78645=( BOUNDED_CURVE ( )  B_SPLINE_CURVE ( 3, ( #72911, #98641, #45530, #64527 ),
 .UNSPECIFIED., .F., .T. ) 
 B_SPLINE_CURVE_WITH_KNOTS ( ( 4, 4 ),
 ( 4.164116178399805079, 5.260656259123209999 ),
 .UNSPECIFIED. ) 
 CURVE ( )  GEOMETRIC_REPRESENTATION_ITEM ( )  RATIONAL_B_SPLINE_CURVE ( ( 1.000000000000000000, 0.9022849824783407691, 0.9022849824783407691, 1.000000000000000000 ) ) 
 REPRESENTATION_ITEM ( '' )  );
#78646=CARTESIAN_POINT ( 'NONE',  ( 2.487935084889999704, 1508.551704408389924, 214.1089244042930204 ) ) ;
#78650=CARTESIAN_POINT ( 'NONE',  ( -0.003583650733678669757, 1485.228942655789979, 198.2304589643989630 ) ) ;
#78651=CARTESIAN_POINT ( 'NONE',  ( 9.903675653824370428, 1469.012720000510171, 207.5205053474399790 ) ) ;
#78655=CARTESIAN_POINT ( 'NONE',  ( 7.729485065020000434, 1423.503497352910017, 212.7167255717090200 ) ) ;
#78666=CARTESIAN_POINT ( 'NONE',  ( -2.600041615418440255, 1436.399642545620054, 227.4320274269610138 ) ) ;
#78670=CARTESIAN_POINT ( 'NONE',  ( -2.409860608258060033, 1457.727041476990053, 219.5092956769670138 ) ) ;
#78671=CARTESIAN_POINT ( 'NONE',  ( 0.1892422376850020072, 1450.986474787589941, 189.9359345321989849 ) ) ;
#78672=CARTESIAN_POINT ( 'NONE',  ( -9.811963572550000734, 1449.015260455689940, 207.4086770326589999 ) ) ;
#78675=CARTESIAN_POINT ( 'NONE',  ( 7.661576622320000141, 1424.780314478109858, 211.9949546932489852 ) ) ;
#78676=CARTESIAN_POINT ( 'NONE',  ( -17.65532971150000208, 1419.497219977419945, 207.2321558962389929 ) ) ;
#78681=CARTESIAN_POINT ( 'NONE',  ( 6.446188137380000072, 1454.172846498590161, 216.1779746046189814 ) ) ;
#78708=CARTESIAN_POINT ( 'NONE',  ( -3.821721059369999729, 1454.437606006089936, 200.1305965264490112 ) ) ;
#78712=ORIENTED_EDGE ( 'NONE', *, *, #45494, .F. ) ;
#78717=B_SPLINE_SURFACE_WITH_KNOTS ( 'NONE', 5, 5, ( 
 ( #58852, #23575, #92984, #66717, #101360, #58302 ),
 ( #25212, #16798, #92424, #84585, #6771, #15160 ),
 ( #100823, #43154, #85133, #8420, #102480, #7876 ),
 ( #51002, #15699, #24650, #101926, #42044, #76196 ),
 ( #84037, #25769, #40935, #49902, #100294, #57768 ),
 ( #7335, #42592, #57, #76745, #34188, #59968 ),
 ( #94083, #17353, #49351, #41499, #51548, #85685 ),
 ( #8982, #75113, #77310, #608, #35855, #70583 ),
 ( #19016, #18463, #95202, #36939, #1716, #52660 ) ),
 .UNSPECIFIED., .F., .F., .F.,
 ( 6, 3, 6 ),
 ( 6, 6 ),
 ( 13.59708442930000061, 23.84265563570000168, 33.33692106499999852 ),
 ( 0.000000000000000000, 2.000000000000000000 ),
 .UNSPECIFIED. ) ;
#78730=AXIS2_PLACEMENT_3D ( 'NONE', #24688, #66207, #23611 ) ;
#78735=CARTESIAN_POINT ( 'NONE',  ( 24.11200303724299943, 1496.633659200180091, 206.8275310043889874 ) ) ;
#78764=CARTESIAN_POINT ( 'NONE',  ( 2.924270561990000239, 1442.750123219389934, 217.5134303114490137 ) ) ;
#78766=CARTESIAN_POINT ( 'NONE',  ( 1829.302631503766179, 11216.44053380570585, 1606.259476111525828 ) ) ;
#78771=CARTESIAN_POINT ( 'NONE',  ( -5.402270704262029710, 1464.396980422829984, 199.5157612532009921 ) ) ;
#78776=ORIENTED_EDGE ( 'NONE', *, *, #33035, .T. ) ;
#78781=CARTESIAN_POINT ( 'NONE',  ( -1.835776439160000217, 1484.769563154189882, 198.4308762110990187 ) ) ;
#78787=CARTESIAN_POINT ( 'NONE',  ( -8.864783858735460598, 1488.500646863400107, 216.8084363924249942 ) ) ;
#78788=CARTESIAN_POINT ( 'NONE',  ( 19.38664720319999901, 1498.811923108090014, 221.8202413673990065 ) ) ;
#78791=CARTESIAN_POINT ( 'NONE',  ( -4.993214567250789493, 1391.653935164599716, 214.7089805434449943 ) ) ;
#78800=ORIENTED_EDGE ( 'NONE', *, *, #41570, .T. ) ;
#78802=CARTESIAN_POINT ( 'NONE',  ( -15.93619147924319890, 1463.426196661189806, 221.8456080550549814 ) ) ;
#78815=CARTESIAN_POINT ( 'NONE',  ( 7.950846525131810338, 1435.011334183859844, 205.5091519021299860 ) ) ;
#78816=CARTESIAN_POINT ( 'NONE',  ( -13.58955623155380188, 1422.057351869020067, 203.7669116114399799 ) ) ;
#78821=CARTESIAN_POINT ( 'NONE',  ( -4.246466822330569713, 1508.879013277289914, 212.8697876484229994 ) ) ;
#78824=ADVANCED_FACE ( 'NONE', ( #108217 ), #32115, .F. ) ;
#78825=CARTESIAN_POINT ( 'NONE',  ( 16.66443530766549941, 1492.498764680389968, 193.3249378481789904 ) ) ;
#78827=CARTESIAN_POINT ( 'NONE',  ( 7.535268056249999624, 1422.940929649649888, 195.7043803497990098 ) ) ;
#78838=CARTESIAN_POINT ( 'NONE',  ( -10.32785586960000046, 1461.601613025990218, 211.2212836765089889 ) ) ;
#78849=B_SPLINE_CURVE_WITH_KNOTS ( 'NONE', 5,
 ( #30442, #83055, #13617, #48927, #89252, #13070 ),
 .UNSPECIFIED., .F., .F.,
 ( 6, 6 ),
 ( 0.000000000000000000, 1.000000000000000000 ),
 .UNSPECIFIED. ) ;
#78852=CARTESIAN_POINT ( 'NONE',  ( 0.8674825893500259788, 1495.985514189309924, 221.4329466185600097 ) ) ;
#78858=EDGE_CURVE ( 'NONE', #63089, #103670, #47759, .T. ) ;
#78859=( BOUNDED_CURVE ( )  B_SPLINE_CURVE ( 3, ( #59147, #49087, #93268, #50722 ),
 .UNSPECIFIED., .F., .T. ) 
 B_SPLINE_CURVE_WITH_KNOTS ( ( 4, 4 ),
 ( 1.028227595440492026, 2.113365490006624992 ),
 .UNSPECIFIED. ) 
 CURVE ( )  GEOMETRIC_REPRESENTATION_ITEM ( )  RATIONAL_B_SPLINE_CURVE ( ( 1.000000000000000000, 0.9042567095595046567, 0.9042567095595046567, 1.000000000000000000 ) ) 
 REPRESENTATION_ITEM ( '' )  );
#78862=CARTESIAN_POINT ( 'NONE',  ( -17.06985514805390025, 1508.522286251240075, 212.9373325725379971 ) ) ;
#78863=CARTESIAN_POINT ( 'NONE',  ( 8.650035068340001132, 1470.670675412089849, 214.4250021573690219 ) ) ;
#78865=CARTESIAN_POINT ( 'NONE',  ( -8.499221297664830033, 1438.111010583779944, 207.3306852776750020 ) ) ;
#78870=CARTESIAN_POINT ( 'NONE',  ( 8.385113454956041323, 1436.167270151570165, 207.1929903346489823 ) ) ;
#78874=ADVANCED_FACE ( 'NONE', ( #95828 ), #35360, .T. ) ;
#78890=CARTESIAN_POINT ( 'NONE',  ( 3.273042392802009815, 1508.551704408389924, 204.1347633686989980 ) ) ;
#78905=CARTESIAN_POINT ( 'NONE',  ( -17.40249709480000107, 1417.619717898290219, 206.9114233350790073 ) ) ;
#78908=CARTESIAN_POINT ( 'NONE',  ( -10.07374399369030016, 1483.508491176670077, 202.7669571214699999 ) ) ;
#78909=EDGE_CURVE ( 'NONE', #69529, #17806, #52337, .T. ) ;
#78912=CARTESIAN_POINT ( 'NONE',  ( -0.1448779671327833363, 1421.022422678020575, 193.7177100718903091 ) ) ;
#78919=CARTESIAN_POINT ( 'NONE',  ( -9.775905228975700467, 1461.154446592330032, 210.2374177378800084 ) ) ;
#78920=CARTESIAN_POINT ( 'NONE',  ( -16.94833435341390171, 1419.662971730580011, 201.4173425967440210 ) ) ;
#78921=VERTEX_POINT ( 'NONE', #78485 ) ;
#78924=EDGE_CURVE ( 'NONE', #104968, #50471, #59075, .T. ) ;
#78926=FACE_OUTER_BOUND ( 'NONE', #17408, .T. ) ;
#78929=CARTESIAN_POINT ( 'NONE',  ( -17.27256466963439863, 1419.895559490180403, 207.2304356867004458 ) ) ;
#78932=CARTESIAN_POINT ( 'NONE',  ( -2.487923629571139994, 1508.884229736110001, 204.6305622231600125 ) ) ;
#78934=CARTESIAN_POINT ( 'NONE',  ( -2173.981453289206911, -8382.262153571264207, 1975.191541669308435 ) ) ;
#78936=CARTESIAN_POINT ( 'NONE',  ( 3.736539510769999684, 1442.283932804090000, 217.1659672788889850 ) ) ;
#78942=CARTESIAN_POINT ( 'NONE',  ( -4.633158249500000103, 1476.260951450290122, 199.8663068878290119 ) ) ;
#78945=CARTESIAN_POINT ( 'NONE',  ( 14.17510881067400064, 1428.761380490490183, 195.0896992289169987 ) ) ;
#78949=CARTESIAN_POINT ( 'NONE',  ( -1.864982813339999934, 1489.661995449090227, 188.3491068096989807 ) ) ;
#78953=CARTESIAN_POINT ( 'NONE',  ( -2.429964404760000196, 1432.449532658489943, 217.5898836994890075 ) ) ;
#78959=CARTESIAN_POINT ( 'NONE',  ( -3.523962699983150149, 1476.511731499819916, 220.0526012347959863 ) ) ;
#78961=CIRCLE ( 'NONE', #53970, 11.73460161499999899 ) ;
#78962=CARTESIAN_POINT ( 'NONE',  ( 10.79524667479070033, 1489.627639623460027, 207.4011449438049794 ) ) ;
#78965=CARTESIAN_POINT ( 'NONE',  ( -19.83859993069999916, 1467.194195006989958, 209.1218459616989946 ) ) ;
#78985=CARTESIAN_POINT ( 'NONE',  ( 0.4117221240290019901, 1496.667641243389880, 196.7318124780990161 ) ) ;
#78986=CARTESIAN_POINT ( 'NONE',  ( -1.133238050829999954, 1495.637768932689823, 220.4196360831990091 ) ) ;
#78998=CARTESIAN_POINT ( 'NONE',  ( -1.222313235619999938, 1487.670855816090125, 219.9174996087990053 ) ) ;
#79003=CARTESIAN_POINT ( 'NONE',  ( 10.81377540340000110, 1493.463431426289844, 215.2021047779490175 ) ) ;
#79004=CARTESIAN_POINT ( 'NONE',  ( 9.698097846587389270, 1462.705833979410045, 208.0596819494889758 ) ) ;
#79005=ADVANCED_FACE ( 'NONE', ( #59908 ), #44330, .F. ) ;
#79008=EDGE_LOOP ( 'NONE', ( #9719, #34154, #48311, #5981, #67473, #105268, #64947, #92974, #80802, #51730, #86000, #27877, #105098 ) ) ;
#79009=CARTESIAN_POINT ( 'NONE',  ( 9.109326017966379752, 1452.537928671039708, 211.6759096298679879 ) ) ;
#79010=CARTESIAN_POINT ( 'NONE',  ( 7.158179755560000856, 1423.953782493189919, 195.2758576736989937 ) ) ;
#79020=CARTESIAN_POINT ( 'NONE',  ( 18.81609481059999922, 1456.479165729590022, 204.5196734937790097 ) ) ;
#79030=CARTESIAN_POINT ( 'NONE',  ( -5.868857667190599869, 1508.551703962909869, 219.6331723996029837 ) ) ;
#79032=CARTESIAN_POINT ( 'NONE',  ( -5.613020775148240382, 1470.678943295929912, 217.6304317108330224 ) ) ;
#79035=CARTESIAN_POINT ( 'NONE',  ( 9.196086508652181024, 1450.899357183659959, 210.0407472026730034 ) ) ;
#79036=CARTESIAN_POINT ( 'NONE',  ( -8.928049104570000338, 1472.922707491090023, 201.8104512964389983 ) ) ;
#79037=CARTESIAN_POINT ( 'NONE',  ( 9.553964019109999484, 1492.165809702890101, 214.7542154822990028 ) ) ;
#79039=CARTESIAN_POINT ( 'NONE',  ( 8.960106487924051066, 1425.021082012188799, 195.6425420597072673 ) ) ;
#79043=CARTESIAN_POINT ( 'NONE',  ( -9.956812081275220550, 1439.552395354249938, 208.2581519739229918 ) ) ;
#79050=CARTESIAN_POINT ( 'NONE',  ( 3.944248398050000048, 1506.370035955090088, 220.2366324052989626 ) ) ;
#79052=CARTESIAN_POINT ( 'NONE',  ( -1.407451548162420130, 1515.079400017670196, 204.7927796877619926 ) ) ;
#79055=DIRECTION ( 'NONE',  ( 1.000000000000000000, 0.000000000000000000, 0.000000000000000000 ) ) ;
#79057=CARTESIAN_POINT ( 'NONE',  ( 5.200787045398697295, 1440.223982444788362, 217.6291937790904285 ) ) ;
#79064=CARTESIAN_POINT ( 'NONE',  ( 9.961228442255011473, 1469.533171005829900, 210.4989064630590008 ) ) ;
#79072=CARTESIAN_POINT ( 'NONE',  ( -5.080289282479999002, 1480.093209919690253, 228.8812397303989883 ) ) ;
#79074=CARTESIAN_POINT ( 'NONE',  ( -3.317807041231336485E-31, 1414.677402202029953, 209.1218459616989946 ) ) ;
#79080=CARTESIAN_POINT ( 'NONE',  ( 18.18312599666770168, 1429.576275455930045, 208.4333127768320253 ) ) ;
#79082=ORIENTED_EDGE ( 'NONE', *, *, #19897, .F. ) ;
#79085=CARTESIAN_POINT ( 'NONE',  ( -12.89242915326980032, 1508.551704408300111, 210.2815080484370185 ) ) ;
#79088=CARTESIAN_POINT ( 'NONE',  ( -11.87098815724909961, 1481.783871394969992, 209.3733780729720024 ) ) ;
#79099=FACE_OUTER_BOUND ( 'NONE', #67031, .T. ) ;
#79103=CARTESIAN_POINT ( 'NONE',  ( 4.548814465829999598, 1424.046559047009850, 193.1022451195989618 ) ) ;
#79107=CARTESIAN_POINT ( 'NONE',  ( 7.830182259921620869, 1460.133318085240035, 228.9032440295520132 ) ) ;
#79111=CARTESIAN_POINT ( 'NONE',  ( -5.146359519290000684, 1391.913486199090130, 203.5916337600390023 ) ) ;
#79113=CARTESIAN_POINT ( 'NONE',  ( -11.77655089729999816, 1490.342630228989947, 209.9285965979820219 ) ) ;
#79120=CARTESIAN_POINT ( 'NONE',  ( 10.93254534338380068, 1502.901713907840076, 213.3630869133220074 ) ) ;
#79128=VERTEX_POINT ( 'NONE', #72711 ) ;
#79129=CARTESIAN_POINT ( 'NONE',  ( -2.283769792747494698, 1456.639021601948798, 199.9092664731689979 ) ) ;
#79139=CARTESIAN_POINT ( 'NONE',  ( -11.60879801380000131, 1421.965952794710120, 210.6472336029989947 ) ) ;
#79142=CARTESIAN_POINT ( 'NONE',  ( -0.002530016318419649971, 1432.316930810580061, 200.6915054315279860 ) ) ;
#79148=CARTESIAN_POINT ( 'NONE',  ( 20.54534055259999903, 1497.714303034489831, 214.2326470396490095 ) ) ;
#79150=CARTESIAN_POINT ( 'NONE',  ( 1.184628359070449832, 1465.692306277839862, 198.1686851201980062 ) ) ;
#79177=DIRECTION ( 'NONE',  ( 0.6339197603454396202, 4.315842897467507453E-06, 0.7733988217116404273 ) ) ;
#79187=ORIENTED_EDGE ( 'NONE', *, *, #43955, .F. ) ;
#79191=CARTESIAN_POINT ( 'NONE',  ( -14.16362978420000118, 1415.677402215299935, 203.9764128900390006 ) ) ;
#79198=ORIENTED_EDGE ( 'NONE', *, *, #75681, .F. ) ;
#79208=CARTESIAN_POINT ( 'NONE',  ( -11.41402561306639996, 1500.969831351809944, 208.5831151434670119 ) ) ;
#79211=CARTESIAN_POINT ( 'NONE',  ( 3.063200971469999701, 1505.793422128889915, 221.5342279770990217 ) ) ;
#79212=CARTESIAN_POINT ( 'NONE',  ( -5.369110597919999783, 1438.274585814490138, 207.8054623959989726 ) ) ;
#79215=CARTESIAN_POINT ( 'NONE',  ( 2.203042164229999766, 1485.447018732490051, 198.5856978324989939 ) ) ;
#79216=CARTESIAN_POINT ( 'NONE',  ( 8.093949986950837783, 1466.712779916819954, 203.1193089748180114 ) ) ;
#79218=B_SPLINE_CURVE_WITH_KNOTS ( 'NONE', 5,
 ( #72058, #3743, #79328, #106174, #97214, #37322 ),
 .UNSPECIFIED., .F., .F.,
 ( 6, 6 ),
 ( 239.1631355520000000, 244.0515247689999967 ),
 .UNSPECIFIED. ) ;
#79219=DIRECTION ( 'NONE',  ( 0.9980318515193541407, 1.681712440757244397E-31, 0.06270903725022322628 ) ) ;
#79231=CARTESIAN_POINT ( 'NONE',  ( -11.39540616852265131, 1501.162789497870790, 208.1690291723011796 ) ) ;
#79233=CARTESIAN_POINT ( 'NONE',  ( -1.254332932929999922, 1509.200097200889786, 218.0171177365190260 ) ) ;
#79235=CARTESIAN_POINT ( 'NONE',  ( -9.962652008186671182, 1439.046469533959907, 209.4352736110479896 ) ) ;
#79240=CARTESIAN_POINT ( 'NONE',  ( 7.684424406179999778, 1424.938446056360135, 211.9182770897589876 ) ) ;
#79241=CARTESIAN_POINT ( 'NONE',  ( -19.73707534100000061, 1467.795347597790169, 204.3773262252089751 ) ) ;
#79247=ORIENTED_EDGE ( 'NONE', *, *, #32911, .F. ) ;
#79264=ORIENTED_EDGE ( 'NONE', *, *, #24897, .T. ) ;
#79268=ORIENTED_EDGE ( 'NONE', *, *, #34941, .T. ) ;
#79269=CARTESIAN_POINT ( 'NONE',  ( -3.980518584870000431, 1455.210856568990039, 200.5685208411690326 ) ) ;
#79274=CARTESIAN_POINT ( 'NONE',  ( 16.56647452670000220, 1428.020747124390027, 201.4090148566590130 ) ) ;
#79288=CARTESIAN_POINT ( 'NONE',  ( -4.860709314987225582, 1442.585814854372302, 201.1804672816271022 ) ) ;
#79294=CARTESIAN_POINT ( 'NONE',  ( 16.01085410965039912, 1427.818095826660056, 200.6391735007109673 ) ) ;
#79295=CARTESIAN_POINT ( 'NONE',  ( -21.47380431054590133, 1487.892812373600009, 202.0847385657529856 ) ) ;
#79303=CARTESIAN_POINT ( 'NONE',  ( -2.792418666239999681, 1429.036568613389818, 200.1755848472290040 ) ) ;
#79314=CARTESIAN_POINT ( 'NONE',  ( 10.21479392009059950, 1470.289319449759887, 209.7510399118739883 ) ) ;
#79320=B_SPLINE_CURVE_WITH_KNOTS ( 'NONE', 3,
 ( #103747, #26472, #94792, #110490, #52263, #16943, #60666, #751, #60108, #85838 ),
 .UNSPECIFIED., .F., .F.,
 ( 4, 2, 2, 2, 4 ),
 ( -2.055505557828499974, -1.540184857421819986, -1.025851360773140097, -0.5122551694543180378, 0.000000000000000000 ),
 .UNSPECIFIED. ) ;
#79322=CARTESIAN_POINT ( 'NONE',  ( 3.007039662469999985, 1441.535621289990104, 218.1727171078889853 ) ) ;
#79328=CARTESIAN_POINT ( 'NONE',  ( -19.70212423939999979, 1465.426585210689836, 207.1871696898290054 ) ) ;
#79337=CARTESIAN_POINT ( 'NONE',  ( -5.090491209510000559, 1484.752177510490128, 198.8227071155990018 ) ) ;
#79338=CARTESIAN_POINT ( 'NONE',  ( -16.67868778038742406, 1417.215853041899663, 207.0928179806824971 ) ) ;
#79340=CARTESIAN_POINT ( 'NONE',  ( 5.312679136500000787, 1493.059131431590231, 218.8466398904690209 ) ) ;
#79343=CARTESIAN_POINT ( 'NONE',  ( -7.440906847757699616, 1489.915291769369787, 217.2245407447130106 ) ) ;
#79344=CARTESIAN_POINT ( 'NONE',  ( 22.14279320874160106, 1473.984109767550081, 210.1089530530229865 ) ) ;
#79357=CARTESIAN_POINT ( 'NONE',  ( -7.828738281090000584, 1492.799651794089868, 208.3779021618599927 ) ) ;
#79361=CARTESIAN_POINT ( 'NONE',  ( 3.706798618510000143, 1486.448926241190065, 219.2581982017989901 ) ) ;
#79363=CARTESIAN_POINT ( 'NONE',  ( 8.977937034530510729, 1435.738637591490033, 208.3987603176270227 ) ) ;
#79365=CARTESIAN_POINT ( 'NONE',  ( 2.452021889690000123, 1486.921751305789940, 216.7943168417889979 ) ) ;
#79371=CARTESIAN_POINT ( 'NONE',  ( -16.41672048914309912, 1420.652106645439744, 203.2831381211010182 ) ) ;
#79375=CARTESIAN_POINT ( 'NONE',  ( -13.02153297019999911, 1507.740364904889930, 209.3504333174379894 ) ) ;
#79376=CARTESIAN_POINT ( 'NONE',  ( -5.367627633762589667, 1490.060063169970135, 185.8829590531140070 ) ) ;
#79390=CARTESIAN_POINT ( 'NONE',  ( -8.012082702599998996, 1424.887577014409999, 210.3493509962989947 ) ) ;
#79399=B_SPLINE_SURFACE_WITH_KNOTS ( 'NONE', 5, 5, ( 
 ( #86589, #18817, #87147, #10435, #61977, #96091, #4783, #6452, #5344 ),
 ( #65821, #73677, #82611, #99385, #107250, #64174, #91559, #5902, #83159 ),
 ( #55221, #22108, #38929, #56863, #29982, #106691, #90993, #89351, #107804 ),
 ( #98295, #73109, #14834, #47354, #89894, #21570, #12645, #80954, #39503 ),
 ( #74229, #90440, #30543, #97746, #46823, #14283, #48473, #64733, #40047 ),
 ( #49023, #40599, #21017, #65272, #56308, #81482, #108359, #23235, #63632 ),
 ( #82038, #31641, #98847, #38388, #22661, #4253, #13718, #74770, #108910 ),
 ( #99940, #57433, #72564, #55780, #13165, #47903, #31090, #32748, #24871 ),
 ( #33846, #15922, #93198, #51210, #42258, #17574, #41703, #68037, #25980 ) ),
 .UNSPECIFIED., .F., .F., .F.,
 ( 6, 3, 6 ),
 ( 6, 3, 6 ),
 ( 19.77745610209999683, 22.54012251900000052, 25.30278893590000067 ),
 ( 0.000000000000000000, 1.500000000000000000, 3.000000000000000000 ),
 .UNSPECIFIED. ) ;
#79405=CARTESIAN_POINT ( 'NONE',  ( -18.67521810751130218, 1508.457196392550031, 210.8041937590900261 ) ) ;
#79406=CARTESIAN_POINT ( 'NONE',  ( 8.695521651920000039, 1472.655120818390060, 215.9601142780390148 ) ) ;
#79407=CARTESIAN_POINT ( 'NONE',  ( -9.393416945061629164, 1439.826643058699801, 207.2591784000079826 ) ) ;
#79412=CARTESIAN_POINT ( 'NONE',  ( -3.750000000000000000, 1524.051704408389924, 209.1218459616989946 ) ) ;
#79418=CARTESIAN_POINT ( 'NONE',  ( -0.3306155012354299871, 1467.554131235530122, 220.2123213960779822 ) ) ;
#79420=CARTESIAN_POINT ( 'NONE',  ( 19.60792669039999936, 1475.100271358290229, 204.3343059087790152 ) ) ;
#79421=B_SPLINE_CURVE_WITH_KNOTS ( 'NONE', 5,
 ( #83158, #32747, #107803, #108909, #66927, #66383, #31640, #6451, #65271 ),
 .UNSPECIFIED., .F., .F.,
 ( 6, 3, 6 ),
 ( 0.000000000000000000, 0.5000000000000001110, 1.000000000000000000 ),
 .UNSPECIFIED. ) ;
#79422=COLOUR_RGB ( '', 0.40784314, 0.44705882, 0.49803922) ;
#79429=EDGE_LOOP ( 'NONE', ( #91850, #101592, #82604, #18991 ) ) ;
#79448=FACE_OUTER_BOUND ( 'NONE', #7665, .T. ) ;
#79449=CARTESIAN_POINT ( 'NONE',  ( -9.542478684123411270, 1481.357605987509942, 204.5426329703269914 ) ) ;
#79450=CARTESIAN_POINT ( 'NONE',  ( -9.587265584406980068, 1483.699063712610041, 202.0552589649070114 ) ) ;
#79453=EDGE_CURVE ( 'NONE', #67656, #51303, #84436, .T. ) ;
#79456=CARTESIAN_POINT ( 'NONE',  ( -10.64712356781720004, 1462.974733331459902, 206.1443014032890062 ) ) ;
#79461=CARTESIAN_POINT ( 'NONE',  ( -9.594642682941978862, 1460.625312738239700, 210.3248870281339862 ) ) ;
#79463=CARTESIAN_POINT ( 'NONE',  ( -17.68330801639999805, 1419.886192764050065, 207.3225218594289743 ) ) ;
#79470=CARTESIAN_POINT ( 'NONE',  ( 12.07139996528260006, 1501.489333478010167, 211.6019455624989973 ) ) ;
#79477=CARTESIAN_POINT ( 'NONE',  ( -4.492641829143109611, 1508.880977751779938, 206.0044442880380018 ) ) ;
#79480=CARTESIAN_POINT ( 'NONE',  ( 203.9558787908000284, -8382.262153571269664, -1760.903728536709878 ) ) ;
#79481=CARTESIAN_POINT ( 'NONE',  ( 8.971908151997389780, 1451.470056219970047, 211.4421882215459902 ) ) ;
#79482=CARTESIAN_POINT ( 'NONE',  ( 3.289090359600000291, 1441.224765589789968, 218.4797294130789851 ) ) ;
#79486=CARTESIAN_POINT ( 'NONE',  ( -4.912638278920000268, 1474.545047148890035, 199.2507986654790102 ) ) ;
#79488=ORIENTED_EDGE ( 'NONE', *, *, #73247, .T. ) ;
#79489=FACE_OUTER_BOUND ( 'NONE', #79008, .T. ) ;
#79493=CARTESIAN_POINT ( 'NONE',  ( -3.866774376410000436, 1489.349301186990033, 188.6533245077989989 ) ) ;
#79496=CARTESIAN_POINT ( 'NONE',  ( 17.10950584751149961, 1472.077583655310036, 198.3318500205459998 ) ) ;
#79497=CARTESIAN_POINT ( 'NONE',  ( -3.117383295799999843, 1432.833160025789994, 217.3708154071790091 ) ) ;
#79498=CARTESIAN_POINT ( 'NONE',  ( -14.74045126690000096, 1418.924813655680055, 213.5838659850790009 ) ) ;
#79503=CARTESIAN_POINT ( 'NONE',  ( 10.03481087325400090, 1426.170452349230118, 208.8300883510670189 ) ) ;
#79505=CARTESIAN_POINT ( 'NONE',  ( 11.65430695225310131, 1491.292500647989982, 207.0498289997640029 ) ) ;
#79507=VERTEX_POINT ( 'NONE', #18282 ) ;
#79508=ORIENTED_EDGE ( 'NONE', *, *, #80218, .F. ) ;
#79510=AXIS2_PLACEMENT_3D ( 'NONE', #33000, #101849, #93455 ) ;
#79513=CARTESIAN_POINT ( 'NONE',  ( 12.27763887519870067, 1427.216651625929899, 207.3866983009849889 ) ) ;
#79525=CARTESIAN_POINT ( 'NONE',  ( -14.85004060048409968, 1489.439381932599872, 194.1045853035489870 ) ) ;
#79543=CARTESIAN_POINT ( 'NONE',  ( -3.829620113920000346, 1515.551704408389924, 206.7917118429090237 ) ) ;
#79547=CARTESIAN_POINT ( 'NONE',  ( 9.261703887511778532, 1452.295026765300008, 211.0154049713290192 ) ) ;
#79549=ADVANCED_FACE ( 'NONE', ( #9897 ), #32716, .F. ) ;
#79551=CARTESIAN_POINT ( 'NONE',  ( -2.469737631213410278, 1507.227429411520006, 221.7265308815400147 ) ) ;
#79552=CARTESIAN_POINT ( 'NONE',  ( -9.670206149040000199, 1461.150141550089984, 208.5232313836649780 ) ) ;
#79555=DIRECTION ( 'NONE',  ( -7.436362843295819681E-17, 1.000000000000000000, -1.457576885956999882E-16 ) ) ;
#79567=EDGE_CURVE ( 'NONE', #77824, #59860, #29696, .T. ) ;
#79572=CARTESIAN_POINT ( 'NONE',  ( -4.767896964821690453, 1508.551704797160028, 219.9121068361049822 ) ) ;
#79574=CARTESIAN_POINT ( 'NONE',  ( -9.699736313928079667, 1472.031488563110088, 212.1561346718199843 ) ) ;
#79578=CARTESIAN_POINT ( 'NONE',  ( -6.386479664280000357, 1475.602365189490001, 200.9502241406889880 ) ) ;
#79579=CARTESIAN_POINT ( 'NONE',  ( -2.187611056739820370, 1421.597788280269924, 193.5642244024440117 ) ) ;
#79581=CARTESIAN_POINT ( 'NONE',  ( 8.936510400883047822, 1425.002876951823964, 195.6473277186463520 ) ) ;
#79582=CARTESIAN_POINT ( 'NONE',  ( -18.11269319780000231, 1504.989642490190136, 208.9951304212659977 ) ) ;
#79593=EDGE_CURVE ( 'NONE', #54152, #77692, #21992, .T. ) ;
#79595=CARTESIAN_POINT ( 'NONE',  ( -14.80753115500000128, 1415.677402202029953, 211.4744607310090032 ) ) ;
#79596=CARTESIAN_POINT ( 'NONE',  ( 12.76115332701539984, 1421.043083730220133, 203.4305847601519872 ) ) ;
#79597=ORIENTED_EDGE ( 'NONE', *, *, #32618, .T. ) ;
#79598=CARTESIAN_POINT ( 'NONE',  ( -16.66450378662129950, 1418.448320473469948, 203.1257116146589965 ) ) ;
#79600=CARTESIAN_POINT ( 'NONE',  ( -15.92611295390000059, 1415.966327314990167, 209.5991268886040189 ) ) ;
#79601=CARTESIAN_POINT ( 'NONE',  ( -1.736489803575699931, 1429.592721204729969, 199.8987770947680076 ) ) ;
#79610=CARTESIAN_POINT ( 'NONE',  ( -3.527120678209999749, 1475.290298288389977, 218.8061202455889998 ) ) ;
#79616=B_SPLINE_SURFACE_WITH_KNOTS ( 'NONE', 5, 5, ( 
 ( #13409, #5593, #73907, #31329, #54370, #80089 ),
 ( #83942, #16166, #7242, #58752, #8328, #101827 ),
 ( #14523, #85037, #42492, #76104, #66626, #83383 ),
 ( #76648, #75014, #57673, #67719, #93436, #82835 ),
 ( #15062, #109164, #110800, #34091, #74468, #32977 ),
 ( #57117, #41403, #49811, #58205, #25120, #68284 ) ),
 .UNSPECIFIED., .F., .F., .F.,
 ( 6, 6 ),
 ( 6, 6 ),
 ( 7.548656686150459372, 12.57640183258060063 ),
 ( 0.000000000000000000, 0.5000176499934829710 ),
 .UNSPECIFIED. ) ;
#79622=CARTESIAN_POINT ( 'NONE',  ( -15.52550892592270060, 1418.207173107500012, 203.0520299323999893 ) ) ;
#79625=CARTESIAN_POINT ( 'NONE',  ( -15.42329654610000134, 1414.772672120240031, 208.8174072822980065 ) ) ;
#79635=CARTESIAN_POINT ( 'NONE',  ( -12.66301831902579877, 1508.551708339549805, 209.9035433704430034 ) ) ;
#79654=CARTESIAN_POINT ( 'NONE',  ( -1.577403822089999963, 1422.569002067519932, 192.5427128247989970 ) ) ;
#79656=B_SPLINE_SURFACE_WITH_KNOTS ( 'NONE', 5, 1, ( 
 ( #46459, #107430 ),
 ( #13909, #54313 ),
 ( #55949, #73295 ),
 ( #48095, #81125 ),
 ( #88978, #12267 ),
 ( #30725, #97923 ) ),
 .UNSPECIFIED., .F., .F., .F.,
 ( 6, 6 ),
 ( 2, 2 ),
 ( 0.000000000000000000, 3.890291737050000087 ),
 ( 0.000000000000000000, 14.00000000000000000 ),
 .UNSPECIFIED. ) ;
#79658=CARTESIAN_POINT ( 'NONE',  ( 20.84774931509999973, 1457.996261225589933, 206.6760932923689893 ) ) ;
#79662=CARTESIAN_POINT ( 'NONE',  ( -5.024578973489999711, 1391.800828890389994, 203.6117233725290134 ) ) ;
#79671=CARTESIAN_POINT ( 'NONE',  ( -11.68980366881247335, 1421.933377081587423, 210.6412079282914362 ) ) ;
#79674=EDGE_LOOP ( 'NONE', ( #10102, #58905, #8644, #24542, #42785 ) ) ;
#79676=ORIENTED_EDGE ( 'NONE', *, *, #19284, .T. ) ;
#79677=DIRECTION ( 'NONE',  ( -1.132411226124150056E-06, 0.9999999999963642416, 2.447241413984286834E-06 ) ) ;
#79684=CARTESIAN_POINT ( 'NONE',  ( -2.130922737000000122, 1467.954349366689939, 220.0452206860990145 ) ) ;
#79689=CARTESIAN_POINT ( 'NONE',  ( -6.696214959435129899, 1424.446799123830033, 209.0310039315669997 ) ) ;
#79692=CARTESIAN_POINT ( 'NONE',  ( -19.86464710129999744, 1441.435714617490021, 212.6459466283089910 ) ) ;
#79696=EDGE_LOOP ( 'NONE', ( #14292, #52043, #25032, #67523 ) ) ;
#79706=CARTESIAN_POINT ( 'NONE',  ( 8.658163031318741432, 1437.533170863820033, 209.0585791703279881 ) ) ;
#79718=CARTESIAN_POINT ( 'NONE',  ( 6.813936602420000099, 1469.517477258589906, 209.5520740031860214 ) ) ;
#79719=CARTESIAN_POINT ( 'NONE',  ( -9.547530987552349302, 1437.933916352150163, 211.7113974646419763 ) ) ;
#79723=CARTESIAN_POINT ( 'NONE',  ( -4.455463436649999664, 1508.108973204389940, 220.6784667051990141 ) ) ;
#79746=CARTESIAN_POINT ( 'NONE',  ( -9.045810569538431878, 1449.339667039310143, 210.6515513332149681 ) ) ;
#79751=CARTESIAN_POINT ( 'NONE',  ( -1.842962231260000028, 1515.064792882589927, 213.4512947377390049 ) ) ;
#79752=ADVANCED_FACE ( 'NONE', ( #48764 ), #33943, .T. ) ;
#79753=CIRCLE ( 'NONE', #10029, 7.799999999999999822 ) ;
#79762=CARTESIAN_POINT ( 'NONE',  ( 0.6715583085099990912, 1506.489872953789927, 221.9351472385990007 ) ) ;
#79767=CARTESIAN_POINT ( 'NONE',  ( 3.535327689299999854, 1487.160995979990048, 197.6951163427989968 ) ) ;
#79768=FACE_OUTER_BOUND ( 'NONE', #91103, .T. ) ;
#79770=CARTESIAN_POINT ( 'NONE',  ( 1.332267629549999902E-15, 1413.913060387330006, 209.1218459616989946 ) ) ;
#79772=EDGE_CURVE ( 'NONE', #28187, #14911, #108435, .T. ) ;
#79776=CARTESIAN_POINT ( 'NONE',  ( -9.779853762240000137, 1481.708752394490148, 205.0329629307690027 ) ) ;
#79784=ORIENTED_EDGE ( 'NONE', *, *, #21439, .F. ) ;
#79785=CARTESIAN_POINT ( 'NONE',  ( -1.813815691101789973, 1436.230605934150162, 227.5234084965020145 ) ) ;
#79786=CARTESIAN_POINT ( 'NONE',  ( -13.58372279061449994, 1508.526660466229941, 210.1193507368990367 ) ) ;
#79792=CARTESIAN_POINT ( 'NONE',  ( -4.761835944330000459, 1382.817942041290053, 203.6389619452989734 ) ) ;
#79793=CARTESIAN_POINT ( 'NONE',  ( 7.638852881150000051, 1424.646166941220145, 212.0768851055590005 ) ) ;
#79810=FACE_OUTER_BOUND ( 'NONE', #104893, .T. ) ;
#79818=ORIENTED_EDGE ( 'NONE', *, *, #81537, .T. ) ;
#79823=CARTESIAN_POINT ( 'NONE',  ( -3.558362537839999895, 1455.955980043889895, 200.3550983807189994 ) ) ;
#79828=DIRECTION ( 'NONE',  ( -9.120877578445558697E-47, 1.000000000000000000, -1.836970198721029688E-16 ) ) ;
#79833=CARTESIAN_POINT ( 'NONE',  ( 11.41833509600000163, 1492.743966792589845, 212.4764448217789834 ) ) ;
#79835=CARTESIAN_POINT ( 'NONE',  ( 9.275662108596250732, 1461.991666016340105, 206.1939425705140252 ) ) ;
#79847=CARTESIAN_POINT ( 'NONE',  ( 11.54155030333390108, 1426.278799798020145, 195.2408946065239945 ) ) ;
#79856=CARTESIAN_POINT ( 'NONE',  ( -4.490619218195398332, 1508.909942012477359, 206.6339108000523481 ) ) ;
#79866=CARTESIAN_POINT ( 'NONE',  ( 10.04531431606059932, 1469.136521703999961, 209.2681548814119878 ) ) ;
#79875=CARTESIAN_POINT ( 'NONE',  ( 3.181172984599999864, 1442.605928313790173, 217.4126502567789885 ) ) ;
#79877=CARTESIAN_POINT ( 'NONE',  ( 10.94754737549849821, 1490.097295750230160, 208.8086307138860036 ) ) ;
#79878=CARTESIAN_POINT ( 'NONE',  ( -17.64146421497870065, 1419.304501645640130, 207.1873797621490212 ) ) ;
#79891=CARTESIAN_POINT ( 'NONE',  ( -4.780581990890000021, 1483.100110836790009, 199.6018351111989944 ) ) ;
#79896=CARTESIAN_POINT ( 'NONE',  ( -11.18353437974609932, 1470.314597740729823, 211.2446877208680007 ) ) ;
#79897=CARTESIAN_POINT ( 'NONE',  ( -6.007801178118840291, 1489.444426110659833, 218.3574661116689981 ) ) ;
#79898=CARTESIAN_POINT ( 'NONE',  ( -21.44637799630000075, 1506.412602296789828, 216.0243671510289971 ) ) ;
#79909=VERTEX_POINT ( 'NONE', #3147 ) ;
#79915=CARTESIAN_POINT ( 'NONE',  ( 8.999746791583771000, 1435.834253586629984, 208.6187618879379784 ) ) ;
#79917=CARTESIAN_POINT ( 'NONE',  ( 3.749012616329999936, 1480.578083832889888, 229.2223542577989974 ) ) ;
#79921=CARTESIAN_POINT ( 'NONE',  ( 1.842963219480119985, 1515.064792700640055, 213.4512947425059792 ) ) ;
#79927=CARTESIAN_POINT ( 'NONE',  ( -11.89363985299999982, 1506.209575258589894, 208.4879603470639893 ) ) ;
#79928=CARTESIAN_POINT ( 'NONE',  ( -11.80575459840840047, 1482.971163947439891, 228.2220767440819884 ) ) ;
#79930=CARTESIAN_POINT ( 'NONE',  ( 10.39122783130000016, 1420.703789618900146, 197.9464487691990087 ) ) ;
#79936=CARTESIAN_POINT ( 'NONE',  ( -6.579934403380000241, 1457.806054071189919, 216.0580061265189897 ) ) ;
#79939=ORIENTED_EDGE ( 'NONE', *, *, #52826, .F. ) ;
#79940=CARTESIAN_POINT ( 'NONE',  ( -9.253356380629998768, 1423.298286757820051, 209.1001181959080100 ) ) ;
#79947=CARTESIAN_POINT ( 'NONE',  ( -1.190766908926550238, 1496.523138748749943, 221.4220572319329960 ) ) ;
#79951=CARTESIAN_POINT ( 'NONE',  ( 6.420745879690000102, 1472.574659317690021, 217.2589463166690109 ) ) ;
#79952=CARTESIAN_POINT ( 'NONE',  ( -8.414692022134790506, 1438.300249502180122, 206.9250335065700028 ) ) ;
#79962=CARTESIAN_POINT ( 'NONE',  ( 2.477236684321269866, 1466.740809377600044, 219.8979591610699913 ) ) ;
#79966=FACE_OUTER_BOUND ( 'NONE', #33510, .T. ) ;
#79972=ORIENTED_EDGE ( 'NONE', *, *, #45953, .T. ) ;
#79980=CARTESIAN_POINT ( 'NONE',  ( -3.815543930780000093, 1414.170066830949963, 206.6642445390390037 ) ) ;
#79984=CARTESIAN_POINT ( 'NONE',  ( 10.84341014260000158, 1490.334183146890155, 204.2640498865189898 ) ) ;
#79991=CARTESIAN_POINT ( 'NONE',  ( -17.28305401740000136, 1417.746658045750110, 207.2609050454489932 ) ) ;
#79994=EDGE_CURVE ( 'NONE', #53103, #88887, #68398, .T. ) ;
#79999=CARTESIAN_POINT ( 'NONE',  ( 17.76546875260000036, 1430.865606781589804, 204.9340536459789917 ) ) ;
#80005=CARTESIAN_POINT ( 'NONE',  ( 11.07831394190110075, 1500.667860359830001, 205.8219701691039916 ) ) ;
#80016=CARTESIAN_POINT ( 'NONE',  ( -16.54816711760097547, 1420.093509083089202, 208.5750742618841400 ) ) ;
#80019=CARTESIAN_POINT ( 'NONE',  ( -4.487359966065140426, 1509.034537944679869, 206.0057109289620030 ) ) ;
#80021=CARTESIAN_POINT ( 'NONE',  ( -14.87918228200000037, 1415.865102022439942, 212.9009079454490063 ) ) ;
#80030=CARTESIAN_POINT ( 'NONE',  ( 11.27336394452900059, 1433.557839144309810, 225.8166928899180164 ) ) ;
#80035=CARTESIAN_POINT ( 'NONE',  ( -2.145980225789999807, 1431.918816440389946, 217.3940193458890064 ) ) ;
#80042=CARTESIAN_POINT ( 'NONE',  ( 11.41327087716770095, 1427.619034137559765, 209.6360973194659891 ) ) ;
#80047=CARTESIAN_POINT ( 'NONE',  ( -2.075886983448210099, 1496.000771925150048, 196.9582277030409898 ) ) ;
#80061=CARTESIAN_POINT ( 'NONE',  ( -2.832179855692609660, 1497.533054541979936, 201.1364361656100073 ) ) ;
#80064=CARTESIAN_POINT ( 'NONE',  ( 11.86100282799569960, 1492.894947744830006, 212.5846961511890072 ) ) ;
#80068=EDGE_CURVE ( 'NONE', #508, #6446, #3700, .T. ) ;
#80069=DIRECTION ( 'NONE',  ( -1.000000000000000000, -2.249639673992789970E-32, -1.224646799147350002E-16 ) ) ;
#80071=CARTESIAN_POINT ( 'NONE',  ( 3.584503077479999966, 1486.500511906190013, 219.3043361389989911 ) ) ;
#80078=CARTESIAN_POINT ( 'NONE',  ( -19.74860284620000073, 1465.132576429690062, 209.4730770639620232 ) ) ;
#80083=CARTESIAN_POINT ( 'NONE',  ( 10.50975973408020003, 1452.933536048200040, 210.5056026378560148 ) ) ;
#80084=CARTESIAN_POINT ( 'NONE',  ( 5.877311519840000997, 1423.581874179079932, 194.6993958404989939 ) ) ;
#80087=CARTESIAN_POINT ( 'NONE',  ( 5.650554513050000338, 1452.063338381489984, 211.4905750950089782 ) ) ;
#80089=CARTESIAN_POINT ( 'NONE',  ( 2.487924132557410406, 1509.038643261319976, 213.6090950281819971 ) ) ;
#80101=VERTEX_POINT ( 'NONE', #87031 ) ;
#80103=CARTESIAN_POINT ( 'NONE',  ( -3.726340750997230167, 1508.413954212639737, 220.4799730696009874 ) ) ;
#80104=CARTESIAN_POINT ( 'NONE',  ( 7.745985074145769644, 1500.304699407309954, 200.5303357369510024 ) ) ;
#80106=CARTESIAN_POINT ( 'NONE',  ( -5.992196956094850258, 1469.346592943629958, 217.7944395441180063 ) ) ;
#80110=CARTESIAN_POINT ( 'NONE',  ( -4.818089418980000538, 1474.858188511989965, 199.5909791398490256 ) ) ;
#80112=CARTESIAN_POINT ( 'NONE',  ( 8.436189838809218244, 1424.545028496175973, 195.7325651230689232 ) ) ;
#80113=CARTESIAN_POINT ( 'NONE',  ( -13.43985408640000045, 1503.346475151690129, 208.6824759411649950 ) ) ;
#80114=CARTESIAN_POINT ( 'NONE',  ( 10.14614976752910103, 1469.287792262710127, 204.1824843846119961 ) ) ;
#80115=CARTESIAN_POINT ( 'NONE',  ( 11.85624328898539837, 1421.937062395870043, 207.3014288908249796 ) ) ;
#80123=CARTESIAN_POINT ( 'NONE',  ( 3.756915432050000003, 1505.735347371189846, 220.9097465364990001 ) ) ;
#80125=CARTESIAN_POINT ( 'NONE',  ( -15.10167272650000037, 1416.016604972820005, 212.2622663138990049 ) ) ;
#80126=CARTESIAN_POINT ( 'NONE',  ( -16.85518942986550073, 1419.928483354570062, 208.4319138966170044 ) ) ;
#80128=CARTESIAN_POINT ( 'NONE',  ( -17.08097489138819824, 1418.110424922289894, 204.4848448838540094 ) ) ;
#80136=CARTESIAN_POINT ( 'NONE',  ( 6.992116644224409150, 1458.468605612649981, 201.2966203680600188 ) ) ;
#80139=CARTESIAN_POINT ( 'NONE',  ( -3.410174724169999561, 1476.067642852090103, 219.2827967179989912 ) ) ;
#80150=CARTESIAN_POINT ( 'NONE',  ( -14.80628304904369941, 1417.712450806070137, 203.2308112443149923 ) ) ;
#80153=CARTESIAN_POINT ( 'NONE',  ( -16.76688489720000064, 1417.005534796029906, 207.9255659622089922 ) ) ;
#80165=CARTESIAN_POINT ( 'NONE',  ( -13.30990274189880118, 1508.450031501719877, 209.7671136656329907 ) ) ;
#80168=CARTESIAN_POINT ( 'NONE',  ( -11.83167355530729914, 1481.599286403459928, 209.9607897767780003 ) ) ;
#80171=EDGE_CURVE ( 'NONE', #35203, #84750, #55117, .T. ) ;
#80180=CARTESIAN_POINT ( 'NONE',  ( -9.234134023826198856, 1461.205490114660051, 206.1827678865119822 ) ) ;
#80181=CARTESIAN_POINT ( 'NONE',  ( 4.328507561560000383, 1515.100736413590084, 208.0459478947190064 ) ) ;
#80187=AXIS2_PLACEMENT_3D ( 'NONE', #35299, #17361, #10095 ) ;
#80192=CARTESIAN_POINT ( 'NONE',  ( 18.91865458690000068, 1456.348387323389943, 200.2117427500890017 ) ) ;
#80198=CARTESIAN_POINT ( 'NONE',  ( 2201.413669186790685, 11221.53578756870047, -1523.112345774690311 ) ) ;
#80200=CARTESIAN_POINT ( 'NONE',  ( 4.261736551907978843, 1515.372048949687269, 206.7917118349798784 ) ) ;
#80204=EDGE_CURVE ( 'NONE', #104137, #16269, #77694, .T. ) ;
#80206=CARTESIAN_POINT ( 'NONE',  ( -13.13304581337124333, 1421.347500487118850, 210.6408966550871185 ) ) ;
#80213=ADVANCED_FACE ( 'NONE', ( #72459 ), #17422, .T. ) ;
#80218=EDGE_CURVE ( 'NONE', #60042, #38113, #44311, .T. ) ;
#80220=CARTESIAN_POINT ( 'NONE',  ( 0.8374757675929990208, 1467.465564401289839, 219.8067306195990227 ) ) ;
#80222=CARTESIAN_POINT ( 'NONE',  ( 10.18158772832410008, 1482.093709488619879, 212.1941923381180004 ) ) ;
#80226=EDGE_LOOP ( 'NONE', ( #17739, #29387, #44556 ) ) ;
#80227=CARTESIAN_POINT ( 'NONE',  ( 18.68390456929999743, 1457.534965338390066, 220.6831945507989872 ) ) ;
#80238=CARTESIAN_POINT ( 'NONE',  ( 10.90118902510000076, 1461.578585159090153, 210.3785431609790066 ) ) ;
#80242=CARTESIAN_POINT ( 'NONE',  ( 2.541857501799999586, 1464.337513799189992, 199.6147521953589887 ) ) ;
#80244=EDGE_CURVE ( 'NONE', #39044, #45555, #26396, .T. ) ;
#80245=ORIENTED_EDGE ( 'NONE', *, *, #7727, .F. ) ;
#80250=ORIENTED_EDGE ( 'NONE', *, *, #47520, .T. ) ;
#80253=CARTESIAN_POINT ( 'NONE',  ( -17.96992599225091425, 1508.456902066601742, 211.9348791936326108 ) ) ;
#80255=CARTESIAN_POINT ( 'NONE',  ( 8.269201957289999072, 1502.749105916489953, 209.6145118388120068 ) ) ;
#80259=DIRECTION ( 'NONE',  ( 0.9989904502035610312, 0.04492303273871367519, 3.913620833796736061E-05 ) ) ;
#80265=VECTOR ( 'NONE', #102348, 1000.000000000000114 ) ;
#80271=VECTOR ( 'NONE', #60880, 1000.000000000000000 ) ;
#80274=CARTESIAN_POINT ( 'NONE',  ( -11.53044373018859758, 1482.676277524829857, 206.1452238863429898 ) ) ;
#80275=CARTESIAN_POINT ( 'NONE',  ( -2.825231993049800217, 1483.605131848210021, 198.8324855003439779 ) ) ;
#80292=CARTESIAN_POINT ( 'NONE',  ( -1.081422847559999845, 1515.099766759590011, 213.4503789145389874 ) ) ;
#80296=CARTESIAN_POINT ( 'NONE',  ( -0.3263425942319403417, 1463.534437392499967, 199.3349841275349945 ) ) ;
#80297=CARTESIAN_POINT ( 'NONE',  ( 21.10389824529999814, 1496.766845313890144, 207.9755595194390025 ) ) ;
#80299=CARTESIAN_POINT ( 'NONE',  ( 3.238872246299508095, 1446.101400423860468, 200.2539368609401151 ) ) ;
#80301=CARTESIAN_POINT ( 'NONE',  ( -15.89684887006662883, 1415.918796183675340, 209.5438883029932242 ) ) ;
#80302=CARTESIAN_POINT ( 'NONE',  ( 2.039270112060000528, 1507.500700221690067, 220.6757736221989887 ) ) ;
#80304=ORIENTED_EDGE ( 'NONE', *, *, #6359, .F. ) ;
#80307=CARTESIAN_POINT ( 'NONE',  ( 5.652561691250400422, 1467.010946599490126, 199.8954101620430208 ) ) ;
#80315=CARTESIAN_POINT ( 'NONE',  ( 12.22153682284019993, 1491.665661494050028, 207.6766598159610169 ) ) ;
#80320=VECTOR ( 'NONE', #41594, 1000.000000000000000 ) ;
#80325=CARTESIAN_POINT ( 'NONE',  ( -11.37608146696432954, 1501.391524824338603, 207.8658177168534564 ) ) ;
#80327=CARTESIAN_POINT ( 'NONE',  ( -7.593205020690000140, 1511.472651697490164, 213.8751816602289750 ) ) ;
#80334=CARTESIAN_POINT ( 'NONE',  ( 7.768668303840000178, 1424.631498856950202, 211.9127687528989838 ) ) ;
#80335=CARTESIAN_POINT ( 'NONE',  ( -12.04602610249999906, 1481.198043686990104, 227.9689298191989622 ) ) ;
#80342=EDGE_LOOP ( 'NONE', ( #59461, #64003, #15332, #47305 ) ) ;
#80352=CARTESIAN_POINT ( 'NONE',  ( -1.551136391885070021, 1463.265703726430047, 199.4650954087569801 ) ) ;
#80365=EDGE_CURVE ( 'NONE', #101100, #42035, #76853, .T. ) ;
#80366=CARTESIAN_POINT ( 'NONE',  ( -3.201475593029999622, 1454.788669051489933, 199.8827623000489666 ) ) ;
#80381=ORIENTED_EDGE ( 'NONE', *, *, #78085, .T. ) ;
#80394=CARTESIAN_POINT ( 'NONE',  ( 14.53924085489259888, 1427.225259935240274, 198.3454325463169994 ) ) ;
#80404=CARTESIAN_POINT ( 'NONE',  ( -2.805169331900000174, 1430.372835222990034, 201.2596692449290003 ) ) ;
#80405=CARTESIAN_POINT ( 'NONE',  ( -2.847678236428970333, 1430.845636561999981, 201.2564352187889938 ) ) ;
#80410=B_SPLINE_CURVE_WITH_KNOTS ( 'NONE', 5,
 ( #20190, #26387, #54388, #88521, #94703, #9588 ),
 .UNSPECIFIED., .F., .F.,
 ( 6, 6 ),
 ( 0.000000000000000000, 1.000000000000000000 ),
 .UNSPECIFIED. ) ;
#80413=CARTESIAN_POINT ( 'NONE',  ( 10.04317674107989156, 1459.686705906630550, 204.8127587888380958 ) ) ;
#80414=CARTESIAN_POINT ( 'NONE',  ( 10.34497362454819935, 1469.890123644820051, 207.2997660916290101 ) ) ;
#80417=CARTESIAN_POINT ( 'NONE',  ( 10.02421119480000122, 1480.534221758890226, 205.8829018067289951 ) ) ;
#80418=EDGE_LOOP ( 'NONE', ( #84104, #26042, #97042, #22362 ) ) ;
#80420=CARTESIAN_POINT ( 'NONE',  ( 4.369470536992099419, 1486.409411101999922, 202.3252857625509762 ) ) ;
#80424=CARTESIAN_POINT ( 'NONE',  ( -0.3697322172690010178, 1443.791874737389890, 218.1763052592289966 ) ) ;
#80426=CARTESIAN_POINT ( 'NONE',  ( 14.46805569519750101, 1471.430981385289897, 194.8600923975780006 ) ) ;
#80429=CARTESIAN_POINT ( 'NONE',  ( -2.301610763810779670, 1464.951938263800002, 198.3549737183319905 ) ) ;
#80431=CARTESIAN_POINT ( 'NONE',  ( 4.989613516749999533, 1487.671035670790161, 198.1975016566989893 ) ) ;
#80433=CARTESIAN_POINT ( 'NONE',  ( -10.08152180407089915, 1472.386940315740048, 210.5255569266109887 ) ) ;
#80436=CARTESIAN_POINT ( 'NONE',  ( -15.33800405639999909, 1508.551704408389924, 214.6490336124689975 ) ) ;
#80447=CARTESIAN_POINT ( 'NONE',  ( -10.22681497006489870, 1488.677241974470007, 215.7752924027969925 ) ) ;
#80448=CARTESIAN_POINT ( 'NONE',  ( -18.32377916267250129, 1464.077737519419998, 217.4721398674979866 ) ) ;
#80459=CARTESIAN_POINT ( 'NONE',  ( -20.70043371970000123, 1486.933533050689903, 208.1069901901390153 ) ) ;
#80470=CARTESIAN_POINT ( 'NONE',  ( -0.08387812424052221161, 1515.158224561690076, 213.4488481431200171 ) ) ;
#80475=ORIENTED_EDGE ( 'NONE', *, *, #34318, .F. ) ;
#80478=CARTESIAN_POINT ( 'NONE',  ( -12.04603955804210003, 1481.197944389760096, 227.9689156426159684 ) ) ;
#80480=CARTESIAN_POINT ( 'NONE',  ( 7.468327728180000236, 1422.304606718539844, 195.6660984653989885 ) ) ;
#80489=CARTESIAN_POINT ( 'NONE',  ( -9.519358615130000700, 1460.477013596890174, 210.7621351733390043 ) ) ;
#80496=ORIENTED_EDGE ( 'NONE', *, *, #2116, .F. ) ;
#80503=B_SPLINE_CURVE_WITH_KNOTS ( 'NONE', 5,
 ( #46586, #105375, #71814, #86909, #54445, #46035 ),
 .UNSPECIFIED., .F., .F.,
 ( 6, 6 ),
 ( 0.000000000000000000, 1.000000000000000000 ),
 .UNSPECIFIED. ) ;
#80505=CARTESIAN_POINT ( 'NONE',  ( -0.7302202251785760989, 1496.394952593959943, 221.4547034809050103 ) ) ;
#80509=CARTESIAN_POINT ( 'NONE',  ( -9.602934085884299975, 1440.348741234980025, 206.2393590046850136 ) ) ;
#80513=CARTESIAN_POINT ( 'NONE',  ( 8.701161615177460007, 1436.141447764929808, 208.2918654964580014 ) ) ;
#80518=CARTESIAN_POINT ( 'NONE',  ( 2.609390164300539716, 1466.696228754160074, 219.8662591647770057 ) ) ;
#80542=CARTESIAN_POINT ( 'NONE',  ( 10.93233376569999926, 1490.536113732890044, 207.1036721549689901 ) ) ;
#80548=CARTESIAN_POINT ( 'NONE',  ( -17.25861218780000073, 1417.514782456119974, 207.1361538078189994 ) ) ;
#80552=CARTESIAN_POINT ( 'NONE',  ( 18.87853829029999986, 1458.344553362990155, 213.8102309971890236 ) ) ;
#80557=LINE ( 'NONE', #2770, #14666 ) ;
#80558=B_SPLINE_SURFACE_WITH_KNOTS ( 'NONE', 5, 5, ( 
 ( #46356, #80489, #70457, #28425, #78838, #87798 ),
 ( #45249, #104578, #96742, #54752, #27314, #105701 ),
 ( #53089, #97275, #63171, #53653, #105135, #71014 ),
 ( #11625, #88882, #37937, #12166, #9962, #61495 ),
 ( #95625, #54208, #10517, #44691, #27873, #11082 ),
 ( #79936, #62054, #2699, #45803, #36824, #3252 ),
 ( #37379, #48548, #47438, #5423, #106770, #4337 ),
 ( #21647, #98375, #55855, #81562, #98922, #22192 ),
 ( #39581, #82685, #100020, #91073, #83232, #73185 ),
 ( #56390, #14906, #73753, #55299, #4865, #89974 ),
 ( #31716, #90522, #56944, #30626, #64814, #66463 ),
 ( #13248, #65902, #23312, #13798, #107876, #31164 ),
 ( #14356, #74305, #49097, #57505, #6523, #100572 ),
 ( #40675, #65354, #30061, #74849, #39008, #47984 ),
 ( #5975, #38468, #91630, #40120, #82121, #107330 ) ),
 .UNSPECIFIED., .F., .F., .F.,
 ( 6, 3, 3, 3, 6 ),
 ( 6, 6 ),
 ( 13.48959176149999983, 23.65970578370000155, 28.35476274839999888, 30.70229123080000022, 33.04981971320000156 ),
 ( 0.000000000000000000, 2.000000000000000000 ),
 .UNSPECIFIED. ) ;
#80559=DIRECTION ( 'NONE',  ( -0.06270903725022231034, 1.833354768615425389E-16, 0.9980318515193542517 ) ) ;
#80562=ORIENTED_EDGE ( 'NONE', *, *, #23436, .T. ) ;
#80571=CARTESIAN_POINT ( 'NONE',  ( -18.80014180510890043, 1505.319237130929878, 222.5373109737209916 ) ) ;
#80576=ORIENTED_EDGE ( 'NONE', *, *, #50827, .T. ) ;
#80580=CARTESIAN_POINT ( 'NONE',  ( 4.836838691807330726, 1508.551704408389924, 205.7765624394519932 ) ) ;
#80583=CARTESIAN_POINT ( 'NONE',  ( -9.299400257574959028, 1446.922142132390036, 190.6945004022419994 ) ) ;
#80589=CARTESIAN_POINT ( 'NONE',  ( 11.36216713388179933, 1503.110266152410077, 211.0233809544849919 ) ) ;
#80590=CARTESIAN_POINT ( 'NONE',  ( -2.418973636230000057, 1431.127469431690088, 217.1544448978289950 ) ) ;
#80592=CARTESIAN_POINT ( 'NONE',  ( -10.08245609418620070, 1472.804170826050040, 207.2994808592069944 ) ) ;
#80598=CARTESIAN_POINT ( 'NONE',  ( 10.98558675269530127, 1490.788211858329987, 209.4256117797519892 ) ) ;
#80599=ORIENTED_EDGE ( 'NONE', *, *, #42824, .F. ) ;
#80603=CARTESIAN_POINT ( 'NONE',  ( -1.878723365004049795, 1496.058737867240097, 196.9227348079259912 ) ) ;
#80618=CARTESIAN_POINT ( 'NONE',  ( 1.791819983609999944, 1496.978182980090196, 196.8421287543990275 ) ) ;
#80621=ORIENTED_EDGE ( 'NONE', *, *, #8529, .F. ) ;
#80629=CARTESIAN_POINT ( 'NONE',  ( 3.394586495530000025, 1484.752177868989975, 220.4731791295990035 ) ) ;
#80640=CARTESIAN_POINT ( 'NONE',  ( 5.583139218519999503, 1422.549100278879905, 194.7453484342989896 ) ) ;
#80643=CARTESIAN_POINT ( 'NONE',  ( -3.145950129948163809, 1420.252270208513437, 194.0299402294517392 ) ) ;
#80659=CARTESIAN_POINT ( 'NONE',  ( -10.50209100468410028, 1480.194371605160086, 208.4668248273180211 ) ) ;
#80660=CARTESIAN_POINT ( 'NONE',  ( -2.168256794737599691, 1508.371295004969852, 220.6985498477429815 ) ) ;
#80661=CARTESIAN_POINT ( 'NONE',  ( 7.937475080669701200, 1499.382778073400004, 200.5719245896989946 ) ) ;
#80663=CARTESIAN_POINT ( 'NONE',  ( -7.723409503819699928, 1470.257994933900136, 215.9036483672630027 ) ) ;
#80665=CARTESIAN_POINT ( 'NONE',  ( 12.17174069520000046, 1420.444189216879977, 199.8097663552590006 ) ) ;
#80670=CARTESIAN_POINT ( 'NONE',  ( -13.52030549040000018, 1503.072261434289885, 208.8037810841129840 ) ) ;
#80674=CARTESIAN_POINT ( 'NONE',  ( -9.637203692943991484, 1440.299518560640081, 206.3693651664740116 ) ) ;
#80680=CARTESIAN_POINT ( 'NONE',  ( 4.151873366180000247, 1507.235155069190114, 220.0634631044989931 ) ) ;
#80681=CARTESIAN_POINT ( 'NONE',  ( -14.92217863770000008, 1415.738355314559840, 212.2123080183590105 ) ) ;
#80682=CARTESIAN_POINT ( 'NONE',  ( -9.806574738260000146, 1463.377913006889912, 203.8363535297289957 ) ) ;
#80683=EDGE_LOOP ( 'NONE', ( #1913, #11554, #109785, #249 ) ) ;
#80684=CARTESIAN_POINT ( 'NONE',  ( 3.770851430420000039, 1430.288814966790142, 217.3901795606089991 ) ) ;
#80687=CARTESIAN_POINT ( 'NONE',  ( -16.10814125329999769, 1416.492096055970023, 209.3578209456409809 ) ) ;
#80688=CARTESIAN_POINT ( 'NONE',  ( -19.68223018519999812, 1464.931511052589940, 211.0302758615490006 ) ) ;
#80696=CARTESIAN_POINT ( 'NONE',  ( -4.456636540849999939, 1476.515883157990174, 218.9574462611590207 ) ) ;
#80711=CARTESIAN_POINT ( 'NONE',  ( -4.045211208830000515, 1515.528099018290050, 207.6335164720289868 ) ) ;
#80713=CARTESIAN_POINT ( 'NONE',  ( 2.779282467552740332, 1456.300107729789943, 219.3762139804350113 ) ) ;
#80721=CARTESIAN_POINT ( 'NONE',  ( -0.5199289187719989824, 1463.450241312990102, 202.1355596697889894 ) ) ;
#80724=CARTESIAN_POINT ( 'NONE',  ( -4.378216884482949212, 1453.707746088449994, 199.6107954155660025 ) ) ;
#80729=CARTESIAN_POINT ( 'NONE',  ( -12.12611261273299945, 1490.951129191179916, 207.2692690533270081 ) ) ;
#80730=CARTESIAN_POINT ( 'NONE',  ( -4.672438357553319932, 1508.551704408389924, 205.4176553271170178 ) ) ;
#80738=VECTOR ( 'NONE', #27479, 1000.000000000000000 ) ;
#80739=CARTESIAN_POINT ( 'NONE',  ( -5.530579386980000400, 1496.346118937389974, 218.9093369348890121 ) ) ;
#80744=CARTESIAN_POINT ( 'NONE',  ( -18.31098522441029885, 1464.870751162060060, 217.5849428054170005 ) ) ;
#80759=CARTESIAN_POINT ( 'NONE',  ( -10.34903246276065758, 1422.477322477220014, 210.6474012835178371 ) ) ;
#80765=CARTESIAN_POINT ( 'NONE',  ( 0.3803298753218480321, 1485.753653569830021, 220.9969941478449869 ) ) ;
#80771=B_SPLINE_CURVE_WITH_KNOTS ( 'NONE', 3,
 ( #72548, #45154, #106679, #37289, #47337, #12633, #81465, #29970, #105041, #55208, #37838, #96644, #64162, #105602, #55767, #19913, #63617, #98280, #79847, #10980, #63081, #22095, #38915, #97180, #54662, #3708, #54114, #73097, #46266, #80394, #72024, #106140, #97734, #21005, #89337, #107236, #79294, #2605, #36729, #46810, #6981, #15366, #41132, #84233, #39489, #22642, #92634, #100488, #90422 ),
 .UNSPECIFIED., .F., .F.,
 ( 4, 3, 3, 3, 3, 3, 3, 3, 3, 3, 3, 3, 3, 3, 3, 3, 4 ),
 ( -7.217395425439999457, -6.314159096166340746, -5.426996328170729633, -4.536566390866929588, -3.643034527830809832, -2.730152093685779491, -1.829978413125148862, -0.9107416021879179979, 0.008495208749310201313, 0.9096077358356460252, 1.811265860083839385, 2.713151777285197852, 3.614808793634290751, 4.515455451585719260, 5.414687769663739658, 6.316041597551869557, 7.217395425439999457 ),
 .UNSPECIFIED. ) ;
#80772=CARTESIAN_POINT ( 'NONE',  ( -1.231622111079999859, 1468.763012560089919, 219.2115919040990093 ) ) ;
#80774=CARTESIAN_POINT ( 'NONE',  ( 10.56018849299529982, 1481.177537964639896, 213.4278321560559846 ) ) ;
#80775=EDGE_CURVE ( 'NONE', #25916, #65578, #13531, .T. ) ;
#80778=CARTESIAN_POINT ( 'NONE',  ( -7.179517906949999251, 1480.902174850589972, 207.6226633918490165 ) ) ;
#80781=CARTESIAN_POINT ( 'NONE',  ( -1.173443483158729927, 1431.768907133609900, 200.7987716776540026 ) ) ;
#80801=CARTESIAN_POINT ( 'NONE',  ( 11.51338207723369855, 1478.865430962250002, 206.7896514733459981 ) ) ;
#80802=ORIENTED_EDGE ( 'NONE', *, *, #35867, .T. ) ;
#80808=CARTESIAN_POINT ( 'NONE',  ( -9.307164086263318481, 1437.573555850379989, 212.3980636621099904 ) ) ;
#80826=CARTESIAN_POINT ( 'NONE',  ( -15.43894024600000137, 1415.776528789690246, 207.8411306001490004 ) ) ;
#80832=CARTESIAN_POINT ( 'NONE',  ( 6.594884990749999787, 1463.733222497789939, 209.8009783769319938 ) ) ;
#80834=ORIENTED_EDGE ( 'NONE', *, *, #32316, .T. ) ;
#80837=CARTESIAN_POINT ( 'NONE',  ( -1.842962231260000028, 1515.551704408389924, 213.1059277140590211 ) ) ;
#80844=CIRCLE ( 'NONE', #20009, 15.41148139973879871 ) ;
#80845=CARTESIAN_POINT ( 'NONE',  ( -6.608531157176709137, 1439.954310736166690, 203.3674198005971618 ) ) ;
#80846=CARTESIAN_POINT ( 'NONE',  ( -4.963305069829999638, 1458.663087589289944, 218.6479516874489946 ) ) ;
#80847=CARTESIAN_POINT ( 'NONE',  ( -6.632177051280000235, 1428.092653318189832, 204.0245593685589824 ) ) ;
#80848=ADVANCED_FACE ( 'NONE', ( #2246 ), #50029, .T. ) ;
#80852=CARTESIAN_POINT ( 'NONE',  ( -4.326992699989999913, 1515.158586642889986, 209.1218459616989946 ) ) ;
#80853=B_SPLINE_CURVE_WITH_KNOTS ( 'NONE', 3,
 ( #25762, #59961, #94076, #87351, #44255, #68921, #90082, #54324, #3918, #13366, #36933, #4454, #21202 ),
 .UNSPECIFIED., .F., .F.,
 ( 4, 3, 3, 3, 4 ),
 ( -1.727219771889999977, -0.7951722241532679369, 0.1344887764924689311, 1.059669685035710129, 1.727219771889999977 ),
 .UNSPECIFIED. ) ;
#80854=ORIENTED_EDGE ( 'NONE', *, *, #95674, .F. ) ;
#80856=ADVANCED_FACE ( 'NONE', ( #104115 ), #14196, .T. ) ;
#80857=CARTESIAN_POINT ( 'NONE',  ( 6.489845843996670638, 1466.368330838150086, 201.4744493398009979 ) ) ;
#80860=CARTESIAN_POINT ( 'NONE',  ( -8.697287760260000056, 1440.006335262490211, 206.1599773368889714 ) ) ;
#80865=CARTESIAN_POINT ( 'NONE',  ( -11.27425270319999839, 1482.889162177290018, 205.2544580881489935 ) ) ;
#80872=CARTESIAN_POINT ( 'NONE',  ( -11.33324210258937192, 1502.232704771361114, 207.2803833977290253 ) ) ;
#80882=CARTESIAN_POINT ( 'NONE',  ( 8.439944554000000210, 1428.238409027789885, 213.1498827361689905 ) ) ;
#80883=CARTESIAN_POINT ( 'NONE',  ( 4.803837674189999518, 1471.771474222590086, 187.6888395837989947 ) ) ;
#80899=CARTESIAN_POINT ( 'NONE',  ( -2.289647404633549765, 1464.762954016199956, 198.7769187872700059 ) ) ;
#80912=ORIENTED_EDGE ( 'NONE', *, *, #21681, .T. ) ;
#80921=EDGE_CURVE ( 'NONE', #94111, #101374, #16306, .T. ) ;
#80934=EDGE_CURVE ( 'NONE', #38761, #87765, #104386, .T. ) ;
#80954=CARTESIAN_POINT ( 'NONE',  ( 12.25490649660000031, 1421.424738529230126, 204.6606925453189945 ) ) ;
#80958=CARTESIAN_POINT ( 'NONE',  ( 10.00951688712369858, 1468.852972450649986, 208.4479931420239893 ) ) ;
#80961=CARTESIAN_POINT ( 'NONE',  ( 10.08517028152789941, 1480.579361189179963, 206.0651545076909770 ) ) ;
#80962=EDGE_LOOP ( 'NONE', ( #13418, #106329, #70149, #34655 ) ) ;
#80966=CARTESIAN_POINT ( 'NONE',  ( 7.926223792202339524, 1423.719494923044977, 195.8478123068922798 ) ) ;
#80967=CARTESIAN_POINT ( 'NONE',  ( 1.101591607640000081, 1442.758995474489893, 218.3133920886989756 ) ) ;
#80978=ORIENTED_EDGE ( 'NONE', *, *, #104372, .T. ) ;
#80980=CARTESIAN_POINT ( 'NONE',  ( -13.27855961070000212, 1508.487312425190112, 216.9533382897689933 ) ) ;
#80984=CARTESIAN_POINT ( 'NONE',  ( -1.726834413310000205, 1484.334256824789918, 198.5613324875990315 ) ) ;
#80989=CARTESIAN_POINT ( 'NONE',  ( 2.461360751019160187, 1493.777257040230097, 219.9857987593770190 ) ) ;
#80991=CARTESIAN_POINT ( 'NONE',  ( 9.738317565070000015, 1493.400072498489862, 188.2659980885989910 ) ) ;
#80992=CARTESIAN_POINT ( 'NONE',  ( -15.39283239035830064, 1415.677402202039957, 209.2531991726660294 ) ) ;
#80995=CARTESIAN_POINT ( 'NONE',  ( -18.51973145710680058, 1443.522805491569898, 212.3835520930680048 ) ) ;
#80996=EDGE_LOOP ( 'NONE', ( #4720, #1909, #53135, #93627 ) ) ;
#81002=CARTESIAN_POINT ( 'NONE',  ( 7.294045558785978045, 1423.346842215470815, 213.7896502874405655 ) ) ;
#81007=CARTESIAN_POINT ( 'NONE',  ( -1.031155851060000073, 1488.425564119090041, 217.1473006051089669 ) ) ;
#81011=CARTESIAN_POINT ( 'NONE',  ( 0.05006135363680530581, 1515.158685764440179, 213.4488360661000002 ) ) ;
#81014=CARTESIAN_POINT ( 'NONE',  ( -10.79334919306910123, 1480.196592731939973, 213.7852440063740289 ) ) ;
#81017=ORIENTED_EDGE ( 'NONE', *, *, #29171, .T. ) ;
#81019=CARTESIAN_POINT ( 'NONE',  ( -11.36958083090000038, 1503.847187927490268, 207.0750579214790150 ) ) ;
#81020=CARTESIAN_POINT ( 'NONE',  ( -5.768266513520000416, 1492.234223000290058, 185.8590593905989863 ) ) ;
#81022=CARTESIAN_POINT ( 'NONE',  ( 8.028494635650000433, 1421.573180670790180, 196.0255996755989827 ) ) ;
#81027=CARTESIAN_POINT ( 'NONE',  ( 0.9885189933060011258, 1456.680325442589947, 199.2944122769889930 ) ) ;
#81028=CARTESIAN_POINT ( 'NONE',  ( -4.082704913390346135, 1515.071394843999087, 205.5354683776590434 ) ) ;
#81033=EDGE_LOOP ( 'NONE', ( #29521, #85534, #106967, #97450 ) ) ;
#81034=VERTEX_POINT ( 'NONE', #66556 ) ;
#81037=DIRECTION ( 'NONE',  ( 0.9996573249755569268, 0.02617694830788839730, 1.176140869340470334E-16 ) ) ;
#81040=ORIENTED_EDGE ( 'NONE', *, *, #94766, .T. ) ;
#81042=CARTESIAN_POINT ( 'NONE',  ( 6.287349243829999601, 1473.446183115890108, 218.1771757008089878 ) ) ;
#81047=CARTESIAN_POINT ( 'NONE',  ( 8.367692836712059545, 1436.613519496920162, 207.0421242491720193 ) ) ;
#81052=CARTESIAN_POINT ( 'NONE',  ( 11.11707036908040003, 1471.687204444999907, 211.7794637602030150 ) ) ;
#81053=ADVANCED_FACE ( 'NONE', ( #67650 ), #91095, .T. ) ;
#81058=CARTESIAN_POINT ( 'NONE',  ( 6.749186742440000053, 1455.205488045889979, 217.3783194977189908 ) ) ;
#81068=EDGE_CURVE ( 'NONE', #14911, #108882, #19268, .T. ) ;
#81083=CARTESIAN_POINT ( 'NONE',  ( -3.152270375085599596, 1474.954422185709745, 198.1306180807430053 ) ) ;
#81090=CARTESIAN_POINT ( 'NONE',  ( -0.08399573354635679612, 1455.696542369420058, 198.5840329839000162 ) ) ;
#81094=CARTESIAN_POINT ( 'NONE',  ( -1.531858734065989602E-13, 1515.051704408389924, 205.2922258481490303 ) ) ;
#81097=EDGE_CURVE ( 'NONE', #51752, #38761, #51054, .T. ) ;
#81098=CARTESIAN_POINT ( 'NONE',  ( -2.487935123034409557, 1508.603735228351297, 213.8522301342857475 ) ) ;
#81102=CARTESIAN_POINT ( 'NONE',  ( 12.18686852027619949, 1501.408139047200166, 211.6432815866139947 ) ) ;
#81103=EDGE_CURVE ( 'NONE', #73081, #23187, #89708, .T. ) ;
#81104=LINE ( 'NONE', #38546, #21667 ) ;
#81107=CARTESIAN_POINT ( 'NONE',  ( -4.678978663885700051, 1508.551704408389924, 205.0635906264530206 ) ) ;
#81108=DIRECTION ( 'NONE',  ( -0.4544580288560248760, -1.636314548565651616E-16, -0.8907681516580486791 ) ) ;
#81115=CARTESIAN_POINT ( 'NONE',  ( -3.151263210079999766, 1476.308150043789965, 199.2625576691089861 ) ) ;
#81117=ORIENTED_EDGE ( 'NONE', *, *, #89477, .T. ) ;
#81118=CARTESIAN_POINT ( 'NONE',  ( 18.32583560018409941, 1473.764173505169765, 194.8973815002569836 ) ) ;
#81123=CARTESIAN_POINT ( 'NONE',  ( -5.302704825520000220, 1464.205378554289837, 199.9536502662190003 ) ) ;
#81125=CARTESIAN_POINT ( 'NONE',  ( 20.84639163829999831, 1494.459648749690132, 206.0923896281290126 ) ) ;
#81136=EDGE_CURVE ( 'NONE', #103262, #108726, #87237, .T. ) ;
#81157=CARTESIAN_POINT ( 'NONE',  ( -18.74294524797809913, 1488.344793556559807, 199.7614651361420215 ) ) ;
#81165=CARTESIAN_POINT ( 'NONE',  ( -0.7156643283900009367, 1487.058471442790051, 220.0700283026990007 ) ) ;
#81172=ORIENTED_EDGE ( 'NONE', *, *, #976, .T. ) ;
#81176=ORIENTED_EDGE ( 'NONE', *, *, #65731, .T. ) ;
#81190=ORIENTED_EDGE ( 'NONE', *, *, #49492, .T. ) ;
#81192=CARTESIAN_POINT ( 'NONE',  ( -2.134361597679850231, 1508.551704408389924, 220.0638607491889900 ) ) ;
#81196=CARTESIAN_POINT ( 'NONE',  ( 8.309581502480000381, 1421.353511227099943, 196.1914330872990035 ) ) ;
#81198=DIRECTION ( 'NONE',  ( 0.9824080081115887930, -2.243614313870717968E-31, 0.1867471702549210744 ) ) ;
#81199=DIRECTION ( 'NONE',  ( -0.9054006440294158908, 0.3019905698272229433, 0.2984147609059379924 ) ) ;
#81205=CARTESIAN_POINT ( 'NONE',  ( -9.758464371257050018, 1440.110776583330107, 206.8639830241129971 ) ) ;
#81212=B_SPLINE_SURFACE_WITH_KNOTS ( 'NONE', 5, 5, ( 
 ( #65138, #99806, #6317, #74639, #100376, #15778 ),
 ( #91433, #57307, #14709, #48898, #90867, #98719 ),
 ( #109344, #23661, #66801, #32625, #100902, #39369 ),
 ( #14155, #57844, #49980, #84117, #90310, #7416 ),
 ( #91971, #72983, #73543, #107121, #21979, #56171 ),
 ( #13588, #47776, #107678, #30963, #99252, #48341 ),
 ( #82480, #16494, #31667, #101065, #49596, #65848 ),
 ( #83728, #84280, #41181, #57998, #42281, #68061 ),
 ( #75355, #32771, #7023, #66955, #93227, #24361 ) ),
 .UNSPECIFIED., .F., .F., .F.,
 ( 6, 3, 6 ),
 ( 6, 6 ),
 ( 11.24104702996040039, 18.80012749189999965, 23.52194917210970004 ),
 ( -0.0001008039396122149963, 2.000000000000000000 ),
 .UNSPECIFIED. ) ;
#81215=CARTESIAN_POINT ( 'NONE',  ( -5.976488786809999176, 1464.287555164190053, 199.8460616603990161 ) ) ;
#81219=CARTESIAN_POINT ( 'NONE',  ( -16.41680482819999654, 1416.781978129459958, 208.2739500234559955 ) ) ;
#81220=CARTESIAN_POINT ( 'NONE',  ( -1.611085750247870152, 1429.654024655400008, 199.8738294952200079 ) ) ;
#81234=ADVANCED_FACE ( 'NONE', ( #55818 ), #74137, .T. ) ;
#81236=CARTESIAN_POINT ( 'NONE',  ( -14.38719234011680115, 1417.088620461709979, 203.2501595028660120 ) ) ;
#81243=CARTESIAN_POINT ( 'NONE',  ( 0.8442079999446018279, 1484.559943106105948, 198.4446501219433969 ) ) ;
#81248=CARTESIAN_POINT ( 'NONE',  ( 2.115055681410000332, 1476.785742702189964, 198.5761133783990147 ) ) ;
#81250=CARTESIAN_POINT ( 'NONE',  ( -11.03560576459999965, 1491.884727983489938, 209.0941458228089971 ) ) ;
#81258=CARTESIAN_POINT ( 'NONE',  ( -12.13697616928110001, 1490.926079256330240, 207.3467037448569954 ) ) ;
#81259=CARTESIAN_POINT ( 'NONE',  ( -9.699660872752350116, 1472.030908259890111, 212.1562907213800031 ) ) ;
#81267=CARTESIAN_POINT ( 'NONE',  ( -11.19681733540000046, 1500.043629866090214, 211.1912691597789831 ) ) ;
#81272=CARTESIAN_POINT ( 'NONE',  ( -16.49003115520000051, 1466.602378028289877, 220.8807112456989898 ) ) ;
#81286=CARTESIAN_POINT ( 'NONE',  ( 11.32068957845180002, 1502.651254573290089, 211.1497440136959938 ) ) ;
#81294=CARTESIAN_POINT ( 'NONE',  ( -21.50400446119279962, 1505.467562055609960, 209.6175409707290100 ) ) ;
#81295=CARTESIAN_POINT ( 'NONE',  ( 12.17073512129999990, 1499.730396594889726, 205.6506568158590085 ) ) ;
#81302=CARTESIAN_POINT ( 'NONE',  ( 11.40628762099720106, 1480.472364249699922, 212.2078988420369967 ) ) ;
#81306=ORIENTED_EDGE ( 'NONE', *, *, #29894, .F. ) ;
#81309=EDGE_LOOP ( 'NONE', ( #6386, #515, #85974, #82637 ) ) ;
#81314=CARTESIAN_POINT ( 'NONE',  ( -18.43525369369999822, 1507.707328976990084, 209.4281662339789705 ) ) ;
#81332=CARTESIAN_POINT ( 'NONE',  ( 8.268934410249999090, 1502.576082311989921, 209.2129076204989815 ) ) ;
#81340=B_SPLINE_SURFACE_WITH_KNOTS ( 'NONE', 5, 1, ( 
 ( #54315, #87908 ),
 ( #3360, #106878 ),
 ( #89535, #12269 ),
 ( #64359, #11197 ),
 ( #54857, #20123 ),
 ( #71690, #45361 ) ),
 .UNSPECIFIED., .F., .F., .F.,
 ( 6, 6 ),
 ( 2, 2 ),
 ( 0.000000000000000000, 16.10685270580000150 ),
 ( 0.000000000000000000, 14.00000000000000000 ),
 .UNSPECIFIED. ) ;
#81349=ORIENTED_EDGE ( 'NONE', *, *, #30231, .F. ) ;
#81353=CARTESIAN_POINT ( 'NONE',  ( -20.69303424980000372, 1486.764600954290017, 209.1218459616989946 ) ) ;
#81366=CARTESIAN_POINT ( 'NONE',  ( -1.454938208119999965, 1515.064792882589927, 213.4512947377390049 ) ) ;
#81373=CARTESIAN_POINT ( 'NONE',  ( -2.137141269540000277, 1508.158423200389961, 220.7965104394990021 ) ) ;
#81374=CARTESIAN_POINT ( 'NONE',  ( -4.274333237420000486, 1515.341807516890185, 210.5964949952889924 ) ) ;
#81376=DIRECTION ( 'NONE',  ( -6.922360974429999144E-17, -1.000000000000000000, 2.302693041820029802E-16 ) ) ;
#81387=CIRCLE ( 'NONE', #51045, 0.4999999999999449329 ) ;
#81393=CARTESIAN_POINT ( 'NONE',  ( -13.58621515471660146, 1508.473582053489963, 209.9518858487339799 ) ) ;
#81394=AXIS2_PLACEMENT_3D ( 'NONE', #71351, #79177, #10285 ) ;
#81395=FACE_OUTER_BOUND ( 'NONE', #42704, .T. ) ;
#81399=CARTESIAN_POINT ( 'NONE',  ( -5.183066490639999913, 1453.381677452690155, 200.4630107504189880 ) ) ;
#81401=CARTESIAN_POINT ( 'NONE',  ( 8.051697842710000330, 1428.206416439490113, 213.2401734540090104 ) ) ;
#81402=CARTESIAN_POINT ( 'NONE',  ( 22.24401329409999661, 1475.958617299990010, 209.7631870919539949 ) ) ;
#81404=CARTESIAN_POINT ( 'NONE',  ( -20.14820771579280034, 1418.607677447980222, 207.2578463169909924 ) ) ;
#81407=CARTESIAN_POINT ( 'NONE',  ( 8.810583203269999331, 1453.517925901990111, 213.4503995737389914 ) ) ;
#81415=CARTESIAN_POINT ( 'NONE',  ( -14.93718008229999938, 1416.181292664740113, 212.9156384192889959 ) ) ;
#81439=CARTESIAN_POINT ( 'NONE',  ( -17.61823560201790073, 1508.551704408389924, 211.7175350862160315 ) ) ;
#81455=ORIENTED_EDGE ( 'NONE', *, *, #76651, .T. ) ;
#81465=CARTESIAN_POINT ( 'NONE',  ( 7.600903732925440082, 1425.252121065440178, 192.7969948842710153 ) ) ;
#81477=EDGE_CURVE ( 'NONE', #3936, #42483, #91324, .T. ) ;
#81479=CARTESIAN_POINT ( 'NONE',  ( 4.832616806509603791, 1508.551704408389924, 206.6339108634079196 ) ) ;
#81481=EDGE_CURVE ( 'NONE', #508, #18362, #60375, .T. ) ;
#81482=CARTESIAN_POINT ( 'NONE',  ( 11.09438297129999995, 1422.716151225649810, 205.9069650321689835 ) ) ;
#81483=CARTESIAN_POINT ( 'NONE',  ( -3.202919937201420097, 1497.488146467896513, 198.3026830809020566 ) ) ;
#81486=CARTESIAN_POINT ( 'NONE',  ( -11.00301372470000061, 1492.094802143589959, 210.0154403701209844 ) ) ;
#81490=CARTESIAN_POINT ( 'NONE',  ( 10.37204961533650049, 1480.880553692909871, 207.1848069682540086 ) ) ;
#81494=CARTESIAN_POINT ( 'NONE',  ( 10.95226140456819941, 1461.055140320559985, 208.9723413537100214 ) ) ;
#81495=CARTESIAN_POINT ( 'NONE',  ( 8.637116716612862177, 1424.696483988998125, 195.7776412112969808 ) ) ;
#81496=CARTESIAN_POINT ( 'NONE',  ( 1.940446769709999852, 1443.740569421090186, 217.8448552839390118 ) ) ;
#81505=CARTESIAN_POINT ( 'NONE',  ( -10.15838176937289994, 1472.546283077140060, 209.8695213180610040 ) ) ;
#81508=CARTESIAN_POINT ( 'NONE',  ( -8.809401951759999960, 1508.551704408389924, 218.7286899463289842 ) ) ;
#81509=CARTESIAN_POINT ( 'NONE',  ( 0.000000000000000000, 1414.421228241719973, 209.1218459616989946 ) ) ;
#81510=CARTESIAN_POINT ( 'NONE',  ( 11.37384798555710042, 1470.779892333479893, 208.4801607157270098 ) ) ;
#81515=CARTESIAN_POINT ( 'NONE',  ( -3.286480964850000408, 1456.341185808290220, 218.0120306903490075 ) ) ;
#81516=CARTESIAN_POINT ( 'NONE',  ( 5.312683756866860563, 1493.059111247549936, 218.8466363622630126 ) ) ;
#81519=AXIS2_PLACEMENT_3D ( 'NONE', #28876, #89326, #44580 ) ;
#81537=EDGE_CURVE ( 'NONE', #56028, #96209, #55036, .T. ) ;
#81543=CARTESIAN_POINT ( 'NONE',  ( 0.7597457875069780764, 1515.127202858759802, 213.4496604749319886 ) ) ;
#81545=CARTESIAN_POINT ( 'NONE',  ( -10.54669675879670088, 1479.991597968870110, 214.2917569529570017 ) ) ;
#81550=ORIENTED_EDGE ( 'NONE', *, *, #52057, .F. ) ;
#81552=CARTESIAN_POINT ( 'NONE',  ( -13.31088003390000019, 1503.456607311290099, 208.6977490917149964 ) ) ;
#81553=CARTESIAN_POINT ( 'NONE',  ( 19.49044434509999846, 1499.602757397389723, 221.7314651344989898 ) ) ;
#81562=CARTESIAN_POINT ( 'NONE',  ( -5.584473570009999221, 1458.593347104090071, 217.4064612629990165 ) ) ;
#81573=CARTESIAN_POINT ( 'NONE',  ( -17.64146421497870065, 1419.304501645640130, 207.1873797621490212 ) ) ;
#81581=CARTESIAN_POINT ( 'NONE',  ( 10.70463268489999997, 1472.030523703590006, 213.2176825260490034 ) ) ;
#81591=CARTESIAN_POINT ( 'NONE',  ( -1.272696501052200002, 1467.775668680739955, 220.1607310847500116 ) ) ;
#81598=CARTESIAN_POINT ( 'NONE',  ( 6.202679998688561014, 1439.658092082629764, 216.9645777206339972 ) ) ;
#81622=CARTESIAN_POINT ( 'NONE',  ( -17.73273491259999801, 1417.940993905429877, 206.5463141675389807 ) ) ;
#81625=DIRECTION ( 'NONE',  ( 4.465978680329379737E-17, 1.000000000000000000, -2.349386720892264891E-16 ) ) ;
#81631=CARTESIAN_POINT ( 'NONE',  ( -1.315889753809829976, 1455.200739381179801, 198.6907887078860142 ) ) ;
#81632=CARTESIAN_POINT ( 'NONE',  ( -3.829620113550000315, 1515.551704408389924, 207.0352977830190184 ) ) ;
#81634=CARTESIAN_POINT ( 'NONE',  ( -9.702020572793150777, 1471.556206313400025, 212.0789205537989801 ) ) ;
#81638=CARTESIAN_POINT ( 'NONE',  ( 10.52836328796560039, 1481.199420803890007, 208.2605164816220054 ) ) ;
#81640=CARTESIAN_POINT ( 'NONE',  ( -1.780534836129999965, 1443.660695742489906, 199.9945852240089721 ) ) ;
#81644=CARTESIAN_POINT ( 'NONE',  ( -1.109176384893529876, 1508.551704408389924, 220.0791009952889965 ) ) ;
#81648=CARTESIAN_POINT ( 'NONE',  ( -11.86289009182950061, 1502.090840157799903, 208.8788401476599859 ) ) ;
#81654=CARTESIAN_POINT ( 'NONE',  ( 3.466266129261410089, 1508.551704408389924, 204.3328199221159878 ) ) ;
#81657=CARTESIAN_POINT ( 'NONE',  ( -17.66148560826829694, 1440.150327659670211, 218.7822435725309731 ) ) ;
#81660=CARTESIAN_POINT ( 'NONE',  ( -3.982959079219469789, 1515.551843419029865, 206.2722837986890170 ) ) ;
#81661=CARTESIAN_POINT ( 'NONE',  ( -4.798573010642852132, 1474.699596436941647, 199.5387037236716594 ) ) ;
#81662=CARTESIAN_POINT ( 'NONE',  ( -4.748707946720000628, 1463.075555322190212, 200.5806829759990251 ) ) ;
#81663=ADVANCED_FACE ( 'NONE', ( #72751 ), #64361, .T. ) ;
#81665=CARTESIAN_POINT ( 'NONE',  ( -10.06325851941720018, 1473.086862127829818, 207.3770336094819982 ) ) ;
#81681=CARTESIAN_POINT ( 'NONE',  ( -15.15615661080000187, 1420.466168034640077, 211.8568737882690129 ) ) ;
#81687=EDGE_CURVE ( 'NONE', #73608, #49951, #2660, .T. ) ;
#81690=CARTESIAN_POINT ( 'NONE',  ( -8.747074744635460419, 1447.713388414080100, 212.1118496456160187 ) ) ;
#81696=CARTESIAN_POINT ( 'NONE',  ( 7.105712853721669831, 1424.913842867449830, 213.0229688049089702 ) ) ;
#81700=CARTESIAN_POINT ( 'NONE',  ( -11.82672846260030042, 1491.252350426499788, 206.7221554372329990 ) ) ;
#81704=CARTESIAN_POINT ( 'NONE',  ( -4.637746460722021347, 1378.072810476678342, 214.3830454900369205 ) ) ;
#81713=ORIENTED_EDGE ( 'NONE', *, *, #106862, .T. ) ;
#81721=ADVANCED_FACE ( 'NONE', ( #8274 ), #26841, .T. ) ;
#81724=ORIENTED_EDGE ( 'NONE', *, *, #104372, .F. ) ;
#81730=CARTESIAN_POINT ( 'NONE',  ( 7.150985165824430112, 1483.211489592900080, 218.5460388441480006 ) ) ;
#81734=CARTESIAN_POINT ( 'NONE',  ( -10.70175718777040075, 1481.110708145740091, 208.7148072333299922 ) ) ;
#81735=CARTESIAN_POINT ( 'NONE',  ( -3.208441210349299855, 1508.400043147619954, 220.5739096555420247 ) ) ;
#81736=CARTESIAN_POINT ( 'NONE',  ( 3.240951521948889802, 1499.214374350819980, 198.1680990744349913 ) ) ;
#81740=EDGE_CURVE ( 'NONE', #64216, #45216, #6794, .T. ) ;
#81741=CARTESIAN_POINT ( 'NONE',  ( -3.132370430190279720, 1476.360346537520172, 220.1606225241589812 ) ) ;
#81742=CARTESIAN_POINT ( 'NONE',  ( -8.219322315134521162, 1493.760598851730037, 199.9648169300360223 ) ) ;
#81747=VECTOR ( 'NONE', #75062, 1000.000000000000114 ) ;
#81748=CARTESIAN_POINT ( 'NONE',  ( 12.03043414124249999, 1426.848548796940122, 206.5778447381370029 ) ) ;
#81753=CARTESIAN_POINT ( 'NONE',  ( 3.858955742690000079, 1472.030406003990038, 215.5337125726789793 ) ) ;
#81759=CARTESIAN_POINT ( 'NONE',  ( 10.30455700085379966, 1426.851391274549997, 209.1700833811410121 ) ) ;
#81761=CARTESIAN_POINT ( 'NONE',  ( -16.08636396047539918, 1420.123211618729783, 209.9761059327369992 ) ) ;
#81763=CARTESIAN_POINT ( 'NONE',  ( 2.885753653580000133, 1430.267042387290076, 217.3699626952389963 ) ) ;
#81769=CARTESIAN_POINT ( 'NONE',  ( 8.701316397187270013, 1436.141094936039735, 208.2917281785899775 ) ) ;
#81774=CARTESIAN_POINT ( 'NONE',  ( 2.463155222774959796, 1474.677674756690067, 220.2738971877009817 ) ) ;
#81781=CARTESIAN_POINT ( 'NONE',  ( 1.106162138419999996, 1515.349603040190004, 204.8392668440190221 ) ) ;
#81782=CARTESIAN_POINT ( 'NONE',  ( 12.49318908552830010, 1427.060670871449929, 206.4845319198009861 ) ) ;
#81788=FACE_OUTER_BOUND ( 'NONE', #38760, .T. ) ;
#81789=CARTESIAN_POINT ( 'NONE',  ( 2.856819527319533147, 1485.195369544046798, 198.7387337485362480 ) ) ;
#81793=VERTEX_POINT ( 'NONE', #20532 ) ;
#81795=CARTESIAN_POINT ( 'NONE',  ( -1.337327472479999946, 1485.289799181490025, 198.0623755896990019 ) ) ;
#81796=CARTESIAN_POINT ( 'NONE',  ( 8.960243246639999271, 1478.398532434489880, 202.8149044888089918 ) ) ;
#81798=CARTESIAN_POINT ( 'NONE',  ( -11.33289292689999961, 1491.456575546390013, 207.4739972654290057 ) ) ;
#81807=CARTESIAN_POINT ( 'NONE',  ( -12.03082246793990073, 1491.135896161340042, 206.7151464320039906 ) ) ;
#81808=CARTESIAN_POINT ( 'NONE',  ( -4.421996589226610652, 1508.551704408389924, 205.0496395602209816 ) ) ;
#81815=CARTESIAN_POINT ( 'NONE',  ( 10.08617654595050084, 1470.665958206250025, 210.9901929890509962 ) ) ;
#81819=CARTESIAN_POINT ( 'NONE',  ( -1.302966447159999985, 1421.690229046850163, 193.6084558154989850 ) ) ;
#81822=CARTESIAN_POINT ( 'NONE',  ( -18.54887138051830320, 1467.029277636209827, 200.9622475402150030 ) ) ;
#81829=CARTESIAN_POINT ( 'NONE',  ( -13.93400296699999963, 1503.656733194990011, 208.7363982927060135 ) ) ;
#81834=FACE_OUTER_BOUND ( 'NONE', #9472, .T. ) ;
#81843=CARTESIAN_POINT ( 'NONE',  ( 1.868158843242359923, 1485.292041900309869, 220.8373525465659668 ) ) ;
#81844=CARTESIAN_POINT ( 'NONE',  ( 11.15670367650000117, 1501.329131309490094, 206.5574276672290068 ) ) ;
#81852=CARTESIAN_POINT ( 'NONE',  ( 6.445592309133529874, 1483.538731108610136, 219.1440388116969871 ) ) ;
#81854=PRODUCT_CONTEXT ( 'NONE', #45628, 'mechanical' ) ;
#81856=B_SPLINE_CURVE_WITH_KNOTS ( 'NONE', 3,
 ( #29428, #79856, #44600, #3167, #2059, #98290 ),
 .UNSPECIFIED., .F., .F.,
 ( 4, 2, 4 ),
 ( 0.000000000000000000, 0.5000000000000000000, 1.000000000000000000 ),
 .UNSPECIFIED. ) ;
#81859=CARTESIAN_POINT ( 'NONE',  ( 18.38166056949999927, 1428.164368492389940, 201.4944003551989908 ) ) ;
#81860=CARTESIAN_POINT ( 'NONE',  ( -2.847678236428970333, 1430.845636561999981, 201.2564352187889938 ) ) ;
#81868=B_SPLINE_CURVE_WITH_KNOTS ( 'NONE', 5,
 ( #74965, #55952, #90074, #23429, #32395, #13356, #23964, #47548, #30170 ),
 .UNSPECIFIED., .F., .F.,
 ( 6, 3, 6 ),
 ( 0.000000000000000000, 0.2526770774007812692, 1.000000000000000000 ),
 .UNSPECIFIED. ) ;
#81872=CARTESIAN_POINT ( 'NONE',  ( 1.907321127619999945, 1465.438333563990000, 199.0325445061990024 ) ) ;
#81873=CARTESIAN_POINT ( 'NONE',  ( -17.43675326300159867, 1417.688629928019964, 206.2161178420579972 ) ) ;
#81886=CARTESIAN_POINT ( 'NONE',  ( -10.31423480426190054, 1462.747221160460185, 206.6676018887629880 ) ) ;
#81897=CARTESIAN_POINT ( 'NONE',  ( -10.44855943793014319, 1480.411207778927064, 207.8053790864071289 ) ) ;
#81907=CARTESIAN_POINT ( 'NONE',  ( 3.209791212160000295, 1508.551704408389924, 219.6807919779989788 ) ) ;
#81913=VECTOR ( 'NONE', #22113, 1000.000000000000227 ) ;
#81927=CARTESIAN_POINT ( 'NONE',  ( -1.151960966433035471, 1463.347226664416667, 199.4035414042922980 ) ) ;
#81928=CARTESIAN_POINT ( 'NONE',  ( 21.12368589899999805, 1496.824149423590143, 208.3574563239919826 ) ) ;
#81934=CARTESIAN_POINT ( 'NONE',  ( -4.329448813750000014, 1515.064791442790010, 210.5737697173989886 ) ) ;
#81946=CARTESIAN_POINT ( 'NONE',  ( 12.31857963777959952, 1491.958284206870076, 208.7100351509869824 ) ) ;
#81947=CARTESIAN_POINT ( 'NONE',  ( 4.987078442593329441, 1508.551704408389924, 206.6339108768089829 ) ) ;
#81955=CARTESIAN_POINT ( 'NONE',  ( 18.99432372851790163, 1459.501274160539879, 220.3864141097060099 ) ) ;
#81959=CARTESIAN_POINT ( 'NONE',  ( -5.616639813079999932, 1453.118421927689951, 200.7460651932889846 ) ) ;
#81961=CARTESIAN_POINT ( 'NONE',  ( 7.671698190030000752, 1427.928538830389925, 213.1259091499790088 ) ) ;
#81962=CARTESIAN_POINT ( 'NONE',  ( -0.03315926146910300187, 1502.038558776489936, 233.2541124319990047 ) ) ;
#81967=CARTESIAN_POINT ( 'NONE',  ( 9.196765935889999355, 1453.799101180989965, 213.5670157982789874 ) ) ;
#81989=ORIENTED_EDGE ( 'NONE', *, *, #44202, .F. ) ;
#81990=ORIENTED_EDGE ( 'NONE', *, *, #47932, .F. ) ;
#81992=CARTESIAN_POINT ( 'NONE',  ( 21.04904418909999819, 1494.916427559390058, 209.1218459616989946 ) ) ;
#81993=AXIS2_PLACEMENT_3D ( 'NONE', #2694, #63165, #71008 ) ;
#81997=FACE_OUTER_BOUND ( 'NONE', #20983, .T. ) ;
#81999=EDGE_LOOP ( 'NONE', ( #35131, #88214, #31594, #28765, #62696 ) ) ;
#82000=FACE_OUTER_BOUND ( 'NONE', #8096, .T. ) ;
#82007=EDGE_LOOP ( 'NONE', ( #40776, #91645, #69210, #90637, #26700 ) ) ;
#82025=CARTESIAN_POINT ( 'NONE',  ( -1.003913049989999973, 1443.013031698689929, 219.0745052372589896 ) ) ;
#82028=LINE ( 'NONE', #5332, #56283 ) ;
#82038=CARTESIAN_POINT ( 'NONE',  ( 12.61062062610000112, 1426.965819617340003, 205.9085298951989671 ) ) ;
#82039=CARTESIAN_POINT ( 'NONE',  ( 0.9741480355934977187, 1498.705209631067646, 197.8347779590515358 ) ) ;
#82048=VERTEX_POINT ( 'NONE', #47962 ) ;
#82051=CARTESIAN_POINT ( 'NONE',  ( 10.88378871588750130, 1461.622812891039985, 210.4881833553409933 ) ) ;
#82052=CARTESIAN_POINT ( 'NONE',  ( 8.953637812627370351, 1424.991390415354317, 195.6949955708311109 ) ) ;
#82053=CARTESIAN_POINT ( 'NONE',  ( 2.589115358950000001, 1442.050439910990008, 217.9721093094690048 ) ) ;
#82069=CARTESIAN_POINT ( 'NONE',  ( 10.24015526565915124, 1427.983981843523225, 211.5553936737110519 ) ) ;
#82081=CARTESIAN_POINT ( 'NONE',  ( -9.579393573437259946, 1460.145585854909996, 210.2509438530599937 ) ) ;
#82094=CARTESIAN_POINT ( 'NONE',  ( 2.966112986920000250, 1454.352909205089873, 218.0484514319589948 ) ) ;
#82099=DIRECTION ( 'NONE',  ( 1.000000000000000000, 0.000000000000000000, 0.000000000000000000 ) ) ;
#82102=CARTESIAN_POINT ( 'NONE',  ( 9.420227998632439537, 1464.385042586709915, 211.9321054643539810 ) ) ;
#82104=CARTESIAN_POINT ( 'NONE',  ( 1.037000659087049748, 1515.105800736289893, 213.4502209092399880 ) ) ;
#82113=CARTESIAN_POINT ( 'NONE',  ( 13.81351351143439921, 1499.702438827800052, 227.7632555812340058 ) ) ;
#82115=CARTESIAN_POINT ( 'NONE',  ( -0.3246279079737399709, 1473.616300012054353, 219.3513874934918420 ) ) ;
#82119=CARTESIAN_POINT ( 'NONE',  ( -19.97968237250000101, 1483.906011188890034, 214.0068283976289933 ) ) ;
#82120=CARTESIAN_POINT ( 'NONE',  ( 17.76546875260000036, 1430.865606781589804, 204.9340536459789917 ) ) ;
#82121=CARTESIAN_POINT ( 'NONE',  ( -3.094819429390000209, 1457.827881892290179, 218.9172904726289914 ) ) ;
#82126=B_SPLINE_CURVE_WITH_KNOTS ( 'NONE', 3,
 ( #1712, #95199, #37497, #27992, #105254, #35852, #18460, #36936, #2817, #62177, #28548, #62747, #45913, #45373, #79513, #2277, #53216, #35289, #71133 ),
 .UNSPECIFIED., .F., .F.,
 ( 4, 3, 3, 3, 3, 3, 4 ),
 ( -8.078122936479999794, -7.682761468106989788, -6.749878609470029822, -5.846755267555650448, -4.962182452275140321, -4.110507351632660011, -3.282019784874940171 ),
 .UNSPECIFIED. ) ;
#82127=ORIENTED_EDGE ( 'NONE', *, *, #104887, .F. ) ;
#82140=AXIS2_PLACEMENT_3D ( 'NONE', #83861, #107959, #49730 ) ;
#82141=EDGE_CURVE ( 'NONE', #19394, #97755, #21452, .T. ) ;
#82152=CARTESIAN_POINT ( 'NONE',  ( 0.6257610854233279785, 1425.690485377240066, 191.1046958424169873 ) ) ;
#82160=CARTESIAN_POINT ( 'NONE',  ( 2.589235753919999445E-16, 1524.551704408390151, 209.1218459616989946 ) ) ;
#82169=CARTESIAN_POINT ( 'NONE',  ( -5.261498365895931784, 1483.803119626035141, 199.8297041156830858 ) ) ;
#82175=CARTESIAN_POINT ( 'NONE',  ( -3.996325623589930043, 1476.488318328419837, 199.5621885948499710 ) ) ;
#82178=AXIS2_PLACEMENT_3D ( 'NONE', #40637, #72602, #47943 ) ;
#82187=CARTESIAN_POINT ( 'NONE',  ( -0.05388807208240130320, 1474.848271548789853, 219.8071399965990054 ) ) ;
#82191=CARTESIAN_POINT ( 'NONE',  ( 1.222622250163819757, 1456.171658986630064, 198.6221278460869826 ) ) ;
#82193=FACE_OUTER_BOUND ( 'NONE', #19281, .T. ) ;
#82194=CARTESIAN_POINT ( 'NONE',  ( 10.15366035715699944, 1499.165878262429942, 202.2600268113060054 ) ) ;
#82195=EDGE_LOOP ( 'NONE', ( #73758, #3417, #15176, #66680 ) ) ;
#82200=CARTESIAN_POINT ( 'NONE',  ( -4.545411974820000367, 1442.929234760589907, 200.6103434261889902 ) ) ;
#82201=CARTESIAN_POINT ( 'NONE',  ( 11.63908763273079927, 1501.958057524839887, 211.3995250518869966 ) ) ;
#82203=CARTESIAN_POINT ( 'NONE',  ( -10.48189203859999985, 1491.372288729389993, 212.4833772739189897 ) ) ;
#82204=CARTESIAN_POINT ( 'NONE',  ( -1.754297334879579839, 1508.551704408389924, 220.0788184290720153 ) ) ;
#82207=CARTESIAN_POINT ( 'NONE',  ( -4.832611099234620511, 1508.551704408389924, 206.6339241720520192 ) ) ;
#82208=EDGE_CURVE ( 'NONE', #60200, #12639, #93792, .T. ) ;
#82210=CARTESIAN_POINT ( 'NONE',  ( -8.998910544736714812, 1424.786834349990158, 213.7129700835037909 ) ) ;
#82213=CARTESIAN_POINT ( 'NONE',  ( 9.218508161488790265, 1451.411218699900019, 210.0414266177820082 ) ) ;
#82219=CARTESIAN_POINT ( 'NONE',  ( 3.274413360505469939, 1508.551704408389924, 204.2617222807819815 ) ) ;
#82222=CARTESIAN_POINT ( 'NONE',  ( -19.86464697889580222, 1441.435563530799982, 212.6459098933489997 ) ) ;
#82228=CARTESIAN_POINT ( 'NONE',  ( -3.829222805975319943, 1515.551704203360032, 206.3208022964049917 ) ) ;
#82231=CARTESIAN_POINT ( 'NONE',  ( -5.077892150579999431, 1463.916894568290218, 200.2638495158990111 ) ) ;
#82234=CARTESIAN_POINT ( 'NONE',  ( -15.18835168660036139, 1420.045948940616654, 212.3480784272774713 ) ) ;
#82244=VERTEX_POINT ( 'NONE', #64654 ) ;
#82259=EDGE_CURVE ( 'NONE', #714, #12462, #6888, .T. ) ;
#82261=CARTESIAN_POINT ( 'NONE',  ( -9.241015495411470937, 1447.557127742399871, 211.4327840398769922 ) ) ;
#82267=CARTESIAN_POINT ( 'NONE',  ( 7.018957632036970651, 1424.891662419710201, 213.1748363253989851 ) ) ;
#82284=CARTESIAN_POINT ( 'NONE',  ( -5.144873395449999443, 1502.885538352589947, 229.8910404859989853 ) ) ;
#82285=VERTEX_POINT ( 'NONE', #67964 ) ;
#82302=CARTESIAN_POINT ( 'NONE',  ( 7.599032816436460003, 1483.004653252710114, 218.1850191645339976 ) ) ;
#82307=CARTESIAN_POINT ( 'NONE',  ( -10.53021734699250089, 1480.655658436720159, 208.5952819463930155 ) ) ;
#82311=CARTESIAN_POINT ( 'NONE',  ( 11.26371720470000071, 1420.479700322569897, 198.6834109214989894 ) ) ;
#82312=CARTESIAN_POINT ( 'NONE',  ( -0.4261653818286619821, 1475.450763992409975, 220.5443349783510314 ) ) ;
#82314=CARTESIAN_POINT ( 'NONE',  ( -5.117938804930000529, 1495.139203109789833, 198.3557955832989990 ) ) ;
#82318=CARTESIAN_POINT ( 'NONE',  ( 10.85780712524829994, 1423.231738543280017, 206.8437564243029954 ) ) ;
#82320=CARTESIAN_POINT ( 'NONE',  ( -9.576991855994098302, 1440.376714694789825, 206.1621517401989934 ) ) ;
#82324=AXIS2_PLACEMENT_3D ( 'NONE', #8174, #74864, #33933 ) ;
#82328=CARTESIAN_POINT ( 'NONE',  ( -15.85633924839999942, 1415.845391443659992, 209.7260009560399965 ) ) ;
#82329=CARTESIAN_POINT ( 'NONE',  ( 10.94394802638720066, 1423.896183310979950, 203.1971050292789869 ) ) ;
#82331=CARTESIAN_POINT ( 'NONE',  ( 3.040651188259999582, 1428.791177441289847, 216.8297566844390190 ) ) ;
#82334=CARTESIAN_POINT ( 'NONE',  ( -16.81730075879999831, 1417.162083013060055, 207.4277520661289884 ) ) ;
#82344=VECTOR ( 'NONE', #61854, 1000.000000000000227 ) ;
#82347=CARTESIAN_POINT ( 'NONE',  ( -12.03392632030000087, 1501.178862756489934, 213.6370645969589930 ) ) ;
#82349=CARTESIAN_POINT ( 'NONE',  ( 12.55412049360000104, 1453.847845034990087, 193.6240741990989989 ) ) ;
#82352=CARTESIAN_POINT ( 'NONE',  ( -14.57244604748959915, 1417.419309545480019, 203.2554935970629799 ) ) ;
#82360=EDGE_CURVE ( 'NONE', #78070, #75164, #33555, .T. ) ;
#82361=CARTESIAN_POINT ( 'NONE',  ( -0.5006798747275272854, 1484.181444057518320, 198.4395552954152038 ) ) ;
#82364=CARTESIAN_POINT ( 'NONE',  ( 1.126960914759999932, 1451.194794027190028, 189.8794982769989872 ) ) ;
#82367=CARTESIAN_POINT ( 'NONE',  ( 8.555072664789999948, 1479.287826498589993, 202.9093910877689950 ) ) ;
#82369=CARTESIAN_POINT ( 'NONE',  ( -11.15057513110000009, 1491.593586447790130, 208.4267869613440212 ) ) ;
#82370=CARTESIAN_POINT ( 'NONE',  ( -9.361471622734621079, 1438.259801222220176, 210.6624890962389998 ) ) ;
#82374=CARTESIAN_POINT ( 'NONE',  ( -18.89419841210175122, 1483.154679543993097, 218.3089908767800580 ) ) ;
#82379=CARTESIAN_POINT ( 'NONE',  ( -3.965129847697639764, 1508.551704408389924, 204.6168180214280028 ) ) ;
#82387=CARTESIAN_POINT ( 'NONE',  ( 10.30586371983499916, 1471.203633962730009, 211.4644565147510207 ) ) ;
#82388=CARTESIAN_POINT ( 'NONE',  ( 10.92857032808210072, 1460.888924644350027, 208.5047758900509791 ) ) ;
#82396=CARTESIAN_POINT ( 'NONE',  ( -18.27580183039999895, 1467.051542642389904, 217.8951514484589893 ) ) ;
#82403=EDGE_CURVE ( 'NONE', #23969, #103706, #99003, .T. ) ;
#82404=CARTESIAN_POINT ( 'NONE',  ( -15.17885259120000008, 1504.055100336790019, 208.8134705691849717 ) ) ;
#82416=CARTESIAN_POINT ( 'NONE',  ( -17.52552833341350080, 1417.778948467160035, 206.7855603744410189 ) ) ;
#82419=CARTESIAN_POINT ( 'NONE',  ( 12.26025649039999976, 1499.789859244890067, 205.9458331038790107 ) ) ;
#82425=CARTESIAN_POINT ( 'NONE',  ( 12.45168873679009991, 1501.262350266580142, 211.7052737702659897 ) ) ;
#82430=CARTESIAN_POINT ( 'NONE',  ( -13.90059962640000180, 1502.276548577589892, 227.4029734405989984 ) ) ;
#82433=ORIENTED_EDGE ( 'NONE', *, *, #42172, .T. ) ;
#82436=CARTESIAN_POINT ( 'NONE',  ( 12.17073519972539941, 1499.730396604210000, 205.6506567772970016 ) ) ;
#82441=LINE ( 'NONE', #56134, #93953 ) ;
#82446=( BOUNDED_CURVE ( )  B_SPLINE_CURVE ( 3, ( #40879, #59365, #31926, #93475 ),
 .UNSPECIFIED., .F., .T. ) 
 B_SPLINE_CURVE_WITH_KNOTS ( ( 4, 4 ),
 ( 3.142686768074915094, 3.147761099832099951 ),
 .UNSPECIFIED. ) 
 CURVE ( )  GEOMETRIC_REPRESENTATION_ITEM ( )  RATIONAL_B_SPLINE_CURVE ( ( 1.000000000000000000, 0.9999978542642524726, 0.9999978542642524726, 1.000000000000000000 ) ) 
 REPRESENTATION_ITEM ( '' )  );
#82451=AXIS2_PLACEMENT_3D ( 'NONE', #11297, #71221, #95834 ) ;
#82455=CARTESIAN_POINT ( 'NONE',  ( 8.441193709969130765, 1428.373632909889920, 213.4378653404860131 ) ) ;
#82457=CARTESIAN_POINT ( 'NONE',  ( -9.607526321970940586, 1460.797498750790055, 207.9656065552430277 ) ) ;
#82477=CARTESIAN_POINT ( 'NONE',  ( 2.407821901370000184, 1507.916632424389945, 220.5940247002990020 ) ) ;
#82479=CARTESIAN_POINT ( 'NONE',  ( -4.660393612750000081, 1436.848553822789881, 227.0391165213990234 ) ) ;
#82480=CARTESIAN_POINT ( 'NONE',  ( -7.749229762881280514, 1439.121665196640151, 205.0683262884020337 ) ) ;
#82485=CARTESIAN_POINT ( 'NONE',  ( -10.45474545596770000, 1481.736993775309884, 206.6726633622900238 ) ) ;
#82496=CARTESIAN_POINT ( 'NONE',  ( -8.106555885276549134, 1438.741351455190170, 205.9368832915250209 ) ) ;
#82502=CARTESIAN_POINT ( 'NONE',  ( -11.27301341819999969, 1500.749601584090215, 213.2292196792290042 ) ) ;
#82505=CARTESIAN_POINT ( 'NONE',  ( -5.498048942630000546, 1436.980437978990039, 209.3664492523469960 ) ) ;
#82516=CARTESIAN_POINT ( 'NONE',  ( 4.487357238568115747, 1509.034509761477011, 212.2379806275817486 ) ) ;
#82517=B_SPLINE_CURVE_WITH_KNOTS ( 'NONE', 3,
 ( #81353, #72982, #106574, #2497, #98718, #71369 ),
 .UNSPECIFIED., .F., .F.,
 ( 4, 2, 4 ),
 ( 0.000000000000000000, 0.2566448165338969800, 0.5131331537284539168 ),
 .UNSPECIFIED. ) ;
#82524=CARTESIAN_POINT ( 'NONE',  ( 10.03307217725760125, 1480.064660596370004, 205.9773996988400029 ) ) ;
#82525=ORIENTED_EDGE ( 'NONE', *, *, #3187, .T. ) ;
#82528=CARTESIAN_POINT ( 'NONE',  ( 0.5708672982295059928, 1460.784242391739781, 230.4191149236459921 ) ) ;
#82530=CARTESIAN_POINT ( 'NONE',  ( -16.36727155057150185, 1416.861723988390168, 208.8581010215799836 ) ) ;
#82537=CARTESIAN_POINT ( 'NONE',  ( 8.136848112800000976, 1426.803698133580156, 211.7678967111889961 ) ) ;
#82540=CARTESIAN_POINT ( 'NONE',  ( -18.43993559601290144, 1419.439711405959997, 205.9910018360060064 ) ) ;
#82542=EDGE_CURVE ( 'NONE', #58839, #52413, #44136, .T. ) ;
#82545=CARTESIAN_POINT ( 'NONE',  ( 8.476386806709999888, 1453.731993414189901, 214.0848624316990083 ) ) ;
#82546=EDGE_LOOP ( 'NONE', ( #86542, #69743, #41941 ) ) ;
#82550=ORIENTED_EDGE ( 'NONE', *, *, #45616, .T. ) ;
#82554=CARTESIAN_POINT ( 'NONE',  ( 2.251242965029999876, 1445.013527181690051, 200.2860235718189870 ) ) ;
#82557=B_SPLINE_CURVE_WITH_KNOTS ( 'NONE', 3,
 ( #39248, #30844, #31949, #22981 ),
 .UNSPECIFIED., .F., .F.,
 ( 4, 4 ),
 ( 0.000000000000000000, 1.000000000000000000 ),
 .UNSPECIFIED. ) ;
#82560=CARTESIAN_POINT ( 'NONE',  ( 5.440512190109999757, 1424.738065781850082, 191.9794586101990319 ) ) ;
#82567=DIRECTION ( 'NONE',  ( 2.491197269910784929E-47, 1.000000000000000000, -1.836970198721029688E-16 ) ) ;
#82577=CARTESIAN_POINT ( 'NONE',  ( -12.80491917260000001, 1502.810374455390047, 208.8309748505670029 ) ) ;
#82583=CARTESIAN_POINT ( 'NONE',  ( -8.212845905083440812, 1452.462047389940153, 204.7396385917020041 ) ) ;
#82592=AXIS2_PLACEMENT_3D ( 'NONE', #32101, #23131, #40497 ) ;
#82597=CARTESIAN_POINT ( 'NONE',  ( 1.042629999269999885, 1442.250188905790083, 219.0243665098589929 ) ) ;
#82601=FACE_OUTER_BOUND ( 'NONE', #71320, .T. ) ;
#82604=ORIENTED_EDGE ( 'NONE', *, *, #4861, .F. ) ;
#82608=DIRECTION ( 'NONE',  ( 0.07512831038525372152, 0.9801898970571882863, 0.1832580221591280645 ) ) ;
#82609=CARTESIAN_POINT ( 'NONE',  ( -3.805396659119999914, 1495.647976226690162, 219.6495707272989932 ) ) ;
#82611=CARTESIAN_POINT ( 'NONE',  ( 11.52427477660000044, 1425.777060552559988, 203.2852374282489905 ) ) ;
#82614=CARTESIAN_POINT ( 'NONE',  ( 4.038582018629999659, 1515.598601288590089, 209.1218459616989946 ) ) ;
#82617=EDGE_LOOP ( 'NONE', ( #86769, #69195, #4979, #57699 ) ) ;
#82620=ORIENTED_EDGE ( 'NONE', *, *, #32954, .F. ) ;
#82625=CARTESIAN_POINT ( 'NONE',  ( 8.512085479599107884, 1424.558304799583993, 195.8049112898494855 ) ) ;
#82627=CARTESIAN_POINT ( 'NONE',  ( 0.1504078502939990014, 1443.159176389090135, 218.4019229827389950 ) ) ;
#82631=CARTESIAN_POINT ( 'NONE',  ( -20.02799630220000182, 1485.574563381989947, 204.1280247810589970 ) ) ;
#82637=ORIENTED_EDGE ( 'NONE', *, *, #90599, .F. ) ;
#82640=CARTESIAN_POINT ( 'NONE',  ( 11.25045121061179998, 1470.461340873429890, 207.4716941246359738 ) ) ;
#82647=CARTESIAN_POINT ( 'NONE',  ( -14.89895980123599983, 1415.677402202029953, 206.9852695848109931 ) ) ;
#82658=CARTESIAN_POINT ( 'NONE',  ( -11.84702048589999812, 1501.805044540989911, 210.3943432492690135 ) ) ;
#82660=CARTESIAN_POINT ( 'NONE',  ( 4.974027067470000674, 1455.144349094690142, 217.5915564868190017 ) ) ;
#82661=CARTESIAN_POINT ( 'NONE',  ( 1.875671004969999833, 1456.514200624189925, 219.5762891113990065 ) ) ;
#82662=CARTESIAN_POINT ( 'NONE',  ( -9.410069260120000223, 1446.992726302889878, 212.1327064560190081 ) ) ;
#82664=CARTESIAN_POINT ( 'NONE',  ( -2.487935123034410001, 1509.038615930399828, 213.6090957347729784 ) ) ;
#82672=CARTESIAN_POINT ( 'NONE',  ( 1.575643331409844361, 1473.864451249795366, 219.2446589862094868 ) ) ;
#82676=CARTESIAN_POINT ( 'NONE',  ( -18.87649402730879800, 1504.135318570910158, 222.3338261055430110 ) ) ;
#82685=CARTESIAN_POINT ( 'NONE',  ( -4.919805416270000009, 1457.514044444589899, 217.2895299339490123 ) ) ;
#82709=ORIENTED_EDGE ( 'NONE', *, *, #81103, .T. ) ;
#82713=CARTESIAN_POINT ( 'NONE',  ( 10.92543524466419846, 1460.873421187279973, 208.4607498083740040 ) ) ;
#82714=CARTESIAN_POINT ( 'NONE',  ( 18.81609481059999922, 1456.479165729590022, 204.5196734937790097 ) ) ;
#82717=CARTESIAN_POINT ( 'NONE',  ( 7.661183502175981985, 1460.828108340008612, 203.1978207858394967 ) ) ;
#82719=CARTESIAN_POINT ( 'NONE',  ( 8.282106953172229780, 1438.168376036569953, 212.2658014659700143 ) ) ;
#82725=CARTESIAN_POINT ( 'NONE',  ( -10.38017169539999962, 1471.876108169690042, 207.0077970564690020 ) ) ;
#82727=ORIENTED_EDGE ( 'NONE', *, *, #93262, .T. ) ;
#82728=CARTESIAN_POINT ( 'NONE',  ( 0.000000000000000000, 1515.551704408389924, 209.1218459616989946 ) ) ;
#82734=CARTESIAN_POINT ( 'NONE',  ( 5.531434274799999606, 1486.727690549889758, 199.8330512247090098 ) ) ;
#82735=CARTESIAN_POINT ( 'NONE',  ( -3.747504258231699747, 1476.575485711930014, 199.4578548330160004 ) ) ;
#82737=CARTESIAN_POINT ( 'NONE',  ( -13.59512407998240135, 1507.703338069740084, 209.3532897553030239 ) ) ;
#82741=CARTESIAN_POINT ( 'NONE',  ( -17.38831264790000120, 1417.589637829370076, 206.5146517552989849 ) ) ;
#82744=CARTESIAN_POINT ( 'NONE',  ( -15.13389074177019999, 1508.450542589140241, 215.3798312893059972 ) ) ;
#82750=B_SPLINE_CURVE_WITH_KNOTS ( 'NONE', 5,
 ( #108226, #100381, #65144, #7421, #41587, #48904, #47781, #58940, #39928, #75742, #99257, #24742 ),
 .UNSPECIFIED., .F., .F.,
 ( 6, 3, 3, 6 ),
 ( -19.23936229089999728, -13.68355489660000046, -9.538385084389998880, -6.352442800617261298 ),
 .UNSPECIFIED. ) ;
#82755=CARTESIAN_POINT ( 'NONE',  ( -9.980609342266690831, 1471.167102018479909, 211.5702527342239989 ) ) ;
#82756=CARTESIAN_POINT ( 'NONE',  ( 9.607334135293850608, 1470.026661626050100, 212.1640507808000109 ) ) ;
#82760=CARTESIAN_POINT ( 'NONE',  ( 10.94662241205340081, 1479.920664513949987, 208.8401849076869894 ) ) ;
#82762=CARTESIAN_POINT ( 'NONE',  ( -4.792996137980000348, 1442.435460035689857, 201.1994128016890215 ) ) ;
#82763=CARTESIAN_POINT ( 'NONE',  ( 7.571421872719999335, 1423.019346856819993, 195.7264222406990086 ) ) ;
#82765=CARTESIAN_POINT ( 'NONE',  ( 10.39912873559759987, 1422.379202795500078, 211.6466214762630216 ) ) ;
#82771=CARTESIAN_POINT ( 'NONE',  ( 11.86058708272519979, 1492.120471498190000, 209.8867464431719725 ) ) ;
#82774=CARTESIAN_POINT ( 'NONE',  ( -4.992349863779999453, 1391.620913471789891, 214.4361776263990009 ) ) ;
#82776=CARTESIAN_POINT ( 'NONE',  ( 4.650616333322320273, 1508.551704408389924, 205.3792392240669926 ) ) ;
#82778=ORIENTED_EDGE ( 'NONE', *, *, #32954, .T. ) ;
#82780=CARTESIAN_POINT ( 'NONE',  ( -4.020407408646379466, 1515.375307573260216, 205.5795248161299753 ) ) ;
#82782=CARTESIAN_POINT ( 'NONE',  ( -10.93162616829999934, 1470.132888108789984, 212.2376404388290041 ) ) ;
#82783=CARTESIAN_POINT ( 'NONE',  ( -5.284442937980000643, 1463.440241038189924, 200.7106537499089711 ) ) ;
#82790=CARTESIAN_POINT ( 'NONE',  ( 1.662820216281789998, 1431.604432834220006, 200.5143882900920005 ) ) ;
#82803=CARTESIAN_POINT ( 'NONE',  ( 20.45347777980000004, 1495.695647834889996, 214.2365953844490036 ) ) ;
#82811=CARTESIAN_POINT ( 'NONE',  ( 7.393437199623040357, 1425.120646642689962, 212.4672936276909923 ) ) ;
#82814=DIRECTION ( 'NONE',  ( 0.000000000000000000, 1.836970198721029688E-16, 1.000000000000000000 ) ) ;
#82824=CARTESIAN_POINT ( 'NONE',  ( 11.35976097320000022, 1500.240390108989914, 205.8138550405789999 ) ) ;
#82826=CARTESIAN_POINT ( 'NONE',  ( 9.783037280509999434, 1463.178299378289921, 209.2268572133950215 ) ) ;
#82835=CARTESIAN_POINT ( 'NONE',  ( 4.240947575409800052, 1509.032041868229953, 212.8661569781619960 ) ) ;
#82844=CARTESIAN_POINT ( 'NONE',  ( 8.631805628161151489, 1482.492055270540050, 217.1926854337019961 ) ) ;
#82850=CARTESIAN_POINT ( 'NONE',  ( -11.27660745936439923, 1481.154147052749977, 210.7583899964359944 ) ) ;
#82853=CARTESIAN_POINT ( 'NONE',  ( -10.50233093623509895, 1470.323195244420049, 212.1312216483660222 ) ) ;
#82854=CARTESIAN_POINT ( 'NONE',  ( 10.57795761202480200, 1502.789340137210047, 216.2109890099079905 ) ) ;
#82855=CARTESIAN_POINT ( 'NONE',  ( 12.40160733289999939, 1420.584110886950157, 200.5244703085189997 ) ) ;
#82857=CARTESIAN_POINT ( 'NONE',  ( -3.411025239260000230, 1429.511272153089976, 201.4092281563090125 ) ) ;
#82858=CARTESIAN_POINT ( 'NONE',  ( -4.932281309879999576, 1495.209075895590104, 198.2667700775990056 ) ) ;
#82862=CARTESIAN_POINT ( 'NONE',  ( 10.68184976760720062, 1424.590726042679989, 206.5862489259359904 ) ) ;
#82867=DIRECTION ( 'NONE',  ( -9.439841191556039654E-47, 1.000000000000000000, -1.836970198721029688E-16 ) ) ;
#82870=CARTESIAN_POINT ( 'NONE',  ( 9.650233255823788880, 1426.324557352379998, 209.5560370033680044 ) ) ;
#82872=CARTESIAN_POINT ( 'NONE',  ( 10.94714963045309908, 1423.994054955890078, 203.1837039224479895 ) ) ;
#82874=CARTESIAN_POINT ( 'NONE',  ( 1.988090766190000025, 1430.930902329289893, 217.9995054648290136 ) ) ;
#82876=CARTESIAN_POINT ( 'NONE',  ( -6.673722543209559710, 1476.318849632387128, 217.0466873364883611 ) ) ;
#82882=CARTESIAN_POINT ( 'NONE',  ( -16.87694756293090137, 1420.409301044890071, 203.4763756665570327 ) ) ;
#82883=CARTESIAN_POINT ( 'NONE',  ( 9.636272919195080888, 1459.879703458749873, 204.9556293222869954 ) ) ;
#82884=CARTESIAN_POINT ( 'NONE',  ( 7.306949285421709739, 1422.442428900340019, 195.7985199449469746 ) ) ;
#82891=CARTESIAN_POINT ( 'NONE',  ( -7.717961373019999627, 1491.908876820690011, 210.2849100519189847 ) ) ;
#82892=CARTESIAN_POINT ( 'NONE',  ( -5.080289282479999002, 1480.093209919690253, 228.8812397303989883 ) ) ;
#82894=CARTESIAN_POINT ( 'NONE',  ( 1.477486471849999816, 1515.342042115489903, 204.8476099990489843 ) ) ;
#82895=CARTESIAN_POINT ( 'NONE',  ( 7.799999999999998934, 1392.213060387289943, 209.1218459616989946 ) ) ;
#82896=CARTESIAN_POINT ( 'NONE',  ( -2.130922739460000326, 1467.954349356489956, 220.0452206896989935 ) ) ;
#82908=CARTESIAN_POINT ( 'NONE',  ( -2.069830134539999644, 1485.439312381189893, 197.8250538963989982 ) ) ;
#82911=CARTESIAN_POINT ( 'NONE',  ( -11.36633173080000070, 1491.361353432889928, 207.7497694925790199 ) ) ;
#82919=CARTESIAN_POINT ( 'NONE',  ( -3.739876349838270109, 1508.551704408389924, 204.4696467160270288 ) ) ;
#82935=CARTESIAN_POINT ( 'NONE',  ( 8.761644880424068305, 1498.445921004877619, 199.9006591228519198 ) ) ;
#82968=CARTESIAN_POINT ( 'NONE',  ( -3.071484426853159810, 1470.850312049700051, 187.3986296107530052 ) ) ;
#82969=LINE ( 'NONE', #109829, #44103 ) ;
#82970=ORIENTED_EDGE ( 'NONE', *, *, #6256, .T. ) ;
#82973=B_SPLINE_CURVE_WITH_KNOTS ( 'NONE', 5,
 ( #44762, #36333, #13309, #38532, #20611, #80552 ),
 .UNSPECIFIED., .F., .F.,
 ( 6, 6 ),
 ( 177.0697656899999970, 181.8804217290000054 ),
 .UNSPECIFIED. ) ;
#82974=CARTESIAN_POINT ( 'NONE',  ( -1.739522437470000016, 1431.560227954390029, 203.6467502218990262 ) ) ;
#82976=CARTESIAN_POINT ( 'NONE',  ( 12.39029448242800058, 1499.902199860550127, 206.4711935520600150 ) ) ;
#82977=CARTESIAN_POINT ( 'NONE',  ( -19.39428932798890060, 1507.987873490819993, 209.4883875057280136 ) ) ;
#82979=CARTESIAN_POINT ( 'NONE',  ( 4.290508147279999740, 1515.379315998089851, 209.1218459616059988 ) ) ;
#82983=CARTESIAN_POINT ( 'NONE',  ( 0.9714241662080010942, 1464.771691177589901, 199.1654275922589932 ) ) ;
#82999=CARTESIAN_POINT ( 'NONE',  ( -9.549407038459840180, 1461.437203121739913, 207.3744785622409665 ) ) ;
#83012=EDGE_CURVE ( 'NONE', #32787, #25418, #26616, .T. ) ;
#83017=CARTESIAN_POINT ( 'NONE',  ( 3.778541329980110053, 1515.551842520359969, 212.4904429341349896 ) ) ;
#83027=CARTESIAN_POINT ( 'NONE',  ( -8.104271283259439684, 1425.304381095269946, 204.5473957581349964 ) ) ;
#83028=ADVANCED_FACE ( 'NONE', ( #59441 ), #15107, .F. ) ;
#83029=CARTESIAN_POINT ( 'NONE',  ( -16.64903386090459847, 1482.394134636929948, 222.3169631199170055 ) ) ;
#83047=CARTESIAN_POINT ( 'NONE',  ( -10.80145638409999975, 1500.322425017390060, 215.2964120902790057 ) ) ;
#83055=CARTESIAN_POINT ( 'NONE',  ( -8.551515107930001136, 1437.707591943389843, 226.0657740139990040 ) ) ;
#83056=CARTESIAN_POINT ( 'NONE',  ( -3.313501335607589748, 1397.551704408390151, 203.0565224509919915 ) ) ;
#83058=LINE ( 'NONE', #7995, #23204 ) ;
#83070=B_SPLINE_SURFACE_WITH_KNOTS ( 'NONE', 5, 5, ( 
 ( #16298, #33665, #53263, #102518, #104744, #17958 ),
 ( #76790, #87402, #59458, #68415, #1761, #86840 ),
 ( #86286, #85178, #106, #19058, #103070, #25809 ),
 ( #51595, #9571, #651, #78447, #52154, #26371 ),
 ( #44304, #69523, #94128, #16843, #60566, #43743 ),
 ( #77894, #77349, #70626, #93568, #60008, #85728 ),
 ( #94686, #10696, #8464, #68969, #61667, #34229 ),
 ( #44868, #42637, #17399, #1201, #9027, #104194 ),
 ( #43197, #34782, #35334, #103643, #70081, #26941 ) ),
 .UNSPECIFIED., .F., .F., .F.,
 ( 6, 3, 6 ),
 ( 6, 6 ),
 ( 2.999964336638760276, 5.147071007630000139, 7.294170209094329671 ),
 ( -0.0003925606712395320248, 2.000000000000000000 ),
 .UNSPECIFIED. ) ;
#83071=LINE ( 'NONE', #22023, #57328 ) ;
#83072=CARTESIAN_POINT ( 'NONE',  ( -13.59404883793579977, 1507.952376021150030, 209.4255341775249804 ) ) ;
#83073=CARTESIAN_POINT ( 'NONE',  ( -19.58884347341419740, 1465.811382977840140, 204.1485388397669851 ) ) ;
#83075=CARTESIAN_POINT ( 'NONE',  ( -2.487935121788300119, 1509.038615937200120, 204.6345961869410246 ) ) ;
#83077=CARTESIAN_POINT ( 'NONE',  ( -14.59898950506980064, 1420.572608572590070, 213.0506973618599886 ) ) ;
#83078=CARTESIAN_POINT ( 'NONE',  ( -5.504476062790000235, 1453.787349605589952, 201.3614901105490276 ) ) ;
#83079=EDGE_CURVE ( 'NONE', #45257, #21520, #75998, .T. ) ;
#83084=CARTESIAN_POINT ( 'NONE',  ( -20.23525057476570055, 1418.571322831110137, 207.2471207475410040 ) ) ;
#83088=ORIENTED_EDGE ( 'NONE', *, *, #4527, .T. ) ;
#83093=VERTEX_POINT ( 'NONE', #11237 ) ;
#83113=ORIENTED_EDGE ( 'NONE', *, *, #4374, .F. ) ;
#83120=CARTESIAN_POINT ( 'NONE',  ( -11.36959371680000075, 1503.847165134090119, 207.0750569533189775 ) ) ;
#83122=ORIENTED_EDGE ( 'NONE', *, *, #68564, .F. ) ;
#83127=EDGE_CURVE ( 'NONE', #86947, #18777, #104726, .T. ) ;
#83136=CARTESIAN_POINT ( 'NONE',  ( 21.04692457260000182, 1494.868043414790009, 208.8005846134330170 ) ) ;
#83137=EDGE_CURVE ( 'NONE', #78921, #104968, #54351, .T. ) ;
#83144=CARTESIAN_POINT ( 'NONE',  ( 2.194612407920000230, 1441.754231285490050, 218.8080856977990152 ) ) ;
#83158=CARTESIAN_POINT ( 'NONE',  ( 10.95098205620359977, 1471.837422849929908, 212.3987392730099657 ) ) ;
#83159=CARTESIAN_POINT ( 'NONE',  ( 12.91968529760000095, 1421.051477647549973, 203.8574114591390014 ) ) ;
#83160=CARTESIAN_POINT ( 'NONE',  ( -2.157645518950584762, 1497.833544052899924, 198.0401058465139670 ) ) ;
#83162=CARTESIAN_POINT ( 'NONE',  ( 9.345710454894810226, 1422.635914553260136, 212.8840094578699791 ) ) ;
#83172=CARTESIAN_POINT ( 'NONE',  ( 10.78424521582030060, 1461.890582932750249, 211.1530446443910023 ) ) ;
#83174=CARTESIAN_POINT ( 'NONE',  ( 8.351838315039440630, 1424.363087015397468, 195.8336220494941529 ) ) ;
#83175=CARTESIAN_POINT ( 'NONE',  ( 4.577412241270000237, 1466.377840905189942, 218.3518450454489823 ) ) ;
#83188=CARTESIAN_POINT ( 'NONE',  ( 11.18053625668549955, 1470.337374907619960, 207.1025468278700146 ) ) ;
#83189=DIRECTION ( 'NONE',  ( -9.152776640618289361E-47, 1.000000000000000000, -1.836970198721029688E-16 ) ) ;
#83192=B_SPLINE_SURFACE_WITH_KNOTS ( 'NONE', 5, 1, ( 
 ( #109193, #89614 ),
 ( #32479, #13999 ),
 ( #81753, #30252 ),
 ( #65543, #57146 ),
 ( #5059, #91273 ),
 ( #39773, #12905 ) ),
 .UNSPECIFIED., .F., .F., .F.,
 ( 6, 6 ),
 ( 2, 2 ),
 ( 0.000000000000000000, 16.96319496739999977 ),
 ( 0.000000000000000000, 14.00000000000000000 ),
 .UNSPECIFIED. ) ;
#83193=CARTESIAN_POINT ( 'NONE',  ( -8.654005124046650010, 1437.544186111149884, 209.5117930731329920 ) ) ;
#83194=CARTESIAN_POINT ( 'NONE',  ( -2.329920886068990171, 1515.492270357839971, 213.2601720499270073 ) ) ;
#83196=CARTESIAN_POINT ( 'NONE',  ( -15.26371167349380009, 1415.677402202059966, 208.6401185093320123 ) ) ;
#83198=CARTESIAN_POINT ( 'NONE',  ( -5.498048945769999918, 1436.980437970689991, 209.3664492512450011 ) ) ;
#83203=EDGE_LOOP ( 'NONE', ( #90135, #8221, #55788, #52632 ) ) ;
#83204=EDGE_LOOP ( 'NONE', ( #83943, #54720, #13251, #105324 ) ) ;
#83207=CARTESIAN_POINT ( 'NONE',  ( 4.594279763170000308, 1454.322381208490015, 217.3118965033989980 ) ) ;
#83209=CARTESIAN_POINT ( 'NONE',  ( -5.723713397950000115, 1444.578274639889969, 217.6728780112489972 ) ) ;
#83223=AXIS2_PLACEMENT_3D ( 'NONE', #49324, #29, #84561 ) ;
#83224=CARTESIAN_POINT ( 'NONE',  ( 19.51639363059999965, 1499.800465969690094, 221.7092710762990180 ) ) ;
#83226=CARTESIAN_POINT ( 'NONE',  ( 0.9833190725767226859, 1473.213984233044357, 219.2916102971160512 ) ) ;
#83232=CARTESIAN_POINT ( 'NONE',  ( -5.038090724669999965, 1458.590897767190199, 218.1407348443790113 ) ) ;
#83254=DIRECTION ( 'NONE',  ( 0.9109372852568263790, 0.3047011255600591273, -0.2781195541693470830 ) ) ;
#83261=CARTESIAN_POINT ( 'NONE',  ( 5.277460848200000498, 1426.742654866309977, 191.8370381630989812 ) ) ;
#83265=CARTESIAN_POINT ( 'NONE',  ( 6.024952519936291218, 1460.026342669724045, 201.5977334549522766 ) ) ;
#83268=CARTESIAN_POINT ( 'NONE',  ( 8.678413303154190572, 1437.443562278949912, 211.8714791696150144 ) ) ;
#83273=CARTESIAN_POINT ( 'NONE',  ( -9.132731034919599367, 1438.960184460119763, 208.5834308107819766 ) ) ;
#83280=CARTESIAN_POINT ( 'NONE',  ( -12.23489732466240021, 1490.237667237379810, 209.6383001084460034 ) ) ;
#83282=CARTESIAN_POINT ( 'NONE',  ( 9.627390985499999942, 1488.793226916890035, 203.8059392817090156 ) ) ;
#83283=CARTESIAN_POINT ( 'NONE',  ( -4.484642789696589915, 1476.314628642159960, 199.7897337046530026 ) ) ;
#83285=PLANE ( 'NONE',  #74583 ) ;
#83288=ORIENTED_EDGE ( 'NONE', *, *, #51714, .T. ) ;
#83291=CARTESIAN_POINT ( 'NONE',  ( -17.76136201589839914, 1508.551704408389924, 211.4804395128520014 ) ) ;
#83295=CARTESIAN_POINT ( 'NONE',  ( -3.076485559970000061, 1476.334861387889987, 220.1839305697990028 ) ) ;
#83299=CARTESIAN_POINT ( 'NONE',  ( -7.633360230528516865, 1508.421455160203095, 219.5388691105322891 ) ) ;
#83304=CARTESIAN_POINT ( 'NONE',  ( 4.328003007221930432, 1515.120004566319949, 208.2632874389240101 ) ) ;
#83305=CARTESIAN_POINT ( 'NONE',  ( 9.327653393340000321, 1434.415568160490011, 206.2244200652989718 ) ) ;
#83306=ORIENTED_EDGE ( 'NONE', *, *, #63149, .T. ) ;
#83307=EDGE_LOOP ( 'NONE', ( #105064, #59146, #27987, #43983 ) ) ;
#83308=CARTESIAN_POINT ( 'NONE',  ( 8.631780704876279131, 1438.018275767699834, 210.0183142686710198 ) ) ;
#83310=CARTESIAN_POINT ( 'NONE',  ( -3.792859824510000255, 1442.868606696990128, 200.6312857326389860 ) ) ;
#83311=CARTESIAN_POINT ( 'NONE',  ( 11.39524851002120087, 1502.549053284450110, 211.1908584932759823 ) ) ;
#83314=CARTESIAN_POINT ( 'NONE',  ( 0.07192813133532849346, 1508.551704408389924, 220.0014440396450084 ) ) ;
#83319=CARTESIAN_POINT ( 'NONE',  ( -11.96237584231419859, 1502.200202672119985, 208.9057378585949891 ) ) ;
#83320=CARTESIAN_POINT ( 'NONE',  ( 10.93055278244830042, 1491.052779700740075, 210.3465334192150067 ) ) ;
#83331=CARTESIAN_POINT ( 'NONE',  ( 3.625350584860000058, 1486.483312423590178, 219.2891606026990132 ) ) ;
#83332=CARTESIAN_POINT ( 'NONE',  ( -8.804296921149999733, 1463.411480388290101, 203.0665974443489858 ) ) ;
#83334=CARTESIAN_POINT ( 'NONE',  ( 0.4757565577110009492, 1443.099148102289973, 202.9022611692290070 ) ) ;
#83335=CARTESIAN_POINT ( 'NONE',  ( -14.33147639189130018, 1508.551704408389924, 215.5212910536350250 ) ) ;
#83339=CARTESIAN_POINT ( 'NONE',  ( 2.952227049714620133, 1431.436650656529991, 200.0252637764760095 ) ) ;
#83347=CARTESIAN_POINT ( 'NONE',  ( -1.250333264278968182, 1515.565566433391041, 213.0675868911715725 ) ) ;
#83354=CARTESIAN_POINT ( 'NONE',  ( -4.775348822359999801, 1443.097051919790147, 200.2639737031189782 ) ) ;
#83359=CARTESIAN_POINT ( 'NONE',  ( 7.425514022726639851, 1425.169617594710189, 212.4007796381419837 ) ) ;
#83360=ORIENTED_EDGE ( 'NONE', *, *, #35850, .T. ) ;
#83381=CARTESIAN_POINT ( 'NONE',  ( 20.45347777980000004, 1495.695647834889996, 214.2365953844490036 ) ) ;
#83383=CARTESIAN_POINT ( 'NONE',  ( 3.744428047356039624, 1509.032041130069956, 213.3627866063060026 ) ) ;
#83396=CARTESIAN_POINT ( 'NONE',  ( 3.722374432750000128, 1427.445946224140016, 212.8307634929090284 ) ) ;
#83403=CARTESIAN_POINT ( 'NONE',  ( 5.931178066143490746, 1504.797995861300024, 220.4212288460319940 ) ) ;
#83404=CARTESIAN_POINT ( 'NONE',  ( 7.749386596619999956, 1421.739053608140011, 195.8155783956989922 ) ) ;
#83405=CARTESIAN_POINT ( 'NONE',  ( 1.285768303291729975, 1431.378437453980041, 218.5251442782430047 ) ) ;
#83406=CARTESIAN_POINT ( 'NONE',  ( -11.48467662286570068, 1491.814333413060012, 204.7694204252460111 ) ) ;
#83407=CARTESIAN_POINT ( 'NONE',  ( -5.218327569770000451, 1496.717035854290089, 199.1635217715490001 ) ) ;
#83411=CARTESIAN_POINT ( 'NONE',  ( 10.69336184592519956, 1424.688236166109846, 206.5739417092179906 ) ) ;
#83419=CARTESIAN_POINT ( 'NONE',  ( 10.69109047475079954, 1427.380511044090099, 209.6415026742359942 ) ) ;
#83420=CARTESIAN_POINT ( 'NONE',  ( 12.26400251256059981, 1421.315719094279984, 203.4348889297749849 ) ) ;
#83421=CARTESIAN_POINT ( 'NONE',  ( 1.618075321620000118, 1431.058998840389904, 218.0723462992190207 ) ) ;
#83426=CARTESIAN_POINT ( 'NONE',  ( -16.79355120555579717, 1420.470915846049820, 203.2250788671829866 ) ) ;
#83434=CARTESIAN_POINT ( 'NONE',  ( -1.096329832589999942, 1473.937728199189905, 216.5791357104590134 ) ) ;
#83441=CARTESIAN_POINT ( 'NONE',  ( 9.504367897392947739, 1467.890094308543212, 205.9436694967274946 ) ) ;
#83454=CARTESIAN_POINT ( 'NONE',  ( -2.469737631213410278, 1507.227429411520006, 221.7265308815400147 ) ) ;
#83461=CARTESIAN_POINT ( 'NONE',  ( 9.840543299160298574, 1424.658749102479987, 208.3834677199979808 ) ) ;
#83465=CARTESIAN_POINT ( 'NONE',  ( 3.843703091317430154, 1437.067272161539904, 227.2460596593799949 ) ) ;
#83467=CARTESIAN_POINT ( 'NONE',  ( 5.469129087219999796, 1473.910357677790216, 219.1569924984989939 ) ) ;
#83468=CARTESIAN_POINT ( 'NONE',  ( 9.600627300107769102, 1470.542558681519949, 212.2539986962150067 ) ) ;
#83470=CARTESIAN_POINT ( 'NONE',  ( 17.69622264849999738, 1430.679833671289771, 213.5595385020990022 ) ) ;
#83477=CARTESIAN_POINT ( 'NONE',  ( 11.23074002719829068, 1499.222125023890158, 203.1659919298568013 ) ) ;
#83478=LINE ( 'NONE', #68372, #101401 ) ;
#83481=CARTESIAN_POINT ( 'NONE',  ( -2.805707806560000073, 1456.378508730689873, 200.0530498395189909 ) ) ;
#83493=CARTESIAN_POINT ( 'NONE',  ( 11.08618182320000045, 1501.737459411990130, 206.1990983140089782 ) ) ;
#83507=CARTESIAN_POINT ( 'NONE',  ( 24.04367183769999983, 1494.655699983489967, 207.1743773500889745 ) ) ;
#83512=CARTESIAN_POINT ( 'NONE',  ( 10.44661746959009996, 1453.078959294469996, 210.9304775587480094 ) ) ;
#83515=CARTESIAN_POINT ( 'NONE',  ( -2.330134121946666692, 1515.499673595108106, 213.2081603283779998 ) ) ;
#83533=EDGE_CURVE ( 'NONE', #88894, #43306, #62765, .T. ) ;
#83535=CARTESIAN_POINT ( 'NONE',  ( -2.958237724348658393, 1515.068899831253702, 213.4511871771338178 ) ) ;
#83539=CARTESIAN_POINT ( 'NONE',  ( -1.531246620494349863E-13, 1515.064792882589927, 204.7923971856590128 ) ) ;
#83553=CARTESIAN_POINT ( 'NONE',  ( -2.466508595303360085, 1483.693203563210091, 198.7383541362370067 ) ) ;
#83554=CARTESIAN_POINT ( 'NONE',  ( -4.261736551907977955, 1515.372048949686587, 211.4519800884182246 ) ) ;
#83555=ORIENTED_EDGE ( 'NONE', *, *, #6559, .T. ) ;
#83557=CARTESIAN_POINT ( 'NONE',  ( 2.375641846589999773, 1508.210248838890038, 220.4645691950989885 ) ) ;
#83559=CARTESIAN_POINT ( 'NONE',  ( -15.55456937169999954, 1415.677402205460112, 209.5577859103179890 ) ) ;
#83562=CARTESIAN_POINT ( 'NONE',  ( -6.021347807395219576, 1427.070447557959824, 201.9849352095830000 ) ) ;
#83564=ADVANCED_FACE ( 'NONE', ( #17242 ), #6173, .T. ) ;
#83566=CARTESIAN_POINT ( 'NONE',  ( -11.05549909325160129, 1482.557859868360083, 206.1126638933569950 ) ) ;
#83568=CARTESIAN_POINT ( 'NONE',  ( -19.23853081770000273, 1466.576780668189940, 213.8528554934590034 ) ) ;
#83572=EDGE_CURVE ( 'NONE', #20921, #79507, #30219, .T. ) ;
#83574=CARTESIAN_POINT ( 'NONE',  ( 10.93965183780649930, 1490.038857010280026, 208.6218812487679770 ) ) ;
#83576=CARTESIAN_POINT ( 'NONE',  ( 2.960916190616809995, 1454.351986964310072, 218.0342237851930065 ) ) ;
#83579=CARTESIAN_POINT ( 'NONE',  ( -15.01829424220000142, 1417.605436662430293, 203.9468348563890174 ) ) ;
#83582=CARTESIAN_POINT ( 'NONE',  ( -5.202920445667687410, 1495.777355175065622, 199.0561123049738512 ) ) ;
#83583=CARTESIAN_POINT ( 'NONE',  ( -4.325805437739999704, 1515.203925700790023, 210.5851323563490212 ) ) ;
#83590=EDGE_CURVE ( 'NONE', #26374, #103670, #37398, .T. ) ;
#83604=CARTESIAN_POINT ( 'NONE',  ( 10.25492199526250126, 1479.646048717419944, 206.2690387796579898 ) ) ;
#83608=CARTESIAN_POINT ( 'NONE',  ( -9.393915101222290787, 1447.312189566800043, 190.7225392970269979 ) ) ;
#83609=CARTESIAN_POINT ( 'NONE',  ( -13.59063756412279922, 1508.278172206230010, 209.6547395369879894 ) ) ;
#83610=CARTESIAN_POINT ( 'NONE',  ( -13.97985296196779892, 1420.196174965909904, 195.9955836505269815 ) ) ;
#83616=ADVANCED_FACE ( 'NONE', ( #96200 ), #925, .T. ) ;
#83621=CARTESIAN_POINT ( 'NONE',  ( -5.376254996749998888E-14, 1377.913060387289988, 209.1218459616989946 ) ) ;
#83623=CARTESIAN_POINT ( 'NONE',  ( -15.98597864390959700, 1420.860748498030034, 203.3503307164980072 ) ) ;
#83629=ORIENTED_EDGE ( 'NONE', *, *, #76872, .T. ) ;
#83637=CARTESIAN_POINT ( 'NONE',  ( -0.2476383817669989829, 1444.562280487289854, 199.4410856530290062 ) ) ;
#83641=CARTESIAN_POINT ( 'NONE',  ( -4.385072903111329801, 1462.684657158180016, 200.4014842359929958 ) ) ;
#83642=CARTESIAN_POINT ( 'NONE',  ( -17.06926747740000039, 1417.584731029579871, 207.6120866810690018 ) ) ;
#83658=CARTESIAN_POINT ( 'NONE',  ( -6.942420851809999682, 1472.648385638490026, 209.3924741736690009 ) ) ;
#83660=ORIENTED_EDGE ( 'NONE', *, *, #11868, .F. ) ;
#83661=CARTESIAN_POINT ( 'NONE',  ( -11.61029339299999918, 1501.887990476489904, 208.8313362839550109 ) ) ;
#83684=CARTESIAN_POINT ( 'NONE',  ( 0.7065304258729989684, 1442.384625720290160, 219.0605242788890052 ) ) ;
#83697=CARTESIAN_POINT ( 'NONE',  ( -2.277036528833521700, 1495.095314405110230, 220.0578060253683361 ) ) ;
#83698=CARTESIAN_POINT ( 'NONE',  ( 6.157268126266139951, 1484.877070555129876, 217.9975064028730287 ) ) ;
#83700=CARTESIAN_POINT ( 'NONE',  ( 3.346707516019999940, 1443.005054410889898, 217.3642451189890323 ) ) ;
#83702=B_SPLINE_CURVE_WITH_KNOTS ( 'NONE', 3,
 ( #25682, #16712, #17266, #94002, #34099, #100735, #58217, #7250, #24571, #43067, #77227, #24019, #529, #92342, #41958, #93443, #41412, #8335, #75579, #102399, #101274, #58762, #76657, #110807, #59875, #68292, #34653, #68837, #102553, #67350, #41582, #8504, #9070, #76833, #93604, #77931, #103683 ),
 .UNSPECIFIED., .F., .F.,
 ( 4, 3, 3, 3, 3, 3, 3, 3, 3, 3, 3, 3, 4 ),
 ( -12.84118046881009967, -12.56545256453010140, -11.90146324839760084, -11.19785799506759894, -10.45680950016819999, -9.662019177287570315, -8.697168689982460066, -7.747513139449250019, -6.994387148789269482, -6.090255947446629570, -5.292960030990699671, -4.586645094369940168, -3.918736331710000798 ),
 .UNSPECIFIED. ) ;
#83705=CARTESIAN_POINT ( 'NONE',  ( -9.135900476020308858, 1449.599620636940244, 210.0844635627520063 ) ) ;
#83706=CARTESIAN_POINT ( 'NONE',  ( 1.550651194191815074, 1515.551704408391060, 205.2291894524878728 ) ) ;
#83707=VECTOR ( 'NONE', #63950, 1000.000000000000114 ) ;
#83708=ORIENTED_EDGE ( 'NONE', *, *, #44618, .F. ) ;
#83715=CARTESIAN_POINT ( 'NONE',  ( -8.392959608848258313, 1461.613719735366431, 204.2281241542300734 ) ) ;
#83716=CARTESIAN_POINT ( 'NONE',  ( -1.693091880119999892, 1443.235800636190106, 218.9922110084989981 ) ) ;
#83720=CARTESIAN_POINT ( 'NONE',  ( 8.559858904628349308, 1437.030483964089854, 207.9845584131589931 ) ) ;
#83728=CARTESIAN_POINT ( 'NONE',  ( -7.942873757061038376, 1438.931140274130030, 205.4976076133249876 ) ) ;
#83736=CARTESIAN_POINT ( 'NONE',  ( -9.539087469214889481, 1439.128768127180138, 208.8797462174109967 ) ) ;
#83752=CARTESIAN_POINT ( 'NONE',  ( 2.090891989490000213, 1455.065938962190103, 218.3193683645590113 ) ) ;
#83753=CARTESIAN_POINT ( 'NONE',  ( 1.782252617107189963, 1456.535908150360001, 219.5922471067279673 ) ) ;
#83754=CARTESIAN_POINT ( 'NONE',  ( -2.236878054880000022, 1443.656060954389886, 218.5246926830890004 ) ) ;
#83758=DIRECTION ( 'NONE',  ( 1.000000000000000000, 0.000000000000000000, 0.000000000000000000 ) ) ;
#83762=CARTESIAN_POINT ( 'NONE',  ( -3.459700914049689491, 1454.194523623659961, 199.2295117871159960 ) ) ;
#83769=ORIENTED_EDGE ( 'NONE', *, *, #50763, .T. ) ;
#83773=CARTESIAN_POINT ( 'NONE',  ( -13.85617977377259891, 1502.671218317619832, 227.4591309510049939 ) ) ;
#83780=CARTESIAN_POINT ( 'NONE',  ( 18.28970766670409986, 1431.718711396310027, 208.8872839595150026 ) ) ;
#83791=CARTESIAN_POINT ( 'NONE',  ( 7.234729710160780591, 1424.755084673710144, 194.1035305753040348 ) ) ;
#83802=DIRECTION ( 'NONE',  ( 1.000000000000000000, 0.000000000000000000, 0.000000000000000000 ) ) ;
#83803=CARTESIAN_POINT ( 'NONE',  ( -20.02800037099130037, 1485.574564704460045, 204.1280240222589839 ) ) ;
#83805=ORIENTED_EDGE ( 'NONE', *, *, #87461, .T. ) ;
#83809=CARTESIAN_POINT ( 'NONE',  ( -0.7718352176453070479, 1425.376890532889774, 191.1258158093919803 ) ) ;
#83823=FACE_OUTER_BOUND ( 'NONE', #92806, .T. ) ;
#83829=CARTESIAN_POINT ( 'NONE',  ( 7.452983947829999956, 1488.341756661690169, 200.6284170905290125 ) ) ;
#83830=CARTESIAN_POINT ( 'NONE',  ( 3.242220536386509977, 1430.716549863509954, 218.0395271528590229 ) ) ;
#83837=ORIENTED_EDGE ( 'NONE', *, *, #49384, .T. ) ;
#83841=CARTESIAN_POINT ( 'NONE',  ( -17.05002540721839921, 1508.551704408389924, 212.5108514724210238 ) ) ;
#83842=AXIS2_PLACEMENT_3D ( 'NONE', #966, #27248, #86597 ) ;
#83845=CARTESIAN_POINT ( 'NONE',  ( -2.410378730680590387, 1422.953362613660147, 191.3737400771369721 ) ) ;
#83846=CARTESIAN_POINT ( 'NONE',  ( -11.35024028979760047, 1471.051957719560050, 207.9336051671150187 ) ) ;
#83847=CARTESIAN_POINT ( 'NONE',  ( -7.393903476774015715, 1508.404769111208452, 219.6263016596369937 ) ) ;
#83852=CARTESIAN_POINT ( 'NONE',  ( -10.03887960096509957, 1471.216923981430227, 211.3304923876179942 ) ) ;
#83861=CARTESIAN_POINT ( 'NONE',  ( -12.51045652733512981, 1414.677402202029953, 206.7437175916260230 ) ) ;
#83867=CARTESIAN_POINT ( 'NONE',  ( 10.78559096389430039, 1490.798478570170118, 211.2342276834129962 ) ) ;
#83868=CARTESIAN_POINT ( 'NONE',  ( 1.117082004689999852, 1456.189923892289926, 218.9231241165990127 ) ) ;
#83874=CARTESIAN_POINT ( 'NONE',  ( 4.913312227257480735, 1508.551704408389924, 206.0253317281220120 ) ) ;
#83877=CYLINDRICAL_SURFACE ( 'NONE', #9918, 0.4999999999999909517 ) ;
#83878=CARTESIAN_POINT ( 'NONE',  ( -2.849563100782699809, 1515.551843419129909, 205.1388868728199952 ) ) ;
#83882=CARTESIAN_POINT ( 'NONE',  ( -7.039396212389999796, 1462.541328984289976, 202.2656929340689942 ) ) ;
#83884=CARTESIAN_POINT ( 'NONE',  ( 0.7784496931670009667, 1443.289378548789955, 202.9161012966990256 ) ) ;
#83886=CARTESIAN_POINT ( 'NONE',  ( -16.00433963532579895, 1508.551704408389924, 213.8256925265339987 ) ) ;
#83890=CARTESIAN_POINT ( 'NONE',  ( 5.802908049555659531, 1433.707189344080007, 202.5774238276749770 ) ) ;
#83899=VECTOR ( 'NONE', #65050, 1000.000000000000227 ) ;
#83901=LINE ( 'NONE', #41910, #33785 ) ;
#83902=CARTESIAN_POINT ( 'NONE',  ( 1.521671328670000101, 1476.675504237689893, 198.4650445948989841 ) ) ;
#83907=CARTESIAN_POINT ( 'NONE',  ( 0.9710166503239879843, 1429.611445877699907, 217.3767824417549832 ) ) ;
#83908=CARTESIAN_POINT ( 'NONE',  ( -8.619814553459999473, 1424.664384728270079, 205.6756477520589783 ) ) ;
#83914=CARTESIAN_POINT ( 'NONE',  ( 7.486382904747519440, 1425.304133027429998, 212.2744240526909891 ) ) ;
#83925=CARTESIAN_POINT ( 'NONE',  ( -1.555712611759999975, 1486.517518480790159, 220.5567381263990114 ) ) ;
#83929=CARTESIAN_POINT ( 'NONE',  ( 12.17073519972539941, 1499.730396604210000, 205.6506567772970016 ) ) ;
#83931=CARTESIAN_POINT ( 'NONE',  ( 10.86917929760000057, 1461.683381044490034, 210.6457789368390081 ) ) ;
#83942=CARTESIAN_POINT ( 'NONE',  ( 3.273053440758749932, 1508.551704408389924, 214.1089286421269833 ) ) ;
#83943=ORIENTED_EDGE ( 'NONE', *, *, #90708, .T. ) ;
#83946=CARTESIAN_POINT ( 'NONE',  ( -7.544775971910000045, 1425.914422796229928, 205.6924955586589761 ) ) ;
#83953=CARTESIAN_POINT ( 'NONE',  ( -10.47089315501180096, 1479.680542141990145, 209.9211099033080075 ) ) ;
#83956=CARTESIAN_POINT ( 'NONE',  ( -3.136939361362319989, 1508.551704408389924, 214.0246383682069791 ) ) ;
#83957=CARTESIAN_POINT ( 'NONE',  ( 11.45359756358510062, 1502.235480409970023, 214.6720392030410096 ) ) ;
#83958=CARTESIAN_POINT ( 'NONE',  ( 7.393048916919999769, 1422.547170412949981, 195.6029701833990089 ) ) ;
#83959=CARTESIAN_POINT ( 'NONE',  ( -1.155858387869529880, 1432.298546261019965, 218.5606594621140175 ) ) ;
#83960=CARTESIAN_POINT ( 'NONE',  ( 10.50353041784589969, 1479.239315140000144, 205.9928938130530014 ) ) ;
#83967=ORIENTED_EDGE ( 'NONE', *, *, #48772, .F. ) ;
#83974=CARTESIAN_POINT ( 'NONE',  ( 11.93448652393150056, 1426.000812207319996, 202.8330995219750150 ) ) ;
#83975=CARTESIAN_POINT ( 'NONE',  ( -10.88408651048750109, 1462.776658813379981, 207.1941354553020176 ) ) ;
#83977=CIRCLE ( 'NONE', #73204, 0.5001123349366123350 ) ;
#83980=CARTESIAN_POINT ( 'NONE',  ( 2.952248067976335655, 1431.436657857991577, 200.0252705656226908 ) ) ;
#83982=CARTESIAN_POINT ( 'NONE',  ( -10.57062719580679833, 1462.108563417960113, 209.4792213203020026 ) ) ;
#83986=CARTESIAN_POINT ( 'NONE',  ( 7.711490135329969853, 1466.076247724719906, 215.4504701760220087 ) ) ;
#83988=CARTESIAN_POINT ( 'NONE',  ( 4.356015308734789926, 1474.202971721140102, 219.6788459741880217 ) ) ;
#83994=CARTESIAN_POINT ( 'NONE',  ( 1.842962231260000028, 1515.492058413689847, 204.9833025705389957 ) ) ;
#83996=CARTESIAN_POINT ( 'NONE',  ( -8.627754931006530015, 1437.492696044950208, 228.3379672962190057 ) ) ;
#83998=CARTESIAN_POINT ( 'NONE',  ( -18.08215423386650045, 1419.595351661949962, 206.0399610832670021 ) ) ;
#84009=CARTESIAN_POINT ( 'NONE',  ( 10.02421119480000122, 1480.534221758890226, 205.8829018067289951 ) ) ;
#84012=CARTESIAN_POINT ( 'NONE',  ( 6.692730968182499574, 1468.376655453269905, 207.5243187692509821 ) ) ;
#84020=CARTESIAN_POINT ( 'NONE',  ( 10.99360220178390080, 1422.464694587929898, 207.9550673526719891 ) ) ;
#84021=ORIENTED_EDGE ( 'NONE', *, *, #43794, .T. ) ;
#84025=CARTESIAN_POINT ( 'NONE',  ( 5.456719627610000067, 1455.595244131089885, 218.2350948550090095 ) ) ;
#84027=CARTESIAN_POINT ( 'NONE',  ( 2.642967448119999840, 1474.430884426989905, 219.8158656094990135 ) ) ;
#84030=CARTESIAN_POINT ( 'NONE',  ( -10.94209231895430179, 1492.979988125699947, 207.3926202358989883 ) ) ;
#84031=AXIS2_PLACEMENT_3D ( 'NONE', #64927, #47563, #66593 ) ;
#84037=CARTESIAN_POINT ( 'NONE',  ( 7.350381515560000523, 1447.407902261689969, 203.5674967681089811 ) ) ;
#84040=CARTESIAN_POINT ( 'NONE',  ( -3.389496885370000268, 1455.558964272489902, 200.3052646134590304 ) ) ;
#84043=EDGE_LOOP ( 'NONE', ( #66523, #96460, #36436, #9147 ) ) ;
#84048=CARTESIAN_POINT ( 'NONE',  ( -17.49566125220889745, 1417.678474892549957, 206.5987077655250062 ) ) ;
#84051=CARTESIAN_POINT ( 'NONE',  ( 11.58467648010000062, 1500.424311713589987, 206.6405206915289909 ) ) ;
#84065=CARTESIAN_POINT ( 'NONE',  ( -22.19117979949999864, 1483.602007700189915, 216.8115292462290142 ) ) ;
#84071=CARTESIAN_POINT ( 'NONE',  ( 10.50325117827930121, 1452.939424683670040, 210.5253075612140208 ) ) ;
#84073=CARTESIAN_POINT ( 'NONE',  ( -9.318301627430487954, 1418.493606820336026, 196.8603084725207566 ) ) ;
#84075=CARTESIAN_POINT ( 'NONE',  ( 3.906031934150000051, 1515.551704408389924, 210.6104729190590206 ) ) ;
#84079=DIRECTION ( 'NONE',  ( 1.000000000000000000, 4.676737444244369870E-15, 0.000000000000000000 ) ) ;
#84082=ORIENTED_EDGE ( 'NONE', *, *, #32981, .T. ) ;
#84091=CARTESIAN_POINT ( 'NONE',  ( 20.54534055259999903, 1497.714303034489831, 214.2326470396490095 ) ) ;
#84099=CARTESIAN_POINT ( 'NONE',  ( 4.349503564207779505, 1466.664839270300035, 198.9308445094160049 ) ) ;
#84102=B_SPLINE_SURFACE_WITH_KNOTS ( 'NONE', 5, 5, ( 
 ( #26384, #9585, #43756, #101421, #58910, #70643 ),
 ( #20187, #61682, #11803, #12338, #54385, #21265 ),
 ( #54924, #55474, #63340, #96920, #97995, #27495 ),
 ( #88518, #45972, #105311, #89600, #2878, #36445 ),
 ( #79032, #46528, #20729, #80106, #95805, #38101 ),
 ( #104760, #11268, #3425, #37556, #71757, #89052 ),
 ( #28603, #28045, #80663, #3977, #97460, #105873 ),
 ( #29154, #72279, #106411, #62235, #87415, #29695 ),
 ( #2333, #70095, #63880, #12893, #47070, #62804 ),
 ( #1774, #35912, #104208, #96361, #19072, #53276 ),
 ( #45430, #44882, #19639, #10710, #53843, #87980 ),
 ( #79574, #36997, #71189, #30795, #82853, #99636 ) ),
 .UNSPECIFIED., .F., .F., .F.,
 ( 6, 3, 3, 6 ),
 ( 6, 6 ),
 ( 12.96038195415450112, 20.44306750080000157, 27.92530488589999749, 32.63944941254549548 ),
 ( -0.0004481616454996779951, 2.000000000000000000 ),
 .UNSPECIFIED. ) ;
#84104=ORIENTED_EDGE ( 'NONE', *, *, #36438, .T. ) ;
#84105=CARTESIAN_POINT ( 'NONE',  ( 0.000000000000000000, 1420.119835273649869, 209.1218459616989946 ) ) ;
#84110=CARTESIAN_POINT ( 'NONE',  ( -12.04464620951310039, 1501.663624780660030, 211.4747504816580204 ) ) ;
#84114=CARTESIAN_POINT ( 'NONE',  ( 0.7957076353959989801, 1507.773683908890007, 220.9213704339990159 ) ) ;
#84116=CARTESIAN_POINT ( 'NONE',  ( -3.795106648980000053, 1436.657525481489984, 227.2555632666989993 ) ) ;
#84117=CARTESIAN_POINT ( 'NONE',  ( -6.669163846439519538, 1441.537731776070132, 202.6633789087379967 ) ) ;
#84118=CARTESIAN_POINT ( 'NONE',  ( -18.83642247210000065, 1444.248298674089938, 209.1218459616989946 ) ) ;
#84119=CARTESIAN_POINT ( 'NONE',  ( -7.986570398085929057, 1425.428834413810137, 204.3462609999209860 ) ) ;
#84133=VECTOR ( 'NONE', #92911, 1000.000000000000000 ) ;
#84134=CARTESIAN_POINT ( 'NONE',  ( -14.20524777670000027, 1416.384019283110092, 203.1488900704489993 ) ) ;
#84138=CARTESIAN_POINT ( 'NONE',  ( -16.52203042950529976, 1419.645406836163829, 209.2874580465681902 ) ) ;
#84139=CARTESIAN_POINT ( 'NONE',  ( -9.358593017869999642, 1499.345927103390068, 216.6356661042690064 ) ) ;
#84140=CARTESIAN_POINT ( 'NONE',  ( -4.623067421070000016, 1470.601194648889987, 189.6761541078989808 ) ) ;
#84141=CARTESIAN_POINT ( 'NONE',  ( -18.73855303819999918, 1441.999967869690181, 210.0191439483600107 ) ) ;
#84144=DIRECTION ( 'NONE',  ( 0.9996573249755517088, 0.02617694830808744988, 0.000000000000000000 ) ) ;
#84160=CARTESIAN_POINT ( 'NONE',  ( -8.388522766530359220, 1438.665884974980145, 228.5043048793920093 ) ) ;
#84162=CARTESIAN_POINT ( 'NONE',  ( 8.129480593693450885, 1461.711641629619862, 228.8738001905419992 ) ) ;
#84164=AXIS2_PLACEMENT_3D ( 'NONE', #14203, #5828, #108274 ) ;
#84169=CARTESIAN_POINT ( 'NONE',  ( 8.600728112939199477, 1449.621004864970018, 203.3312769315649859 ) ) ;
#84171=CIRCLE ( 'NONE', #46655, 7.799999999999999822 ) ;
#84174=DIRECTION ( 'NONE',  ( 9.120238070098449704E-47, -1.000000000000000000, 1.836970198721029688E-16 ) ) ;
#84175=B_SPLINE_CURVE_WITH_KNOTS ( 'NONE', 3,
 ( #93488, #58806, #110300, #49311, #16758, #58263 ),
 .UNSPECIFIED., .F., .F.,
 ( 4, 2, 4 ),
 ( 0.000000000000000000, 0.5000000000000000000, 1.000000000000000000 ),
 .UNSPECIFIED. ) ;
#84181=VERTEX_POINT ( 'NONE', #81873 ) ;
#84182=ORIENTED_EDGE ( 'NONE', *, *, #55600, .F. ) ;
#84186=CARTESIAN_POINT ( 'NONE',  ( -18.15654714260000091, 1466.352650648189865, 200.0994765531190183 ) ) ;
#84189=CARTESIAN_POINT ( 'NONE',  ( 0.3721991211270009869, 1444.512068895790208, 199.7834513889890218 ) ) ;
#84195=CARTESIAN_POINT ( 'NONE',  ( -4.291074684768139136, 1463.648453777529994, 200.1571786948010185 ) ) ;
#84205=ORIENTED_EDGE ( 'NONE', *, *, #30305, .F. ) ;
#84213=CARTESIAN_POINT ( 'NONE',  ( -13.31089767809999991, 1503.456584348290107, 208.6977459381109838 ) ) ;
#84228=CARTESIAN_POINT ( 'NONE',  ( 6.163562822530000318, 1453.283431879389809, 216.1943447892690244 ) ) ;
#84233=CARTESIAN_POINT ( 'NONE',  ( 17.12862684171479799, 1428.407653715900096, 203.1217192725700045 ) ) ;
#84238=CARTESIAN_POINT ( 'NONE',  ( 9.404231802118440342, 1434.496204735389938, 206.4601034896920169 ) ) ;
#84239=CARTESIAN_POINT ( 'NONE',  ( 0.000000000000000000, 1391.913060387289988, 209.1218459616989946 ) ) ;
#84240=VECTOR ( 'NONE', #48406, 1000.000000000000000 ) ;
#84248=CARTESIAN_POINT ( 'NONE',  ( -14.17232384770000131, 1420.119835273649869, 215.1506258166890007 ) ) ;
#84250=CARTESIAN_POINT ( 'NONE',  ( 0.5112448275903194173, 1494.259742798005163, 220.2441603401746022 ) ) ;
#84252=CARTESIAN_POINT ( 'NONE',  ( -4.602356253840000022, 1468.583955076089978, 189.7619545879989857 ) ) ;
#84257=CARTESIAN_POINT ( 'NONE',  ( -9.300631542242799199, 1448.922893710790049, 209.3136721124899964 ) ) ;
#84259=VERTEX_POINT ( 'NONE', #21942 ) ;
#84266=CARTESIAN_POINT ( 'NONE',  ( 4.165856372939999552, 1466.952023279489822, 218.2924068021489745 ) ) ;
#84277=CIRCLE ( 'NONE', #73593, 3.458500000000000352 ) ;
#84279=ORIENTED_EDGE ( 'NONE', *, *, #2290, .F. ) ;
#84280=CARTESIAN_POINT ( 'NONE',  ( -8.021408998099778032, 1439.374425103640078, 205.6230372236330197 ) ) ;
#84298=CARTESIAN_POINT ( 'NONE',  ( 6.922360974429970794E-17, 1415.677402202029953, 209.1218459616989946 ) ) ;
#84303=CARTESIAN_POINT ( 'NONE',  ( 4.899054846310000322, 1455.523628246389990, 218.0750725402190255 ) ) ;
#84305=CARTESIAN_POINT ( 'NONE',  ( -1.329478768440000014, 1444.143597569490112, 218.0942856802089977 ) ) ;
#84327=DIRECTION ( 'NONE',  ( -9.153092986051941045E-47, 1.000000000000000000, -1.836970198721029688E-16 ) ) ;
#84330=CARTESIAN_POINT ( 'NONE',  ( -8.732873948900369498, 1448.331813658970077, 211.7966235495169940 ) ) ;
#84337=ADVANCED_FACE ( 'NONE', ( #14111 ), #15740, .T. ) ;
#84340=CARTESIAN_POINT ( 'NONE',  ( 5.972104285402170198, 1424.417304221970198, 193.5739037265429943 ) ) ;
#84349=ADVANCED_FACE ( 'NONE', ( #41541 ), #83070, .T. ) ;
#84356=ORIENTED_EDGE ( 'NONE', *, *, #17976, .T. ) ;
#84357=CARTESIAN_POINT ( 'NONE',  ( 4.124127541549999165, 1440.791920158089852, 218.1322488136489994 ) ) ;
#84361=CARTESIAN_POINT ( 'NONE',  ( -1.542835357908670213, 1425.203189277900037, 191.1789319604989714 ) ) ;
#84378=ORIENTED_EDGE ( 'NONE', *, *, #26100, .T. ) ;
#84379=CARTESIAN_POINT ( 'NONE',  ( 20.16980298980000086, 1476.181277814190025, 211.1145665738389710 ) ) ;
#84383=CARTESIAN_POINT ( 'NONE',  ( -12.28650587490000134, 1415.606339304159974, 207.8979284120589739 ) ) ;
#84385=CARTESIAN_POINT ( 'NONE',  ( 4.229271784049999816, 1486.647279628789875, 199.0365265047990135 ) ) ;
#84386=CARTESIAN_POINT ( 'NONE',  ( 4.815666442453239604, 1430.144935948600050, 217.2987612619500055 ) ) ;
#84388=EDGE_CURVE ( 'NONE', #51752, #77903, #88503, .T. ) ;
#84395=CARTESIAN_POINT ( 'NONE',  ( -16.43158760069999857, 1420.644935630800092, 203.2808212549389850 ) ) ;
#84398=CARTESIAN_POINT ( 'NONE',  ( 0.2114266107359989988, 1473.440120809589871, 219.3699305249989777 ) ) ;
#84400=CARTESIAN_POINT ( 'NONE',  ( -2.795964621609999590, 1422.864594294989956, 191.4386244948990168 ) ) ;
#84401=DIRECTION ( 'NONE',  ( 0.3463916474862910877, -0.4475252625663905248, -0.8244598024868261543 ) ) ;
#84402=CARTESIAN_POINT ( 'NONE',  ( -6.383994317592076584, 1508.334478455586122, 219.9868654066591773 ) ) ;
#84407=CARTESIAN_POINT ( 'NONE',  ( -6.335383617200819550, 1419.419978031070059, 194.8118966042659963 ) ) ;
#84408=CARTESIAN_POINT ( 'NONE',  ( -4.869818399669999742, 1491.215867106689984, 188.8099941780989752 ) ) ;
#84420=DIRECTION ( 'NONE',  ( -0.6205445805634668410, -0.7071067811868648745, 0.3390050494208930454 ) ) ;
#84425=CARTESIAN_POINT ( 'NONE',  ( 10.04089988029999958, 1469.832478305790119, 209.8601729685539965 ) ) ;
#84426=CARTESIAN_POINT ( 'NONE',  ( 10.90104120139269916, 1491.125730471760107, 210.6098627452870176 ) ) ;
#84427=CARTESIAN_POINT ( 'NONE',  ( 1.423783606090000209, 1455.243702336090109, 218.4445187910790196 ) ) ;
#84436=B_SPLINE_CURVE_WITH_KNOTS ( 'NONE', 3,
 ( #67620, #59769, #83299, #41303, #83847, #8227, #17156, #108501, #58115, #68187, #49165, #40743, #25575, #76001, #93890, #7146, #75476, #31787, #74919, #92248, #84402, #51348, #109609, #59225, #109069, #32883, #24474, #67074, #101179, #110153, #33424, #25022, #58662, #32351, #50272, #100634, #92798, #85481, #93341, #16069, #16607, #50804, #84934, #40193, #42393, #76548, #57572, #74375, #65978, #100101, #23381, #43517, #42961, #17714, #60317, #70396, #77122, #86058 ),
 .UNSPECIFIED., .F., .F.,
 ( 4, 2, 2, 1, 1, 1, 2, 2, 2, 1, 1, 1, 1, 2, 2, 2, 2, 2, 1, 1, 2, 2, 2, 1, 1, 1, 1, 2, 2, 2, 2, 1, 1, 1, 2, 2, 4 ),
 ( 0.000000000000000000, 0.06249999999997843392, 0.09374999999996395939, 0.1093749999999522465, 0.1171874999999481665, 0.1210937499999469452, 0.1230468749999446831, 0.1249999999999424072, 0.1874999999998670508, 0.2187499999998282207, 0.2343749999998072653, 0.2421874999997992994, 0.2460937499997886690, 0.2480468749997860878, 0.2499999999997835343, 0.3749999999996027067, 0.4374999999995103361, 0.4687499999994658162, 0.4843749999994422240, 0.4921874999994306221, 0.4960937499994216848, 0.4999999999994128030, 0.5624999999992654764, 0.5937499999991936450, 0.6093749999991554533, 0.6171874999991310284, 0.6210937499991219246, 0.6230468749991209254, 0.6249999999991199262, 0.6874999999992971178, 0.7187499999993872679, 0.7343749999994357847, 0.7421874999994599875, 0.7460937499994694244, 0.7480468749994741984, 0.7499999999994789723, 1.000000000000000000 ),
 .UNSPECIFIED. ) ;
#84441=CARTESIAN_POINT ( 'NONE',  ( -9.400435900700001568, 1463.222323258790311, 204.0377083383889953 ) ) ;
#84445=CARTESIAN_POINT ( 'NONE',  ( -2.195064489079999959, 1456.689498309789997, 202.6654703318990300 ) ) ;
#84447=CARTESIAN_POINT ( 'NONE',  ( -0.5794993947522789624, 1485.974153057100011, 197.2331900926350272 ) ) ;
#84448=CARTESIAN_POINT ( 'NONE',  ( 3.566694622846560137, 1432.299330911419929, 200.9781325985559874 ) ) ;
#84452=ORIENTED_EDGE ( 'NONE', *, *, #96111, .F. ) ;
#84453=CARTESIAN_POINT ( 'NONE',  ( -19.79636808800000125, 1468.588933445289967, 204.4688411793389946 ) ) ;
#84461=CARTESIAN_POINT ( 'NONE',  ( 0.7400002793700010129, 1477.398841704889946, 198.7251293859989971 ) ) ;
#84467=CARTESIAN_POINT ( 'NONE',  ( -7.737164119570000054, 1425.957155233719959, 206.5199506646890200 ) ) ;
#84472=CARTESIAN_POINT ( 'NONE',  ( 7.495651997220180718, 1425.996480991439967, 212.3299467758739922 ) ) ;
#84476=CARTESIAN_POINT ( 'NONE',  ( -11.05827631052790139, 1492.152225823860135, 207.1157292965639840 ) ) ;
#84478=CARTESIAN_POINT ( 'NONE',  ( -19.70220409820000285, 1465.426396456590055, 207.1886372403690189 ) ) ;
#84479=CARTESIAN_POINT ( 'NONE',  ( -16.38962540390479816, 1508.551704408489968, 213.5063151782250088 ) ) ;
#84480=CARTESIAN_POINT ( 'NONE',  ( 8.192509002470000468, 1427.073616020289819, 211.9190997776489951 ) ) ;
#84488=ORIENTED_EDGE ( 'NONE', *, *, #29894, .T. ) ;
#84506=ADVANCED_FACE ( 'NONE', ( #7115 ), #77800, .F. ) ;
#84507=CARTESIAN_POINT ( 'NONE',  ( 5.390485732382727768, 1434.547431617676921, 202.5152773920257800 ) ) ;
#84508=CARTESIAN_POINT ( 'NONE',  ( -3.626138226838250045, 1508.551704408389924, 213.8360464113480077 ) ) ;
#84509=CARTESIAN_POINT ( 'NONE',  ( 8.172889386072169415, 1503.933201077479907, 218.9089046230789961 ) ) ;
#84510=ADVANCED_FACE ( 'NONE', ( #7657 ), #92020, .T. ) ;
#84511=CARTESIAN_POINT ( 'NONE',  ( 7.468327728180000236, 1422.304606718539844, 195.6660984653989885 ) ) ;
#84513=CARTESIAN_POINT ( 'NONE',  ( 10.09505638416009887, 1480.032748459799905, 205.9636802426639974 ) ) ;
#84524=CARTESIAN_POINT ( 'NONE',  ( -10.59266146615069992, 1483.275693043989804, 203.6749203483539929 ) ) ;
#84525=EDGE_CURVE ( 'NONE', #7222, #32267, #41021, .T. ) ;
#84527=CARTESIAN_POINT ( 'NONE',  ( 9.345988979242928707, 1422.635736885719780, 212.8844760481530045 ) ) ;
#84528=CARTESIAN_POINT ( 'NONE',  ( 11.46771554947700089, 1425.480055491239909, 202.9414045442640031 ) ) ;
#84529=CARTESIAN_POINT ( 'NONE',  ( -11.02103722150159903, 1462.518561201050034, 208.4069885853160145 ) ) ;
#84533=LINE ( 'NONE', #57160, #91568 ) ;
#84536=CARTESIAN_POINT ( 'NONE',  ( 12.24079733762730093, 1421.235242715860068, 203.4476007142680203 ) ) ;
#84537=CARTESIAN_POINT ( 'NONE',  ( 6.713874036901299469, 1465.139200243409960, 217.4101378742359998 ) ) ;
#84545=CARTESIAN_POINT ( 'NONE',  ( 9.279405586231710856, 1450.853110869679995, 207.7367179206380001 ) ) ;
#84547=CARTESIAN_POINT ( 'NONE',  ( -9.573037427669609301, 1423.427966565790030, 192.3355729243529879 ) ) ;
#84550=CARTESIAN_POINT ( 'NONE',  ( -14.68398163311469951, 1420.764401514960127, 209.3424412080640025 ) ) ;
#84561=DIRECTION ( 'NONE',  ( 0.8775825618903763115, 0.000000000000000000, -0.4794255386041963996 ) ) ;
#84563=CARTESIAN_POINT ( 'NONE',  ( 1.514120561980000183E-16, 1515.551704408389924, 209.1218459616989946 ) ) ;
#84564=CARTESIAN_POINT ( 'NONE',  ( -0.5682668705760020034, 1506.801775235190007, 221.9434713837989932 ) ) ;
#84571=CARTESIAN_POINT ( 'NONE',  ( 11.08034903154059947, 1427.227500383180086, 208.8464042652539945 ) ) ;
#84577=DIRECTION ( 'NONE',  ( 9.341989762165448955E-47, -1.000000000000000000, 1.836970198721029688E-16 ) ) ;
#84578=CARTESIAN_POINT ( 'NONE',  ( 18.17556130014969895, 1429.975338228749933, 210.2973223115409951 ) ) ;
#84580=CARTESIAN_POINT ( 'NONE',  ( -11.00351831549999915, 1492.170254952789946, 204.4829265568189953 ) ) ;
#84584=FACE_OUTER_BOUND ( 'NONE', #71732, .T. ) ;
#84585=CARTESIAN_POINT ( 'NONE',  ( 9.348472636800000402, 1450.695831709190088, 206.5041896299389919 ) ) ;
#84588=CARTESIAN_POINT ( 'NONE',  ( -2.418203496729999902, 1454.903534402890045, 199.2876688155090221 ) ) ;
#84591=ORIENTED_EDGE ( 'NONE', *, *, #14729, .T. ) ;
#84592=CARTESIAN_POINT ( 'NONE',  ( -1.682837345762272729, 1464.049852190644287, 199.4516691750211521 ) ) ;
#84593=CARTESIAN_POINT ( 'NONE',  ( -2.911830323659999831, 1496.243737683489826, 197.8821088022990011 ) ) ;
#84606=CARTESIAN_POINT ( 'NONE',  ( 10.89260962470000038, 1478.390639884389884, 204.6475587744990037 ) ) ;
#84612=CARTESIAN_POINT ( 'NONE',  ( -18.29179302776010019, 1466.060351544859941, 217.7541585804449937 ) ) ;
#84619=CARTESIAN_POINT ( 'NONE',  ( -13.58885879944450004, 1508.451085982560016, 209.7742480560209799 ) ) ;
#84620=CARTESIAN_POINT ( 'NONE',  ( 4.326992699839999901, 1515.158586648489973, 209.4786834863980118 ) ) ;
#84621=CARTESIAN_POINT ( 'NONE',  ( -5.906564182353549519, 1454.472896573619892, 201.8136876099350161 ) ) ;
#84630=ORIENTED_EDGE ( 'NONE', *, *, #96749, .F. ) ;
#84633=ORIENTED_EDGE ( 'NONE', *, *, #23551, .F. ) ;
#84637=CARTESIAN_POINT ( 'NONE',  ( -17.30321976762949987, 1420.074570463099917, 205.0181995903979839 ) ) ;
#84638=CARTESIAN_POINT ( 'NONE',  ( -3.660324660266798702, 1488.780526855528251, 219.3830879640146350 ) ) ;
#84639=B_SPLINE_CURVE_WITH_KNOTS ( 'NONE', 3,
 ( #53368, #9679, #36003, #70196, #10803, #43848, #74845, #32273, #17503, #51702, #1300, #34883, #80759, #72912, #21909, #62907, #89152, #45531, #4602, #12440, #105410, #88073, #29248, #71854, #11900, #4067, #46625, #38192, #54483, #11360, #79671, #28702, #46074, #106503, #98091, #19738, #72374, #104854, #80206, #88620, #29792, #3524, #44973, #2976, #37094, #71296, #97018 ),
 .UNSPECIFIED., .F., .F.,
 ( 4, 2, 1, 1, 1, 2, 2, 2, 1, 1, 1, 1, 2, 2, 2, 1, 1, 1, 2, 2, 2, 1, 2, 2, 2, 1, 1, 2, 2, 4 ),
 ( 0.000000000000000000, 0.06249999999977556842, 0.09374999999964436781, 0.1093749999995976691, 0.1171874999995746874, 0.1210937499995635575, 0.1249999999995524136, 0.1874999999989931387, 0.2187499999986940447, 0.2343749999985445254, 0.2421874999984697518, 0.2460937499984326982, 0.2480468749984321430, 0.2499999999984315602, 0.3124999999987914667, 0.3437499999989717669, 0.3593749999990795141, 0.3671874999991333044, 0.3710937499991602273, 0.3749999999991870947, 0.4374999999993113287, 0.4687499999993546829, 0.4843749999993763877, 0.4999999999993980371, 0.6249999999994978461, 0.6874999999995653477, 0.7187499999995988764, 0.7343749999996155298, 0.7499999999996322941, 1.000000000000000000 ),
 .UNSPECIFIED. ) ;
#84642=CARTESIAN_POINT ( 'NONE',  ( -9.165442406359998628, 1473.716948313090143, 204.3954301531890110 ) ) ;
#84643=CARTESIAN_POINT ( 'NONE',  ( 6.766670517840000620, 1494.440262355989717, 218.9700614872689926 ) ) ;
#84656=CARTESIAN_POINT ( 'NONE',  ( -4.325405441708600307, 1515.219201591195315, 211.4519800884384608 ) ) ;
#84659=CARTESIAN_POINT ( 'NONE',  ( 0.6929005668539989227, 1508.551703792989883, 220.2186279790989829 ) ) ;
#84662=CARTESIAN_POINT ( 'NONE',  ( 1.639265462144630092, 1430.995086660350125, 199.7986407524330161 ) ) ;
#84663=CARTESIAN_POINT ( 'NONE',  ( -10.92959825596109980, 1462.004401642820085, 210.4728761127730081 ) ) ;
#84664=CARTESIAN_POINT ( 'NONE',  ( 2.968865197519999555, 1449.559759134390106, 190.1955703363989869 ) ) ;
#84666=CARTESIAN_POINT ( 'NONE',  ( 11.13973213087689906, 1470.272412021129867, 206.9146623043149873 ) ) ;
#84668=CARTESIAN_POINT ( 'NONE',  ( -10.37387122080000168, 1479.853456435389944, 210.7819233329290114 ) ) ;
#84682=CARTESIAN_POINT ( 'NONE',  ( -14.68950664279999963, 1417.178464496219931, 203.9617939164890004 ) ) ;
#84686=CARTESIAN_POINT ( 'NONE',  ( -4.165531658079999922, 1496.711016394489889, 219.7171372811990295 ) ) ;
#84687=CARTESIAN_POINT ( 'NONE',  ( 1.113400972200000005, 1478.239378852390018, 201.5788048326690216 ) ) ;
#84689=CARTESIAN_POINT ( 'NONE',  ( -10.99386358867370106, 1508.551709148380041, 208.1089302384970097 ) ) ;
#84690=CARTESIAN_POINT ( 'NONE',  ( -2.472546487080370170, 1422.360492482099744, 192.6709265187130029 ) ) ;
#84699=CARTESIAN_POINT ( 'NONE',  ( -15.55458060831606382, 1415.677404892448294, 209.5577834297775155 ) ) ;
#84700=CARTESIAN_POINT ( 'NONE',  ( -2.330134126090000368, 1515.551704408389924, 205.2922258481490303 ) ) ;
#84704=CARTESIAN_POINT ( 'NONE',  ( 4.702100396339999655, 1484.396536161289987, 219.5556203100990160 ) ) ;
#84706=CARTESIAN_POINT ( 'NONE',  ( 10.35103189252669864, 1480.844217530770038, 207.0564529105199938 ) ) ;
#84707=CARTESIAN_POINT ( 'NONE',  ( -5.790397269885580123, 1452.878744171119934, 206.0071839347059779 ) ) ;
#84708=CARTESIAN_POINT ( 'NONE',  ( -19.40999286329999762, 1446.496631621190090, 200.0861365869990038 ) ) ;
#84710=CARTESIAN_POINT ( 'NONE',  ( -22.19117979951819919, 1483.602007699049864, 216.8115292459999921 ) ) ;
#84714=CARTESIAN_POINT ( 'NONE',  ( -2.469737522550000453, 1507.227429587890128, 221.7265305498989960 ) ) ;
#84721=DIRECTION ( 'NONE',  ( 9.500914144214121536E-47, -1.000000000000000000, 1.836970198721029688E-16 ) ) ;
#84736=CARTESIAN_POINT ( 'NONE',  ( 2.531901238200000126, 1444.224916984790070, 200.5256934874690273 ) ) ;
#84741=CARTESIAN_POINT ( 'NONE',  ( 0.7491281650140010351, 1417.862047144630196, 204.0277727146790028 ) ) ;
#84742=B_SPLINE_SURFACE_WITH_KNOTS ( 'NONE', 5, 5, ( 
 ( #88449, #104139, #87914, #52648, #63277, #10641 ),
 ( #46466, #80598, #1701, #45907, #105814, #3364 ),
 ( #96294, #44808, #72221, #106343, #3913, #86785 ),
 ( #62168, #11201, #27424, #71694, #19574, #61607 ),
 ( #37491, #20660, #20127, #28540, #29629, #53777 ),
 ( #38042, #95190, #45366, #29092, #44249, #2810 ),
 ( #97389, #19004, #36929, #10074, #79505, #54862 ),
 ( #78392, #71126, #2269, #88985, #70026, #18449 ),
 ( #78962, #105247, #62739, #11738, #53204, #87345 ) ),
 .UNSPECIFIED., .F., .F., .F.,
 ( 6, 3, 6 ),
 ( 6, 6 ),
 ( 3.182111802360319874, 6.655162634330000770, 7.748822666508919710 ),
 ( -0.0004160027669829020002, 2.000000000000000000 ),
 .UNSPECIFIED. ) ;
#84747=ORIENTED_EDGE ( 'NONE', *, *, #7727, .T. ) ;
#84750=VERTEX_POINT ( 'NONE', #100487 ) ;
#84751=ORIENTED_EDGE ( 'NONE', *, *, #41192, .T. ) ;
#84758=CARTESIAN_POINT ( 'NONE',  ( 11.73855662635810049, 1421.952273329259924, 209.4052689870339918 ) ) ;
#84768=DIRECTION ( 'NONE',  ( 0.9999994573234139983, 9.540975887252238799E-32, -0.001041802705676339504 ) ) ;
#84773=CARTESIAN_POINT ( 'NONE',  ( 5.641423425050000162, 1453.485726096290136, 216.6286100207389893 ) ) ;
#84775=B_SPLINE_SURFACE_WITH_KNOTS ( 'NONE', 5, 1, ( 
 ( #79233, #106073 ),
 ( #46193, #38303 ),
 ( #96577, #45647 ),
 ( #72484, #62454 ),
 ( #80327, #2542 ),
 ( #10918, #12013 ) ),
 .UNSPECIFIED., .F., .F., .F.,
 ( 6, 6 ),
 ( 2, 2 ),
 ( -3.552713678800000397E-15, 17.98770270289999829 ),
 ( 0.000000000000000000, 14.00000000000000000 ),
 .UNSPECIFIED. ) ;
#84777=CARTESIAN_POINT ( 'NONE',  ( -2.739337719001559979, 1429.065489528160015, 200.1608258868419910 ) ) ;
#84782=CARTESIAN_POINT ( 'NONE',  ( 9.760716701452610167, 1435.124984824069998, 208.1605893237319833 ) ) ;
#84791=CARTESIAN_POINT ( 'NONE',  ( -2.373667526830000263, 1462.975913846089952, 202.4942268867290238 ) ) ;
#84805=CARTESIAN_POINT ( 'NONE',  ( -1.142849984530000196, 1443.644273027190138, 218.3503460313989990 ) ) ;
#84815=CARTESIAN_POINT ( 'NONE',  ( 9.698064461892839105, 1462.705242386489999, 208.0596150282290182 ) ) ;
#84817=CARTESIAN_POINT ( 'NONE',  ( 11.40070752235540041, 1470.941042065359852, 209.0206955636659814 ) ) ;
#84822=CARTESIAN_POINT ( 'NONE',  ( 7.106794650369999466, 1425.525179449380175, 212.0614358484589843 ) ) ;
#84823=CARTESIAN_POINT ( 'NONE',  ( -2.936816566051450028, 1515.374151772610048, 213.3816236500609875 ) ) ;
#84829=EDGE_LOOP ( 'NONE', ( #79676, #95858, #69078, #46960 ) ) ;
#84832=CARTESIAN_POINT ( 'NONE',  ( 4.141698392683508700, 1493.371568340419344, 219.5018937535342900 ) ) ;
#84835=CARTESIAN_POINT ( 'NONE',  ( -8.881784197000000993E-16, 1414.413060387330006, 209.1218459616989946 ) ) ;
#84839=CARTESIAN_POINT ( 'NONE',  ( -1.676218328139999825, 1445.210232295889909, 217.9771989461590351 ) ) ;
#84847=CARTESIAN_POINT ( 'NONE',  ( -6.519909027102049670, 1477.757526204120040, 213.0818532017610210 ) ) ;
#84860=CARTESIAN_POINT ( 'NONE',  ( -2.476313965196780043, 1475.157094210569994, 197.9550708103259922 ) ) ;
#84864=CARTESIAN_POINT ( 'NONE',  ( -10.28551112630600173, 1447.520881842850031, 210.2972423999289902 ) ) ;
#84875=CARTESIAN_POINT ( 'NONE',  ( 5.178343518078389884, 1424.209805733240046, 193.3007077610879776 ) ) ;
#84881=VERTEX_POINT ( 'NONE', #32734 ) ;
#84883=B_SPLINE_CURVE_WITH_KNOTS ( 'NONE', 5,
 ( #89375, #44632, #2641, #87740, #80431, #12667, #69846, #19391, #106176, #53034, #104521, #1523, #103964, #78211, #11018 ),
 .UNSPECIFIED., .F., .F.,
 ( 6, 3, 3, 3, 6 ),
 ( 0.000000000000000000, 0.1200066420014513496, 0.2400132840077169871, 0.4800265680154341408, 1.000000000000000000 ),
 .UNSPECIFIED. ) ;
#84895=CARTESIAN_POINT ( 'NONE',  ( 19.32263322520000060, 1455.378559704889767, 209.1218459616989946 ) ) ;
#84899=CARTESIAN_POINT ( 'NONE',  ( 10.41177329615350011, 1460.024665156439823, 205.9063136364349873 ) ) ;
#84911=CARTESIAN_POINT ( 'NONE',  ( 7.358001737349999516, 1481.503913299690112, 209.0774419860809985 ) ) ;
#84918=CARTESIAN_POINT ( 'NONE',  ( 3.689783165729999759, 1486.815214840489944, 198.5515965981990121 ) ) ;
#84922=CARTESIAN_POINT ( 'NONE',  ( -1.842963721827329815, 1515.551704300040001, 205.2922259627210053 ) ) ;
#84928=ORIENTED_EDGE ( 'NONE', *, *, #8810, .F. ) ;
#84929=CARTESIAN_POINT ( 'NONE',  ( -17.32162814183379851, 1508.551704408389924, 212.1341644048549995 ) ) ;
#84934=CARTESIAN_POINT ( 'NONE',  ( -4.303904342535483707, 1508.176176452014033, 220.6005507373670014 ) ) ;
#84936=CARTESIAN_POINT ( 'NONE',  ( 5.808294004517759568, 1494.502801637436960, 219.1507311820781752 ) ) ;
#84938=FACE_OUTER_BOUND ( 'NONE', #48825, .T. ) ;
#84940=CARTESIAN_POINT ( 'NONE',  ( -2.379179684863220068, 1422.184173668060112, 193.0946223031349689 ) ) ;
#84952=CARTESIAN_POINT ( 'NONE',  ( 10.18770750727360053, 1422.434970378240223, 211.9211229168350030 ) ) ;
#84953=CARTESIAN_POINT ( 'NONE',  ( 3.115880651068799967, 1508.551704408389924, 219.3718644903320012 ) ) ;
#84954=CARTESIAN_POINT ( 'NONE',  ( -19.86464703721610192, 1441.435635517049832, 212.6459273959629854 ) ) ;
#84957=CARTESIAN_POINT ( 'NONE',  ( -9.783936650027678539, 1438.409968310599879, 210.7790528106160082 ) ) ;
#84958=CARTESIAN_POINT ( 'NONE',  ( 11.41815806276019885, 1492.743991988549851, 212.4766916504889878 ) ) ;
#84959=CARTESIAN_POINT ( 'NONE',  ( -2.288930271459999943, 1457.528235387290124, 219.1297011245989950 ) ) ;
#84973=CARTESIAN_POINT ( 'NONE',  ( -7.459107715590000076, 1463.395188125190089, 202.0447620364989803 ) ) ;
#84975=CARTESIAN_POINT ( 'NONE',  ( 11.36216713388179933, 1503.110266152410077, 211.0233809544849919 ) ) ;
#84976=CARTESIAN_POINT ( 'NONE',  ( -11.91658583868719923, 1508.551704408389924, 217.2927667623789887 ) ) ;
#84980=CARTESIAN_POINT ( 'NONE',  ( 2.301917092608350313, 1432.768594694289959, 200.9374038220679779 ) ) ;
#84986=CARTESIAN_POINT ( 'NONE',  ( 4.967313642998160361, 1470.582637015879982, 187.7810769942950060 ) ) ;
#84996=CARTESIAN_POINT ( 'NONE',  ( -2.737226383349999903, 1476.451468402690125, 199.1237168845889869 ) ) ;
#85003=CARTESIAN_POINT ( 'NONE',  ( -8.112741595579999299, 1424.858451744329841, 208.8832813207109780 ) ) ;
#85004=EDGE_CURVE ( 'NONE', #22042, #24522, #65313, .T. ) ;
#85010=CARTESIAN_POINT ( 'NONE',  ( 7.279817883549699609, 1426.451502940120008, 212.8375798222039919 ) ) ;
#85017=( BOUNDED_SURFACE ( )  B_SPLINE_SURFACE ( 1, 2, ( 
 ( #58549, #7576, #41731 ),
 ( #50154, #77002, #45627 ) ),
 .UNSPECIFIED., .F., .F., .F. ) 
 B_SPLINE_SURFACE_WITH_KNOTS ( ( 2, 2 ),
 ( 3, 3 ),
 ( -10000.00000000000000, 10000.00000000000000 ),
 ( 5.770213224421889997, 5.870145916345279602 ),
 .UNSPECIFIED. ) 
 GEOMETRIC_REPRESENTATION_ITEM ( )  RATIONAL_B_SPLINE_SURFACE ( (
 ( 0.8711730262222420196, 0.8776363487315159695, 0.8864705793990830252),
 ( 0.8711730262222420196, 0.8776363487315159695, 0.8864705793990830252) ) ) 
 REPRESENTATION_ITEM ( '' )  SURFACE ( )  );
#85020=CARTESIAN_POINT ( 'NONE',  ( 4.811281351129999884, 1423.102872354400233, 207.5441001112789934 ) ) ;
#85027=CARTESIAN_POINT ( 'NONE',  ( 9.401681046103311346, 1434.490268153120041, 206.4448289074559852 ) ) ;
#85032=CARTESIAN_POINT ( 'NONE',  ( -11.87328627558470018, 1482.014094172719979, 208.6022272904490080 ) ) ;
#85037=CARTESIAN_POINT ( 'NONE',  ( 3.961944270670380241, 1508.551704410290085, 213.6667069116419952 ) ) ;
#85046=CARTESIAN_POINT ( 'NONE',  ( 16.48525259900869955, 1431.535382936039923, 217.4038343007140099 ) ) ;
#85048=CARTESIAN_POINT ( 'NONE',  ( 4.487249066482500659, 1509.038643261319976, 206.6339218291419968 ) ) ;
#85049=CARTESIAN_POINT ( 'NONE',  ( 5.866456971857230585, 1434.780192336125992, 202.9178924053972253 ) ) ;
#85050=CARTESIAN_POINT ( 'NONE',  ( -4.932890325499830197, 1508.551704408389924, 212.1343244586070114 ) ) ;
#85052=CARTESIAN_POINT ( 'NONE',  ( 7.345629923129999739, 1422.263538441430001, 195.5717800564989943 ) ) ;
#85053=CARTESIAN_POINT ( 'NONE',  ( -2.901039365278310189, 1433.100862733600252, 218.2186568973889962 ) ) ;
#85068=CARTESIAN_POINT ( 'NONE',  ( 8.758531138563899532, 1427.348527690079891, 211.4847147330029884 ) ) ;
#85069=CARTESIAN_POINT ( 'NONE',  ( 1.598766419041605991, 1421.472867901786003, 193.7976631032935870 ) ) ;
#85077=CARTESIAN_POINT ( 'NONE',  ( -16.83242346257729949, 1420.442304662440165, 203.3407665278299703 ) ) ;
#85079=CARTESIAN_POINT ( 'NONE',  ( 7.695203452936191013, 1464.811393429670034, 216.0057213840310055 ) ) ;
#85082=B_SPLINE_CURVE_WITH_KNOTS ( 'NONE', 5,
 ( #49291, #100757, #48190, #107522, #22947, #30813 ),
 .UNSPECIFIED., .F., .F.,
 ( 6, 6 ),
 ( 302.8993106099999864, 307.9376145470000097 ),
 .UNSPECIFIED. ) ;
#85086=CARTESIAN_POINT ( 'NONE',  ( 0.1128880363801176290, 1477.705586754096430, 198.7092162523474599 ) ) ;
#85089=CARTESIAN_POINT ( 'NONE',  ( 12.73796549575709847, 1426.755042289380071, 204.5610647559049937 ) ) ;
#85090=CARTESIAN_POINT ( 'NONE',  ( -5.221955725866830100, 1489.269540765400052, 185.8916489472570106 ) ) ;
#85093=CARTESIAN_POINT ( 'NONE',  ( -12.46613533405179908, 1422.637669668850094, 203.9783536675730033 ) ) ;
#85110=CARTESIAN_POINT ( 'NONE',  ( -3.967003077310200077, 1433.325234434820004, 217.0778631506990166 ) ) ;
#85112=CARTESIAN_POINT ( 'NONE',  ( -16.20017219800000063, 1416.460102861859923, 208.9420928254820069 ) ) ;
#85117=CARTESIAN_POINT ( 'NONE',  ( 10.17807908018379770, 1423.278369623310027, 208.7639352597529978 ) ) ;
#85124=CARTESIAN_POINT ( 'NONE',  ( 2.587119683470000098, 1473.233209539489962, 219.0154824371090001 ) ) ;
#85125=CARTESIAN_POINT ( 'NONE',  ( 5.871367194876985884, 1422.630051726727743, 194.8466533618984897 ) ) ;
#85132=CARTESIAN_POINT ( 'NONE',  ( 9079.130222195200986, 5181.793945261120825, 1985.491949542980137 ) ) ;
#85133=CARTESIAN_POINT ( 'NONE',  ( 8.789267444210000946, 1449.799573326989957, 205.7427481119990205 ) ) ;
#85138=EDGE_CURVE ( 'NONE', #41237, #13558, #100068, .T. ) ;
#85142=CARTESIAN_POINT ( 'NONE',  ( -1.954686510389999965, 1496.240076336090169, 197.3202119613989964 ) ) ;
#85143=CARTESIAN_POINT ( 'NONE',  ( -0.1165868996460010104, 1494.887927287289813, 220.3098612586990157 ) ) ;
#85144=ORIENTED_EDGE ( 'NONE', *, *, #58223, .T. ) ;
#85149=DIRECTION ( 'NONE',  ( 1.000000000000000000, 0.000000000000000000, 0.000000000000000000 ) ) ;
#85160=CARTESIAN_POINT ( 'NONE',  ( 2.927652146237840203, 1508.551704408389924, 214.0699139930379715 ) ) ;
#85164=CARTESIAN_POINT ( 'NONE',  ( 10.92858942872100059, 1460.889019201350038, 208.5050433691779972 ) ) ;
#85167=ORIENTED_EDGE ( 'NONE', *, *, #62384, .F. ) ;
#85168=ORIENTED_EDGE ( 'NONE', *, *, #65995, .F. ) ;
#85170=CARTESIAN_POINT ( 'NONE',  ( 9.018703368920000685, 1425.148033156689962, 195.5914714850989924 ) ) ;
#85172=CARTESIAN_POINT ( 'NONE',  ( -13.71322468297814723, 1416.698495194484849, 202.0650518266237725 ) ) ;
#85173=EDGE_CURVE ( 'NONE', #96209, #89343, #44640, .T. ) ;
#85174=CARTESIAN_POINT ( 'NONE',  ( 4.123250153539999907, 1515.545045452190152, 209.8706226742160084 ) ) ;
#85178=CARTESIAN_POINT ( 'NONE',  ( 9.246914999585321482, 1451.227871316439860, 209.6132637504499883 ) ) ;
#85185=CARTESIAN_POINT ( 'NONE',  ( 19.31456092990000073, 1455.192895371089890, 208.1952086544899885 ) ) ;
#85191=CARTESIAN_POINT ( 'NONE',  ( -3.624924048459783776, 1488.770799682897859, 219.3952194504361159 ) ) ;
#85195=CARTESIAN_POINT ( 'NONE',  ( 6.042689891000001090, 1492.864352563789907, 218.4381426803390127 ) ) ;
#85201=CARTESIAN_POINT ( 'NONE',  ( -13.96269180912499941, 1502.379650475309973, 226.3091602680140113 ) ) ;
#85208=ORIENTED_EDGE ( 'NONE', *, *, #10863, .T. ) ;
#85210=CARTESIAN_POINT ( 'NONE',  ( -0.3329474806990009861, 1507.873469256489898, 221.0089344693989801 ) ) ;
#85213=CARTESIAN_POINT ( 'NONE',  ( -10.77150947492019917, 1461.758312437779978, 211.3157053564689818 ) ) ;
#85214=CARTESIAN_POINT ( 'NONE',  ( -4.367937192439999450, 1447.898255911189835, 190.6350925615990093 ) ) ;
#85215=CARTESIAN_POINT ( 'NONE',  ( -4.030172342475210279, 1428.333731443729903, 200.6736590918410172 ) ) ;
#85218=CARTESIAN_POINT ( 'NONE',  ( -10.47826420840229922, 1480.900688901569993, 207.8449939762269878 ) ) ;
#85219=CARTESIAN_POINT ( 'NONE',  ( -0.9205759414320010547, 1469.929133752490088, 216.3346150940489849 ) ) ;
#85226=CARTESIAN_POINT ( 'NONE',  ( 4.329448776040000446, 1515.064792882589927, 209.0973262533439936 ) ) ;
#85227=CARTESIAN_POINT ( 'NONE',  ( 4.144002508462048873, 1453.992169703209811, 217.5342908371910084 ) ) ;
#85230=CARTESIAN_POINT ( 'NONE',  ( -14.62060631049999770, 1416.594821258409866, 204.2386896224389830 ) ) ;
#85233=CARTESIAN_POINT ( 'NONE',  ( -16.18859208205868683, 1419.742601152931002, 209.9822759361395015 ) ) ;
#85234=CARTESIAN_POINT ( 'NONE',  ( -4.318206861440000210, 1497.528676090189947, 220.7835062296990145 ) ) ;
#85238=CARTESIAN_POINT ( 'NONE',  ( -11.60674054546250034, 1507.508082460230071, 207.5537236852100023 ) ) ;
#85241=CARTESIAN_POINT ( 'NONE',  ( -5.909698491649999497, 1449.521837735690042, 210.1656816284789784 ) ) ;
#85253=CARTESIAN_POINT ( 'NONE',  ( 3.933180850559999886, 1485.871275756990144, 219.1485422991989935 ) ) ;
#85254=FACE_OUTER_BOUND ( 'NONE', #97303, .T. ) ;
#85255=ADVANCED_FACE ( 'NONE', ( #38594 ), #94775, .T. ) ;
#85256=CARTESIAN_POINT ( 'NONE',  ( -17.33962108957659964, 1446.210180764470124, 200.4727308985020215 ) ) ;
#85258=CARTESIAN_POINT ( 'NONE',  ( 20.40402507730000181, 1433.421378987090065, 214.6266990018290244 ) ) ;
#85264=CARTESIAN_POINT ( 'NONE',  ( 9.687311913827020504, 1436.266597529439878, 210.8265562985189945 ) ) ;
#85265=DIRECTION ( 'NONE',  ( 1.000000000000000000, 0.000000000000000000, 0.000000000000000000 ) ) ;
#85266=CARTESIAN_POINT ( 'NONE',  ( 5.304930756692599836, 1447.452529283679951, 200.4004275134280135 ) ) ;
#85272=CARTESIAN_POINT ( 'NONE',  ( 10.86417644130879978, 1503.361827989980156, 213.1981603545889925 ) ) ;
#85282=CARTESIAN_POINT ( 'NONE',  ( -4.408349274510000804, 1512.051704408390151, 206.7128113371389873 ) ) ;
#85287=CARTESIAN_POINT ( 'NONE',  ( 3.401541474679999677, 1468.225229937389940, 218.5224292272789910 ) ) ;
#85289=( NAMED_UNIT ( * ) SI_UNIT ( $, .STERADIAN. ) SOLID_ANGLE_UNIT ( ) );
#85290=CARTESIAN_POINT ( 'NONE',  ( 14.79681306129999996, 1434.437610817989935, 221.1969614931990122 ) ) ;
#85293=CARTESIAN_POINT ( 'NONE',  ( 1.657820374930000007, 1433.671037157990213, 203.5362873279890152 ) ) ;
#85294=ORIENTED_EDGE ( 'NONE', *, *, #15165, .F. ) ;
#85316=CARTESIAN_POINT ( 'NONE',  ( -4.175281431485900363, 1433.777855993409958, 217.7638082317450028 ) ) ;
#85319=CARTESIAN_POINT ( 'NONE',  ( -13.94448290884199970, 1508.551704408389924, 210.3470438395370081 ) ) ;
#85326=CARTESIAN_POINT ( 'NONE',  ( -3.292573594295789885, 1428.757065012120165, 200.3549139475240111 ) ) ;
#85333=ORIENTED_EDGE ( 'NONE', *, *, #79994, .F. ) ;
#85336=CARTESIAN_POINT ( 'NONE',  ( 10.67800209769209907, 1490.926871433870247, 211.7224831522450188 ) ) ;
#85340=CARTESIAN_POINT ( 'NONE',  ( -0.8597107444419990196, 1463.363299253190007, 202.2013017319989956 ) ) ;
#85349=CARTESIAN_POINT ( 'NONE',  ( -11.29483889965070098, 1508.440183434380060, 218.1662304949769862 ) ) ;
#85353=CARTESIAN_POINT ( 'NONE',  ( -13.41054182479114054, 1504.856770982285980, 208.9138911101860288 ) ) ;
#85355=CARTESIAN_POINT ( 'NONE',  ( 3.691669781079999879, 1467.622943078690014, 218.3869275675289998 ) ) ;
#85362=CARTESIAN_POINT ( 'NONE',  ( 11.55216494016860018, 1480.217685936279850, 211.4791692585090175 ) ) ;
#85367=CARTESIAN_POINT ( 'NONE',  ( 2.407076450357060082, 1456.389291684359932, 219.4682715861369786 ) ) ;
#85368=CARTESIAN_POINT ( 'NONE',  ( 11.40561765973709996, 1470.999254084470067, 209.2195126300399863 ) ) ;
#85371=CARTESIAN_POINT ( 'NONE',  ( 11.44311708750000101, 1501.817457268189855, 208.4257042509889857 ) ) ;
#85372=VECTOR ( 'NONE', #56183, 1000.000000000000114 ) ;
#85375=CARTESIAN_POINT ( 'NONE',  ( 7.236738478339999503, 1426.973880016789963, 212.3972659138590018 ) ) ;
#85376=CARTESIAN_POINT ( 'NONE',  ( -3.912776123225929936, 1515.493282983300105, 212.5868990599399808 ) ) ;
#85383=CARTESIAN_POINT ( 'NONE',  ( 1.711055448681089940E-31, 1424.874073124720098, 209.1218459616989946 ) ) ;
#85387=CARTESIAN_POINT ( 'NONE',  ( -4.313829138780000072, 1500.726371502089933, 230.0083276664990137 ) ) ;
#85388=CARTESIAN_POINT ( 'NONE',  ( -15.56794941087492390, 1415.969174529124075, 207.8815349042810112 ) ) ;
#85390=CARTESIAN_POINT ( 'NONE',  ( 1.111422967361669789, 1456.698882163199869, 219.6849870739549999 ) ) ;
#85395=CARTESIAN_POINT ( 'NONE',  ( 7.890413475299999924, 1422.993678601120109, 213.8680409669790095 ) ) ;
#85396=CARTESIAN_POINT ( 'NONE',  ( -2.515613294380000031, 1448.349718812090032, 188.5842421506989979 ) ) ;
#85401=ORIENTED_EDGE ( 'NONE', *, *, #110557, .T. ) ;
#85402=ORIENTED_EDGE ( 'NONE', *, *, #45616, .F. ) ;
#85405=CARTESIAN_POINT ( 'NONE',  ( 1.847634001515719993, 1478.089546411300262, 198.8590795898780073 ) ) ;
#85407=CARTESIAN_POINT ( 'NONE',  ( 9.407330927246226437, 1500.876264887889647, 202.6219334492917596 ) ) ;
#85421=EDGE_LOOP ( 'NONE', ( #89522, #29674, #1754, #96143, #95907 ) ) ;
#85424=CARTESIAN_POINT ( 'NONE',  ( 14.91143818900724405, 1416.177402202029953, 209.1063111766177940 ) ) ;
#85428=CARTESIAN_POINT ( 'NONE',  ( -10.50234776566190043, 1470.323106409019829, 212.1315068601290079 ) ) ;
#85449=CARTESIAN_POINT ( 'NONE',  ( 8.832258665910320161, 1437.105706114509985, 211.2299904616040180 ) ) ;
#85450=CARTESIAN_POINT ( 'NONE',  ( 5.702926893268910113, 1484.838078577319948, 214.7898773046569829 ) ) ;
#85458=CARTESIAN_POINT ( 'NONE',  ( -11.67167393029579969, 1491.623603738560178, 205.3077603581180028 ) ) ;
#85464=CARTESIAN_POINT ( 'NONE',  ( 4.617112521066619735, 1430.220117714789922, 217.4127892114239842 ) ) ;
#85465=CARTESIAN_POINT ( 'NONE',  ( 9.831195291770230327, 1461.796653735920017, 208.3421129756590062 ) ) ;
#85473=CARTESIAN_POINT ( 'NONE',  ( -16.72711410799999854, 1420.480869615339998, 203.4938400411990074 ) ) ;
#85475=CARTESIAN_POINT ( 'NONE',  ( 7.450245527241210475, 1489.014956828029881, 206.3621210875100189 ) ) ;
#85476=B_SPLINE_CURVE_WITH_KNOTS ( 'NONE', 5,
 ( #70262, #20352, #54556, #69137, #103240, #5217, #13041, #73546, #65140, #74093, #23103, #47778, #47230, #39371, #39924, #4670, #22532, #55649, #72445, #3598, #108222 ),
 .UNSPECIFIED., .F., .F.,
 ( 6, 3, 3, 3, 3, 3, 6 ),
 ( -12.02704502919999996, -11.38341475070000008, -10.53188235890000080, -9.802594204569999192, -8.789679567349999445, -5.488753621229999879, 1.776356839400250465E-15 ),
 .UNSPECIFIED. ) ;
#85477=CARTESIAN_POINT ( 'NONE',  ( -8.655671105859999770, 1512.830360918489987, 210.0583268009119990 ) ) ;
#85479=CARTESIAN_POINT ( 'NONE',  ( 0.9134330820525868866, 1423.706385267109908, 191.2040966441970227 ) ) ;
#85481=CARTESIAN_POINT ( 'NONE',  ( -4.462107437047291292, 1508.188283896733537, 220.5629211818961721 ) ) ;
#85483=CARTESIAN_POINT ( 'NONE',  ( -3.271538019026510202, 1454.292002138270163, 199.1638778078030043 ) ) ;
#85488=CARTESIAN_POINT ( 'NONE',  ( -4.727379727993030301, 1421.625110441430024, 193.4326326425589855 ) ) ;
#85494=CARTESIAN_POINT ( 'NONE',  ( -4.038582018749999669, 1515.598601288590089, 209.1218459616989946 ) ) ;
#85501=CARTESIAN_POINT ( 'NONE',  ( 2.855157077230529694, 1508.551704408389924, 219.4496006082999884 ) ) ;
#85508=CARTESIAN_POINT ( 'NONE',  ( 10.38805000968689995, 1451.723873411300019, 207.4476418283009878 ) ) ;
#85510=AXIS2_PLACEMENT_3D ( 'NONE', #20021, #81037, #3261 ) ;
#85513=CARTESIAN_POINT ( 'NONE',  ( 4.987078438843329131, 1508.551704408389924, 206.5718281456429963 ) ) ;
#85515=ORIENTED_EDGE ( 'NONE', *, *, #94927, .T. ) ;
#85522=CARTESIAN_POINT ( 'NONE',  ( 11.77118616850890120, 1479.407637630939917, 208.8749157105980032 ) ) ;
#85530=CARTESIAN_POINT ( 'NONE',  ( -9.205625138637591576, 1450.204495207709897, 208.8293812459489800 ) ) ;
#85531=CARTESIAN_POINT ( 'NONE',  ( -14.53343879676760153, 1421.577982565850107, 203.5955589198449900 ) ) ;
#85534=ORIENTED_EDGE ( 'NONE', *, *, #75423, .T. ) ;
#85535=CARTESIAN_POINT ( 'NONE',  ( 4.694859187580000537, 1472.563992416889960, 187.6273510758990142 ) ) ;
#85541=CARTESIAN_POINT ( 'NONE',  ( 10.41177329615350011, 1460.024665156439823, 205.9063136364349873 ) ) ;
#85545=CARTESIAN_POINT ( 'NONE',  ( -1.993348244980000183, 1477.149067790089930, 198.9137608980990137 ) ) ;
#85557=CARTESIAN_POINT ( 'NONE',  ( 7.367553984658170130, 1426.317790364889788, 212.6468799033240202 ) ) ;
#85561=CARTESIAN_POINT ( 'NONE',  ( -11.18131722815940066, 1491.896203582180078, 207.0175328158499610 ) ) ;
#85565=CARTESIAN_POINT ( 'NONE',  ( 8.413970532630001387, 1428.089005924990033, 212.8939830477889927 ) ) ;
#85566=CARTESIAN_POINT ( 'NONE',  ( -3.852420766530000318, 1461.443526049990169, 228.3501068971989980 ) ) ;
#85571=DIRECTION ( 'NONE',  ( -1.305148739725796033E-31, 1.000000000000000000, -1.836970198721029688E-16 ) ) ;
#85586=CARTESIAN_POINT ( 'NONE',  ( -4.979428188690000034, 1427.783661369190213, 201.1078272686790172 ) ) ;
#85593=CARTESIAN_POINT ( 'NONE',  ( 4.544860949943270612, 1508.551704410290085, 205.1599016910289777 ) ) ;
#85597=CARTESIAN_POINT ( 'NONE',  ( 7.854071199910000800, 1421.721864916329878, 195.9105866898989916 ) ) ;
#85599=CARTESIAN_POINT ( 'NONE',  ( -3.589794993429999970, 1496.402118238189814, 198.3466359645990167 ) ) ;
#85610=B_SPLINE_CURVE_WITH_KNOTS ( 'NONE', 5,
 ( #102506, #25796, #59995, #94673, #43185, #77337, #34768, #80078, #72794 ),
 .UNSPECIFIED., .F., .F.,
 ( 6, 3, 6 ),
 ( 234.3510616479999840, 237.3878297990000021, 239.1631355520000000 ),
 .UNSPECIFIED. ) ;
#85615=CARTESIAN_POINT ( 'NONE',  ( 9.936711670530231189, 1422.499099451789789, 212.2361507557569951 ) ) ;
#85618=CARTESIAN_POINT ( 'NONE',  ( -10.97606361528359997, 1462.640992382440118, 207.8491965332009954 ) ) ;
#85624=CARTESIAN_POINT ( 'NONE',  ( -9.850099335591719907, 1461.427211915769931, 209.3139255674489903 ) ) ;
#85626=CARTESIAN_POINT ( 'NONE',  ( 18.29793613913720307, 1429.923626251509859, 201.0778461450230168 ) ) ;
#85627=CARTESIAN_POINT ( 'NONE',  ( 11.99876342961469966, 1425.975962788000288, 199.1838357467620142 ) ) ;
#85628=CARTESIAN_POINT ( 'NONE',  ( 9.503369802446668402, 1463.703997095049999, 211.5558214296420090 ) ) ;
#85629=EDGE_CURVE ( 'NONE', #44333, #65430, #35122, .T. ) ;
#85639=CARTESIAN_POINT ( 'NONE',  ( 5.076283936602980162, 1469.790178403189884, 187.8425608794819937 ) ) ;
#85642=CARTESIAN_POINT ( 'NONE',  ( -16.44758872147649953, 1420.160613029469914, 207.7350616873459899 ) ) ;
#85644=CARTESIAN_POINT ( 'NONE',  ( 3.775107361939999961, 1441.398020315490157, 217.5130260360689931 ) ) ;
#85652=B_SPLINE_SURFACE_WITH_KNOTS ( 'NONE', 5, 5, ( 
 ( #85238, #94756, #33187, #58960, #76305, #60632 ),
 ( #76864, #50563, #42708, #175, #84689, #67378 ),
 ( #9636, #101476, #18033, #86353, #7988, #68478 ),
 ( #42154, #58412, #102579, #25877, #60077, #92538 ),
 ( #94193, #17463, #43810, #43265, #77412, #34847 ),
 ( #69036, #32648, #27555, #62869, #79635, #2392 ),
 ( #62294, #52771, #53903, #88038, #69592, #79085 ),
 ( #10199, #37612, #88580, #80165, #70704, #78519 ),
 ( #44938, #36510, #105935, #104816, #11322, #12401 ) ),
 .UNSPECIFIED., .F., .F., .F.,
 ( 6, 3, 6 ),
 ( 6, 6 ),
 ( -9.415047822849649119E-06, 2.934247638910000067, 4.839418697517819723 ),
 ( 0.000000000000000000, 1.000009415047820038 ),
 .UNSPECIFIED. ) ;
#85659=CARTESIAN_POINT ( 'NONE',  ( -6.958135218038119518, 1434.179671701880125, 214.2270546061249945 ) ) ;
#85667=CARTESIAN_POINT ( 'NONE',  ( 11.27279626876990015, 1426.317628015930040, 206.4670722515049874 ) ) ;
#85674=CARTESIAN_POINT ( 'NONE',  ( 4.889046445280000874, 1473.841289047790042, 218.9857726612289923 ) ) ;
#85680=CARTESIAN_POINT ( 'NONE',  ( -10.94209233289999972, 1492.979988313090189, 207.3926202980489961 ) ) ;
#85684=CARTESIAN_POINT ( 'NONE',  ( -1778.930368298719941, -2340.220200558880151, 9317.326275786501355 ) ) ;
#85685=CARTESIAN_POINT ( 'NONE',  ( 5.296871147660000112, 1447.430519322290138, 200.3058700119589730 ) ) ;
#85688=CARTESIAN_POINT ( 'NONE',  ( -2.124993027169999493, 1455.769608825389923, 199.7713323867489805 ) ) ;
#85695=CARTESIAN_POINT ( 'NONE',  ( -3.355411835910000029, 1495.471247818590200, 219.8040188672989927 ) ) ;
#85711=CARTESIAN_POINT ( 'NONE',  ( 3.096514233597529753, 1508.551704408389924, 214.0351581889520105 ) ) ;
#85715=CARTESIAN_POINT ( 'NONE',  ( 9.655324750296419012, 1461.352300578269933, 207.1780675101539941 ) ) ;
#85719=CARTESIAN_POINT ( 'NONE',  ( 8.916387934133441107, 1452.089085741889903, 211.7557271715180320 ) ) ;
#85720=CARTESIAN_POINT ( 'NONE',  ( -1.910237665331893986, 1487.499208352387313, 219.7920233817232543 ) ) ;
#85721=EDGE_CURVE ( 'NONE', #23359, #21788, #103690, .T. ) ;
#85723=CARTESIAN_POINT ( 'NONE',  ( -14.74124171903659963, 1508.249207875330058, 209.5562123098220013 ) ) ;
#85728=CARTESIAN_POINT ( 'NONE',  ( 10.48352362072680144, 1451.966107083780116, 207.9936217224200163 ) ) ;
#85729=CARTESIAN_POINT ( 'NONE',  ( -5.144873395449999443, 1502.885538352589947, 229.8910404859989853 ) ) ;
#85731=ORIENTED_EDGE ( 'NONE', *, *, #39288, .T. ) ;
#85742=CARTESIAN_POINT ( 'NONE',  ( -16.99050533527280038, 1420.323706995179919, 203.8408272025779979 ) ) ;
#85743=CARTESIAN_POINT ( 'NONE',  ( -3.378218165227587555, 1488.703315969531104, 219.4764361902140877 ) ) ;
#85746=EDGE_CURVE ( 'NONE', #50492, #86906, #105150, .T. ) ;
#85747=CARTESIAN_POINT ( 'NONE',  ( 10.58168742575649901, 1469.969853788360069, 207.1021894818239844 ) ) ;
#85749=CARTESIAN_POINT ( 'NONE',  ( 6.225972109890000716, 1494.795958560490135, 219.7811165620990153 ) ) ;
#85753=CARTESIAN_POINT ( 'NONE',  ( 4.601013853250220720, 1466.751833711500012, 199.0309000631700087 ) ) ;
#85754=B_SPLINE_CURVE_WITH_KNOTS ( 'NONE', 3,
 ( #103660, #61148, #55478, #38104, #14541, #71760, #90700, #21820, #20732, #38648, #13426, #73370, #64435, #5048, #65532, #3428, #63883, #82312, #89603, #107508, #30798, #5610, #72823, #12896, #97998, #90143, #39763, #47073, #97463, #106956, #29157, #106415, #99639, #81741, #91262, #54927, #47616 ),
 .UNSPECIFIED., .F., .F.,
 ( 4, 3, 3, 3, 3, 3, 3, 3, 3, 3, 3, 3, 4 ),
 ( -13.29188980189490010, -13.07961419483339860, -12.37600827227140066, -11.63118760886860059, -10.84675077014980005, -10.00729710514400139, -9.011581114248389923, -8.034184604791839490, -7.287185506055469553, -6.316933981596370096, -5.489728945046230102, -4.759576170441491172, -4.070471747090000036 ),
 .UNSPECIFIED. ) ;
#85756=CARTESIAN_POINT ( 'NONE',  ( -20.86258279118739978, 1504.682079557240058, 214.2158750867690173 ) ) ;
#85763=CARTESIAN_POINT ( 'NONE',  ( -14.29558945610000009, 1415.677402202029953, 213.3792774005289914 ) ) ;
#85764=CARTESIAN_POINT ( 'NONE',  ( -0.4393421190897080497, 1515.147356017569791, 204.7945591776110064 ) ) ;
#85765=ORIENTED_EDGE ( 'NONE', *, *, #107050, .T. ) ;
#85767=CARTESIAN_POINT ( 'NONE',  ( 0.000000000000000000, 1397.913060387289988, 209.1218459616989946 ) ) ;
#85771=CARTESIAN_POINT ( 'NONE',  ( -11.02705047837450181, 1462.270517538050171, 209.4579406216429902 ) ) ;
#85778=CARTESIAN_POINT ( 'NONE',  ( -9.845631732519999346, 1478.475703631090028, 212.8873760790889946 ) ) ;
#85792=CARTESIAN_POINT ( 'NONE',  ( -16.50171772879999921, 1417.502270639089829, 205.9476994086790000 ) ) ;
#85795=CARTESIAN_POINT ( 'NONE',  ( -4.413317922511070357, 1485.124240097989968, 198.0652374695790172 ) ) ;
#85796=CARTESIAN_POINT ( 'NONE',  ( -8.629049563562299241, 1437.597470000089970, 208.3922918523649912 ) ) ;
#85812=B_SPLINE_SURFACE_WITH_KNOTS ( 'NONE', 5, 1, ( 
 ( #45897, #87901 ),
 ( #28527, #11727 ),
 ( #19560, #54307 ),
 ( #12818, #21743 ),
 ( #38565, #44796 ),
 ( #55396, #78949 ),
 ( #20115, #96283 ),
 ( #98474, #79493 ),
 ( #71682, #106333 ) ),
 .UNSPECIFIED., .F., .F., .F.,
 ( 6, 3, 6 ),
 ( 2, 2 ),
 ( 0.000000000000000000, 3.905343215419999847, 7.794752761919999884 ),
 ( 0.000000000000000000, 14.00000000000000000 ),
 .UNSPECIFIED. ) ;
#85813=CARTESIAN_POINT ( 'NONE',  ( -6.184151071931365706, 1496.325375897394451, 199.7106397341868274 ) ) ;
#85820=CARTESIAN_POINT ( 'NONE',  ( 10.46985159624440165, 1480.586287654560010, 207.8944363599310066 ) ) ;
#85823=CARTESIAN_POINT ( 'NONE',  ( -19.86654541609999924, 1443.778853391489974, 213.2156533979290032 ) ) ;
#85824=CARTESIAN_POINT ( 'NONE',  ( -4.038582018736554424, 1515.598601288560985, 209.4326227434377472 ) ) ;
#85825=CARTESIAN_POINT ( 'NONE',  ( -4.705736654693100540, 1479.984769896650278, 230.9466533013020069 ) ) ;
#85832=CARTESIAN_POINT ( 'NONE',  ( -11.12609309039999950, 1491.160357135190225, 209.7795743302380060 ) ) ;
#85833=CARTESIAN_POINT ( 'NONE',  ( 9.406850844429460068, 1450.347115270439872, 204.6358555677470008 ) ) ;
#85838=CARTESIAN_POINT ( 'NONE',  ( 4.208240993269999564, 1434.939300248989866, 227.0651965576989824 ) ) ;
#85848=ORIENTED_EDGE ( 'NONE', *, *, #27154, .F. ) ;
#85850=CARTESIAN_POINT ( 'NONE',  ( -10.36562125464200079, 1447.972358732529983, 209.1898071262730241 ) ) ;
#85851=CARTESIAN_POINT ( 'NONE',  ( 3.586360116007059506, 1515.071395204220153, 205.0390662864990077 ) ) ;
#85863=ORIENTED_EDGE ( 'NONE', *, *, #93216, .F. ) ;
#85870=CARTESIAN_POINT ( 'NONE',  ( -12.20493911282916422, 1503.566106373808225, 208.5052164380747115 ) ) ;
#85890=CARTESIAN_POINT ( 'NONE',  ( -13.82318464736509966, 1508.551704408389924, 210.3452327715689876 ) ) ;
#85893=DIRECTION ( 'NONE',  ( 1.000000000000000000, 2.249639673992789970E-32, 1.224646799147350002E-16 ) ) ;
#85895=CARTESIAN_POINT ( 'NONE',  ( -2.569297563752009683, 1429.158925392049923, 200.1088665598680052 ) ) ;
#85906=EDGE_CURVE ( 'NONE', #56028, #73491, #57195, .T. ) ;
#85916=CARTESIAN_POINT ( 'NONE',  ( -10.36432893639859998, 1448.249851073609989, 208.5380077942650132 ) ) ;
#85918=EDGE_LOOP ( 'NONE', ( #88727, #36257, #110534, #76906 ) ) ;
#85920=CARTESIAN_POINT ( 'NONE',  ( -12.99645283652920114, 1508.444770402639961, 217.1333260180389857 ) ) ;
#85923=EDGE_CURVE ( 'NONE', #53131, #51303, #10342, .T. ) ;
#85925=CARTESIAN_POINT ( 'NONE',  ( -8.099005836065213515, 1461.719615227744953, 203.7568343392296129 ) ) ;
#85927=CARTESIAN_POINT ( 'NONE',  ( 2.016490277786251450, 1468.747382109811042, 218.9369546187164417 ) ) ;
#85933=CARTESIAN_POINT ( 'NONE',  ( 10.77478558037159928, 1480.716566089449998, 211.2105078800119884 ) ) ;
#85934=CARTESIAN_POINT ( 'NONE',  ( 4.836622313100200188, 1506.975876971950129, 219.7632233975940323 ) ) ;
#85935=DIRECTION ( 'NONE',  ( 1.000000000000000000, 2.249639673992789970E-32, 1.224646799147350002E-16 ) ) ;
#85943=B_SPLINE_CURVE_WITH_KNOTS ( 'NONE', 5,
 ( #37741, #12538, #65157, #80847, #99271, #72461 ),
 .UNSPECIFIED., .F., .F.,
 ( 6, 6 ),
 ( -41.05058650750000027, -28.72930409989999845 ),
 .UNSPECIFIED. ) ;
#85944=CARTESIAN_POINT ( 'NONE',  ( 11.54017902740000068, 1501.914511391590167, 210.4796054250789723 ) ) ;
#85952=CARTESIAN_POINT ( 'NONE',  ( -7.844819027749999840, 1484.029266062490024, 200.6142659637689860 ) ) ;
#85961=CARTESIAN_POINT ( 'NONE',  ( -0.2280590849522179941, 1435.891982273890108, 227.5921632324569828 ) ) ;
#85962=CARTESIAN_POINT ( 'NONE',  ( -14.93183294469202949, 1416.109101684369762, 205.2149106319410237 ) ) ;
#85964=CARTESIAN_POINT ( 'NONE',  ( -9.788466504199840656, 1438.420938493939957, 210.7573931614269895 ) ) ;
#85968=CARTESIAN_POINT ( 'NONE',  ( -19.86464710129999744, 1441.435714617490021, 212.6459466283089910 ) ) ;
#85972=CARTESIAN_POINT ( 'NONE',  ( 5.920481487290000011, 1454.372615866290062, 216.6343245259689922 ) ) ;
#85974=ORIENTED_EDGE ( 'NONE', *, *, #68866, .F. ) ;
#85982=CARTESIAN_POINT ( 'NONE',  ( 1.810149460082830064, 1476.164246713959983, 197.7790825785519928 ) ) ;
#86000=ORIENTED_EDGE ( 'NONE', *, *, #59785, .T. ) ;
#86010=AXIS2_PLACEMENT_3D ( 'NONE', #23794, #92119, #94308 ) ;
#86013=VERTEX_POINT ( 'NONE', #58972 ) ;
#86025=FACE_OUTER_BOUND ( 'NONE', #33928, .T. ) ;
#86032=CARTESIAN_POINT ( 'NONE',  ( -10.30791481292679990, 1492.690696011769887, 202.4224590082119732 ) ) ;
#86033=VERTEX_POINT ( 'NONE', #84700 ) ;
#86035=EDGE_CURVE ( 'NONE', #81793, #21520, #50022, .T. ) ;
#86039=CARTESIAN_POINT ( 'NONE',  ( 3.629223372069999787, 1485.493217076989822, 199.0019188288989938 ) ) ;
#86040=CARTESIAN_POINT ( 'NONE',  ( 3.084333964535199701, 1430.771674455919992, 218.0971261273060122 ) ) ;
#86050=VECTOR ( 'NONE', #99509, 1000.000000000000000 ) ;
#86056=CARTESIAN_POINT ( 'NONE',  ( 5.128935729357530171, 1424.665416358850052, 191.8839303524709976 ) ) ;
#86058=CARTESIAN_POINT ( 'NONE',  ( -2.188078410709979771, 1508.020976590390092, 220.9453026643990086 ) ) ;
#86061=CARTESIAN_POINT ( 'NONE',  ( -6.628886050447888145, 1457.835213357252087, 215.9907006640574423 ) ) ;
#86065=CARTESIAN_POINT ( 'NONE',  ( -14.20525606923979822, 1416.383994347770113, 203.1489080140429735 ) ) ;
#86068=CARTESIAN_POINT ( 'NONE',  ( -7.649964371800000329, 1508.551704408389924, 219.0282674226889981 ) ) ;
#86076=CARTESIAN_POINT ( 'NONE',  ( -4.038581993089999322, 1515.598601291389969, 208.7452962358790103 ) ) ;
#86083=CARTESIAN_POINT ( 'NONE',  ( 10.45300839642550095, 1451.886422029280084, 207.8125584717180061 ) ) ;
#86090=CARTESIAN_POINT ( 'NONE',  ( -7.756928808066270165, 1508.430203411700177, 219.4938965895260026 ) ) ;
#86095=CARTESIAN_POINT ( 'NONE',  ( 8.743403136036231871, 1436.332529221019968, 208.7150008048009795 ) ) ;
#86101=CARTESIAN_POINT ( 'NONE',  ( 3.535327672168380175, 1487.160996015089950, 197.6951163816430039 ) ) ;
#86103=CARTESIAN_POINT ( 'NONE',  ( 9.005225986101351054, 1434.097730569279975, 205.2808843445390039 ) ) ;
#86104=CARTESIAN_POINT ( 'NONE',  ( -11.82672180567140074, 1422.987463746610047, 204.1159878212820047 ) ) ;
#86107=EDGE_LOOP ( 'NONE', ( #105234, #60881, #85167, #96337 ) ) ;
#86108=CARTESIAN_POINT ( 'NONE',  ( -12.92111071619999940, 1506.047764528690095, 209.0897718066489688 ) ) ;
#86109=CARTESIAN_POINT ( 'NONE',  ( -3.219437420819999840, 1471.841586492590068, 187.3725962029989773 ) ) ;
#86117=CARTESIAN_POINT ( 'NONE',  ( -11.77719994004817039, 1507.564759764977225, 208.2431318170986572 ) ) ;
#86124=CARTESIAN_POINT ( 'NONE',  ( -7.990476243889999886, 1424.874074065990271, 210.4763446083090059 ) ) ;
#86129=CARTESIAN_POINT ( 'NONE',  ( 7.326032238172809130, 1426.385876809990123, 212.7391182884030059 ) ) ;
#86138=CARTESIAN_POINT ( 'NONE',  ( -0.3143867530260010534, 1455.265365023490176, 215.8131651789690011 ) ) ;
#86144=LINE ( 'NONE', #42481, #37558 ) ;
#86152=B_SPLINE_CURVE_WITH_KNOTS ( 'NONE', 3,
 ( #90810, #82425, #31451, #74030, #108162, #97032, #88635, #46090, #4081, #71869, #105986, #55040, #93550, #75680, #50484, #91910, #40957, #108717, #6797, #57790, #101384, #67292, #15187, #76222, #16281, #101949, #66197, #25236, #110365, #32008, #42617, #49375, #14653, #59440 ),
 .UNSPECIFIED., .F., .F.,
 ( 4, 3, 3, 3, 3, 3, 3, 3, 3, 3, 3, 4 ),
 ( -7.942685506149999242, -7.854675769405689678, -7.548843613729729896, -7.215342110406210097, -6.846990903797389727, -6.377391753856749723, -5.953803517216489816, -5.599849543008009967, -5.359340702741580031, -4.827138227139039728, -4.194202119578910093, -3.257013150989999772 ),
 .UNSPECIFIED. ) ;
#86164=ORIENTED_EDGE ( 'NONE', *, *, #105580, .F. ) ;
#86165=CARTESIAN_POINT ( 'NONE',  ( 3.744311016462700259, 1509.032041868229953, 204.8808983862890045 ) ) ;
#86167=CARTESIAN_POINT ( 'NONE',  ( -3.053241897311849584, 1508.551704408389924, 214.0456212180230011 ) ) ;
#86169=CARTESIAN_POINT ( 'NONE',  ( 7.526678075229999543, 1423.047586979970220, 195.6744525590990236 ) ) ;
#86183=CARTESIAN_POINT ( 'NONE',  ( -6.504448388238199819, 1484.623890501229880, 199.1483530729989866 ) ) ;
#86185=CARTESIAN_POINT ( 'NONE',  ( 12.67629937430701936, 1426.478869958664063, 202.7079000866955028 ) ) ;
#86192=CARTESIAN_POINT ( 'NONE',  ( -17.59937028154769934, 1418.719235195160081, 207.0514148608630194 ) ) ;
#86193=CARTESIAN_POINT ( 'NONE',  ( -1.842962214296178569, 1515.219201590507282, 213.4472514034267761 ) ) ;
#86203=CARTESIAN_POINT ( 'NONE',  ( -16.53114555299940136, 1465.611457094120169, 220.7423133389369809 ) ) ;
#86205=CARTESIAN_POINT ( 'NONE',  ( -20.36885094410000008, 1418.422628033280034, 210.1555047974290176 ) ) ;
#86206=CARTESIAN_POINT ( 'NONE',  ( 9.008848419482919923, 1451.404950095520007, 211.2754342882610104 ) ) ;
#86207=CARTESIAN_POINT ( 'NONE',  ( 3.711571330249999967, 1441.008188660590122, 218.3178908880789777 ) ) ;
#86208=VERTEX_POINT ( 'NONE', #59529 ) ;
#86213=CARTESIAN_POINT ( 'NONE',  ( -8.627785716502410551, 1437.492545073600013, 228.3379458911339839 ) ) ;
#86217=CARTESIAN_POINT ( 'NONE',  ( 6.326340444085493786, 1446.650791557884077, 202.6322225399144372 ) ) ;
#86234=CARTESIAN_POINT ( 'NONE',  ( 5.145309177750649887, 1422.426130283250131, 194.5914460530619863 ) ) ;
#86236=CARTESIAN_POINT ( 'NONE',  ( -12.02051099930000078, 1491.153688734890011, 206.6632163140190244 ) ) ;
#86240=CARTESIAN_POINT ( 'NONE',  ( -7329.274061526074547, -2340.220200558883789, -10678.01295216180006 ) ) ;
#86248=CARTESIAN_POINT ( 'NONE',  ( -3.490463098060000213, 1496.905315118289991, 198.4270279902989955 ) ) ;
#86249=CARTESIAN_POINT ( 'NONE',  ( -2.215101663730000059, 1496.819187201989962, 221.3100143584990178 ) ) ;
#86267=EDGE_CURVE ( 'NONE', #86906, #41878, #75808, .T. ) ;
#86268=CARTESIAN_POINT ( 'NONE',  ( -4.995284487919999350, 1391.732982292789984, 214.7012254044889801 ) ) ;
#86272=CARTESIAN_POINT ( 'NONE',  ( 10.84791127679310030, 1460.615700148999849, 207.7176790179939871 ) ) ;
#86276=CARTESIAN_POINT ( 'NONE',  ( 9.296700322752400325, 1453.078792441659971, 212.1083447425310169 ) ) ;
#86277=FACE_OUTER_BOUND ( 'NONE', #106506, .T. ) ;
#86281=CARTESIAN_POINT ( 'NONE',  ( -9.418564982631906446, 1418.460837828868989, 196.9369629217839872 ) ) ;
#86282=VECTOR ( 'NONE', #23385, 1000.000000000000000 ) ;
#86286=CARTESIAN_POINT ( 'NONE',  ( 9.216280896211529239, 1450.783082650540109, 209.7718718314580144 ) ) ;
#86287=CARTESIAN_POINT ( 'NONE',  ( 6.063466849340000131, 1461.859068790690117, 206.6237464808990012 ) ) ;
#86298=CARTESIAN_POINT ( 'NONE',  ( -7.170583105241029820, 1508.384145562859885, 219.7141895747710123 ) ) ;
#86305=CARTESIAN_POINT ( 'NONE',  ( -12.72940262790820043, 1502.367719156869953, 210.1495042875829995 ) ) ;
#86309=CARTESIAN_POINT ( 'NONE',  ( 8.400941578297418388, 1424.507064994723351, 195.7368743825176125 ) ) ;
#86310=CARTESIAN_POINT ( 'NONE',  ( -4.171844745047410541, 1497.126029642969797, 198.6588305097009766 ) ) ;
#86319=CARTESIAN_POINT ( 'NONE',  ( -14.85992380390000100, 1416.181292664740113, 213.2198171372490094 ) ) ;
#86320=CARTESIAN_POINT ( 'NONE',  ( -0.1141777317403989966, 1515.158022524200078, 204.7948384897389928 ) ) ;
#86326=CARTESIAN_POINT ( 'NONE',  ( -10.98329405719170104, 1462.122223828419919, 210.0364276692640146 ) ) ;
#86331=CARTESIAN_POINT ( 'NONE',  ( -10.44853431733320015, 1480.978285847389998, 207.5981847469569743 ) ) ;
#86353=CARTESIAN_POINT ( 'NONE',  ( -11.43249851594280031, 1508.430448985320027, 208.4158283025909952 ) ) ;
#86358=EDGE_CURVE ( 'NONE', #8084, #52143, #76842, .T. ) ;
#86362=DIRECTION ( 'NONE',  ( -0.1528503721702839657, -0.4524026203659298195, -0.8786174553316397073 ) ) ;
#86371=CARTESIAN_POINT ( 'NONE',  ( 3.939553394270000286, 1484.542612446990006, 220.2950041541989776 ) ) ;
#86372=ADVANCED_FACE ( 'NONE', ( #24102 ), #102784, .F. ) ;
#86373=CARTESIAN_POINT ( 'NONE',  ( 11.30263822180440059, 1479.449500025850057, 208.3515620824809957 ) ) ;
#86375=CARTESIAN_POINT ( 'NONE',  ( 8.316512080489999903, 1462.697935791190048, 228.8554007396989789 ) ) ;
#86377=CARTESIAN_POINT ( 'NONE',  ( 18.46110511457829872, 1471.786120933839811, 195.2229451478879980 ) ) ;
#86381=CARTESIAN_POINT ( 'NONE',  ( 2.475018616569089946, 1497.111080321040163, 196.9667222483770104 ) ) ;
#86382=CARTESIAN_POINT ( 'NONE',  ( -14.77932465454309963, 1420.552195126709876, 212.5457007543760142 ) ) ;
#86383=CARTESIAN_POINT ( 'NONE',  ( 7.882146126611630166, 1449.075262138320113, 202.4510296736249870 ) ) ;
#86384=CARTESIAN_POINT ( 'NONE',  ( 10.78159844869479933, 1461.896569297480028, 211.1674770051990038 ) ) ;
#86398=CARTESIAN_POINT ( 'NONE',  ( -2.571036083430311869, 1463.062948214519793, 199.6378877115486148 ) ) ;
#86401=CARTESIAN_POINT ( 'NONE',  ( -4.832616806509495433, 1508.551704408389924, 211.6097810599876254 ) ) ;
#86411=CARTESIAN_POINT ( 'NONE',  ( -5.292247061280000331, 1391.913060387289988, 203.8075142969990168 ) ) ;
#86413=ORIENTED_EDGE ( 'NONE', *, *, #66461, .F. ) ;
#86415=CARTESIAN_POINT ( 'NONE',  ( -14.52721453695589915, 1441.419400887780057, 221.0377524652309944 ) ) ;
#86423=CARTESIAN_POINT ( 'NONE',  ( 10.49215165150000040, 1461.076717947590168, 208.4970850545110181 ) ) ;
#86427=FACE_OUTER_BOUND ( 'NONE', #13841, .T. ) ;
#86444=CYLINDRICAL_SURFACE ( 'NONE', #28436, 1.999999999999997335 ) ;
#86449=CARTESIAN_POINT ( 'NONE',  ( -2.518237780042220209, 1429.186867776430063, 200.0939789790910197 ) ) ;
#86453=CARTESIAN_POINT ( 'NONE',  ( -11.86162332674610020, 1482.094478540630007, 208.3237497903899964 ) ) ;
#86458=CARTESIAN_POINT ( 'NONE',  ( 10.46269364489999987, 1491.122602117189899, 212.5073291737689942 ) ) ;
#86464=CARTESIAN_POINT ( 'NONE',  ( -9.157365711123761187, 1450.019713085520152, 208.1727642848220228 ) ) ;
#86473=CARTESIAN_POINT ( 'NONE',  ( 4.760896992130000172, 1449.971761959190189, 190.6385172635989704 ) ) ;
#86477=CARTESIAN_POINT ( 'NONE',  ( -2.018623677739999955, 1430.846887013590049, 200.9911499127990169 ) ) ;
#86479=CARTESIAN_POINT ( 'NONE',  ( -1.049859350909999822, 1507.477610268389981, 221.1890539870990153 ) ) ;
#86480=( BOUNDED_CURVE ( )  B_SPLINE_CURVE ( 3, ( #95857, #96417, #4561, #64486 ),
 .UNSPECIFIED., .F., .T. ) 
 B_SPLINE_CURVE_WITH_KNOTS ( ( 4, 4 ),
 ( 0.9877503981440959313, 2.153842406702509926 ),
 .UNSPECIFIED. ) 
 CURVE ( )  GEOMETRIC_REPRESENTATION_ITEM ( )  RATIONAL_B_SPLINE_CURVE ( ( 1.000000000000000000, 0.8898596592221782453, 0.8898596592221782453, 1.000000000000000000 ) ) 
 REPRESENTATION_ITEM ( '' )  );
#86487=CARTESIAN_POINT ( 'NONE',  ( 0.2004702986640009843, 1484.367984788590093, 198.3959036849990127 ) ) ;
#86488=FACE_OUTER_BOUND ( 'NONE', #52024, .T. ) ;
#86490=CARTESIAN_POINT ( 'NONE',  ( 11.46077257159999974, 1502.847332571289826, 210.2224670152189958 ) ) ;
#86492=CARTESIAN_POINT ( 'NONE',  ( 8.778597385549998577, 1422.758389211139956, 213.4479247216190174 ) ) ;
#86496=CARTESIAN_POINT ( 'NONE',  ( -6.025150679499999384, 1484.743688571590155, 198.8560548609989951 ) ) ;
#86501=EDGE_CURVE ( 'NONE', #22363, #110093, #93028, .T. ) ;
#86506=CARTESIAN_POINT ( 'NONE',  ( 0.6226065275839990365, 1494.171460328590001, 217.4567746792189666 ) ) ;
#86507=CARTESIAN_POINT ( 'NONE',  ( -14.92639605204266928, 1416.110071989740163, 205.1965795451626775 ) ) ;
#86509=CARTESIAN_POINT ( 'NONE',  ( 0.6804202724532750768, 1456.809669822820069, 219.7230711736309843 ) ) ;
#86510=VECTOR ( 'NONE', #83254, 1000.000000000000114 ) ;
#86516=CARTESIAN_POINT ( 'NONE',  ( 7.630837923450000559, 1424.601304396760042, 212.1062089104590029 ) ) ;
#86517=CARTESIAN_POINT ( 'NONE',  ( -18.47518245119999847, 1466.235720591789914, 200.8822878489689856 ) ) ;
#86521=CARTESIAN_POINT ( 'NONE',  ( 5.355729600950000169, 1454.568469885690092, 217.0404969026290019 ) ) ;
#86522=EDGE_LOOP ( 'NONE', ( #46721, #22523, #1611, #61983, #108961 ) ) ;
#86527=CARTESIAN_POINT ( 'NONE',  ( 7.534083176413666649, 1500.276886300912111, 200.5709797116870163 ) ) ;
#86530=EDGE_CURVE ( 'NONE', #43306, #37624, #50423, .T. ) ;
#86531=CARTESIAN_POINT ( 'NONE',  ( 0.1665620115664219747, 1475.825097533989947, 197.6600777373799929 ) ) ;
#86537=ADVANCED_FACE ( 'NONE', ( #5400 ), #8875, .F. ) ;
#86542=ORIENTED_EDGE ( 'NONE', *, *, #56468, .F. ) ;
#86543=EDGE_LOOP ( 'NONE', ( #78180, #54883, #87256, #51204 ) ) ;
#86545=CARTESIAN_POINT ( 'NONE',  ( -4.523943953710000798, 1455.378620544990099, 200.8408221482090141 ) ) ;
#86558=CARTESIAN_POINT ( 'NONE',  ( 9.695068361086670805, 1462.695882120360011, 208.0360144262189976 ) ) ;
#86561=ORIENTED_EDGE ( 'NONE', *, *, #31314, .F. ) ;
#86572=CARTESIAN_POINT ( 'NONE',  ( 9.561971226590548767, 1436.616785344690015, 211.5587197113850095 ) ) ;
#86574=CARTESIAN_POINT ( 'NONE',  ( -5.221927606092449992, 1489.269388166920180, 185.8916506247110192 ) ) ;
#86579=CARTESIAN_POINT ( 'NONE',  ( 3.313501335607582643, 1397.551704408390151, 215.1871694724064810 ) ) ;
#86583=CARTESIAN_POINT ( 'NONE',  ( -3.531493108469999864, 1429.908133670090137, 201.5805818289689739 ) ) ;
#86585=B_SPLINE_SURFACE_WITH_KNOTS ( 'NONE', 5, 1, ( 
 ( #94152, #85756 ),
 ( #51074, #677 ),
 ( #18535, #134 ),
 ( #70108, #85201 ),
 ( #104221, #68995 ),
 ( #103096, #34255 ) ),
 .UNSPECIFIED., .F., .F., .F.,
 ( 6, 6 ),
 ( 2, 2 ),
 ( -3.220373955451920388E-05, 18.01490009493960187 ),
 ( 0.000000000000000000, 14.00003220373960033 ),
 .UNSPECIFIED. ) ;
#86589=CARTESIAN_POINT ( 'NONE',  ( 12.67630892740000093, 1426.478874823920023, 202.7079035067189920 ) ) ;
#86597=DIRECTION ( 'NONE',  ( -0.9996573249755517088, -0.02617694830808747070, 0.000000000000000000 ) ) ;
#86602=CARTESIAN_POINT ( 'NONE',  ( 2.973593887119999835, 1441.553271505090152, 218.1843342212790162 ) ) ;
#86607=CARTESIAN_POINT ( 'NONE',  ( -9.078760040516870689, 1459.398684262878078, 212.3905513612093046 ) ) ;
#86610=CARTESIAN_POINT ( 'NONE',  ( -13.87318377641789979, 1417.128397284559924, 202.3536462288429902 ) ) ;
#86617=CARTESIAN_POINT ( 'NONE',  ( 8.887359343084140662, 1425.078831941400040, 195.6980871684259853 ) ) ;
#86622=CARTESIAN_POINT ( 'NONE',  ( 2.586839709529719755, 1508.551704408389924, 219.5247725683019837 ) ) ;
#86628=DIRECTION ( 'NONE',  ( -1.699538841806929935E-33, 1.000000000000000000, -1.698192320643030073E-16 ) ) ;
#86641=CARTESIAN_POINT ( 'NONE',  ( 8.629414813098978954, 1437.378993763129984, 209.7946259206210016 ) ) ;
#86647=CIRCLE ( 'NONE', #100936, 0.4999999999999995559 ) ;
#86649=CARTESIAN_POINT ( 'NONE',  ( 7.785771676495370386, 1435.464459252629922, 205.4398922123320119 ) ) ;
#86653=ORIENTED_EDGE ( 'NONE', *, *, #1011, .T. ) ;
#86656=CARTESIAN_POINT ( 'NONE',  ( -13.40940820319999993, 1470.117754583789974, 192.0205833154989818 ) ) ;
#86670=VERTEX_POINT ( 'NONE', #23833 ) ;
#86671=CARTESIAN_POINT ( 'NONE',  ( -8.364654381539999406, 1423.448482863899926, 210.5916039729090130 ) ) ;
#86676=CARTESIAN_POINT ( 'NONE',  ( 7.539467915018410515, 1425.654756675969793, 212.1861668026819814 ) ) ;
#86678=CARTESIAN_POINT ( 'NONE',  ( -0.2833403650370509563, 1496.275355223149973, 221.4684270307890017 ) ) ;
#86684=CIRCLE ( 'NONE', #36656, 0.4999999999999996114 ) ;
#86685=( BOUNDED_CURVE ( )  B_SPLINE_CURVE ( 3, ( #97175, #79288, #36723, #20448 ),
 .UNSPECIFIED., .F., .T. ) 
 B_SPLINE_CURVE_WITH_KNOTS ( ( 4, 4 ),
 ( 4.149166158125050075, 5.275619312941369543 ),
 .UNSPECIFIED. ) 
 CURVE ( )  GEOMETRIC_REPRESENTATION_ITEM ( )  RATIONAL_B_SPLINE_CURVE ( ( 1.000000000000000000, 0.8970245268685778095, 0.8970245268685778095, 1.000000000000000000 ) ) 
 REPRESENTATION_ITEM ( '' )  );
#86687=CARTESIAN_POINT ( 'NONE',  ( -18.60629936281669927, 1508.494392593700013, 210.7647685123470183 ) ) ;
#86688=CARTESIAN_POINT ( 'NONE',  ( 4.780307568339999591, 1467.625956517089890, 217.8721402715589761 ) ) ;
#86689=CARTESIAN_POINT ( 'NONE',  ( -8.697277070075241312, 1440.006333808949876, 206.1599688172080107 ) ) ;
#86705=ORIENTED_EDGE ( 'NONE', *, *, #100921, .T. ) ;
#86712=CARTESIAN_POINT ( 'NONE',  ( 2.473110443770000000, 1437.362874199289763, 227.5249784694989899 ) ) ;
#86715=EDGE_LOOP ( 'NONE', ( #70256, #48645, #80854 ) ) ;
#86716=CARTESIAN_POINT ( 'NONE',  ( 4.058188250227919625, 1508.551704408389924, 204.4428604963009946 ) ) ;
#86729=CARTESIAN_POINT ( 'NONE',  ( -15.84432591830269743, 1419.853212859319910, 210.7451195136700051 ) ) ;
#86735=CARTESIAN_POINT ( 'NONE',  ( -12.68810582867495640, 1464.870331481658241, 224.6384026358888377 ) ) ;
#86739=CARTESIAN_POINT ( 'NONE',  ( 0.1794159432210164773, 1421.105753184904643, 193.7169311276417716 ) ) ;
#86740=CARTESIAN_POINT ( 'NONE',  ( -4.328907235665659492, 1515.085473475149911, 207.8086220615720094 ) ) ;
#86745=B_SPLINE_SURFACE_WITH_KNOTS ( 'NONE', 5, 5, ( 
 ( #74891, #109042, #57548, #75448, #91671, #14945 ),
 ( #109584, #67047, #7662, #83273, #101154, #6570 ),
 ( #32325, #66507, #58636, #92682, #83736, #75894 ),
 ( #14865, #32237, #58004, #47939, #57464, #74262 ),
 ( #108947, #24368, #49057, #49604, #23268, #91590 ),
 ( #40633, #83193, #41735, #91027, #93235, #6481 ),
 ( #73712, #23813, #65855, #32777, #92140, #110046 ),
 ( #22697, #107836, #65307, #7580, #74804, #33318 ),
 ( #7031, #100533, #58554, #5936, #67515, #15413 ) ),
 .UNSPECIFIED., .F., .F., .F.,
 ( 6, 3, 6 ),
 ( 6, 6 ),
 ( 2.948979317598059868, 5.061843608070000222, 7.174698196173030063 ),
 ( -0.0004176450428783939949, 2.000000000000000000 ),
 .UNSPECIFIED. ) ;
#86748=CARTESIAN_POINT ( 'NONE',  ( -17.25816047809999887, 1421.803897450879958, 201.8596040855890124 ) ) ;
#86760=CARTESIAN_POINT ( 'NONE',  ( 8.129468112789759004, 1461.711575812669935, 228.8738014183659857 ) ) ;
#86762=CARTESIAN_POINT ( 'NONE',  ( 9.178714075745430634, 1450.974408660679956, 210.2178452082900151 ) ) ;
#86763=CARTESIAN_POINT ( 'NONE',  ( 3.181164613930000051, 1442.605935617189971, 217.4126579123289957 ) ) ;
#86769=ORIENTED_EDGE ( 'NONE', *, *, #97876, .T. ) ;
#86770=CARTESIAN_POINT ( 'NONE',  ( -17.65533568451049717, 1419.497303018139974, 207.2321751882169849 ) ) ;
#86772=AXIS2_PLACEMENT_3D ( 'NONE', #51567, #75671, #85149 ) ;
#86777=CARTESIAN_POINT ( 'NONE',  ( -0.2632583344880010112, 1431.930419643889991, 218.6352234134390073 ) ) ;
#86785=CARTESIAN_POINT ( 'NONE',  ( 12.32884901062990046, 1491.954766579230181, 208.6881790030290063 ) ) ;
#86790=CARTESIAN_POINT ( 'NONE',  ( 6.052710029050000884, 1450.431596175490085, 208.9426997230080190 ) ) ;
#86792=CARTESIAN_POINT ( 'NONE',  ( -5.264764398929999700, 1496.215621365389779, 199.2138428350390029 ) ) ;
#86810=EDGE_CURVE ( 'NONE', #39044, #23842, #38297, .T. ) ;
#86811=DIRECTION ( 'NONE',  ( -1.000000000000000000, 0.000000000000000000, 0.000000000000000000 ) ) ;
#86823=CARTESIAN_POINT ( 'NONE',  ( 3.966481540897129232, 1508.551704408389924, 213.6259163359240176 ) ) ;
#86827=CARTESIAN_POINT ( 'NONE',  ( 9.808454316486640678, 1461.705508564400134, 208.1084590643120009 ) ) ;
#86829=VERTEX_POINT ( 'NONE', #76408 ) ;
#86830=VERTEX_POINT ( 'NONE', #59624 ) ;
#86831=CARTESIAN_POINT ( 'NONE',  ( 10.27958569201449990, 1453.357447123039947, 211.7732196989560123 ) ) ;
#86835=CARTESIAN_POINT ( 'NONE',  ( -10.15866205370000053, 1462.015553540890096, 208.6820378064900012 ) ) ;
#86840=CARTESIAN_POINT ( 'NONE',  ( 10.57398797330110085, 1452.565052662689823, 209.4913240895520232 ) ) ;
#86841=CARTESIAN_POINT ( 'NONE',  ( 4.329448776274299249, 1515.064792882709980, 211.4519800890089982 ) ) ;
#86850=CARTESIAN_POINT ( 'NONE',  ( -7.723857300294940664, 1508.513725859440001, 219.3188919284999940 ) ) ;
#86857=CARTESIAN_POINT ( 'NONE',  ( -12.61701280676319925, 1502.098792127180104, 210.9886739834400089 ) ) ;
#86858=CARTESIAN_POINT ( 'NONE',  ( 10.82744532179999908, 1493.119756917389850, 214.1919876165190146 ) ) ;
#86860=CARTESIAN_POINT ( 'NONE',  ( 8.931923137804934854, 1424.999313002464532, 195.6482533560690058 ) ) ;
#86862=CARTESIAN_POINT ( 'NONE',  ( 9.168936444336990732, 1468.675008117680136, 202.6297543281519893 ) ) ;
#86870=CARTESIAN_POINT ( 'NONE',  ( 3.920837378839999943, 1505.974547704289989, 220.4971537480990094 ) ) ;
#86872=CARTESIAN_POINT ( 'NONE',  ( -0.8972167985107359911, 1515.116734647830071, 204.7937573286989732 ) ) ;
#86877=CARTESIAN_POINT ( 'NONE',  ( 1.914156610164409855, 1431.087920293139859, 199.8421651263110164 ) ) ;
#86883=CARTESIAN_POINT ( 'NONE',  ( 17.69622264849999738, 1430.679833671289771, 213.5595385020990022 ) ) ;
#86887=CARTESIAN_POINT ( 'NONE',  ( 10.93677819324079969, 1460.929513094869890, 208.6200360033440120 ) ) ;
#86895=CARTESIAN_POINT ( 'NONE',  ( -11.25901873334290038, 1500.172003390719965, 210.8567363214919794 ) ) ;
#86896=CARTESIAN_POINT ( 'NONE',  ( 15.17118851365313681, 1478.360907884334210, 223.3047515974349153 ) ) ;
#86898=CARTESIAN_POINT ( 'NONE',  ( -16.79918157119999833, 1416.515139567399729, 209.6726229222840061 ) ) ;
#86905=CARTESIAN_POINT ( 'NONE',  ( 1.248319867352440049, 1432.832940376729994, 200.7627304351539976 ) ) ;
#86906=VERTEX_POINT ( 'NONE', #16471 ) ;
#86909=CARTESIAN_POINT ( 'NONE',  ( -4.885446997243459322, 1463.524418545851404, 200.4816647042127329 ) ) ;
#86921=CARTESIAN_POINT ( 'NONE',  ( 4.325805437739999704, 1515.203925700790023, 207.6585595670590010 ) ) ;
#86925=CARTESIAN_POINT ( 'NONE',  ( 3.499910042949999855, 1484.886116685890102, 220.0290872740989983 ) ) ;
#86926=CARTESIAN_POINT ( 'NONE',  ( 4.423690678889999894, 1423.173374607840060, 194.1945114146989795 ) ) ;
#86928=CARTESIAN_POINT ( 'NONE',  ( -2.809383017458359610, 1449.519851564760074, 188.5656358724000086 ) ) ;
#86930=CARTESIAN_POINT ( 'NONE',  ( 22.24401671484320175, 1475.958684028669950, 209.7631754067580232 ) ) ;
#86931=CARTESIAN_POINT ( 'NONE',  ( -16.82744758394869677, 1417.384158686259980, 208.0241611917670070 ) ) ;
#86934=LINE ( 'NONE', #84714, #75487 ) ;
#86935=CARTESIAN_POINT ( 'NONE',  ( -11.51646780219999933, 1489.881239353890123, 211.6099079467890078 ) ) ;
#86938=CARTESIAN_POINT ( 'NONE',  ( 10.01433557240000027, 1462.389869715989789, 210.8954298964690111 ) ) ;
#86946=ORIENTED_EDGE ( 'NONE', *, *, #9215, .F. ) ;
#86947=VERTEX_POINT ( 'NONE', #17013 ) ;
#86962=CARTESIAN_POINT ( 'NONE',  ( -7.446477803703490217, 1423.701825524609831, 209.9841580610070082 ) ) ;
#86966=CARTESIAN_POINT ( 'NONE',  ( 1.234341273178619858, 1432.827581395659990, 200.7608884223369898 ) ) ;
#86967=ORIENTED_EDGE ( 'NONE', *, *, #43589, .T. ) ;
#86968=VERTEX_POINT ( 'NONE', #42260 ) ;
#86973=CARTESIAN_POINT ( 'NONE',  ( -4.487357341475295414, 1509.034509733380446, 206.0057038257949671 ) ) ;
#86975=CARTESIAN_POINT ( 'NONE',  ( 9.765834982210000348, 1462.985811087089814, 208.7590207740749975 ) ) ;
#86977=CARTESIAN_POINT ( 'NONE',  ( 11.23571964750900065, 1422.131126052970103, 210.3743327618489900 ) ) ;
#86991=CARTESIAN_POINT ( 'NONE',  ( -0.6021969839118817003, 1455.373305037211594, 218.5407630597736954 ) ) ;
#86992=CARTESIAN_POINT ( 'NONE',  ( -4.869818399669999742, 1491.215867106689984, 188.8099941780989752 ) ) ;
#86994=CARTESIAN_POINT ( 'NONE',  ( -2.244413514000000109, 1507.820143033590057, 221.0491532391990006 ) ) ;
#87004=CARTESIAN_POINT ( 'NONE',  ( -11.77257222062089781, 1482.353834374220014, 207.3907860494599902 ) ) ;
#87014=DIRECTION ( 'NONE',  ( -0.9233374271748948647, -0.3766813615418239114, -0.07455969048382228570 ) ) ;
#87024=B_SPLINE_CURVE_WITH_KNOTS ( 'NONE', 3,
 ( #52432, #86558, #9854, #72951, #56696, #2036, #28317, #45140, #56139, #61950, #98686, #47742, #53539, #79835, #36169, #107644 ),
 .UNSPECIFIED., .F., .F.,
 ( 4, 3, 3, 3, 3, 4 ),
 ( -7.359819276019999634, -7.224550556550780378, -6.183163466960579946, -5.141872062630270079, -4.100202402597499685, -3.013663444789999701 ),
 .UNSPECIFIED. ) ;
#87028=CARTESIAN_POINT ( 'NONE',  ( 20.49831092009999978, 1496.178973653789853, 204.1013708937389879 ) ) ;
#87029=CARTESIAN_POINT ( 'NONE',  ( -0.7326187029203401480, 1469.562181525167944, 219.1516452693006727 ) ) ;
#87031=CARTESIAN_POINT ( 'NONE',  ( -15.46337563405010052, 1415.677402202039957, 209.5778891453549875 ) ) ;
#87034=CARTESIAN_POINT ( 'NONE',  ( 0.2136919556920010010, 1431.040275962890064, 200.3703063552589754 ) ) ;
#87035=EDGE_CURVE ( 'NONE', #18362, #22689, #10307, .T. ) ;
#87038=CARTESIAN_POINT ( 'NONE',  ( 1.888458389810000027, 1506.668004227690062, 221.0469516508989898 ) ) ;
#87043=CARTESIAN_POINT ( 'NONE',  ( 3.511586131400000088, 1485.920068215290030, 198.9399327136989655 ) ) ;
#87044=CARTESIAN_POINT ( 'NONE',  ( 3.350799455140170302, 1464.627286088550136, 199.8699596448449824 ) ) ;
#87046=CARTESIAN_POINT ( 'NONE',  ( 12.70729947579999930, 1500.570810271889968, 209.2766994282530106 ) ) ;
#87048=CARTESIAN_POINT ( 'NONE',  ( 7.987775376090000101, 1423.444922220860008, 212.4896135368290118 ) ) ;
#87052=CARTESIAN_POINT ( 'NONE',  ( -9.749017428870001112, 1483.358875000189983, 202.9209122778790118 ) ) ;
#87061=CARTESIAN_POINT ( 'NONE',  ( -11.34479132750911390, 1501.899302646182832, 207.4495276564311155 ) ) ;
#87064=CARTESIAN_POINT ( 'NONE',  ( -3.470364637360000337, 1448.107370639490000, 190.4136600830990176 ) ) ;
#87066=CARTESIAN_POINT ( 'NONE',  ( -1.780593273166600099, 1457.520619209220058, 219.6239990789049727 ) ) ;
#87070=CARTESIAN_POINT ( 'NONE',  ( -8.723783498850000484, 1451.961142758290180, 205.5456223906990090 ) ) ;
#87072=CARTESIAN_POINT ( 'NONE',  ( 7.892648486029999688, 1424.312437875390060, 211.9575832887890101 ) ) ;
#87074=CARTESIAN_POINT ( 'NONE',  ( -16.83568192250000095, 1418.884533543920043, 201.2565368162689765 ) ) ;
#87075=CARTESIAN_POINT ( 'NONE',  ( -21.12854635009999882, 1507.715432716589703, 209.4790063781609888 ) ) ;
#87077=ADVANCED_FACE ( 'NONE', ( #94171 ), #106304, .T. ) ;
#87085=CARTESIAN_POINT ( 'NONE',  ( 2.744925583754461940, 1499.105962719451554, 198.1014308731936069 ) ) ;
#87088=CARTESIAN_POINT ( 'NONE',  ( -1.841894009802319987, 1475.332893174979972, 197.8298818394579826 ) ) ;
#87100=CARTESIAN_POINT ( 'NONE',  ( -3.637379841050000007, 1454.260016440290201, 199.7007646786289854 ) ) ;
#87120=CARTESIAN_POINT ( 'NONE',  ( 3.074703527060000052, 1441.333178254290033, 218.5515148082390056 ) ) ;
#87122=CARTESIAN_POINT ( 'NONE',  ( -9.157150010547340457, 1440.811674898089223, 204.9830327270436499 ) ) ;
#87123=CARTESIAN_POINT ( 'NONE',  ( -14.47420009890000081, 1416.181292664740113, 214.4142689833190047 ) ) ;
#87137=ORIENTED_EDGE ( 'NONE', *, *, #22433, .F. ) ;
#87140=CARTESIAN_POINT ( 'NONE',  ( -2.451814761660000119, 1429.700538131990015, 200.7967561671190140 ) ) ;
#87145=ADVANCED_FACE ( 'NONE', ( #82193 ), #109928, .T. ) ;
#87147=CARTESIAN_POINT ( 'NONE',  ( 11.48577098159999998, 1425.717070342639772, 202.9081124425690064 ) ) ;
#87158=ADVANCED_FACE ( 'NONE', ( #95019 ), #41992, .T. ) ;
#87159=CARTESIAN_POINT ( 'NONE',  ( -17.21060100480000088, 1507.583332828389985, 209.3895586510680005 ) ) ;
#87161=CARTESIAN_POINT ( 'NONE',  ( 3.023734050500000325, 1442.695058689789903, 217.4756557394289871 ) ) ;
#87175=CARTESIAN_POINT ( 'NONE',  ( -4.492641941105690151, 1508.880976867409800, 212.2392493694379993 ) ) ;
#87179=CARTESIAN_POINT ( 'NONE',  ( -4.528990542849999024, 1484.552700007790008, 198.9721756806989958 ) ) ;
#87180=CARTESIAN_POINT ( 'NONE',  ( -10.48842657476610185, 1479.773419084050147, 209.6713063323329891 ) ) ;
#87183=EDGE_CURVE ( 'NONE', #21410, #33283, #84883, .T. ) ;
#87184=CARTESIAN_POINT ( 'NONE',  ( -10.05468035857399833, 1491.062548945049912, 213.6251199428619714 ) ) ;
#87190=CARTESIAN_POINT ( 'NONE',  ( 10.56624192506330040, 1452.381986011830122, 209.0163554798489827 ) ) ;
#87203=CARTESIAN_POINT ( 'NONE',  ( -3.951796886255740215, 1495.396716508259942, 197.4422882964240102 ) ) ;
#87207=CARTESIAN_POINT ( 'NONE',  ( -9.828024340748898524, 1446.801136768030119, 212.2328356403849909 ) ) ;
#87212=CARTESIAN_POINT ( 'NONE',  ( -8.977835948444159442, 1424.635420156040027, 204.7825922023490079 ) ) ;
#87216=ORIENTED_EDGE ( 'NONE', *, *, #88299, .F. ) ;
#87217=CARTESIAN_POINT ( 'NONE',  ( -3.865424752135750097, 1508.610338626970133, 213.5325984595829993 ) ) ;
#87218=CARTESIAN_POINT ( 'NONE',  ( 18.37994959805489970, 1472.972861928199791, 195.0276218624729836 ) ) ;
#87237=CIRCLE ( 'NONE', #55130, 0.9999999999998898659 ) ;
#87240=FACE_OUTER_BOUND ( 'NONE', #90122, .T. ) ;
#87245=CARTESIAN_POINT ( 'NONE',  ( 7.069913306463050162, 1426.666554464499995, 213.2414280066960259 ) ) ;
#87247=CARTESIAN_POINT ( 'NONE',  ( 6.824562263029999798, 1471.929136523390071, 216.7044338043689891 ) ) ;
#87248=CARTESIAN_POINT ( 'NONE',  ( -8.611006801263458854, 1438.354984712640089, 207.9016507195429995 ) ) ;
#87256=ORIENTED_EDGE ( 'NONE', *, *, #102475, .F. ) ;
#87259=CARTESIAN_POINT ( 'NONE',  ( -20.06562366400000030, 1485.934169092390221, 214.0282076738189971 ) ) ;
#87260=CIRCLE ( 'NONE', #62269, 0.9999999999999971134 ) ;
#87261=CARTESIAN_POINT ( 'NONE',  ( 19.18645890815103883, 1474.831003437985828, 202.6579824388850568 ) ) ;
#87269=CARTESIAN_POINT ( 'NONE',  ( -3.806848320439999878, 1438.700957657089930, 227.3446634402990014 ) ) ;
#87271=B_SPLINE_CURVE_WITH_KNOTS ( 'NONE', 3,
 ( #79543, #47587, #96890, #11772, #21236, #88487 ),
 .UNSPECIFIED., .F., .F.,
 ( 4, 2, 4 ),
 ( 0.000000000000000000, 0.5000000000000000000, 1.000000000000000000 ),
 .UNSPECIFIED. ) ;
#87278=CARTESIAN_POINT ( 'NONE',  ( -4.329448776040000446, 1515.064792882589927, 209.0973262533439936 ) ) ;
#87282=CARTESIAN_POINT ( 'NONE',  ( -3.829620113920000346, 1515.551704408389924, 206.7917118429090237 ) ) ;
#87290=VERTEX_POINT ( 'NONE', #70402 ) ;
#87295=VECTOR ( 'NONE', #30623, 1000.000000000000000 ) ;
#87297=CARTESIAN_POINT ( 'NONE',  ( 0.5152534324233022378, 1421.192241663663026, 193.7244559836547353 ) ) ;
#87298=CARTESIAN_POINT ( 'NONE',  ( -10.69735147599770109, 1462.941248850579996, 206.3316273933290006 ) ) ;
#87305=CARTESIAN_POINT ( 'NONE',  ( -10.03542548471770068, 1461.476867323560100, 210.6072180941889940 ) ) ;
#87306=CARTESIAN_POINT ( 'NONE',  ( -14.58152186650000104, 1423.117512814019847, 196.4410428726990006 ) ) ;
#87315=CARTESIAN_POINT ( 'NONE',  ( -16.38987313889203534, 1420.134888794942754, 208.8825633451824331 ) ) ;
#87318=( BOUNDED_CURVE ( )  B_SPLINE_CURVE ( 3, ( #76289, #110439, #25858, #67911 ),
 .UNSPECIFIED., .F., .T. ) 
 B_SPLINE_CURVE_WITH_KNOTS ( ( 4, 4 ),
 ( 1.009533648558965879, 2.132059403723200131 ),
 .UNSPECIFIED. ) 
 CURVE ( )  GEOMETRIC_REPRESENTATION_ITEM ( )  RATIONAL_B_SPLINE_CURVE ( ( 1.000000000000000000, 0.8977224082826531504, 0.8977224082826531504, 1.000000000000000000 ) ) 
 REPRESENTATION_ITEM ( '' )  );
#87323=CARTESIAN_POINT ( 'NONE',  ( 3.916630911069999943, 1442.176737572990078, 217.0733355794490080 ) ) ;
#87329=VERTEX_POINT ( 'NONE', #22686 ) ;
#87330=CARTESIAN_POINT ( 'NONE',  ( -6.473263611634259895, 1508.551704408380147, 219.3223280905850174 ) ) ;
#87335=CARTESIAN_POINT ( 'NONE',  ( 7.066689964004210012, 1470.190416163020245, 190.3198042189900150 ) ) ;
#87336=CARTESIAN_POINT ( 'NONE',  ( -14.96589995520845129, 1420.088422609285089, 212.9477210871714874 ) ) ;
#87337=CARTESIAN_POINT ( 'NONE',  ( -10.78537409608540010, 1471.596790556679935, 206.8701440394590065 ) ) ;
#87345=CARTESIAN_POINT ( 'NONE',  ( 12.03443371747400015, 1491.353303888329947, 206.6665118833500117 ) ) ;
#87346=CARTESIAN_POINT ( 'NONE',  ( -2.210067589258040144, 1438.358026146749808, 227.5735626261489983 ) ) ;
#87351=CARTESIAN_POINT ( 'NONE',  ( -18.43163825505950015, 1441.474363498949970, 212.3696370042599995 ) ) ;
#87370=CARTESIAN_POINT ( 'NONE',  ( -1.029855757680000039, 1496.295066548290151, 221.0588599254990072 ) ) ;
#87383=CARTESIAN_POINT ( 'NONE',  ( -0.9775750227080020061, 1486.139233187990158, 221.0121526945989672 ) ) ;
#87387=ORIENTED_EDGE ( 'NONE', *, *, #26492, .F. ) ;
#87389=CARTESIAN_POINT ( 'NONE',  ( 10.47311736184310149, 1460.984455949540006, 208.2454930404500146 ) ) ;
#87390=CARTESIAN_POINT ( 'NONE',  ( 1.842962231260000028, 1515.064792882589927, 204.7923971856590128 ) ) ;
#87391=ORIENTED_EDGE ( 'NONE', *, *, #77426, .F. ) ;
#87393=CARTESIAN_POINT ( 'NONE',  ( 10.21177956804319997, 1453.436188331060066, 212.0248552912580067 ) ) ;
#87394=CARTESIAN_POINT ( 'NONE',  ( 7.276655529890000196, 1423.040021778160053, 195.5065388737989736 ) ) ;
#87395=ORIENTED_EDGE ( 'NONE', *, *, #42858, .T. ) ;
#87402=CARTESIAN_POINT ( 'NONE',  ( 9.235753568799740520, 1451.320621426679963, 209.8280334265319880 ) ) ;
#87408=ORIENTED_EDGE ( 'NONE', *, *, #68595, .F. ) ;
#87415=CARTESIAN_POINT ( 'NONE',  ( -9.185273275535660531, 1469.775230892159925, 215.0640531001920124 ) ) ;
#87419=CARTESIAN_POINT ( 'NONE',  ( -5.693467891879999243, 1475.871200527190013, 200.4602000259690158 ) ) ;
#87420=CARTESIAN_POINT ( 'NONE',  ( 10.21325682510000021, 1491.315150049489830, 213.3055097826090218 ) ) ;
#87422=CARTESIAN_POINT ( 'NONE',  ( 9.651063919191019025, 1425.440657924460083, 195.4941620015079877 ) ) ;
#87423=CARTESIAN_POINT ( 'NONE',  ( -16.27918300179999989, 1504.249498869590070, 208.8571777317940246 ) ) ;
#87425=CARTESIAN_POINT ( 'NONE',  ( 11.07149624271129973, 1422.788788392120068, 206.9676479960040183 ) ) ;
#87426=CARTESIAN_POINT ( 'NONE',  ( -9.942063362116220659, 1439.630728003020067, 208.0683743633950087 ) ) ;
#87432=B_SPLINE_SURFACE_WITH_KNOTS ( 'NONE', 5, 5, ( 
 ( #58026, #92161, #15434, #25487, #15981, #42873 ),
 ( #24926, #26034, #110066, #77576, #7056, #85395 ),
 ( #75914, #51262, #8143, #41212, #42309, #884 ),
 ( #109521, #8692, #66438, #32797, #66981, #24391 ),
 ( #336, #7601, #58576, #34463, #92704, #76463 ),
 ( #60228, #17625, #59678, #50182, #41755, #102739 ),
 ( #33342, #67537, #101637, #59136, #93790, #45100 ),
 ( #70311, #52936, #1418, #62462, #88736, #69188 ),
 ( #27171, #37228, #52393, #86516, #88186, #63025 ),
 ( #11478, #78114, #60797, #79793, #104424, #87072 ),
 ( #26601, #2548, #10358, #78675, #80334, #20399 ),
 ( #94923, #18742, #70866, #79240, #12019, #3098 ),
 ( #18196, #71424, #9809, #105540, #54059, #53493 ),
 ( #35558, #45654, #19293, #69753, #97130, #28827 ),
 ( #54604, #103871, #46200, #27717, #35007, #103294 ),
 ( #36673, #43975, #61356, #95475, #44530, #104978 ),
 ( #1992, #96584, #61904, #36127, #96021, #87638 ),
 ( #10924, #28268, #19856, #65194, #98771, #97675 ),
 ( #57359, #99860, #37780, #99306, #91483, #12571 ),
 ( #106081, #22033, #14208, #21489, #72490, #82537 ),
 ( #13638, #47827, #74148, #65742, #5267, #29905 ),
 ( #3651, #38311, #106619, #90922, #63560, #64098 ),
 ( #48394, #98219, #56784, #5832, #14762, #23157 ),
 ( #71969, #22580, #73599, #4178, #55701, #46751 ),
 ( #39422, #29359, #108279, #31014, #107729, #31566 ),
 ( #39973, #48950, #20947, #55153, #89274, #80882 ),
 ( #89822, #13094, #47278, #81961, #81401, #4713 ) ),
 .UNSPECIFIED., .F., .F., .F.,
 ( 6, 3, 3, 3, 3, 3, 3, 3, 6 ),
 ( 6, 6 ),
 ( 0.000000000000000000, 1.995983313780000046, 2.887652819479999966, 3.183319327139999988, 3.726393308010000016, 4.077147875629999696, 4.748093181249999795, 5.511025199249999673, 7.372157449769999538 ),
 ( 0.000000000000000000, 2.000000000000000000 ),
 .UNSPECIFIED. ) ;
#87434=B_SPLINE_CURVE_WITH_KNOTS ( 'NONE', 5,
 ( #21569, #98294, #30542, #39502, #72037, #73676, #106153, #29432, #28342 ),
 .UNSPECIFIED., .F., .F.,
 ( 6, 3, 6 ),
 ( 462.9758374870000353, 468.8934854820000169, 473.4384810120000111 ),
 .UNSPECIFIED. ) ;
#87437=CARTESIAN_POINT ( 'NONE',  ( -1.351910739713730214, 1515.082829241050149, 204.7928694849069871 ) ) ;
#87439=CARTESIAN_POINT ( 'NONE',  ( -15.88445676962039599, 1415.959459656937725, 209.7365985937010180 ) ) ;
#87442=CARTESIAN_POINT ( 'NONE',  ( -1.040347359575360064, 1429.922094406420001, 199.7824833409709981 ) ) ;
#87446=B_SPLINE_CURVE_WITH_KNOTS ( 'NONE', 3,
 ( #3007, #69101, #20311, #27085, #95385, #52299, #87546, #70227, #54514, #78584, #786, #35471, #103784, #69661, #1331, #97048, #36037, #34916, #104332, #88651, #10836, #26508, #79150, #53969, #94827, #53397, #103203, #27625, #96487, #71329, #61270, #11389, #18649, #88102, #60703, #105442, #11928 ),
 .UNSPECIFIED., .F., .F.,
 ( 4, 3, 3, 3, 3, 3, 3, 3, 3, 3, 3, 3, 4 ),
 ( -12.92009077346300039, -12.71598438484270055, -12.02692291841409933, -11.29816837385320127, -10.53156648978099952, -9.713214318400439140, -8.755060695329159870, -7.805279224055939657, -7.050688516310069431, -6.129046816252760266, -5.323559768139629611, -4.615615438122199876, -3.948767879309999174 ),
 .UNSPECIFIED. ) ;
#87450=CARTESIAN_POINT ( 'NONE',  ( 9.934261248579540293, 1469.591094200070074, 210.6863934935470013 ) ) ;
#87459=B_SPLINE_CURVE_WITH_KNOTS ( 'NONE', 5,
 ( #2237, #64334, #88417, #28509, #62710, #53751 ),
 .UNSPECIFIED., .F., .F.,
 ( 6, 6 ),
 ( 0.000000000000000000, 1.000000000000000000 ),
 .UNSPECIFIED. ) ;
#87461=EDGE_CURVE ( 'NONE', #19417, #55990, #76987, .T. ) ;
#87465=CARTESIAN_POINT ( 'NONE',  ( -15.46123378547330063, 1418.179543175669778, 203.0721989172009785 ) ) ;
#87468=CARTESIAN_POINT ( 'NONE',  ( -15.89311463129999780, 1416.118927280270100, 209.3720684979659836 ) ) ;
#87482=VECTOR ( 'NONE', #27331, 1000.000000000000114 ) ;
#87496=CARTESIAN_POINT ( 'NONE',  ( 3.256084378020000170, 1422.858183810449873, 193.8949459527989916 ) ) ;
#87498=CARTESIAN_POINT ( 'NONE',  ( -4.250000000000000000, 1516.051704408390151, 209.1218459616989946 ) ) ;
#87499=CARTESIAN_POINT ( 'NONE',  ( -3.103172482810000243, 1450.690062953990036, 188.5470283436989973 ) ) ;
#87503=CARTESIAN_POINT ( 'NONE',  ( -5.277971523409999755, 1391.913060387289988, 203.7647467602490110 ) ) ;
#87505=CARTESIAN_POINT ( 'NONE',  ( -14.87341339970349985, 1420.535920296580116, 212.2959427910559782 ) ) ;
#87513=AXIS2_PLACEMENT_3D ( 'NONE', #84563, #109773, #586 ) ;
#87516=ORIENTED_EDGE ( 'NONE', *, *, #86530, .T. ) ;
#87522=CARTESIAN_POINT ( 'NONE',  ( 11.01589229730000064, 1501.204512814589862, 206.0337867319090037 ) ) ;
#87526=CIRCLE ( 'NONE', #82140, 0.9999999999999971134 ) ;
#87538=CARTESIAN_POINT ( 'NONE',  ( 0.3848239385950819602, 1432.484357106330208, 200.6930806709059993 ) ) ;
#87546=CARTESIAN_POINT ( 'NONE',  ( -1.498494647347079933, 1465.094162369539845, 198.2212222711209790 ) ) ;
#87552=CARTESIAN_POINT ( 'NONE',  ( 8.583222999044879842, 1437.099971295089972, 208.1373760821520307 ) ) ;
#87557=CARTESIAN_POINT ( 'NONE',  ( 11.60117971636739931, 1478.974074431269855, 207.2346898377800244 ) ) ;
#87562=FACE_OUTER_BOUND ( 'NONE', #53209, .T. ) ;
#87564=CARTESIAN_POINT ( 'NONE',  ( 2.193121967036330222, 1423.464081223100038, 192.6388440160779965 ) ) ;
#87566=CARTESIAN_POINT ( 'NONE',  ( -803.2235323108749299, 1451.575432553050177, 209.0911897361090155 ) ) ;
#87568=CARTESIAN_POINT ( 'NONE',  ( -7.756964262599999493, 1508.430205954690109, 219.4938836478990254 ) ) ;
#87571=AXIS2_PLACEMENT_3D ( 'NONE', #72773, #59157, #39141 ) ;
#87581=EDGE_LOOP ( 'NONE', ( #57409, #33332, #106662, #16425 ) ) ;
#87585=CARTESIAN_POINT ( 'NONE',  ( 6.644648847156787497, 1485.119973938482872, 217.5961942112708982 ) ) ;
#87592=CARTESIAN_POINT ( 'NONE',  ( -8.621728156553459144, 1448.683718559020008, 212.1725994164930000 ) ) ;
#87607=CARTESIAN_POINT ( 'NONE',  ( -1.204685347530000117, 1506.953552699789952, 221.9093730674989899 ) ) ;
#87612=CARTESIAN_POINT ( 'NONE',  ( 2.067823311539999764, 1486.525342903789806, 197.7722860763989843 ) ) ;
#87613=CARTESIAN_POINT ( 'NONE',  ( 10.56485853567840039, 1469.565006426170157, 204.9063131257589987 ) ) ;
#87621=CARTESIAN_POINT ( 'NONE',  ( -9.968894432999999111, 1482.167632919289872, 205.0619827550790149 ) ) ;
#87628=CARTESIAN_POINT ( 'NONE',  ( -11.33396083898640860, 1502.204733694695051, 207.2924597943140270 ) ) ;
#87630=CARTESIAN_POINT ( 'NONE',  ( 3.827053565004849833, 1515.145425758850251, 209.1218459614979963 ) ) ;
#87632=CARTESIAN_POINT ( 'NONE',  ( -9.952950791904509487, 1438.984619552230015, 209.5724956438699849 ) ) ;
#87638=CARTESIAN_POINT ( 'NONE',  ( 7.998636686930000295, 1425.977676336709919, 211.5360327896089814 ) ) ;
#87644=CARTESIAN_POINT ( 'NONE',  ( 6.455724313810000226, 1455.041435863090101, 217.0620835976089893 ) ) ;
#87650=CARTESIAN_POINT ( 'NONE',  ( 2.317667528355622508, 1499.011937117496473, 198.0143009028709855 ) ) ;
#87662=CARTESIAN_POINT ( 'NONE',  ( 3.711571330249999967, 1441.008188660590122, 218.3178908880789777 ) ) ;
#87665=EDGE_LOOP ( 'NONE', ( #107226, #3420, #65771, #45158 ) ) ;
#87666=CARTESIAN_POINT ( 'NONE',  ( -4.222077225850000559, 1454.203573669889920, 200.3246332114389929 ) ) ;
#87670=B_SPLINE_CURVE_WITH_KNOTS ( 'NONE', 5,
 ( #37023, #79057, #54413, #97486, #2361, #55499, #12914, #104787, #47094 ),
 .UNSPECIFIED., .F., .F.,
 ( 6, 3, 6 ),
 ( 0.000000000000000000, 0.6258773692719435955, 1.000000000000000000 ),
 .UNSPECIFIED. ) ;
#87672=CARTESIAN_POINT ( 'NONE',  ( 8.309621275030000476, 1427.613389394789920, 212.3081093229889973 ) ) ;
#87674=ADVANCED_FACE ( 'NONE', ( #78084 ), #61759, .T. ) ;
#87690=CARTESIAN_POINT ( 'NONE',  ( 4.408349274510000804, 1512.051704408390151, 206.7128113371389873 ) ) ;
#87701=CARTESIAN_POINT ( 'NONE',  ( 13.52265959860729971, 1497.923474612530072, 227.8730153353740207 ) ) ;
#87719=AXIS2_PLACEMENT_3D ( 'NONE', #11878, #45507, #104280 ) ;
#87721=CARTESIAN_POINT ( 'NONE',  ( 6.825131319317435441, 1424.845011660433101, 213.4895702506433963 ) ) ;
#87723=CARTESIAN_POINT ( 'NONE',  ( 11.31530712674089934, 1470.580251583589870, 207.8288594857730232 ) ) ;
#87724=ORIENTED_EDGE ( 'NONE', *, *, #37865, .T. ) ;
#87726=LINE ( 'NONE', #54135, #80271 ) ;
#87732=CARTESIAN_POINT ( 'NONE',  ( 2.936686034740000117, 1441.572633673089967, 218.1969960917990079 ) ) ;
#87740=CARTESIAN_POINT ( 'NONE',  ( 4.414384251610000476, 1487.467097172089780, 197.9737507085990273 ) ) ;
#87741=CARTESIAN_POINT ( 'NONE',  ( 4.329448781177520189, 1515.064792686469900, 207.2788827064790098 ) ) ;
#87743=EDGE_LOOP ( 'NONE', ( #32031, #57679, #72201 ) ) ;
#87753=CARTESIAN_POINT ( 'NONE',  ( -10.61843432092680040, 1489.244268642379893, 214.1625968120690118 ) ) ;
#87754=CARTESIAN_POINT ( 'NONE',  ( 24.11200011979999758, 1496.633574749990203, 206.8275458132090137 ) ) ;
#87765=VERTEX_POINT ( 'NONE', #32644 ) ;
#87774=EDGE_CURVE ( 'NONE', #37552, #109438, #90249, .T. ) ;
#87775=CARTESIAN_POINT ( 'NONE',  ( -3.160255966859999877, 1481.778611285589932, 229.3886674967989734 ) ) ;
#87778=EDGE_CURVE ( 'NONE', #83093, #777, #99553, .T. ) ;
#87782=CARTESIAN_POINT ( 'NONE',  ( -16.06071031163280338, 1420.824417172319954, 203.3393085456370102 ) ) ;
#87785=ORIENTED_EDGE ( 'NONE', *, *, #40371, .F. ) ;
#87787=CARTESIAN_POINT ( 'NONE',  ( -5.440472735201729471, 1490.455374013109804, 185.8786135604090362 ) ) ;
#87798=CARTESIAN_POINT ( 'NONE',  ( -10.76610287370000130, 1461.751116408590178, 211.3389343564790011 ) ) ;
#87807=CARTESIAN_POINT ( 'NONE',  ( -9.472336532046449875, 1447.006353964749906, 212.1615584954940061 ) ) ;
#87810=CARTESIAN_POINT ( 'NONE',  ( 2.188321237025089960, 1495.686656333250085, 221.2656737636790183 ) ) ;
#87813=CARTESIAN_POINT ( 'NONE',  ( 3.628818056492709943, 1505.602008419380127, 221.3635114792730292 ) ) ;
#87815=EDGE_CURVE ( 'NONE', #41237, #15707, #28787, .T. ) ;
#87818=CARTESIAN_POINT ( 'NONE',  ( -18.37965383104189954, 1508.494210133719889, 211.1516869488499992 ) ) ;
#87819=CARTESIAN_POINT ( 'NONE',  ( 6.246736226000000336, 1472.130509067990033, 217.1982816640689862 ) ) ;
#87820=CARTESIAN_POINT ( 'NONE',  ( -8.792731325493480909, 1438.786328558429886, 208.0437710220710130 ) ) ;
#87825=CARTESIAN_POINT ( 'NONE',  ( 8.530885801226901322, 1436.944794269080148, 207.7948910702020271 ) ) ;
#87834=EDGE_CURVE ( 'NONE', #41116, #87329, #839, .T. ) ;
#87863=CARTESIAN_POINT ( 'NONE',  ( -9.751878866779549071, 1483.635755006349882, 202.2899340601439917 ) ) ;
#87865=B_SPLINE_CURVE_WITH_KNOTS ( 'NONE', 3,
 ( #16951, #51709, #86398, #58454 ),
 .UNSPECIFIED., .F., .F.,
 ( 4, 4 ),
 ( 0.000000000000000000, 1.000000000000000000 ),
 .UNSPECIFIED. ) ;
#87874=CARTESIAN_POINT ( 'NONE',  ( 14.27741977803430196, 1427.979761714439974, 195.2518213606840050 ) ) ;
#87877=CARTESIAN_POINT ( 'NONE',  ( 10.12814239611219946, 1462.553068569410243, 212.1302522725090114 ) ) ;
#87883=CARTESIAN_POINT ( 'NONE',  ( -15.86366695747779332, 1420.273692602325809, 209.9455591108094836 ) ) ;
#87886=CARTESIAN_POINT ( 'NONE',  ( -4.556906648196700438, 1508.729448895619953, 205.9844575237659967 ) ) ;
#87888=CARTESIAN_POINT ( 'NONE',  ( -234.5897387251999930, 11221.53578756869865, 2175.945776423289772 ) ) ;
#87890=CARTESIAN_POINT ( 'NONE',  ( 17.76546875260000036, 1430.865606781589804, 204.9340536459789917 ) ) ;
#87891=VERTEX_POINT ( 'NONE', #14591 ) ;
#87897=CARTESIAN_POINT ( 'NONE',  ( -2.525895663881050357, 1508.551704408389924, 220.0390078997519936 ) ) ;
#87900=CARTESIAN_POINT ( 'NONE',  ( 1.514120561980000183E-16, 1515.551704408389924, 209.1218459616989946 ) ) ;
#87901=CARTESIAN_POINT ( 'NONE',  ( 5.151097723079999469, 1490.744826430290004, 188.9005472705989916 ) ) ;
#87905=CARTESIAN_POINT ( 'NONE',  ( 0.4974867301289990218, 1430.722264131989959, 217.6047022486590095 ) ) ;
#87906=CARTESIAN_POINT ( 'NONE',  ( 1.842963673760084298, 1515.499673569527658, 213.2081603882464265 ) ) ;
#87908=CARTESIAN_POINT ( 'NONE',  ( 4.617353517619999792, 1460.098150474590057, 228.0971968620989969 ) ) ;
#87914=CARTESIAN_POINT ( 'NONE',  ( 11.13873845943729890, 1491.363418941899909, 209.7176399918620007 ) ) ;
#87920=CARTESIAN_POINT ( 'NONE',  ( 0.5070043562000440263, 1496.683860206890131, 196.7605787459179965 ) ) ;
#87933=CARTESIAN_POINT ( 'NONE',  ( 0.6649116665570009577, 1498.634995304990071, 197.7885086964990080 ) ) ;
#87954=EDGE_LOOP ( 'NONE', ( #9777, #13724, #70764, #95719 ) ) ;
#87956=CARTESIAN_POINT ( 'NONE',  ( 6.112774900040000681, 1424.453475662199935, 193.6149460215989961 ) ) ;
#87961=CARTESIAN_POINT ( 'NONE',  ( -1.920602012799999869, 1420.567466289690174, 193.8392733480989989 ) ) ;
#87977=CARTESIAN_POINT ( 'NONE',  ( 0.7957076353827553516, 1507.773683909243118, 220.9213704339180993 ) ) ;
#87978=CARTESIAN_POINT ( 'NONE',  ( -7.056546027978409796, 1508.551704406279896, 219.2861282186669882 ) ) ;
#87980=CARTESIAN_POINT ( 'NONE',  ( -10.75669312256790100, 1470.034964047250014, 212.8110033683189783 ) ) ;
#87984=CARTESIAN_POINT ( 'NONE',  ( -4.912635829359999207, 1474.545048648290049, 199.2507989359390024 ) ) ;
#87985=CARTESIAN_POINT ( 'NONE',  ( -2.316872680442880306, 1421.992067379949958, 193.2449569725669960 ) ) ;
#87988=CARTESIAN_POINT ( 'NONE',  ( -15.05518181500000097, 1503.464336090389907, 209.0350305184400099 ) ) ;
#87990=CARTESIAN_POINT ( 'NONE',  ( 11.12319339834159848, 1422.705095784430114, 206.9939503724160090 ) ) ;
#88000=CARTESIAN_POINT ( 'NONE',  ( 3.529344918850000123, 1506.116810151690061, 220.6266479957990043 ) ) ;
#88001=( BOUNDED_SURFACE ( )  B_SPLINE_SURFACE ( 1, 2, ( 
 ( #85132, #76195, #42591, #33614, #59967, #52110, #24649, #60516, #93528 ),
 ( #94639, #86240, #16797, #102479, #25768, #109798, #85684, #1161, #35291 ) ),
 .UNSPECIFIED., .F., .T., .F. ) 
 B_SPLINE_SURFACE_WITH_KNOTS ( ( 2, 2 ),
 ( 3, 2, 2, 2, 3 ),
 ( -10000.00000000000000, 10000.00000000000000 ),
 ( 0.000000000000000000, 1.570796326794899889, 3.141592653589790007, 4.712388980384689674, 6.283185307179590673 ),
 .UNSPECIFIED. ) 
 GEOMETRIC_REPRESENTATION_ITEM ( )  RATIONAL_B_SPLINE_SURFACE ( (
 ( 1.000000000000000000, 0.7071067811865480168, 1.000000000000000000, 0.7071067811865480168, 1.000000000000000000, 0.7071067811865480168, 1.000000000000000000, 0.7071067811865480168, 1.000000000000000000),
 ( 1.000000000000000000, 0.7071067811865480168, 1.000000000000000000, 0.7071067811865480168, 1.000000000000000000, 0.7071067811865480168, 1.000000000000000000, 0.7071067811865480168, 1.000000000000000000) ) ) 
 REPRESENTATION_ITEM ( '' )  SURFACE ( )  );
#88002=EDGE_CURVE ( 'NONE', #74404, #53058, #30155, .T. ) ;
#88003=CARTESIAN_POINT ( 'NONE',  ( -15.46337283059999912, 1415.677402202029953, 209.5778880887239950 ) ) ;
#88005=CARTESIAN_POINT ( 'NONE',  ( -1.771280571366619982, 1515.064792319160006, 204.7923971709010118 ) ) ;
#88007=CARTESIAN_POINT ( 'NONE',  ( -15.92986207429999901, 1416.139014782290133, 209.7537124246929920 ) ) ;
#88010=CARTESIAN_POINT ( 'NONE',  ( -1.484755140834890019, 1429.714486269279860, 199.8512846474560263 ) ) ;
#88016=CARTESIAN_POINT ( 'NONE',  ( -8.895549977471178593, 1462.225664532283872, 227.1186910807994934 ) ) ;
#88026=CARTESIAN_POINT ( 'NONE',  ( -15.39825232982659919, 1418.148438324100198, 203.0909429379779851 ) ) ;
#88029=CARTESIAN_POINT ( 'NONE',  ( -15.89396736049999959, 1416.225531559500041, 209.0250895600429999 ) ) ;
#88037=CARTESIAN_POINT ( 'NONE',  ( -18.80299996640602700, 1468.065468973505176, 202.3792621952166257 ) ) ;
#88038=CARTESIAN_POINT ( 'NONE',  ( -13.03265074581759997, 1508.448609993070022, 209.7186198884500072 ) ) ;
#88059=CARTESIAN_POINT ( 'NONE',  ( 0.8763902003015829889, 1462.562412067790092, 230.5019338175040104 ) ) ;
#88063=CARTESIAN_POINT ( 'NONE',  ( -4.995284477430000258, 1391.732982068790079, 203.5424665078789985 ) ) ;
#88065=CARTESIAN_POINT ( 'NONE',  ( -10.47439550540000042, 1490.889281562089991, 212.4388770995890070 ) ) ;
#88067=CARTESIAN_POINT ( 'NONE',  ( 9.677596299730000240, 1463.237928047889909, 210.5383460088689844 ) ) ;
#88072=CARTESIAN_POINT ( 'NONE',  ( 12.21456615412630065, 1501.625727090829969, 212.8586461374000010 ) ) ;
#88073=CARTESIAN_POINT ( 'NONE',  ( -10.88610090654533913, 1422.259895732163159, 210.6369494421302875 ) ) ;
#88085=CARTESIAN_POINT ( 'NONE',  ( -1.921751667499999927, 1468.480854157690146, 219.3342396420989928 ) ) ;
#88090=CARTESIAN_POINT ( 'NONE',  ( -9.997338218269998578, 1422.621669173350028, 210.6353445619989770 ) ) ;
#88092=ORIENTED_EDGE ( 'NONE', *, *, #96519, .T. ) ;
#88093=CARTESIAN_POINT ( 'NONE',  ( 14.43085696089999992, 1426.807557149800004, 195.4949581795989957 ) ) ;
#88094=FACE_OUTER_BOUND ( 'NONE', #9096, .T. ) ;
#88102=CARTESIAN_POINT ( 'NONE',  ( 2.902893324140370268, 1466.180773484049951, 198.4663733987970033 ) ) ;
#88103=CARTESIAN_POINT ( 'NONE',  ( -18.86884385042500156, 1508.513763835350119, 210.1416286062879806 ) ) ;
#88112=CARTESIAN_POINT ( 'NONE',  ( 11.35705511386439959, 1478.717693206790045, 206.1553733900099985 ) ) ;
#88115=EDGE_CURVE ( 'NONE', #50172, #70893, #4268, .T. ) ;
#88124=CARTESIAN_POINT ( 'NONE',  ( -5.690400742829999636, 1508.048825776489821, 220.5583476148989917 ) ) ;
#88126=CARTESIAN_POINT ( 'NONE',  ( 18.30025784240000064, 1431.961054190390087, 210.0255047360110154 ) ) ;
#88128=DIRECTION ( 'NONE',  ( 0.8832694794843597430, 0.3761007072180699295, -0.2799701495543689411 ) ) ;
#88139=CARTESIAN_POINT ( 'NONE',  ( -5.169271338600384347, 1487.151140008964830, 220.0115120792558798 ) ) ;
#88140=CARTESIAN_POINT ( 'NONE',  ( -15.66247007830000015, 1415.943430100450087, 208.3724989932889855 ) ) ;
#88145=CARTESIAN_POINT ( 'NONE',  ( -9.881594800496241504, 1448.777576682979770, 207.8817744914870218 ) ) ;
#88150=CARTESIAN_POINT ( 'NONE',  ( -1.093792492990000031, 1515.225200552689785, 213.4470939808389858 ) ) ;
#88160=CARTESIAN_POINT ( 'NONE',  ( 2.484221813290000025, 1505.974367507990110, 221.6747987149990138 ) ) ;
#88164=CARTESIAN_POINT ( 'NONE',  ( 3.082592223099999806, 1485.754465970690035, 198.7996944297989899 ) ) ;
#88165=CARTESIAN_POINT ( 'NONE',  ( 10.48885285482030127, 1469.765830575109931, 206.0548704900310213 ) ) ;
#88186=CARTESIAN_POINT ( 'NONE',  ( 7.751138421380000310, 1424.420707150859926, 212.0424422646189839 ) ) ;
#88214=ORIENTED_EDGE ( 'NONE', *, *, #32949, .T. ) ;
#88215=CARTESIAN_POINT ( 'NONE',  ( -3.497772968360000512, 1454.175141309589890, 199.2405839609089924 ) ) ;
#88219=B_SPLINE_SURFACE_WITH_KNOTS ( 'NONE', 5, 5, ( 
 ( #101493, #82524, #50578, #109926, #108817, #100417 ),
 ( #23699, #57884, #83604, #6902, #39960, #41057 ),
 ( #15823, #109386, #32663, #100950, #50028, #7459 ),
 ( #41621, #102055, #33205, #59533, #67395, #24781 ),
 ( #84706, #8005, #76323, #110473, #51682, #16927 ),
 ( #9657, #18052, #1282, #69610, #43829, #8553 ),
 ( #9119, #85820, #76883, #733, #27031, #104837 ),
 ( #53351, #193, #94774, #35423, #86373, #104285 ),
 ( #60093, #68495, #70174, #103730, #61220, #95882 ) ),
 .UNSPECIFIED., .F., .F., .F.,
 ( 6, 3, 6 ),
 ( 6, 6 ),
 ( 3.046255633294209897, 5.238805263900000675, 7.431354894495790120 ),
 ( -0.0004283937457940030003, 2.000000000000000000 ),
 .UNSPECIFIED. ) ;
#88224=ADVANCED_FACE ( 'NONE', ( #77014 ), #14425, .T. ) ;
#88227=CARTESIAN_POINT ( 'NONE',  ( 18.87853829029999986, 1458.344553362990155, 213.8102309971890236 ) ) ;
#88233=ORIENTED_EDGE ( 'NONE', *, *, #32082, .T. ) ;
#88246=DIRECTION ( 'NONE',  ( 0.000000000000000000, -1.836970198721029688E-16, -1.000000000000000000 ) ) ;
#88251=CARTESIAN_POINT ( 'NONE',  ( -3.304790277399999976, 1430.055923981690057, 201.4699411825889968 ) ) ;
#88259=CARTESIAN_POINT ( 'NONE',  ( -3.338347951516314360, 1495.922107008597777, 197.9787877121366648 ) ) ;
#88260=CARTESIAN_POINT ( 'NONE',  ( 10.86756440871599949, 1470.431609380819964, 207.9091087289500308 ) ) ;
#88269=CARTESIAN_POINT ( 'NONE',  ( 3.365684841717370368, 1424.260763520689807, 191.4759580909079943 ) ) ;
#88289=CARTESIAN_POINT ( 'NONE',  ( -10.50807510266660039, 1489.705281234110089, 213.5102346389539889 ) ) ;
#88290=CARTESIAN_POINT ( 'NONE',  ( -21.46486249247640288, 1504.440131453050071, 215.6677484931969957 ) ) ;
#88299=EDGE_CURVE ( 'NONE', #1788, #77903, #102345, .T. ) ;
#88317=CARTESIAN_POINT ( 'NONE',  ( -9.315871017458929870, 1479.165496450050114, 216.1736367611900107 ) ) ;
#88319=CARTESIAN_POINT ( 'NONE',  ( -12.51045652733512981, 1414.677402202029953, 206.7437175916260230 ) ) ;
#88322=CARTESIAN_POINT ( 'NONE',  ( -11.61654445250000123, 1506.309187293489913, 207.9630299090890162 ) ) ;
#88323=CARTESIAN_POINT ( 'NONE',  ( 9.941274985550709431, 1491.817956606359985, 188.4486685046520051 ) ) ;
#88326=CARTESIAN_POINT ( 'NONE',  ( 8.209570662930000040, 1421.454114719120298, 196.1494337501989946 ) ) ;
#88337=CARTESIAN_POINT ( 'NONE',  ( -8.090248624290001800, 1425.035463411989895, 209.7688195370299979 ) ) ;
#88345=CARTESIAN_POINT ( 'NONE',  ( -3.141362685563839907, 1497.118792551569868, 221.1081249425609769 ) ) ;
#88347=ORIENTED_EDGE ( 'NONE', *, *, #63153, .T. ) ;
#88351=CARTESIAN_POINT ( 'NONE',  ( 10.38136293080000172, 1472.225397094090113, 214.0145097960790110 ) ) ;
#88353=CARTESIAN_POINT ( 'NONE',  ( -8.371011905599029745, 1438.923880247289844, 206.6694023295629847 ) ) ;
#88363=CARTESIAN_POINT ( 'NONE',  ( 11.26621375010180159, 1471.492305945939961, 211.0164925480820273 ) ) ;
#88376=VERTEX_POINT ( 'NONE', #81947 ) ;
#88393=CARTESIAN_POINT ( 'NONE',  ( -16.98382822079999954, 1417.304183444519822, 207.5927344675390032 ) ) ;
#88394=CARTESIAN_POINT ( 'NONE',  ( -6.103113815119999508, 1482.731685980090106, 200.3426744219489990 ) ) ;
#88395=CARTESIAN_POINT ( 'NONE',  ( -9.917060407088358787, 1483.572227753479865, 202.5254192721800166 ) ) ;
#88398=CARTESIAN_POINT ( 'NONE',  ( -4.326992699989999913, 1515.158586642790169, 209.1218459619010162 ) ) ;
#88403=CARTESIAN_POINT ( 'NONE',  ( -10.87726901145729919, 1461.906291937230208, 210.8265890786230159 ) ) ;
#88411=CARTESIAN_POINT ( 'NONE',  ( 11.85959186116559927, 1501.678157499889949, 211.5145819234840019 ) ) ;
#88417=CARTESIAN_POINT ( 'NONE',  ( 7.671698190030000752, 1427.928538830389925, 213.1259091499790088 ) ) ;
#88420=DIRECTION ( 'NONE',  ( 9.341989762165448955E-47, -1.000000000000000000, 1.836970198721029688E-16 ) ) ;
#88425=CARTESIAN_POINT ( 'NONE',  ( 5.151097723079999469, 1490.744826430290004, 188.9005472705989916 ) ) ;
#88431=ORIENTED_EDGE ( 'NONE', *, *, #46991, .T. ) ;
#88432=CARTESIAN_POINT ( 'NONE',  ( -2.861085386292339994, 1508.551704408389924, 220.0095495000269921 ) ) ;
#88438=CARTESIAN_POINT ( 'NONE',  ( 3.879020388191510182, 1465.465499240460076, 203.2370418086409813 ) ) ;
#88441=CARTESIAN_POINT ( 'NONE',  ( -10.10631778097200062, 1472.663248310899917, 207.2585624568480114 ) ) ;
#88447=CARTESIAN_POINT ( 'NONE',  ( 10.28019753094960009, 1422.778998439059933, 209.5284952118790045 ) ) ;
#88449=CARTESIAN_POINT ( 'NONE',  ( 10.93675118801170143, 1490.434561969760125, 209.9324825431089891 ) ) ;
#88452=EDGE_CURVE ( 'NONE', #80101, #36031, #46271, .T. ) ;
#88455=CARTESIAN_POINT ( 'NONE',  ( -0.5371945001445930234, 1496.425099764140214, 196.7755987515499783 ) ) ;
#88463=CARTESIAN_POINT ( 'NONE',  ( 3.628818059389999906, 1505.602008401590183, 221.3635115024989943 ) ) ;
#88465=EDGE_CURVE ( 'NONE', #70633, #52400, #106319, .T. ) ;
#88471=CARTESIAN_POINT ( 'NONE',  ( -17.61758723057469922, 1488.711492928860025, 197.7573658785580051 ) ) ;
#88481=CARTESIAN_POINT ( 'NONE',  ( 2.480332738680000038, 1486.002627324889772, 219.7500672349989941 ) ) ;
#88482=CARTESIAN_POINT ( 'NONE',  ( -5.100031674329999376, 1391.870658628590036, 214.4808810019090117 ) ) ;
#88484=VERTEX_POINT ( 'NONE', #76318 ) ;
#88487=CARTESIAN_POINT ( 'NONE',  ( -4.329448776275169664, 1515.064792882719985, 206.7917118343879963 ) ) ;
#88503=LINE ( 'NONE', #53827, #92812 ) ;
#88505=ADVANCED_FACE ( 'NONE', ( #8547 ), #69792, .T. ) ;
#88516=CARTESIAN_POINT ( 'NONE',  ( -4.886558140047800869, 1508.210669107129888, 220.4867294332269978 ) ) ;
#88517=CARTESIAN_POINT ( 'NONE',  ( 3.314513664071169874, 1498.768387937489933, 198.2102665491759979 ) ) ;
#88518=CARTESIAN_POINT ( 'NONE',  ( -4.092846354029450850, 1470.326128854550007, 218.4017925004950200 ) ) ;
#88521=CARTESIAN_POINT ( 'NONE',  ( 4.240938128610653557, 1509.032014137962506, 205.3774164840951357 ) ) ;
#88522=CARTESIAN_POINT ( 'NONE',  ( -6.927514301909999617, 1474.889786700390005, 201.4444059491990231 ) ) ;
#88523=CARTESIAN_POINT ( 'NONE',  ( 10.69530588519999981, 1492.057806767089915, 212.3894099842489993 ) ) ;
#88525=CARTESIAN_POINT ( 'NONE',  ( 7.937011329750911059, 1423.927594114607018, 195.7595643984233220 ) ) ;
#88526=CARTESIAN_POINT ( 'NONE',  ( -14.30100077960000071, 1503.190056882890076, 209.1269527976280074 ) ) ;
#88538=CARTESIAN_POINT ( 'NONE',  ( 4.581657872230000095, 1506.594992437789870, 219.8628132245989946 ) ) ;
#88539=CARTESIAN_POINT ( 'NONE',  ( -15.01049612569999958, 1415.677402202029953, 210.8311137397190009 ) ) ;
#88540=CARTESIAN_POINT ( 'NONE',  ( -5.534100668969379910, 1464.371862158079921, 199.5915835189479992 ) ) ;
#88543=ADVANCED_FACE ( 'NONE', ( #95328 ), #59107, .T. ) ;
#88555=CARTESIAN_POINT ( 'NONE',  ( -8.725374284720000873, 1478.773129111890057, 217.0898278110490196 ) ) ;
#88576=CARTESIAN_POINT ( 'NONE',  ( 5.898235284490000119, 1476.924971998690125, 199.0552711020989705 ) ) ;
#88580=CARTESIAN_POINT ( 'NONE',  ( -13.34067739081810089, 1508.245746154080052, 209.5313100501030021 ) ) ;
#88584=CARTESIAN_POINT ( 'NONE',  ( -11.79463582115499953, 1481.484189516729884, 210.3155264287200055 ) ) ;
#88592=EDGE_CURVE ( 'NONE', #288, #89851, #10832, .T. ) ;
#88599=CARTESIAN_POINT ( 'NONE',  ( -9.094607871690000067, 1498.018996692389919, 216.1637154482390031 ) ) ;
#88601=CARTESIAN_POINT ( 'NONE',  ( 1.778378100730000133, 1422.883737999489995, 193.3551376869990008 ) ) ;
#88605=CARTESIAN_POINT ( 'NONE',  ( -3.201099014209999982, 1451.080120310989969, 188.5408260424989919 ) ) ;
#88609=CARTESIAN_POINT ( 'NONE',  ( -5.087358518910000349, 1391.865222393290196, 203.6716085637289950 ) ) ;
#88611=CARTESIAN_POINT ( 'NONE',  ( -203.9558787908000284, -8382.262153571269664, 2179.147420460110425 ) ) ;
#88620=CARTESIAN_POINT ( 'NONE',  ( -13.34182121425549994, 1421.262884902478618, 210.6379646114695277 ) ) ;
#88633=CARTESIAN_POINT ( 'NONE',  ( -2.031695188920000117, 1468.162652163589883, 219.6587382871989860 ) ) ;
#88635=CARTESIAN_POINT ( 'NONE',  ( 12.49721897139709981, 1501.189573146680004, 211.4713583651110014 ) ) ;
#88639=CIRCLE ( 'NONE', #97575, 7.500000000000000000 ) ;
#88642=FACE_OUTER_BOUND ( 'NONE', #22481, .T. ) ;
#88643=CARTESIAN_POINT ( 'NONE',  ( -1.541238598094009972E-13, 1515.051704408389924, 212.9514660752490158 ) ) ;
#88651=CARTESIAN_POINT ( 'NONE',  ( 0.6565761022465029795, 1465.559853904359898, 198.1292258770540116 ) ) ;
#88662=VERTEX_POINT ( 'NONE', #31970 ) ;
#88665=CARTESIAN_POINT ( 'NONE',  ( -18.74471293385864712, 1508.457619993740082, 210.6713976521029110 ) ) ;
#88672=CARTESIAN_POINT ( 'NONE',  ( -5.584613240470000406, 1508.184945842690013, 220.3909862082990117 ) ) ;
#88688=CARTESIAN_POINT ( 'NONE',  ( -15.56145363769999967, 1415.973220584759929, 207.8153022160889805 ) ) ;
#88699=CARTESIAN_POINT ( 'NONE',  ( 1.471738374290000095, 1515.341568496189893, 213.3962787526390059 ) ) ;
#88700=AXIS2_PLACEMENT_3D ( 'NONE', #83621, #84174, #6375 ) ;
#88707=CARTESIAN_POINT ( 'NONE',  ( -0.6251419943069990159, 1430.668067383890047, 200.4025769807989832 ) ) ;
#88709=CARTESIAN_POINT ( 'NONE',  ( -15.94269987122453536, 1416.079329809435649, 209.7066221775000656 ) ) ;
#88710=CARTESIAN_POINT ( 'NONE',  ( -0.7502145772460020456, 1508.757402103690083, 220.8877261029990109 ) ) ;
#88711=CARTESIAN_POINT ( 'NONE',  ( -18.74729292449999818, 1442.199705176290081, 209.1218459616989946 ) ) ;
#88714=CARTESIAN_POINT ( 'NONE',  ( 9.577710299738889432, 1468.749342511669965, 205.5349571559659978 ) ) ;
#88722=CARTESIAN_POINT ( 'NONE',  ( -10.10336395149999866, 1482.676368233689800, 204.5951876114990000 ) ) ;
#88727=ORIENTED_EDGE ( 'NONE', *, *, #105580, .T. ) ;
#88728=CARTESIAN_POINT ( 'NONE',  ( -11.36969477628213276, 1501.477747086209320, 207.7773368182330671 ) ) ;
#88735=CARTESIAN_POINT ( 'NONE',  ( -4.993214560040000194, 1391.653934889589891, 203.5347113830289913 ) ) ;
#88736=CARTESIAN_POINT ( 'NONE',  ( 7.733699955179999641, 1424.219764885950099, 212.1813203967790002 ) ) ;
#88737=CARTESIAN_POINT ( 'NONE',  ( -21.59687142900000012, 1507.523380033690046, 209.4572543540780032 ) ) ;
#88740=ADVANCED_FACE ( 'NONE', ( #56636 ), #44768, .T. ) ;
#88742=CARTESIAN_POINT ( 'NONE',  ( 8.498877730000000241, 1453.128683867390009, 213.4054510080989928 ) ) ;
#88743=ORIENTED_EDGE ( 'NONE', *, *, #33017, .T. ) ;
#88748=CARTESIAN_POINT ( 'NONE',  ( 6.034821872916185548, 1499.876410579053299, 199.4702867286800938 ) ) ;
#88751=EDGE_CURVE ( 'NONE', #44452, #41116, #107577, .T. ) ;
#88771=ORIENTED_EDGE ( 'NONE', *, *, #15487, .F. ) ;
#88777=CARTESIAN_POINT ( 'NONE',  ( -11.96800804735369894, 1489.717015978450036, 211.5846796328700066 ) ) ;
#88786=CARTESIAN_POINT ( 'NONE',  ( 8.968032268709999144, 1477.614756788489785, 227.8520689727990032 ) ) ;
#88794=ORIENTED_EDGE ( 'NONE', *, *, #87774, .T. ) ;
#88800=CARTESIAN_POINT ( 'NONE',  ( -2.670663765640000520, 1430.456430591890012, 201.2104194720490113 ) ) ;
#88807=CARTESIAN_POINT ( 'NONE',  ( -3.393904228248314947, 1496.579901245492465, 198.4093902612280260 ) ) ;
#88808=CARTESIAN_POINT ( 'NONE',  ( 10.54397772302610115, 1470.567053305489935, 209.2853404595599898 ) ) ;
#88815=CARTESIAN_POINT ( 'NONE',  ( 17.69622264849999738, 1430.679833671289771, 213.5595385020990022 ) ) ;
#88817=CARTESIAN_POINT ( 'NONE',  ( 0.02750565378459880056, 1442.646891867090062, 219.1054768861489777 ) ) ;
#88830=CARTESIAN_POINT ( 'NONE',  ( -9.519511910620000350, 1508.480989645490126, 218.8877205799990122 ) ) ;
#88832=CARTESIAN_POINT ( 'NONE',  ( -19.39503999260000100, 1507.708763760590045, 209.4440057405769835 ) ) ;
#88834=CARTESIAN_POINT ( 'NONE',  ( -16.66194338029631439, 1417.248714584018671, 206.9614914337466587 ) ) ;
#88837=CARTESIAN_POINT ( 'NONE',  ( -3.829620113550000315, 1515.051704408389924, 209.0973262533439936 ) ) ;
#88839=CARTESIAN_POINT ( 'NONE',  ( -11.10192713642759976, 1489.530782677959905, 213.0257327280270090 ) ) ;
#88841=CARTESIAN_POINT ( 'NONE',  ( -17.55007709685750328, 1487.029497697219995, 194.9701149225189738 ) ) ;
#88851=ORIENTED_EDGE ( 'NONE', *, *, #79772, .F. ) ;
#88852=VERTEX_POINT ( 'NONE', #84025 ) ;
#88853=CARTESIAN_POINT ( 'NONE',  ( -7.799113859560000250, 1493.006535639589856, 207.9966435741489761 ) ) ;
#88860=CARTESIAN_POINT ( 'NONE',  ( -2.174738361970000255, 1481.606857451690075, 229.5102325974989981 ) ) ;
#88865=CARTESIAN_POINT ( 'NONE',  ( 1.771280571301239837, 1515.064792319160006, 213.4512947524970059 ) ) ;
#88869=CARTESIAN_POINT ( 'NONE',  ( -15.62861634609999761, 1418.244678181539939, 203.0179525210089935 ) ) ;
#88870=ORIENTED_EDGE ( 'NONE', *, *, #29653, .T. ) ;
#88872=CARTESIAN_POINT ( 'NONE',  ( -12.30879063490000114, 1505.268327336890025, 208.7613493058290146 ) ) ;
#88874=CARTESIAN_POINT ( 'NONE',  ( -11.88584868791679838, 1482.380097381399992, 228.1376906553660149 ) ) ;
#88882=CARTESIAN_POINT ( 'NONE',  ( -8.494894331139999366, 1459.365948010190095, 213.8040489441289935 ) ) ;
#88887=VERTEX_POINT ( 'NONE', #7867 ) ;
#88893=CARTESIAN_POINT ( 'NONE',  ( 2.034091252963869945, 1495.719183412219991, 221.2929912278799804 ) ) ;
#88894=VERTEX_POINT ( 'NONE', #15149 ) ;
#88904=ORIENTED_EDGE ( 'NONE', *, *, #77703, .T. ) ;
#88908=CARTESIAN_POINT ( 'NONE',  ( 19.04497961809999751, 1456.669328884790048, 205.4206990132790054 ) ) ;
#88935=CARTESIAN_POINT ( 'NONE',  ( -7.027952441359999192, 1482.449581481789892, 201.0380530320790058 ) ) ;
#88944=CARTESIAN_POINT ( 'NONE',  ( -10.47157504770849989, 1461.831102136270147, 210.4833357475050093 ) ) ;
#88949=CARTESIAN_POINT ( 'NONE',  ( 10.51777314836719945, 1480.734379257120054, 208.3815665556330146 ) ) ;
#88950=CIRCLE ( 'NONE', #33461, 9.341369339569999042 ) ;
#88952=CARTESIAN_POINT ( 'NONE',  ( -1.399663831989999885, 1443.805352974990228, 199.9250768807590077 ) ) ;
#88958=CARTESIAN_POINT ( 'NONE',  ( -21.59687146514269784, 1507.523380887320172, 209.4572544992919916 ) ) ;
#88960=CARTESIAN_POINT ( 'NONE',  ( -1966.823930461590180, 11221.53578756869865, -25.46789276350280318 ) ) ;
#88967=CARTESIAN_POINT ( 'NONE',  ( -5.062212445509999270, 1474.342205042089972, 198.8731682765990172 ) ) ;
#88971=CARTESIAN_POINT ( 'NONE',  ( -8.229004279106218789, 1439.448159900319979, 228.6152177230760003 ) ) ;
#88976=CARTESIAN_POINT ( 'NONE',  ( 6.315236557301221687, 1506.394552972206839, 218.9623958905396819 ) ) ;
#88977=CARTESIAN_POINT ( 'NONE',  ( -2.097032581780000182, 1432.708420430490150, 218.4264516295189935 ) ) ;
#88978=CARTESIAN_POINT ( 'NONE',  ( 7.700010710769999989, 1490.081763956990017, 208.3600023555910070 ) ) ;
#88985=CARTESIAN_POINT ( 'NONE',  ( 11.23938785293669795, 1490.970187199380234, 207.0635000114160107 ) ) ;
#88987=ORIENTED_EDGE ( 'NONE', *, *, #7765, .T. ) ;
#88990=CARTESIAN_POINT ( 'NONE',  ( -2.251423912408169858, 1495.949164212019923, 196.9898274163030010 ) ) ;
#89001=AXIS2_PLACEMENT_3D ( 'NONE', #51516, #578, #50431 ) ;
#89006=CARTESIAN_POINT ( 'NONE',  ( -10.48474110849999974, 1480.275079708390194, 208.2232256045050178 ) ) ;
#89024=ORIENTED_EDGE ( 'NONE', *, *, #42040, .T. ) ;
#89025=CIRCLE ( 'NONE', #24584, 0.5001123349366123350 ) ;
#89026=CARTESIAN_POINT ( 'NONE',  ( 9.707007897230489846, 1452.234270665119993, 209.8038064800559823 ) ) ;
#89027=CARTESIAN_POINT ( 'NONE',  ( 5.485856304330000377, 1423.003856355439893, 194.7031335851989695 ) ) ;
#89030=CARTESIAN_POINT ( 'NONE',  ( -5.824210366952714324, 1419.534194419528376, 194.8654209611248120 ) ) ;
#89049=CARTESIAN_POINT ( 'NONE',  ( -2.146051933368469999, 1508.551704408360138, 220.2827628139220053 ) ) ;
#89050=CARTESIAN_POINT ( 'NONE',  ( 3.424621566958379937, 1498.316785755180035, 198.1282711917500023 ) ) ;
#89052=CARTESIAN_POINT ( 'NONE',  ( -7.941319541319999509, 1469.154588994090091, 217.1846401660390029 ) ) ;
#89054=CARTESIAN_POINT ( 'NONE',  ( 11.16376535829999916, 1420.610325767149789, 198.7943618068990190 ) ) ;
#89056=CARTESIAN_POINT ( 'NONE',  ( -5.445054425793269814, 1494.866999379700246, 198.0707246423999948 ) ) ;
#89060=CARTESIAN_POINT ( 'NONE',  ( -19.24236553089999902, 1505.018157644889925, 209.0733177765920345 ) ) ;
#89064=CARTESIAN_POINT ( 'NONE',  ( -9.851036438101349546, 1439.921995732989899, 207.3463547441290302 ) ) ;
#89071=CARTESIAN_POINT ( 'NONE',  ( 5.237925579300000578, 1505.876516098390084, 219.6658948394990034 ) ) ;
#89074=CARTESIAN_POINT ( 'NONE',  ( -8.107801870790000365, 1463.844143246390104, 201.5100198155989801 ) ) ;
#89079=CARTESIAN_POINT ( 'NONE',  ( -1.337785777300729784, 1429.784825555620046, 199.8250566260579717 ) ) ;
#89081=CYLINDRICAL_SURFACE ( 'NONE', #49183, 0.4999999999999449329 ) ;
#89082=EDGE_CURVE ( 'NONE', #26024, #3898, #16630, .T. ) ;
#89084=CARTESIAN_POINT ( 'NONE',  ( 8.289359074433349406, 1461.164466581640227, 203.9471711042499749 ) ) ;
#89088=CARTESIAN_POINT ( 'NONE',  ( 10.01013843233299916, 1469.369181467840008, 209.9819040969830155 ) ) ;
#89094=EDGE_CURVE ( 'NONE', #31217, #108726, #84171, .T. ) ;
#89098=CARTESIAN_POINT ( 'NONE',  ( -14.24733479436660133, 1416.667683397399969, 203.2028330777899896 ) ) ;
#89103=CARTESIAN_POINT ( 'NONE',  ( -4.138993620949999119, 1515.551749212189861, 208.7474755485019955 ) ) ;
#89111=CARTESIAN_POINT ( 'NONE',  ( -11.00301364519999936, 1492.094801868890045, 210.0154387525699917 ) ) ;
#89121=CARTESIAN_POINT ( 'NONE',  ( -12.18503172777290011, 1490.802926859980062, 207.7326696222349938 ) ) ;
#89122=CARTESIAN_POINT ( 'NONE',  ( -3.548015302541859928, 1508.551704408389924, 204.3702150974099823 ) ) ;
#89133=CARTESIAN_POINT ( 'NONE',  ( -4.584247552609999943, 1495.956452401090019, 219.3622640912990107 ) ) ;
#89138=CARTESIAN_POINT ( 'NONE',  ( -16.49825404190000100, 1466.404193669789947, 220.8530316403990241 ) ) ;
#89144=CARTESIAN_POINT ( 'NONE',  ( -11.79257197010000091, 1490.424928053189888, 209.6468059298940148 ) ) ;
#89145=CARTESIAN_POINT ( 'NONE',  ( 17.00810803830026074, 1492.794519359084234, 195.6196894796988488 ) ) ;
#89151=CARTESIAN_POINT ( 'NONE',  ( -9.200421138165051360, 1422.937291722789951, 210.7384568321920142 ) ) ;
#89152=CARTESIAN_POINT ( 'NONE',  ( -10.64684140641754517, 1422.356867849525770, 210.6398257839229871 ) ) ;
#89155=ORIENTED_EDGE ( 'NONE', *, *, #69154, .T. ) ;
#89165=CARTESIAN_POINT ( 'NONE',  ( -0.06658362883100119034, 1468.466425048889960, 219.2800796028990078 ) ) ;
#89167=CARTESIAN_POINT ( 'NONE',  ( 8.099523513883839954, 1483.863015130160193, 216.2634084175389830 ) ) ;
#89170=CARTESIAN_POINT ( 'NONE',  ( 14.98723526979999932, 1429.231381954089784, 197.7821723486989924 ) ) ;
#89172=CARTESIAN_POINT ( 'NONE',  ( 0.5708672984259970384, 1460.784242392889837, 230.4191149236990270 ) ) ;
#89174=CARTESIAN_POINT ( 'NONE',  ( 5.312679136500000787, 1493.059131431590231, 218.8466398904690209 ) ) ;
#89200=CARTESIAN_POINT ( 'NONE',  ( 20.12203338850000023, 1473.683243806589871, 208.1564127194919820 ) ) ;
#89201=CARTESIAN_POINT ( 'NONE',  ( -5.652324135034829666, 1434.623555776060130, 216.9489395581130111 ) ) ;
#89209=AXIS2_PLACEMENT_3D ( 'NONE', #99888, #82567, #23186 ) ;
#89218=CARTESIAN_POINT ( 'NONE',  ( -5.010230764180000129, 1425.855359435129913, 208.5321074068529867 ) ) ;
#89223=CARTESIAN_POINT ( 'NONE',  ( -14.94752639080000023, 1415.823955448430070, 205.5818586423190197 ) ) ;
#89234=EDGE_CURVE ( 'NONE', #55990, #59685, #17684, .T. ) ;
#89235=CARTESIAN_POINT ( 'NONE',  ( 1.082449427709999856, 1515.225850744089939, 213.4470767797189978 ) ) ;
#89238=CARTESIAN_POINT ( 'NONE',  ( -4.623067421070000016, 1470.601194648889987, 189.6761541078989808 ) ) ;
#89240=CARTESIAN_POINT ( 'NONE',  ( -6.725822268156810502, 1439.879530295837412, 203.5093415176590383 ) ) ;
#89241=CARTESIAN_POINT ( 'NONE',  ( -3.703897191089999819, 1458.190786016390120, 219.1639864912989992 ) ) ;
#89249=CARTESIAN_POINT ( 'NONE',  ( 8.483440609833868606, 1468.250586555449900, 202.2169064785170178 ) ) ;
#89252=CARTESIAN_POINT ( 'NONE',  ( -17.18726318579999912, 1440.321463842890125, 217.4344804300990290 ) ) ;
#89257=CARTESIAN_POINT ( 'NONE',  ( 12.03449227190490056, 1491.353386486839781, 206.6667661091970274 ) ) ;
#89258=CARTESIAN_POINT ( 'NONE',  ( -10.67819692480000171, 1482.848997777490240, 204.9256918032390047 ) ) ;
#89265=CARTESIAN_POINT ( 'NONE',  ( -2.991447891192810182, 1436.484000074640107, 227.3801637149809949 ) ) ;
#89274=CARTESIAN_POINT ( 'NONE',  ( 8.060566621569998702, 1428.063481974589877, 213.0156338157989921 ) ) ;
#89294=CARTESIAN_POINT ( 'NONE',  ( -1.935216760905889899, 1464.825770518590161, 198.7112181189110061 ) ) ;
#89302=ORIENTED_EDGE ( 'NONE', *, *, #23308, .T. ) ;
#89326=DIRECTION ( 'NONE',  ( -9.341989762165448955E-47, 1.000000000000000000, -1.836970198721029688E-16 ) ) ;
#89329=CARTESIAN_POINT ( 'NONE',  ( 12.96503937710000010, 1476.856299447390029, 225.6431713718990011 ) ) ;
#89334=EDGE_CURVE ( 'NONE', #77692, #76715, #95415, .T. ) ;
#89337=CARTESIAN_POINT ( 'NONE',  ( 15.62837127357619771, 1427.648990501440039, 199.9598782853679779 ) ) ;
#89343=VERTEX_POINT ( 'NONE', #65264 ) ;
#89346=CARTESIAN_POINT ( 'NONE',  ( -2.847681058950000121, 1430.845634743689970, 201.2564363298089916 ) ) ;
#89351=CARTESIAN_POINT ( 'NONE',  ( 12.26530152830000020, 1421.362759829509969, 204.2608483305789946 ) ) ;
#89354=CARTESIAN_POINT ( 'NONE',  ( -16.70830179842720042, 1417.149226859160080, 207.3570905742490140 ) ) ;
#89360=CARTESIAN_POINT ( 'NONE',  ( 10.28987036248729936, 1480.775536434839751, 206.8081037193859970 ) ) ;
#89365=ADVANCED_FACE ( 'NONE', ( #82601 ), #50112, .T. ) ;
#89366=CARTESIAN_POINT ( 'NONE',  ( 7.948444925817987006, 1423.758263538081110, 195.8503688939058804 ) ) ;
#89368=CARTESIAN_POINT ( 'NONE',  ( 1.329590663860000133, 1443.548274132990173, 217.9512969677389833 ) ) ;
#89373=CARTESIAN_POINT ( 'NONE',  ( -2.834860085976320221, 1464.859481028689970, 198.4842492681709984 ) ) ;
#89375=CARTESIAN_POINT ( 'NONE',  ( 3.535327672168380175, 1487.160996015089950, 197.6951163816430039 ) ) ;
#89378=EDGE_LOOP ( 'NONE', ( #78776, #82620, #50491, #2026, #87391, #83660 ) ) ;
#89383=CARTESIAN_POINT ( 'NONE',  ( -2.170628039509999940, 1485.611815934889819, 197.4219877966989998 ) ) ;
#89388=B_SPLINE_SURFACE_WITH_KNOTS ( 'NONE', 5, 1, ( 
 ( #47205, #46125 ),
 ( #37147, #105457 ),
 ( #81332, #72960 ),
 ( #80255, #107097 ),
 ( #71899, #30386 ),
 ( #57280, #84091 ) ),
 .UNSPECIFIED., .F., .F., .F.,
 ( 6, 6 ),
 ( 2, 2 ),
 ( 0.000000000000000000, 4.001056960039999666 ),
 ( 0.000000000000000000, 14.00000000000000000 ),
 .UNSPECIFIED. ) ;
#89392=CARTESIAN_POINT ( 'NONE',  ( -9.838233766173130945, 1462.268829427310038, 227.9668122194469788 ) ) ;
#89393=CARTESIAN_POINT ( 'NONE',  ( -14.94996665966239924, 1415.677402202029953, 207.1999397929429847 ) ) ;
#89395=CARTESIAN_POINT ( 'NONE',  ( 4.506137960680000276, 1429.623679839590068, 216.5655692257590204 ) ) ;
#89414=CARTESIAN_POINT ( 'NONE',  ( -0.1187972037638400091, 1515.157712620099801, 213.4488615487820198 ) ) ;
#89416=CARTESIAN_POINT ( 'NONE',  ( -10.41014360099929981, 1479.888900791299875, 214.5375557550950134 ) ) ;
#89420=ORIENTED_EDGE ( 'NONE', *, *, #57002, .F. ) ;
#89422=CARTESIAN_POINT ( 'NONE',  ( -21.55607067240000063, 1488.682141303889921, 202.2062732307990132 ) ) ;
#89424=CARTESIAN_POINT ( 'NONE',  ( 7.634170062339999063, 1421.957731401030060, 195.7691812542990135 ) ) ;
#89432=CARTESIAN_POINT ( 'NONE',  ( -3.586339042944182598, 1515.071394417498368, 205.0391425136844248 ) ) ;
#89441=CARTESIAN_POINT ( 'NONE',  ( -10.93363683719999813, 1471.692480041690033, 205.6467075678189929 ) ) ;
#89442=FACE_OUTER_BOUND ( 'NONE', #54898, .T. ) ;
#89446=ORIENTED_EDGE ( 'NONE', *, *, #100468, .F. ) ;
#89449=CARTESIAN_POINT ( 'NONE',  ( 7.800297031879999565, 1471.072109769290137, 215.6814025974289848 ) ) ;
#89459=CARTESIAN_POINT ( 'NONE',  ( 1.836900179243859954, 1466.949332984869898, 220.0337271301659996 ) ) ;
#89460=CARTESIAN_POINT ( 'NONE',  ( 19.33955305990000184, 1457.046069667190068, 207.2605506525090107 ) ) ;
#89464=CARTESIAN_POINT ( 'NONE',  ( 10.13545575494789830, 1453.511789163979984, 212.2748783515349942 ) ) ;
#89477=EDGE_CURVE ( 'NONE', #58839, #38904, #103530, .T. ) ;
#89479=CARTESIAN_POINT ( 'NONE',  ( -3.709420239419999987, 1414.325356040540100, 206.4743715362490093 ) ) ;
#89503=CARTESIAN_POINT ( 'NONE',  ( 9.817766946204249834, 1499.485800321180022, 202.4310653781669771 ) ) ;
#89507=CARTESIAN_POINT ( 'NONE',  ( -2.746473951679999637, 1441.879883984389835, 200.6855579648789956 ) ) ;
#89509=CARTESIAN_POINT ( 'NONE',  ( -10.87194929170000002, 1491.777874968590140, 211.0477909272190118 ) ) ;
#89512=CARTESIAN_POINT ( 'NONE',  ( -3.176055666263430055, 1508.610720281340036, 204.4420550583219836 ) ) ;
#89514=CARTESIAN_POINT ( 'NONE',  ( -11.50607850114139907, 1501.456740653870156, 208.7151705893799942 ) ) ;
#89520=CARTESIAN_POINT ( 'NONE',  ( -3.428118280760000136, 1475.747349183789993, 199.2424158423789891 ) ) ;
#89522=ORIENTED_EDGE ( 'NONE', *, *, #72271, .T. ) ;
#89523=CARTESIAN_POINT ( 'NONE',  ( -4.705763804352860014, 1479.984617471649926, 230.9466402758990000 ) ) ;
#89525=B_SPLINE_CURVE_WITH_KNOTS ( 'NONE', 5,
 ( #81083, #49158, #97875, #4399, #38527, #90581, #48045, #21705, #106829 ),
 .UNSPECIFIED., .F., .F.,
 ( 6, 3, 6 ),
 ( -24.01273564469999755, -22.33923004749999919, -20.66572445029999727 ),
 .UNSPECIFIED. ) ;
#89535=CARTESIAN_POINT ( 'NONE',  ( 3.354719857970000163, 1453.857986919590076, 214.8728744567289937 ) ) ;
#89546=B_SPLINE_CURVE_WITH_KNOTS ( 'NONE', 3,
 ( #38451, #46888, #107860, #105684, #64236, #63157, #20533, #47422, #39563, #3788, #37921, #31149, #13782, #89958, #22175, #72101, #65337, #55837, #98905, #73170, #107314, #64796, #29499, #30044, #54190, #106217, #88317, #13233, #11611, #45788, #97804, #21631, #21082, #89416, #81545, #12704, #81014, #4320, #106755, #4846, #30608, #56374, #90504, #32262, #65883, #100004 ),
 .UNSPECIFIED., .F., .F.,
 ( 4, 3, 3, 3, 3, 3, 3, 3, 3, 3, 3, 3, 3, 3, 3, 4 ),
 ( -34.67967148219459972, -33.25777146041880172, -31.83587143864300018, -30.43034291442640082, -29.01390005850370102, -27.61223930463379972, -26.21389002340420049, -24.81975935856400284, -23.82611339485449875, -22.43810463356840046, -21.04786899275110201, -19.65824082723219846, -18.27352136797000171, -16.89443640706300087, -15.52263656855669893, -14.15949905700000144 ),
 .UNSPECIFIED. ) ;
#89554=CARTESIAN_POINT ( 'NONE',  ( 1.514120561980000183E-16, 1515.551704408389924, 209.1218459616989946 ) ) ;
#89559=FACE_OUTER_BOUND ( 'NONE', #48401, .T. ) ;
#89562=ORIENTED_EDGE ( 'NONE', *, *, #103560, .F. ) ;
#89569=CARTESIAN_POINT ( 'NONE',  ( -0.2696770069730009545, 1486.167527700089977, 220.6462483113989776 ) ) ;
#89573=CARTESIAN_POINT ( 'NONE',  ( 11.24566101859999812, 1493.273975466890079, 214.3640310562390141 ) ) ;
#89578=CARTESIAN_POINT ( 'NONE',  ( 9.394927480355990568, 1451.851897013709959, 209.9054632338170165 ) ) ;
#89581=CARTESIAN_POINT ( 'NONE',  ( -3.847666503130200422, 1440.496978037559984, 204.4642126257899974 ) ) ;
#89582=DIRECTION ( 'NONE',  ( 0.000000000000000000, -1.836970198721029688E-16, -1.000000000000000000 ) ) ;
#89593=CARTESIAN_POINT ( 'NONE',  ( 6.919958127207899601, 1483.315291266040049, 218.7186626761050263 ) ) ;
#89600=CARTESIAN_POINT ( 'NONE',  ( -4.438955121070089938, 1469.007804208310063, 218.6173878029609909 ) ) ;
#89602=CARTESIAN_POINT ( 'NONE',  ( 10.46957727719999909, 1420.496586446350193, 197.8100847527989856 ) ) ;
#89603=CARTESIAN_POINT ( 'NONE',  ( -0.6258287210304879222, 1475.511722453250059, 220.5356275081750255 ) ) ;
#89609=CARTESIAN_POINT ( 'NONE',  ( 11.35837942423910008, 1422.392381634520007, 207.1029687616070021 ) ) ;
#89611=CARTESIAN_POINT ( 'NONE',  ( -9.552138306242289545, 1440.406794419209973, 206.0807338902480126 ) ) ;
#89613=EDGE_LOOP ( 'NONE', ( #57401, #12998, #48308, #64817, #81724 ) ) ;
#89614=CARTESIAN_POINT ( 'NONE',  ( 4.687651746879999415, 1478.378160227390254, 228.9010599218989910 ) ) ;
#89615=CARTESIAN_POINT ( 'NONE',  ( -16.94401720158110081, 1417.331033520996471, 206.9668984956705629 ) ) ;
#89618=CARTESIAN_POINT ( 'NONE',  ( -15.28223244349999987, 1416.009837697190051, 211.6183304183890073 ) ) ;
#89620=CARTESIAN_POINT ( 'NONE',  ( -10.61999372029469946, 1462.990852176999852, 206.0510140530389833 ) ) ;
#89625=CARTESIAN_POINT ( 'NONE',  ( -7.005911337589346921, 1476.499442542723500, 216.7627521230403431 ) ) ;
#89626=CARTESIAN_POINT ( 'NONE',  ( -1.968833673825499897, 1429.476492495610046, 199.9497084242159985 ) ) ;
#89630=CARTESIAN_POINT ( 'NONE',  ( 2.981764581055819985, 1456.749145475010209, 198.8578628538780322 ) ) ;
#89643=CARTESIAN_POINT ( 'NONE',  ( 12.45662817246929954, 1427.088122696140090, 206.6493147128259977 ) ) ;
#89644=DIRECTION ( 'NONE',  ( 1.224227143275519934E-16, 0.02617694830788819954, -0.9996573249755569268 ) ) ;
#89648=CARTESIAN_POINT ( 'NONE',  ( -4.328507300020000059, 1515.100746401290053, 208.0463350318690061 ) ) ;
#89649=CARTESIAN_POINT ( 'NONE',  ( 0.4812364869308506932, 1484.453808314565094, 198.4264615785256467 ) ) ;
#89654=CARTESIAN_POINT ( 'NONE',  ( 2.224758152370000186, 1476.466451172889947, 198.2506516725989911 ) ) ;
#89656=CARTESIAN_POINT ( 'NONE',  ( -11.00740228139999921, 1492.792315462490023, 207.9066467806190133 ) ) ;
#89657=CARTESIAN_POINT ( 'NONE',  ( 0.1903840683780030074, 1469.229546031989912, 189.1368665698990128 ) ) ;
#89665=CARTESIAN_POINT ( 'NONE',  ( -12.24498567495730050, 1490.542231505709879, 208.5855889815660191 ) ) ;
#89666=CARTESIAN_POINT ( 'NONE',  ( -4.943465364638519155, 1508.551704408389924, 206.1607460916300170 ) ) ;
#89669=CARTESIAN_POINT ( 'NONE',  ( 0.9157618521929991040, 1508.480794317990103, 218.1010525276389842 ) ) ;
#89674=ADVANCED_FACE ( 'NONE', ( #62395 ), #37632, .F. ) ;
#89682=CARTESIAN_POINT ( 'NONE',  ( -9.838236027148290930, 1462.268809849160107, 227.9668099468159710 ) ) ;
#89695=CARTESIAN_POINT ( 'NONE',  ( -8843.778997819570577, -2339.246371527898646, 3013.944470869236739 ) ) ;
#89708=B_SPLINE_CURVE_WITH_KNOTS ( 'NONE', 3,
 ( #56354, #71541, #97784, #80995, #89936, #2663, #20510, #37344, #98886, #45768, #105097, #4301, #28387 ),
 .UNSPECIFIED., .F., .F.,
 ( 4, 3, 3, 3, 4 ),
 ( 0.000000000000000000, 0.9326141499816539282, 1.865530147010150186, 2.798283637250339684, 3.468500186270000007 ),
 .UNSPECIFIED. ) ;
#89713=CARTESIAN_POINT ( 'NONE',  ( 10.77494494982569861, 1480.716361118370060, 211.2102488021930071 ) ) ;
#89717=CARTESIAN_POINT ( 'NONE',  ( 8.897749601629998395, 1427.579448381289922, 192.9038597873990284 ) ) ;
#89718=CARTESIAN_POINT ( 'NONE',  ( 10.75631864630000045, 1451.138109685189875, 190.3409053448989994 ) ) ;
#89722=ADVANCED_FACE ( 'NONE', ( #59486 ), #65425, .T. ) ;
#89723=ORIENTED_EDGE ( 'NONE', *, *, #110291, .F. ) ;
#89724=B_SPLINE_CURVE_WITH_KNOTS ( 'NONE', 3,
 ( #51040, #6271, #40419, #57803, #74596, #32023 ),
 .UNSPECIFIED., .F., .F.,
 ( 4, 2, 4 ),
 ( 0.000000000000000000, 0.5000000000000000000, 1.000000000000000000 ),
 .UNSPECIFIED. ) ;
#89730=CARTESIAN_POINT ( 'NONE',  ( -18.52166933778729785, 1508.551400274589923, 210.3449052712999787 ) ) ;
#89736=ORIENTED_EDGE ( 'NONE', *, *, #103476, .T. ) ;
#89746=B_SPLINE_CURVE_WITH_KNOTS ( 'NONE', 3,
 ( #72814, #98543, #31895, #23490, #57682, #107497, #91796, #30789, #46522, #106405 ),
 .UNSPECIFIED., .F., .F.,
 ( 4, 2, 2, 2, 4 ),
 ( 0.000000000000000000, 0.2500000000000000000, 0.5000000000000000000, 0.7500000000000000000, 1.000000000000000000 ),
 .UNSPECIFIED. ) ;
#89748=CARTESIAN_POINT ( 'NONE',  ( -7.332452461205139826, 1435.726086304749970, 215.5220642470920325 ) ) ;
#89757=CARTESIAN_POINT ( 'NONE',  ( -0.9205759412220010374, 1469.929133761889943, 216.3346150991189916 ) ) ;
#89763=CARTESIAN_POINT ( 'NONE',  ( -3.264420175239999722, 1430.087089178589849, 204.4765990926489962 ) ) ;
#89768=CARTESIAN_POINT ( 'NONE',  ( -2.170627987649289992, 1485.611815795640041, 197.4219879416550327 ) ) ;
#89770=CARTESIAN_POINT ( 'NONE',  ( -14.72897262537098584, 1415.677402202029953, 211.7043269262228762 ) ) ;
#89771=CARTESIAN_POINT ( 'NONE',  ( -13.35314405190779929, 1481.629087625479769, 225.5920811498180001 ) ) ;
#89777=ORIENTED_EDGE ( 'NONE', *, *, #46047, .F. ) ;
#89786=CARTESIAN_POINT ( 'NONE',  ( -10.13093604337480080, 1447.191456030310064, 211.1552813046679944 ) ) ;
#89810=CARTESIAN_POINT ( 'NONE',  ( -2.656558671120380133, 1508.551704408389924, 204.1390352724760078 ) ) ;
#89819=CARTESIAN_POINT ( 'NONE',  ( -7.160726076929999628, 1452.136940029189873, 201.9019911547090089 ) ) ;
#89822=CARTESIAN_POINT ( 'NONE',  ( 7.069913304450000879, 1426.666554455719961, 213.2414280093890113 ) ) ;
#89823=CARTESIAN_POINT ( 'NONE',  ( 16.66442743440000029, 1492.498864364090196, 193.3249227319990098 ) ) ;
#89828=EDGE_CURVE ( 'NONE', #60200, #41219, #44649, .T. ) ;
#89829=CARTESIAN_POINT ( 'NONE',  ( 8.723132970039999989, 1451.781319090490115, 212.2855359169589917 ) ) ;
#89838=CARTESIAN_POINT ( 'NONE',  ( -21.50507852072029991, 1505.473545802760100, 209.5822816567780080 ) ) ;
#89851=VERTEX_POINT ( 'NONE', #1653 ) ;
#89854=CARTESIAN_POINT ( 'NONE',  ( 12.32716646574370145, 1492.190914138330072, 209.5898718627249764 ) ) ;
#89862=CARTESIAN_POINT ( 'NONE',  ( -17.97364528888469692, 1508.456286852059975, 211.9534032401529942 ) ) ;
#89872=ORIENTED_EDGE ( 'NONE', *, *, #61336, .F. ) ;
#89873=DIRECTION ( 'NONE',  ( 1.000000000000000000, 0.000000000000000000, 0.000000000000000000 ) ) ;
#89894=CARTESIAN_POINT ( 'NONE',  ( 10.78022355800000120, 1423.856158455210107, 204.2982030289390138 ) ) ;
#89900=CARTESIAN_POINT ( 'NONE',  ( 10.38868706420140064, 1469.976612653159918, 207.5338502487639971 ) ) ;
#89908=CARTESIAN_POINT ( 'NONE',  ( 2.729745825120000191, 1442.383552003789873, 217.6907392106589896 ) ) ;
#89915=CARTESIAN_POINT ( 'NONE',  ( 2.719262146893400038E-32, 1524.051704408389924, 209.1218459616989946 ) ) ;
#89919=ORIENTED_EDGE ( 'NONE', *, *, #48082, .F. ) ;
#89922=CARTESIAN_POINT ( 'NONE',  ( -8.869906122459999764, 1508.539665163490099, 218.9157064153390024 ) ) ;
#89924=CARTESIAN_POINT ( 'NONE',  ( 11.34715271451710095, 1470.684505017819902, 208.1686757782699999 ) ) ;
#89931=CARTESIAN_POINT ( 'NONE',  ( -17.84103545810000213, 1489.004099770289940, 195.1797354288989936 ) ) ;
#89933=CARTESIAN_POINT ( 'NONE',  ( -9.658033403218869495, 1460.449140326730003, 209.2581822647210004 ) ) ;
#89936=CARTESIAN_POINT ( 'NONE',  ( -18.59348773727160165, 1443.611734087849982, 211.9870899472090002 ) ) ;
#89943=FACE_OUTER_BOUND ( 'NONE', #6415, .T. ) ;
#89948=EDGE_CURVE ( 'NONE', #52143, #8084, #35923, .T. ) ;
#89949=CARTESIAN_POINT ( 'NONE',  ( 9.682472890002770782, 1436.279939607890128, 210.8543570392099866 ) ) ;
#89952=DIRECTION ( 'NONE',  ( 0.9236442117861071166, -0.3798549797792020732, 0.05090740978445951193 ) ) ;
#89954=CARTESIAN_POINT ( 'NONE',  ( 9.371512452695059281, 1464.461258777040030, 212.0981161559300290 ) ) ;
#89958=CARTESIAN_POINT ( 'NONE',  ( -6.828376997004060200, 1477.897708468349947, 218.4866115316829962 ) ) ;
#89960=EDGE_CURVE ( 'NONE', #101100, #67656, #24566, .T. ) ;
#89963=VERTEX_POINT ( 'NONE', #44487 ) ;
#89965=CARTESIAN_POINT ( 'NONE',  ( -12.86821319049999879, 1505.199346322990095, 208.9590989587390197 ) ) ;
#89966=CARTESIAN_POINT ( 'NONE',  ( -11.99264260133359983, 1481.591995386910185, 228.0251739801319957 ) ) ;
#89974=CARTESIAN_POINT ( 'NONE',  ( -4.963305069829999638, 1458.663087589289944, 218.6479516874489946 ) ) ;
#89983=CARTESIAN_POINT ( 'NONE',  ( -8.610796597750850268, 1448.268247762119927, 212.2416356316149972 ) ) ;
#89993=CARTESIAN_POINT ( 'NONE',  ( 9.563615785819999715, 1471.196293976290008, 212.9450669879490192 ) ) ;
#90002=CARTESIAN_POINT ( 'NONE',  ( 1.144541242519509838, 1467.157765914260153, 220.1362019054899974 ) ) ;
#90015=CARTESIAN_POINT ( 'NONE',  ( -5.292247061280000331, 1391.913060387289988, 214.4361776263990009 ) ) ;
#90021=CARTESIAN_POINT ( 'NONE',  ( 10.58556907870000074, 1489.200871216989981, 206.2039989270789988 ) ) ;
#90036=CARTESIAN_POINT ( 'NONE',  ( -0.2705593682478190098, 1455.625011699110019, 198.5897262588950127 ) ) ;
#90039=CARTESIAN_POINT ( 'NONE',  ( 10.83571774430070001, 1499.415958313539932, 203.3525490312119928 ) ) ;
#90060=CARTESIAN_POINT ( 'NONE',  ( 4.206093649894939723, 1508.551704408389924, 204.8199791756389914 ) ) ;
#90062=ORIENTED_EDGE ( 'NONE', *, *, #89477, .F. ) ;
#90063=CARTESIAN_POINT ( 'NONE',  ( -16.61338081808710143, 1463.629459303540216, 220.4654957482720192 ) ) ;
#90074=CARTESIAN_POINT ( 'NONE',  ( 18.30701642943642327, 1458.756281124563429, 215.8796111928478467 ) ) ;
#90082=CARTESIAN_POINT ( 'NONE',  ( -18.61360911655499706, 1441.740792946530064, 211.1815796315490275 ) ) ;
#90087=CARTESIAN_POINT ( 'NONE',  ( -14.90843596520000069, 1420.513868878929998, 212.4962506662589874 ) ) ;
#90095=CARTESIAN_POINT ( 'NONE',  ( -9.436093020126769204, 1447.921129549329862, 210.5458514588860055 ) ) ;
#90099=EDGE_CURVE ( 'NONE', #86013, #25072, #107540, .T. ) ;
#90104=DIRECTION ( 'NONE',  ( 0.000000000000000000, -1.000000000000000000, 0.000000000000000000 ) ) ;
#90118=ORIENTED_EDGE ( 'NONE', *, *, #2155, .T. ) ;
#90122=EDGE_LOOP ( 'NONE', ( #21024, #45942, #108676, #108662, #108352 ) ) ;
#90124=CARTESIAN_POINT ( 'NONE',  ( 3.394586472146719824, 1484.752177823880174, 220.4731790846979891 ) ) ;
#90133=CARTESIAN_POINT ( 'NONE',  ( 9.365354866811589574, 1482.088108353989810, 216.3257182807389825 ) ) ;
#90135=ORIENTED_EDGE ( 'NONE', *, *, #80244, .T. ) ;
#90137=CARTESIAN_POINT ( 'NONE',  ( 1.909107468229654714, 1507.666028270077504, 220.7249166300547358 ) ) ;
#90139=CARTESIAN_POINT ( 'NONE',  ( 5.663308409567039625, 1499.770466072930049, 199.1301411769080119 ) ) ;
#90143=CARTESIAN_POINT ( 'NONE',  ( -1.848955060214049873, 1475.902979036260149, 220.4212878429429736 ) ) ;
#90144=CARTESIAN_POINT ( 'NONE',  ( -8.008213785660771578, 1493.854461180789940, 199.7736228595420016 ) ) ;
#90150=CARTESIAN_POINT ( 'NONE',  ( 10.79885338082780066, 1425.173319402769948, 206.5250427735439871 ) ) ;
#90160=CARTESIAN_POINT ( 'NONE',  ( 10.85890618524230078, 1422.250279490929870, 211.0007653617559811 ) ) ;
#90161=CARTESIAN_POINT ( 'NONE',  ( -15.99559901427390152, 1420.209675652329906, 209.9241255724960240 ) ) ;
#90162=ORIENTED_EDGE ( 'NONE', *, *, #17925, .F. ) ;
#90163=CARTESIAN_POINT ( 'NONE',  ( 3.972455588910000390, 1429.380171581789909, 216.5671372490689919 ) ) ;
#90165=CARTESIAN_POINT ( 'NONE',  ( -16.91437598810000154, 1417.214259571060211, 207.5096547060990133 ) ) ;
#90174=CARTESIAN_POINT ( 'NONE',  ( 5.826428076080000906, 1473.811884028689974, 218.9454251420289950 ) ) ;
#90180=CARTESIAN_POINT ( 'NONE',  ( 0.008839277919110500800, 1515.608558013090033, 205.0604244730189976 ) ) ;
#90188=CARTESIAN_POINT ( 'NONE',  ( -1.427677631911417722, 1483.943482002980318, 198.5321935292907938 ) ) ;
#90193=CARTESIAN_POINT ( 'NONE',  ( 0.9648462396720020040, 1486.192668660790105, 197.6233019413989780 ) ) ;
#90194=CARTESIAN_POINT ( 'NONE',  ( 7.697536492340000258, 1477.591864417890065, 200.7729169044390005 ) ) ;
#90196=CARTESIAN_POINT ( 'NONE',  ( -12.16861649890000052, 1490.861372319089924, 207.5435353620889884 ) ) ;
#90197=CARTESIAN_POINT ( 'NONE',  ( 4.032933083790000595, 1469.757081955990088, 189.5597133099989833 ) ) ;
#90200=CARTESIAN_POINT ( 'NONE',  ( 8.877584795860000710, 1422.885319099519847, 212.4206523501590027 ) ) ;
#90204=CARTESIAN_POINT ( 'NONE',  ( -12.22107531762499910, 1490.677116594589961, 208.1386805918920118 ) ) ;
#90205=CARTESIAN_POINT ( 'NONE',  ( -4.923477628844170617, 1508.551704408389924, 206.0739344081519846 ) ) ;
#90213=CARTESIAN_POINT ( 'NONE',  ( 9.751547273671640426, 1469.879570846299885, 211.6488722629640051 ) ) ;
#90214=CARTESIAN_POINT ( 'NONE',  ( -3.805396659119999914, 1495.647976226690162, 219.6495707272989932 ) ) ;
#90221=CARTESIAN_POINT ( 'NONE',  ( -13.29931690873070060, 1469.324185722580069, 191.9832587503309753 ) ) ;
#90241=CARTESIAN_POINT ( 'NONE',  ( 4.270716329343290596, 1515.320037145160768, 207.2788824689123146 ) ) ;
#90243=CARTESIAN_POINT ( 'NONE',  ( 0.1723259509675250101, 1485.814687721770042, 221.0067211994579850 ) ) ;
#90249=B_SPLINE_CURVE_WITH_KNOTS ( 'NONE', 3,
 ( #77406, #92532, #7983, #76300, #169, #66280, #75756, #24221, #9094, #109366, #57864, #33729, #85796, #15269, #49460, #25316 ),
 .UNSPECIFIED., .F., .F.,
 ( 4, 3, 3, 3, 3, 4 ),
 ( -7.174280551130140182, -6.801970038525639417, -5.833526344350429937, -4.869644975469700654, -3.907991620792370391, -2.949396961919999782 ),
 .UNSPECIFIED. ) ;
#90253=CARTESIAN_POINT ( 'NONE',  ( 10.47513610250140026, 1482.040573979539886, 210.7457604718050277 ) ) ;
#90258=CARTESIAN_POINT ( 'NONE',  ( -17.11734146840720072, 1420.830825731939967, 201.6585919051609892 ) ) ;
#90259=CARTESIAN_POINT ( 'NONE',  ( -3.628948333386136760, 1428.810397315499131, 201.2247650147968443 ) ) ;
#90261=ORIENTED_EDGE ( 'NONE', *, *, #28676, .F. ) ;
#90268=CARTESIAN_POINT ( 'NONE',  ( -0.4093345880009989779, 1463.508080861789949, 199.3143980028889928 ) ) ;
#90285=CARTESIAN_POINT ( 'NONE',  ( -9.511752073085270709, 1460.963492925100127, 207.2886318349059991 ) ) ;
#90286=CARTESIAN_POINT ( 'NONE',  ( -9.735527157094869821, 1438.291168724430008, 211.0143517203420060 ) ) ;
#90296=CARTESIAN_POINT ( 'NONE',  ( -10.48474110849999974, 1480.275079708390194, 208.2232256045050178 ) ) ;
#90299=EDGE_CURVE ( 'NONE', #46147, #54902, #54000, .T. ) ;
#90300=CARTESIAN_POINT ( 'NONE',  ( 2.329906356571290083, 1515.372228416479857, 213.3835081553520183 ) ) ;
#90308=CARTESIAN_POINT ( 'NONE',  ( -14.35836953849999986, 1415.677402244120003, 204.5300376431989946 ) ) ;
#90310=CARTESIAN_POINT ( 'NONE',  ( -6.997302092268090412, 1441.814629485520072, 202.4571293489870243 ) ) ;
#90320=CARTESIAN_POINT ( 'NONE',  ( -1.842962231260000028, 1515.551704408389924, 212.9514660752490158 ) ) ;
#90324=DIRECTION ( 'NONE',  ( -0.1612154892182530996, 0.3709952640053770789, 0.9145338047998552433 ) ) ;
#90326=CARTESIAN_POINT ( 'NONE',  ( -7.368358975295519642, 1439.428462140772353, 204.4148736406934574 ) ) ;
#90338=DIRECTION ( 'NONE',  ( 0.02091224828123159837, -0.9990482215818557998, 0.03827961371219689574 ) ) ;
#90347=CARTESIAN_POINT ( 'NONE',  ( 12.54950410350970103, 1421.558086165679924, 207.1374001497979975 ) ) ;
#90354=CARTESIAN_POINT ( 'NONE',  ( -18.29179276165280044, 1466.060368039130026, 217.7541609266880016 ) ) ;
#90361=CARTESIAN_POINT ( 'NONE',  ( 19.38664720319999901, 1498.811923108090014, 221.8202413673990065 ) ) ;
#90363=CARTESIAN_POINT ( 'NONE',  ( -17.65294116109440026, 1419.923224108780005, 204.6037421101960376 ) ) ;
#90366=LINE ( 'NONE', #106088, #44352 ) ;
#90387=ORIENTED_EDGE ( 'NONE', *, *, #86501, .T. ) ;
#90397=CARTESIAN_POINT ( 'NONE',  ( -17.33117438843089886, 1508.522386692640112, 212.5847705537780143 ) ) ;
#90404=ORIENTED_EDGE ( 'NONE', *, *, #4245, .T. ) ;
#90407=B_SPLINE_SURFACE_WITH_KNOTS ( 'NONE', 5, 1, ( 
 ( #15807, #42157 ),
 ( #25880, #103141 ),
 ( #17467, #102038 ),
 ( #27014, #8537 ),
 ( #77960, #58963 ),
 ( #85241, #60080 ) ),
 .UNSPECIFIED., .F., .F., .F.,
 ( 6, 6 ),
 ( 2, 2 ),
 ( 0.000000000000000000, 3.468500186270000007 ),
 ( 0.000000000000000000, 14.00000000000000000 ),
 .UNSPECIFIED. ) ;
#90422=CARTESIAN_POINT ( 'NONE',  ( 17.68711869539999881, 1428.828027849089949, 204.9896315466789929 ) ) ;
#90440=CARTESIAN_POINT ( 'NONE',  ( 12.09917978440000041, 1426.493404676209821, 204.7338120852189718 ) ) ;
#90441=CARTESIAN_POINT ( 'NONE',  ( 0.5706190868331736388, 1498.604900413591395, 197.8127445519372429 ) ) ;
#90445=LINE ( 'NONE', #5906, #94297 ) ;
#90453=CARTESIAN_POINT ( 'NONE',  ( 10.86847934145580119, 1461.672329020349935, 210.6140132405090242 ) ) ;
#90454=CARTESIAN_POINT ( 'NONE',  ( 9.085958642259313933, 1425.096540595445731, 195.6575571040253578 ) ) ;
#90455=ADVANCED_FACE ( 'NONE', ( #78926 ), #2771, .T. ) ;
#90456=CARTESIAN_POINT ( 'NONE',  ( 1.049495711600000103, 1442.456986865990075, 218.6426261805090121 ) ) ;
#90458=B_SPLINE_CURVE_WITH_KNOTS ( 'NONE', 5,
 ( #33026, #57718, #76146, #109211, #16749, #23525 ),
 .UNSPECIFIED., .F., .F.,
 ( 6, 6 ),
 ( -2.000000000000000000, 0.000000000000000000 ),
 .UNSPECIFIED. ) ;
#90461=CARTESIAN_POINT ( 'NONE',  ( 8.332914826467142433, 1487.564149926648042, 202.1864945295145333 ) ) ;
#90469=CARTESIAN_POINT ( 'NONE',  ( 19.52205342210000083, 1473.076230373790168, 204.3554439105789982 ) ) ;
#90470=CARTESIAN_POINT ( 'NONE',  ( -16.45895393019999986, 1508.541852756190110, 213.5615360674089800 ) ) ;
#90473=CARTESIAN_POINT ( 'NONE',  ( 9.490649882959999672, 1424.812065698590004, 209.0802308740339868 ) ) ;
#90482=AXIS2_PLACEMENT_3D ( 'NONE', #72539, #49000, #89873 ) ;
#90483=CARTESIAN_POINT ( 'NONE',  ( -15.03565728386930012, 1415.677402202029953, 207.5762112621430049 ) ) ;
#90485=CARTESIAN_POINT ( 'NONE',  ( 6.048624176389999718, 1428.948518799289786, 215.4589177655589936 ) ) ;
#90487=ORIENTED_EDGE ( 'NONE', *, *, #18138, .T. ) ;
#90490=ORIENTED_EDGE ( 'NONE', *, *, #62431, .F. ) ;
#90492=CARTESIAN_POINT ( 'NONE',  ( -11.89756941249999933, 1501.968939201889953, 209.9094283132900216 ) ) ;
#90502=CARTESIAN_POINT ( 'NONE',  ( -0.1829789114686829754, 1515.156771665009956, 213.4488861885569975 ) ) ;
#90504=CARTESIAN_POINT ( 'NONE',  ( -11.39145936318320018, 1480.805290751239909, 212.2135522325029910 ) ) ;
#90508=AXIS2_PLACEMENT_3D ( 'NONE', #59051, #93172, #84768 ) ;
#90512=CARTESIAN_POINT ( 'NONE',  ( -12.25782077130000047, 1504.418297784690139, 208.6334560855260065 ) ) ;
#90513=EDGE_CURVE ( 'NONE', #75598, #73362, #110716, .T. ) ;
#90514=CARTESIAN_POINT ( 'NONE',  ( -21.45746880365630105, 1505.229108085560028, 215.8103938400879827 ) ) ;
#90516=CARTESIAN_POINT ( 'NONE',  ( -11.71397076299980000, 1489.483175994190105, 212.5377881273170146 ) ) ;
#90519=CARTESIAN_POINT ( 'NONE',  ( 4.327610416713549846, 1515.134996992909919, 209.7706221774439825 ) ) ;
#90520=CARTESIAN_POINT ( 'NONE',  ( -7.243607538500000054, 1479.647667750989967, 210.0496944616339761 ) ) ;
#90521=CARTESIAN_POINT ( 'NONE',  ( 10.02498596419820132, 1468.967489302699960, 208.7758262183099873 ) ) ;
#90522=CARTESIAN_POINT ( 'NONE',  ( -4.281982111149999604, 1457.235994440989771, 217.6311433004889864 ) ) ;
#90525=VERTEX_POINT ( 'NONE', #94447 ) ;
#90533=CARTESIAN_POINT ( 'NONE',  ( -17.64534983439791915, 1419.607322530220472, 207.0962554418724153 ) ) ;
#90557=CARTESIAN_POINT ( 'NONE',  ( 7.619397864431079803, 1439.068296834260082, 213.8493076897310061 ) ) ;
#90559=EDGE_CURVE ( 'NONE', #2539, #60200, #67260, .T. ) ;
#90568=CARTESIAN_POINT ( 'NONE',  ( -5.606087537083091377, 1484.450325178786443, 199.4839161291210416 ) ) ;
#90573=CARTESIAN_POINT ( 'NONE',  ( 11.59735442540000072, 1491.204275857490074, 206.7872505231089804 ) ) ;
#90579=ORIENTED_EDGE ( 'NONE', *, *, #34447, .T. ) ;
#90581=CARTESIAN_POINT ( 'NONE',  ( -4.504196618690000875, 1474.524975280490025, 198.6118189482990033 ) ) ;
#90585=VECTOR ( 'NONE', #94090, 1000.000000000000114 ) ;
#90588=CARTESIAN_POINT ( 'NONE',  ( 0.8033873907879990339, 1473.261709371789948, 219.3248484348989962 ) ) ;
#90595=CARTESIAN_POINT ( 'NONE',  ( -10.14352525432950003, 1472.500047657160167, 210.0566532823200134 ) ) ;
#90596=CARTESIAN_POINT ( 'NONE',  ( 10.55744888006389992, 1501.358431704350096, 204.5464156931330137 ) ) ;
#90599=EDGE_CURVE ( 'NONE', #22353, #100464, #41842, .T. ) ;
#90600=CARTESIAN_POINT ( 'NONE',  ( 10.92990887285729862, 1479.841612654799974, 208.5736869255739805 ) ) ;
#90602=CARTESIAN_POINT ( 'NONE',  ( -3.753656485510000085, 1441.439124929289846, 201.1135183436689999 ) ) ;
#90603=CARTESIAN_POINT ( 'NONE',  ( 7.443252959589999662, 1423.092343121310023, 195.6161912809990326 ) ) ;
#90604=CARTESIAN_POINT ( 'NONE',  ( 3.313501335607582643, 1397.551704408390151, 215.1871694724064810 ) ) ;
#90609=CARTESIAN_POINT ( 'NONE',  ( -4.491283723408599826, 1508.884229729929757, 206.6339223154620015 ) ) ;
#90614=ORIENTED_EDGE ( 'NONE', *, *, #18175, .F. ) ;
#90617=CARTESIAN_POINT ( 'NONE',  ( 3.301717781941579943, 1508.551704408389924, 204.2711418796440057 ) ) ;
#90620=CARTESIAN_POINT ( 'NONE',  ( 4.803826041432978755, 1471.771558818840049, 187.6888330202939983 ) ) ;
#90623=CARTESIAN_POINT ( 'NONE',  ( -2.956827888069649912, 1515.222544093250008, 204.7977243774139993 ) ) ;
#90624=CARTESIAN_POINT ( 'NONE',  ( -5.062212390315069754, 1474.342205398819942, 198.8731691453010058 ) ) ;
#90627=CARTESIAN_POINT ( 'NONE',  ( 4.270716320241006336, 1515.320037165009126, 211.4519800868023083 ) ) ;
#90634=B_SPLINE_CURVE_WITH_KNOTS ( 'NONE', 5,
 ( #13621, #82516, #108256, #73017, #30448, #56767 ),
 .UNSPECIFIED., .F., .F.,
 ( 6, 6 ),
 ( 0.000000000000000000, 1.000000000000000000 ),
 .UNSPECIFIED. ) ;
#90637=ORIENTED_EDGE ( 'NONE', *, *, #21709, .F. ) ;
#90643=CARTESIAN_POINT ( 'NONE',  ( -15.50787399150000034, 1420.315084950680102, 211.2763647146890094 ) ) ;
#90650=CARTESIAN_POINT ( 'NONE',  ( -9.189592411000269578, 1448.419325144910090, 210.4171903414359974 ) ) ;
#90651=B_SPLINE_CURVE_WITH_KNOTS ( 'NONE', 5,
 ( #97078, #98157, #20344, #71363, #55089, #55641, #21972, #28207, #104922 ),
 .UNSPECIFIED., .F., .F.,
 ( 6, 3, 6 ),
 ( 0.000000000000000000, 0.2390991004796381159, 1.000000000000000000 ),
 .UNSPECIFIED. ) ;
#90657=CARTESIAN_POINT ( 'NONE',  ( 6.992375725325399749, 1424.886399156210018, 213.2204113455599952 ) ) ;
#90658=EDGE_LOOP ( 'NONE', ( #29026, #56447, #61734, #12318 ) ) ;
#90670=CARTESIAN_POINT ( 'NONE',  ( 11.74132753969999854, 1499.920429264490167, 205.7525976432890218 ) ) ;
#90672=CARTESIAN_POINT ( 'NONE',  ( 11.33291839610000018, 1501.995980221090122, 207.2411316382289783 ) ) ;
#90680=CARTESIAN_POINT ( 'NONE',  ( -15.22835610959999997, 1415.677402202029953, 206.7258912741390020 ) ) ;
#90689=CARTESIAN_POINT ( 'NONE',  ( 10.39781522345580100, 1481.413011136829937, 214.7151440750830034 ) ) ;
#90693=CARTESIAN_POINT ( 'NONE',  ( 3.406450987864870328, 1507.508084575899829, 220.3277226881679951 ) ) ;
#90694=ADVANCED_FACE ( 'NONE', ( #13748 ), #107279, .F. ) ;
#90700=CARTESIAN_POINT ( 'NONE',  ( 1.407091184820499885, 1474.938609241890163, 220.4531082379680242 ) ) ;
#90707=CARTESIAN_POINT ( 'NONE',  ( 12.36845973521560005, 1427.047203898280031, 206.6331761361700217 ) ) ;
#90708=EDGE_CURVE ( 'NONE', #100027, #81793, #28566, .T. ) ;
#90709=CARTESIAN_POINT ( 'NONE',  ( -9.773688900458409989, 1440.083893828079908, 206.9335397354529960 ) ) ;
#90710=B_SPLINE_CURVE_WITH_KNOTS ( 'NONE', 3,
 ( #589, #9513, #87906, #11195, #18442, #68907 ),
 .UNSPECIFIED., .F., .F.,
 ( 4, 2, 4 ),
 ( 0.000000000000000000, 0.5000000000000000000, 1.000000000000000000 ),
 .UNSPECIFIED. ) ;
#90712=EDGE_LOOP ( 'NONE', ( #71751, #53000, #3766, #81990, #95613 ) ) ;
#90717=EDGE_CURVE ( 'NONE', #96418, #78070, #24363, .T. ) ;
#90719=CARTESIAN_POINT ( 'NONE',  ( 10.14664409362030106, 1422.547896506549932, 210.8756393921580070 ) ) ;
#90720=CARTESIAN_POINT ( 'NONE',  ( 11.02200761809709917, 1424.480284645659822, 203.1122766956139856 ) ) ;
#90721=VERTEX_POINT ( 'NONE', #67508 ) ;
#90722=CARTESIAN_POINT ( 'NONE',  ( 4.085147076609999317, 1428.826406437490050, 216.3215770461389980 ) ) ;
#90724=CARTESIAN_POINT ( 'NONE',  ( -16.77180262980000336, 1417.238431246169966, 208.0779775581890192 ) ) ;
#90725=CARTESIAN_POINT ( 'NONE',  ( -13.31089767776890120, 1503.456584347970193, 208.6977459380580058 ) ) ;
#90728=( BOUNDED_CURVE ( )  B_SPLINE_CURVE ( 3, ( #62727, #71115, #11728, #71683 ),
 .UNSPECIFIED., .F., .T. ) 
 B_SPLINE_CURVE_WITH_KNOTS ( ( 4, 4 ),
 ( 1.013149129984646013, 2.128443654157999632 ),
 .UNSPECIFIED. ) 
 CURVE ( )  GEOMETRIC_REPRESENTATION_ITEM ( )  RATIONAL_B_SPLINE_CURVE ( ( 1.000000000000000000, 0.8990016712204955684, 0.8990016712204955684, 1.000000000000000000 ) ) 
 REPRESENTATION_ITEM ( '' )  );
#90729=CARTESIAN_POINT ( 'NONE',  ( 8.562022419562680398, 1436.588812126380162, 208.1472598823880276 ) ) ;
#90733=CARTESIAN_POINT ( 'NONE',  ( 1.959285284397550120, 1474.800623515119923, 220.3715842348549927 ) ) ;
#90738=CARTESIAN_POINT ( 'NONE',  ( -4.922266137120000273, 1497.746000166390104, 220.5680551797990177 ) ) ;
#90740=FACE_OUTER_BOUND ( 'NONE', #70928, .T. ) ;
#90742=CARTESIAN_POINT ( 'NONE',  ( 1.491125504899999843, 1515.528285129289998, 205.0771167131389916 ) ) ;
#90743=CARTESIAN_POINT ( 'NONE',  ( 12.56817824281639950, 1426.998444030340124, 206.1059456672400074 ) ) ;
#90753=CARTESIAN_POINT ( 'NONE',  ( -4.390466737189999691, 1449.947854720489886, 190.5483265708990075 ) ) ;
#90755=CARTESIAN_POINT ( 'NONE',  ( -1.637258856660000150, 1483.893433971690001, 198.5669146070989939 ) ) ;
#90758=CARTESIAN_POINT ( 'NONE',  ( -11.59964767839999844, 1491.341587614589798, 206.7829318209490168 ) ) ;
#90763=CARTESIAN_POINT ( 'NONE',  ( 8.405796826027030377, 1426.718799454960163, 211.2874649559879856 ) ) ;
#90768=CARTESIAN_POINT ( 'NONE',  ( -4.878845441898269186, 1508.551704408389924, 205.9013857386030111 ) ) ;
#90771=CARTESIAN_POINT ( 'NONE',  ( 1.766195777250000098, 1508.139388919589919, 217.9383592619290084 ) ) ;
#90774=CARTESIAN_POINT ( 'NONE',  ( 11.27533154505640134, 1471.493970385359944, 211.0173010655499866 ) ) ;
#90775=CARTESIAN_POINT ( 'NONE',  ( 18.11996117484120106, 1430.141981561779858, 211.0753063895589889 ) ) ;
#90780=DIRECTION ( 'NONE',  ( -0.3596128954806624978, -0.9141289860956119950, -0.1872078048154584839 ) ) ;
#90781=CARTESIAN_POINT ( 'NONE',  ( -20.45337306669999933, 1467.535200901489816, 211.3000096380390005 ) ) ;
#90787=CARTESIAN_POINT ( 'NONE',  ( -1732.234191736389675, 11221.53578756870047, -1992.291823225089274 ) ) ;
#90793=ORIENTED_EDGE ( 'NONE', *, *, #100062, .F. ) ;
#90794=DIRECTION ( 'NONE',  ( -0.8907681516580484571, 1.273087901431153894E-31, 0.4544580288560254311 ) ) ;
#90804=CARTESIAN_POINT ( 'NONE',  ( 12.22918170280000005, 1500.524921488590053, 208.3556390005750245 ) ) ;
#90810=CARTESIAN_POINT ( 'NONE',  ( 12.44780704128189974, 1501.268281525590055, 211.7240718234590133 ) ) ;
#90815=CARTESIAN_POINT ( 'NONE',  ( -0.03315026662488079756, 1502.038609099889982, 233.2541149014899986 ) ) ;
#90841=CARTESIAN_POINT ( 'NONE',  ( -10.76391066127440155, 1462.897227275840123, 206.5781441640729952 ) ) ;
#90843=CARTESIAN_POINT ( 'NONE',  ( -10.16240527536719895, 1472.558926193989919, 209.8189312950259762 ) ) ;
#90858=CARTESIAN_POINT ( 'NONE',  ( 3.983717799493539324, 1515.551844914359890, 211.4517850689670126 ) ) ;
#90864=ADVANCED_FACE ( 'NONE', ( #93230 ), #85017, .F. ) ;
#90867=CARTESIAN_POINT ( 'NONE',  ( -5.750181936253229154, 1442.413653245499972, 201.3643156640750078 ) ) ;
#90872=CARTESIAN_POINT ( 'NONE',  ( -10.20774725584609932, 1481.348133439640151, 206.3586384583620088 ) ) ;
#90882=CARTESIAN_POINT ( 'NONE',  ( -0.6806208766845354141, 1463.451559807898320, 199.3558502068030407 ) ) ;
#90886=CARTESIAN_POINT ( 'NONE',  ( -5.292981110492219976, 1440.702993122236194, 202.0789376815712899 ) ) ;
#90891=CARTESIAN_POINT ( 'NONE',  ( -12.05448508470000135, 1501.734409265689919, 211.4994548164490027 ) ) ;
#90893=B_SPLINE_CURVE_WITH_KNOTS ( 'NONE', 3,
 ( #34224, #103638, #85172, #8458, #50496, #77344, #76782, #77889, #7913, #76234, #100, #102513, #68409, #26935, #16837, #42084, #101963, #110380, #60561, #647, #94122, #25250, #9020, #15735, #51039, #43193, #34778, #68964, #103066, #94681, #52148, #86281, #9567, #43737, #84073, #45948, #2853, #54365, #46510, #53257, #70619, #36427, #19621, #104739, #104190, #63321, #53822, #89030, #97440, #105855, #28583, #71737, #80643, #27472, #87961 ),
 .UNSPECIFIED., .F., .F.,
 ( 4, 2, 2, 2, 1, 1, 1, 1, 2, 2, 2, 2, 1, 1, 1, 2, 2, 2, 1, 1, 1, 1, 2, 2, 2, 2, 2, 1, 1, 1, 1, 2, 2, 2, 4 ),
 ( 0.000000000000000000, 0.1249999999999774070, 0.1874999999999732714, 0.2187499999999759637, 0.2343749999999773515, 0.2421874999999807654, 0.2460937499999825417, 0.2480468749999878431, 0.2490234374999844291, 0.2499999999999810707, 0.3125000000001457723, 0.3437500000002332023, 0.3593750000002768896, 0.3671875000002988165, 0.3710937500003113065, 0.3730468750003188005, 0.3750000000003263501, 0.4375000000002042255, 0.4687500000001482148, 0.4843750000001165734, 0.4921875000001021960, 0.4960937500000987543, 0.4980468750001019740, 0.5000000000001052491, 0.6249999999999911182, 0.6874999999999353850, 0.7187499999999140687, 0.7343749999999044098, 0.7421874999998996358, 0.7460937499999017453, 0.7480468749999027445, 0.7490234374999034106, 0.7499999999999039657, 0.8749999999999519273, 1.000000000000000000 ),
 .UNSPECIFIED. ) ;
#90894=B_SPLINE_CURVE_WITH_KNOTS ( 'NONE', 3,
 ( #41744, #84832, #110055, #41201 ),
 .UNSPECIFIED., .F., .F.,
 ( 4, 4 ),
 ( 0.000000000000000000, 1.000000000000000000 ),
 .UNSPECIFIED. ) ;
#90905=CARTESIAN_POINT ( 'NONE',  ( 1.338019250827790163, 1431.361302059610125, 218.5179660117710227 ) ) ;
#90910=CARTESIAN_POINT ( 'NONE',  ( 12.82193333132650004, 1421.326950664900096, 205.6957921146359922 ) ) ;
#90914=CARTESIAN_POINT ( 'NONE',  ( -13.59112270319939952, 1508.247351304150015, 209.6221426111970061 ) ) ;
#90915=CARTESIAN_POINT ( 'NONE',  ( -9.573053049599600683, 1423.428031588070098, 192.3355779375469865 ) ) ;
#90920=CARTESIAN_POINT ( 'NONE',  ( -4.254366313090000240, 1454.573790823890022, 200.5971711135589999 ) ) ;
#90922=CARTESIAN_POINT ( 'NONE',  ( 7.798665745000000982, 1426.844771716620244, 212.1118124881890026 ) ) ;
#90925=CARTESIAN_POINT ( 'NONE',  ( -17.29057999663249845, 1420.088377186219759, 204.6564600065449895 ) ) ;
#90942=CARTESIAN_POINT ( 'NONE',  ( -17.26926088820000160, 1417.734849473969916, 207.2874629064689884 ) ) ;
#90947=ORIENTED_EDGE ( 'NONE', *, *, #1108, .T. ) ;
#90952=CARTESIAN_POINT ( 'NONE',  ( -16.76078030769999927, 1420.494757909599912, 203.1294657649889928 ) ) ;
#90966=CARTESIAN_POINT ( 'NONE',  ( -8.681250099826490541, 1451.825605612139952, 205.8309633687780149 ) ) ;
#90980=CARTESIAN_POINT ( 'NONE',  ( 12.10943595246970084, 1492.670318175190232, 211.5635330023629876 ) ) ;
#90987=ORIENTED_EDGE ( 'NONE', *, *, #17644, .T. ) ;
#90992=FACE_OUTER_BOUND ( 'NONE', #33821, .T. ) ;
#90993=CARTESIAN_POINT ( 'NONE',  ( 11.67793025129999940, 1421.804042185309982, 204.2098866971190034 ) ) ;
#90998=CARTESIAN_POINT ( 'NONE',  ( 11.13967540296130032, 1470.272324673559979, 206.9144120771860003 ) ) ;
#91001=CARTESIAN_POINT ( 'NONE',  ( 10.46969661486759939, 1481.045827775979888, 207.7546358525030143 ) ) ;
#91006=CARTESIAN_POINT ( 'NONE',  ( 10.85999110878850082, 1461.697261943650119, 210.6766943065500186 ) ) ;
#91007=CARTESIAN_POINT ( 'NONE',  ( 8.693632405113794093, 1424.753903042060301, 195.7638379925143965 ) ) ;
#91008=CARTESIAN_POINT ( 'NONE',  ( 2.563330864020000099, 1442.944485697089931, 217.6409014154289991 ) ) ;
#91010=CARTESIAN_POINT ( 'NONE',  ( 18.18716276245509889, 1472.405785144279889, 200.2358052267980213 ) ) ;
#91013=CARTESIAN_POINT ( 'NONE',  ( 7.620481068300741789, 1487.192915415723746, 201.4288594422998244 ) ) ;
#91019=B_SPLINE_CURVE_WITH_KNOTS ( 'NONE', 5,
 ( #10961, #77203, #71463, #43046, #19889, #3135, #68814, #110784, #2584, #51435, #101812, #92874, #27749, #37267, #53532, #11514, #16690, #68269, #102377, #45689, #84480, #28309, #87672, #96060, #85565, #54095, #7768 ),
 .UNSPECIFIED., .F., .F.,
 ( 6, 3, 3, 3, 3, 3, 3, 3, 6 ),
 ( 0.000000000000000000, 0.2707461590965168363, 0.3916971170454437989, 0.4318029489778890673, 0.5054684918763174828, 0.5530467713704623200, 0.6440574843390157733, 0.7475457811094275984, 1.000000000000000000 ),
 .UNSPECIFIED. ) ;
#91023=CARTESIAN_POINT ( 'NONE',  ( 11.23532873895420181, 1470.432715234180023, 207.3851918988540035 ) ) ;
#91024=CARTESIAN_POINT ( 'NONE',  ( -5.552493783490000112, 1484.291247502590068, 199.5131655642589976 ) ) ;
#91027=CARTESIAN_POINT ( 'NONE',  ( -9.088229089533928828, 1438.332110391349943, 209.8720988501380020 ) ) ;
#91031=CARTESIAN_POINT ( 'NONE',  ( -15.11464394393560084, 1415.677402202029953, 207.9357332300280063 ) ) ;
#91032=AXIS2_PLACEMENT_3D ( 'NONE', #59810, #67665, #43554 ) ;
#91040=ORIENTED_EDGE ( 'NONE', *, *, #11516, .T. ) ;
#91041=CARTESIAN_POINT ( 'NONE',  ( -11.55195656709999952, 1501.414664579589726, 210.2508352412490069 ) ) ;
#91043=CARTESIAN_POINT ( 'NONE',  ( 2.011313522410000054, 1455.968210837190099, 218.7648719726389857 ) ) ;
#91048=CARTESIAN_POINT ( 'NONE',  ( -5.199570078000000706, 1391.913060387289988, 203.8075142969990168 ) ) ;
#91050=CARTESIAN_POINT ( 'NONE',  ( 9.659982096821350339, 1463.878250764609902, 210.8181782570380278 ) ) ;
#91052=CARTESIAN_POINT ( 'NONE',  ( -0.9184306762050470363, 1515.115092018379983, 213.4499776085069982 ) ) ;
#91058=ORIENTED_EDGE ( 'NONE', *, *, #16095, .F. ) ;
#91060=CARTESIAN_POINT ( 'NONE',  ( -11.84615870340000043, 1505.361144464890003, 208.3660837394670295 ) ) ;
#91062=ADVANCED_FACE ( 'NONE', ( #10899 ), #47509, .T. ) ;
#91063=CARTESIAN_POINT ( 'NONE',  ( -13.70067222254309947, 1504.052900633450008, 227.6557303632510241 ) ) ;
#91072=CARTESIAN_POINT ( 'NONE',  ( 6.225972109890000716, 1494.795958560490135, 219.7811165620990153 ) ) ;
#91073=CARTESIAN_POINT ( 'NONE',  ( -4.923014981580000615, 1458.312473659190118, 217.7805121944490168 ) ) ;
#91081=CARTESIAN_POINT ( 'NONE',  ( -8.828681655797659289, 1447.722821479130062, 212.1466095620490080 ) ) ;
#91088=B_SPLINE_SURFACE_WITH_KNOTS ( 'NONE', 5, 1, ( 
 ( #16362, #84140 ),
 ( #67375, #42152 ),
 ( #94191, #76303 ),
 ( #102033, #25319 ),
 ( #24760, #50561 ),
 ( #75217, #76861 ),
 ( #109368, #22143 ),
 ( #50007, #100926 ),
 ( #84687, #172 ) ),
 .UNSPECIFIED., .F., .F., .F.,
 ( 6, 3, 6 ),
 ( 2, 2 ),
 ( 0.000000000000000000, 3.733858336720000004, 7.455685587529999658 ),
 ( 0.000000000000000000, 14.00000000000000000 ),
 .UNSPECIFIED. ) ;
#91089=ORIENTED_EDGE ( 'NONE', *, *, #27586, .T. ) ;
#91095=B_SPLINE_SURFACE_WITH_KNOTS ( 'NONE', 5, 5, ( 
 ( #58688, #31264, #58140, #59249, #99556, #57600 ),
 ( #92821, #24498, #74947, #65446, #76028, #31816 ),
 ( #108524, #16092, #22840, #33449, #84959, #75499 ),
 ( #15541, #100661, #101202, #93367, #6065, #109094 ),
 ( #41872, #50830, #57046, #14994, #101758, #48644 ),
 ( #91171, #40218, #16633, #32376, #23944, #74399 ),
 ( #92272, #7171, #66004, #25046, #8253, #73840 ),
 ( #100124, #23408, #49741, #83868, #50300, #41330 ),
 ( #109633, #84427, #32907, #67099, #7713, #102314 ) ),
 .UNSPECIFIED., .F., .F., .F.,
 ( 6, 3, 6 ),
 ( 6, 6 ),
 ( 3.881604426910000072, 7.667864109139999940, 12.69765133870000007 ),
 ( 0.000000000000000000, 2.000000000000000000 ),
 .UNSPECIFIED. ) ;
#91103=EDGE_LOOP ( 'NONE', ( #13517, #66726, #72480, #49539 ) ) ;
#91109=CARTESIAN_POINT ( 'NONE',  ( 19.41157449629999832, 1457.417846740989944, 209.1218459616989946 ) ) ;
#91113=CARTESIAN_POINT ( 'NONE',  ( 6.164918445296012628, 1460.089225756436917, 201.7079981919788167 ) ) ;
#91116=DIRECTION ( 'NONE',  ( 1.224646799147350002E-16, -1.836970198721029688E-16, -1.000000000000000000 ) ) ;
#91119=VERTEX_POINT ( 'NONE', #43675 ) ;
#91121=CARTESIAN_POINT ( 'NONE',  ( -10.10379226119999885, 1472.617050353389914, 207.7708162939690055 ) ) ;
#91130=CARTESIAN_POINT ( 'NONE',  ( 7.424447884040000112, 1487.091156260190019, 201.2206016250389951 ) ) ;
#91134=DIRECTION ( 'NONE',  ( -0.9996573249755569268, 0.02617694830788839730, -1.272313417210569287E-16 ) ) ;
#91135=DIRECTION ( 'NONE',  ( 0.8750399157388792926, -0.3840929811364761082, 0.2945805962812040324 ) ) ;
#91140=DIRECTION ( 'NONE',  ( 0.9824080081115887930, -2.243614313870717968E-31, 0.1867471702549210744 ) ) ;
#91141=CARTESIAN_POINT ( 'NONE',  ( -15.86751291366650030, 1508.452568328270218, 214.6320188443539791 ) ) ;
#91142=CARTESIAN_POINT ( 'NONE',  ( 1.498519443250000194, 1473.533415296189787, 219.2408100347990114 ) ) ;
#91148=CARTESIAN_POINT ( 'NONE',  ( -0.8168837593883370163, 1455.407754195820189, 198.6297299609340143 ) ) ;
#91149=LINE ( 'NONE', #32885, #100585 ) ;
#91151=CARTESIAN_POINT ( 'NONE',  ( -9.839566507713760402, 1471.648513791290043, 211.6171294469720010 ) ) ;
#91152=CARTESIAN_POINT ( 'NONE',  ( -6.475563477829999748, 1476.191846288490069, 217.2936124755890148 ) ) ;
#91153=CARTESIAN_POINT ( 'NONE',  ( 2.782628547279999864, 1480.749758698789947, 229.4592195060989752 ) ) ;
#91159=CARTESIAN_POINT ( 'NONE',  ( -1.730029831119999972, 1444.010312626490077, 199.6239785729489995 ) ) ;
#91160=CARTESIAN_POINT ( 'NONE',  ( 11.37179842121179973, 1502.689078123959916, 211.1467236230820106 ) ) ;
#91163=CARTESIAN_POINT ( 'NONE',  ( 10.70745313423520173, 1422.293419597579941, 211.2167388469730156 ) ) ;
#91165=CARTESIAN_POINT ( 'NONE',  ( 0.9261100251351479518, 1508.551704408389924, 219.8874203466220081 ) ) ;
#91169=CARTESIAN_POINT ( 'NONE',  ( -12.68115466278469938, 1502.671228371769985, 209.0114104908589638 ) ) ;
#91171=CARTESIAN_POINT ( 'NONE',  ( -0.2871112535150010525, 1455.269628498290103, 218.5715099901590008 ) ) ;
#91176=CARTESIAN_POINT ( 'NONE',  ( 2.640559408228119853, 1508.551704408389924, 204.1382632388410059 ) ) ;
#91181=CARTESIAN_POINT ( 'NONE',  ( -4.261662194147370464, 1515.372228416580128, 206.7919396095460058 ) ) ;
#91184=CARTESIAN_POINT ( 'NONE',  ( -5.070280933269999402, 1462.534208498590033, 200.7832906722389907 ) ) ;
#91186=CARTESIAN_POINT ( 'NONE',  ( 3.712013955199999771, 1466.291930614589774, 219.5294839965989979 ) ) ;
#91193=B_SPLINE_CURVE_WITH_KNOTS ( 'NONE', 5,
 ( #93947, #51409, #75529, #16126, #17770, #51973 ),
 .UNSPECIFIED., .F., .F.,
 ( 6, 6 ),
 ( 0.000000000000000000, 1.000000000000000000 ),
 .UNSPECIFIED. ) ;
#91195=EDGE_LOOP ( 'NONE', ( #76245, #51728, #25146, #51357 ) ) ;
#91196=ADVANCED_FACE ( 'NONE', ( #1135 ), #97540, .T. ) ;
#91215=CARTESIAN_POINT ( 'NONE',  ( 7.490788429555370165, 1425.317015923290001, 212.2654107691739966 ) ) ;
#91216=ADVANCED_FACE ( 'NONE', ( #65947 ), #86745, .T. ) ;
#91219=CARTESIAN_POINT ( 'NONE',  ( -9.975542809210001138, 1421.165924026620132, 193.6282031886989898 ) ) ;
#91223=CIRCLE ( 'NONE', #84031, 4.250000000000000000 ) ;
#91225=CARTESIAN_POINT ( 'NONE',  ( -4.636950470105315247, 1378.041548212150929, 214.3403514578957925 ) ) ;
#91228=ORIENTED_EDGE ( 'NONE', *, *, #2530, .T. ) ;
#91229=CARTESIAN_POINT ( 'NONE',  ( -3.179033943583710276, 1457.997354099609993, 219.3203918230290128 ) ) ;
#91232=CARTESIAN_POINT ( 'NONE',  ( 9.772933234099999922, 1463.374803562589932, 209.6899480743859954 ) ) ;
#91246=CARTESIAN_POINT ( 'NONE',  ( -6.499023713309999728, 1427.690723050089900, 203.8816284302589850 ) ) ;
#91254=ORIENTED_EDGE ( 'NONE', *, *, #27606, .T. ) ;
#91255=DIRECTION ( 'NONE',  ( -4.110483225678505215E-05, -1.788365258186560565E-06, 0.9999999991535972743 ) ) ;
#91256=CARTESIAN_POINT ( 'NONE',  ( 7.735002320672926146, 1435.902786767089538, 205.2877876006086808 ) ) ;
#91259=CARTESIAN_POINT ( 'NONE',  ( 9.850217353651350649, 1503.174886245870084, 217.1987157647029960 ) ) ;
#91260=VECTOR ( 'NONE', #85571, 1000.000000000000000 ) ;
#91261=FACE_OUTER_BOUND ( 'NONE', #19048, .T. ) ;
#91262=CARTESIAN_POINT ( 'NONE',  ( -3.263756439183980174, 1476.410057112220102, 220.1266873629019756 ) ) ;
#91265=CARTESIAN_POINT ( 'NONE',  ( 10.16454034401940021, 1479.821216484649995, 205.9845809784859796 ) ) ;
#91269=CARTESIAN_POINT ( 'NONE',  ( 10.82434022283250030, 1423.324388501479916, 206.8207127886749959 ) ) ;
#91272=ORIENTED_EDGE ( 'NONE', *, *, #20626, .T. ) ;
#91273=CARTESIAN_POINT ( 'NONE',  ( 18.51068734469999910, 1475.362681785890118, 218.3399159096489939 ) ) ;
#91277=CARTESIAN_POINT ( 'NONE',  ( 10.31326332856479944, 1422.496447624620032, 210.6272975906319971 ) ) ;
#91278=CARTESIAN_POINT ( 'NONE',  ( 11.42162556611340030, 1422.176594433650052, 203.3886333800170121 ) ) ;
#91280=CARTESIAN_POINT ( 'NONE',  ( 1.680959541130000012, 1430.284313584789970, 217.4307392857090235 ) ) ;
#91287=CARTESIAN_POINT ( 'NONE',  ( -4.035334156310671716, 1456.652990358677243, 217.7497121191034353 ) ) ;
#91294=CARTESIAN_POINT ( 'NONE',  ( -20.49359230279999977, 1486.268284136490138, 212.0880304968289636 ) ) ;
#91298=CARTESIAN_POINT ( 'NONE',  ( 12.74682077097699917, 1426.700036781529889, 204.1990136926680179 ) ) ;
#91299=CARTESIAN_POINT ( 'NONE',  ( 18.28863234242390234, 1430.119122075690029, 201.0315569595829857 ) ) ;
#91305=AXIS2_PLACEMENT_3D ( 'NONE', #26672, #110136, #109595 ) ;
#91313=CARTESIAN_POINT ( 'NONE',  ( 9.682949316780000260, 1479.800193431990010, 204.8983903314390034 ) ) ;
#91315=CARTESIAN_POINT ( 'NONE',  ( -11.02925645290000034, 1492.700458242990180, 208.1688302671739734 ) ) ;
#91324=LINE ( 'NONE', #74542, #83707 ) ;
#91325=CARTESIAN_POINT ( 'NONE',  ( -4.714156601264419599, 1508.551704408389924, 205.4956836294300047 ) ) ;
#91329=CARTESIAN_POINT ( 'NONE',  ( 12.45662858640000081, 1427.088122356749864, 206.6493127654890145 ) ) ;
#91336=CIRCLE ( 'NONE', #43068, 4.250000000000000000 ) ;
#91342=CARTESIAN_POINT ( 'NONE',  ( -20.44684673909999617, 1467.336849514990035, 211.2727642411090017 ) ) ;
#91344=CARTESIAN_POINT ( 'NONE',  ( 12.17073519972539941, 1499.730396604210000, 205.6506567772970016 ) ) ;
#91355=ORIENTED_EDGE ( 'NONE', *, *, #3509, .F. ) ;
#91360=ORIENTED_EDGE ( 'NONE', *, *, #35240, .T. ) ;
#91362=ORIENTED_EDGE ( 'NONE', *, *, #99531, .F. ) ;
#91365=CARTESIAN_POINT ( 'NONE',  ( 1.318491153889610024, 1485.468798185310106, 220.9179226408149930 ) ) ;
#91372=CARTESIAN_POINT ( 'NONE',  ( -2.330134118790000208, 1515.551704408389924, 212.9514660756190096 ) ) ;
#91378=CARTESIAN_POINT ( 'NONE',  ( 9.992001554820001630, 1491.422527302990147, 188.4943246008990059 ) ) ;
#91384=VECTOR ( 'NONE', #7701, 1000.000000000000000 ) ;
#91385=CARTESIAN_POINT ( 'NONE',  ( 12.52351530970569904, 1500.052013425719906, 207.1430829055039737 ) ) ;
#91386=CARTESIAN_POINT ( 'NONE',  ( -19.39503999260000100, 1507.708763760590045, 209.4440057405769835 ) ) ;
#91389=CARTESIAN_POINT ( 'NONE',  ( 3.970164549720000213, 1515.569681836989957, 210.2459363763389888 ) ) ;
#91392=CARTESIAN_POINT ( 'NONE',  ( -15.74179306318853833, 1484.201616316254785, 223.2977079293126224 ) ) ;
#91400=VERTEX_POINT ( 'NONE', #42849 ) ;
#91407=CARTESIAN_POINT ( 'NONE',  ( -4.082703448014748382, 1515.071394417499505, 212.7081850046428713 ) ) ;
#91409=CARTESIAN_POINT ( 'NONE',  ( -5.615127104817688952, 1507.508085020990166, 198.8434247404759958 ) ) ;
#91416=CARTESIAN_POINT ( 'NONE',  ( 20.13561634019999858, 1473.995504141989841, 210.1093940072919963 ) ) ;
#91420=B_SPLINE_CURVE_WITH_KNOTS ( 'NONE', 3,
 ( #59246, #93365, #50828, #3214, #18305, #11588, #96703, #96135, #60909, #78229, #19974, #62015, #1542, #107152, #38838, #78791 ),
 .UNSPECIFIED., .F., .F.,
 ( 4, 2, 1, 1, 2, 2, 2, 2, 4 ),
 ( 0.000000000000000000, 0.2500000000001725287, 0.3750000000000902056, 0.4375000000000508482, 0.4687499999998230860, 0.4999999999995953792, 0.6249999999999499289, 0.7500000000003045342, 1.000000000000000000 ),
 .UNSPECIFIED. ) ;
#91427=CARTESIAN_POINT ( 'NONE',  ( -11.63277241116059990, 1501.279596332750089, 211.2803251540719884 ) ) ;
#91433=CARTESIAN_POINT ( 'NONE',  ( -4.881006452805260132, 1440.913765093959910, 201.7555229531890291 ) ) ;
#91444=CARTESIAN_POINT ( 'NONE',  ( 10.95543255003150129, 1490.155657787360042, 208.9951350640439784 ) ) ;
#91447=CARTESIAN_POINT ( 'NONE',  ( 9.788553136239070085, 1435.243871060430138, 208.4607419252359932 ) ) ;
#91448=VECTOR ( 'NONE', #68994, 1000.000000000000114 ) ;
#91449=CARTESIAN_POINT ( 'NONE',  ( -8.881784197000000993E-16, 1392.213060387289943, 209.1218459616989946 ) ) ;
#91453=CARTESIAN_POINT ( 'NONE',  ( -2.034008778210000035, 1508.605352629489971, 220.7050406583989854 ) ) ;
#91454=CARTESIAN_POINT ( 'NONE',  ( -11.62426067770000060, 1501.026510252989965, 213.4445963220190094 ) ) ;
#91461=CARTESIAN_POINT ( 'NONE',  ( -8.377805553860001808, 1439.624828044090009, 206.1458839272790158 ) ) ;
#91465=CARTESIAN_POINT ( 'NONE',  ( 12.04503635791889948, 1491.368323112810003, 206.7127955739260017 ) ) ;
#91470=CARTESIAN_POINT ( 'NONE',  ( 12.91552263953340152, 1421.111598984989996, 204.2664607796000098 ) ) ;
#91472=ADVANCED_FACE ( 'NONE', ( #68615 ), #106489, .T. ) ;
#91476=CARTESIAN_POINT ( 'NONE',  ( -13.32685111460899918, 1469.522659984069833, 191.9925937506160096 ) ) ;
#91481=CARTESIAN_POINT ( 'NONE',  ( -5.104341685840000586, 1454.049460953489870, 201.0800892362090053 ) ) ;
#91483=CARTESIAN_POINT ( 'NONE',  ( 7.925563889120000205, 1426.364738259879914, 211.7377644087189879 ) ) ;
#91486=CARTESIAN_POINT ( 'NONE',  ( -21.69813442400969805, 1417.904383893920112, 208.5544938348409687 ) ) ;
#91494=EDGE_CURVE ( 'NONE', #2433, #69308, #105516, .T. ) ;
#91500=CARTESIAN_POINT ( 'NONE',  ( -15.20906659412241702, 1416.167321952329530, 211.8455853713288946 ) ) ;
#91501=CARTESIAN_POINT ( 'NONE',  ( 2.175596292269999843, 1445.361571848690119, 200.0046556085490010 ) ) ;
#91504=CARTESIAN_POINT ( 'NONE',  ( -5.534144808426719742, 1464.371868907480120, 199.5915608675260273 ) ) ;
#91506=CARTESIAN_POINT ( 'NONE',  ( -17.35635886029999853, 1417.798318063129955, 207.1516956251389843 ) ) ;
#91521=ORIENTED_EDGE ( 'NONE', *, *, #49492, .F. ) ;
#91522=CARTESIAN_POINT ( 'NONE',  ( -11.41402558200000072, 1500.969830860790125, 208.5831166258960252 ) ) ;
#91538=CARTESIAN_POINT ( 'NONE',  ( 20.58082067220000155, 1494.260204254890141, 204.7904675245989665 ) ) ;
#91544=CARTESIAN_POINT ( 'NONE',  ( -1.349081561059999990, 1443.127676870989944, 219.0403161255090083 ) ) ;
#91559=CARTESIAN_POINT ( 'NONE',  ( 11.67048048849999908, 1421.742781192700249, 203.8252195604689803 ) ) ;
#91563=CARTESIAN_POINT ( 'NONE',  ( 0.8871466948159980603, 1460.711025077289833, 228.7960624615990071 ) ) ;
#91564=CARTESIAN_POINT ( 'NONE',  ( 10.04184886183580083, 1469.459372728499829, 207.3535612217320079 ) ) ;
#91568=VECTOR ( 'NONE', #56593, 1000.000000000000227 ) ;
#91571=( BOUNDED_CURVE ( )  B_SPLINE_CURVE ( 3, ( #33859, #85353, #110574, #102696 ),
 .UNSPECIFIED., .F., .F. ) 
 B_SPLINE_CURVE_WITH_KNOTS ( ( 4, 4 ),
 ( 1.083108237977496113, 1.126222521644246077 ),
 .UNSPECIFIED. ) 
 CURVE ( )  GEOMETRIC_REPRESENTATION_ITEM ( )  RATIONAL_B_SPLINE_CURVE ( ( 1.000000000000000000, 0.9998451025440023843, 0.9998451025440023843, 1.000000000000000000 ) ) 
 REPRESENTATION_ITEM ( '' )  );
#91572=CARTESIAN_POINT ( 'NONE',  ( -12.78943302956389871, 1502.708798875820094, 209.0180534851929792 ) ) ;
#91573=CARTESIAN_POINT ( 'NONE',  ( 8.380001589455886801, 1424.398767409684297, 195.8291005401241591 ) ) ;
#91590=CARTESIAN_POINT ( 'NONE',  ( -9.956881614119650337, 1438.965782279799896, 209.6194444277939795 ) ) ;
#91591=CARTESIAN_POINT ( 'NONE',  ( -4.077241479695540960, 1515.224507089990084, 212.7046478782430086 ) ) ;
#91606=CARTESIAN_POINT ( 'NONE',  ( -6.344682030749999591, 1447.083671391689904, 215.8265176690789815 ) ) ;
#91612=CARTESIAN_POINT ( 'NONE',  ( -4.378216884482949212, 1453.707746088449994, 199.6107954155660025 ) ) ;
#91617=ORIENTED_EDGE ( 'NONE', *, *, #77428, .F. ) ;
#91618=VERTEX_POINT ( 'NONE', #20378 ) ;
#91621=CARTESIAN_POINT ( 'NONE',  ( -13.58959795930000070, 1505.039793835389901, 227.7961552795990201 ) ) ;
#91623=CARTESIAN_POINT ( 'NONE',  ( -2.876354336597070294, 1474.536642632726171, 218.9936859356158152 ) ) ;
#91625=LINE ( 'NONE', #55296, #34032 ) ;
#91630=CARTESIAN_POINT ( 'NONE',  ( -3.084096054229999773, 1457.182013962589963, 218.2582502859689839 ) ) ;
#91634=CARTESIAN_POINT ( 'NONE',  ( -4.329358020582379396, 1515.068258693859889, 210.7645756910659998 ) ) ;
#91638=CARTESIAN_POINT ( 'NONE',  ( -8.582505635693420842, 1448.408617315599940, 212.2769557201809789 ) ) ;
#91645=ORIENTED_EDGE ( 'NONE', *, *, #57841, .T. ) ;
#91659=CARTESIAN_POINT ( 'NONE',  ( 10.91833819165210073, 1460.842557474800060, 208.3727220096430131 ) ) ;
#91663=CARTESIAN_POINT ( 'NONE',  ( 3.062858194097104914, 1458.818553845532279, 199.9951087153910976 ) ) ;
#91665=CARTESIAN_POINT ( 'NONE',  ( 8.472423600081759432, 1438.684924725989958, 211.2764949506089920 ) ) ;
#91671=CARTESIAN_POINT ( 'NONE',  ( -9.522283751578990874, 1439.330121708799879, 208.4248680932010132 ) ) ;
#91680=CARTESIAN_POINT ( 'NONE',  ( 6.289965333610000542, 1487.835111632490225, 199.7689564727890001 ) ) ;
#91687=CARTESIAN_POINT ( 'NONE',  ( -17.28245522079999930, 1417.580815317299994, 206.4386048391490078 ) ) ;
#91689=CARTESIAN_POINT ( 'NONE',  ( -16.33552025180029688, 1508.551704408389924, 213.4320397940620069 ) ) ;
#91690=CARTESIAN_POINT ( 'NONE',  ( -16.32932620218339892, 1508.453868990269939, 214.1093932417330166 ) ) ;
#91692=CARTESIAN_POINT ( 'NONE',  ( -3.028748347090000070, 1475.522729171590072, 219.1245829792990207 ) ) ;
#91693=CARTESIAN_POINT ( 'NONE',  ( -20.86254339170000094, 1504.682062816289999, 214.2159060785090219 ) ) ;
#91698=EDGE_CURVE ( 'NONE', #77826, #5707, #108808, .T. ) ;
#91699=CARTESIAN_POINT ( 'NONE',  ( -0.9914680223604751541, 1455.336337171600235, 198.6483182256660029 ) ) ;
#91703=CARTESIAN_POINT ( 'NONE',  ( -10.08495433981949851, 1472.385695682990217, 210.5310355009019929 ) ) ;
#91704=CARTESIAN_POINT ( 'NONE',  ( 4.327511837212730583, 1515.138761592180117, 208.5315405873499799 ) ) ;
#91708=CARTESIAN_POINT ( 'NONE',  ( 10.68372146313839899, 1480.504181365129853, 209.2647601501510053 ) ) ;
#91711=CARTESIAN_POINT ( 'NONE',  ( 8.890886715069999724, 1425.078558200960060, 195.7078080160990226 ) ) ;
#91712=CARTESIAN_POINT ( 'NONE',  ( -230.7985005798999794, 11216.44053380570040, 2175.332171792929785 ) ) ;
#91718=CARTESIAN_POINT ( 'NONE',  ( -11.77312369862629993, 1501.973685400810155, 208.8494367388649948 ) ) ;
#91719=CARTESIAN_POINT ( 'NONE',  ( 10.58757398251879955, 1491.532463854900016, 212.1720164327929865 ) ) ;
#91724=CARTESIAN_POINT ( 'NONE',  ( -2.762666289370000250, 1431.313464822989999, 217.0512884656089909 ) ) ;
#91732=CARTESIAN_POINT ( 'NONE',  ( -8.170216832330000400, 1462.724072430790102, 203.3866392159690122 ) ) ;
#91734=CARTESIAN_POINT ( 'NONE',  ( 3.235048515759559873, 1466.472015849239824, 219.6884157167970102 ) ) ;
#91735=CARTESIAN_POINT ( 'NONE',  ( -13.54908436191989907, 1508.551704408389924, 216.1707514617089885 ) ) ;
#91739=CARTESIAN_POINT ( 'NONE',  ( 3.097291077214380017, 1433.546567555699994, 201.1395984631290048 ) ) ;
#91741=DIRECTION ( 'NONE',  ( -1.000000000000000000, 0.000000000000000000, 0.000000000000000000 ) ) ;
#91747=CARTESIAN_POINT ( 'NONE',  ( -1.842962231260000028, 1515.551704408389924, 212.9514660752490158 ) ) ;
#91750=CARTESIAN_POINT ( 'NONE',  ( -4.390466737189999691, 1449.947854720489886, 190.5483265708990075 ) ) ;
#91755=CARTESIAN_POINT ( 'NONE',  ( -7.845640617949999118, 1425.340740689890026, 205.7634566372090319 ) ) ;
#91760=CARTESIAN_POINT ( 'NONE',  ( 7.126030816970708948, 1424.920809236449941, 212.9863649234119976 ) ) ;
#91775=CARTESIAN_POINT ( 'NONE',  ( 10.44621597880000152, 1461.871091769490022, 210.5497379424390090 ) ) ;
#91776=ORIENTED_EDGE ( 'NONE', *, *, #703, .F. ) ;
#91780=EDGE_CURVE ( 'NONE', #59183, #1876, #48631, .T. ) ;
#91789=B_SPLINE_CURVE_WITH_KNOTS ( 'NONE', 3,
 ( #29819, #44439, #78582, #45004, #73497, #74593, #30366, #108729, #13547, #91385, #47732, #98674, #48293, #82976, #49387, #55604, #107631, #56129, #82436 ),
 .UNSPECIFIED., .F., .F.,
 ( 4, 3, 3, 3, 3, 3, 4 ),
 ( -7.762943616236829492, -7.540944356910980417, -6.384229433512970786, -5.472533626251030014, -4.715605178811290266, -3.910860172016169756, -3.182123501529999565 ),
 .UNSPECIFIED. ) ;
#91793=ORIENTED_EDGE ( 'NONE', *, *, #85923, .F. ) ;
#91794=CARTESIAN_POINT ( 'NONE',  ( 6.201377858498039686, 1483.628135010170126, 219.2029351982129981 ) ) ;
#91796=CARTESIAN_POINT ( 'NONE',  ( 5.405194353942709640, 1478.857543658343957, 200.1157415609600321 ) ) ;
#91798=CARTESIAN_POINT ( 'NONE',  ( -10.51062080119100095, 1480.296605995150003, 210.9546507189759836 ) ) ;
#91799=CARTESIAN_POINT ( 'NONE',  ( 5.482251411591255064, 1434.591294175683743, 202.5885199238377368 ) ) ;
#91801=CARTESIAN_POINT ( 'NONE',  ( 9.661401783296120982, 1503.269051499499938, 217.4307197796210005 ) ) ;
#91803=CARTESIAN_POINT ( 'NONE',  ( 7.374483138519999592, 1422.905762710230192, 195.5806561682990150 ) ) ;
#91805=CARTESIAN_POINT ( 'NONE',  ( -10.88362670706469970, 1492.306448310009955, 203.4235623022770199 ) ) ;
#91806=CARTESIAN_POINT ( 'NONE',  ( 10.60329135936409983, 1479.127526841280087, 205.9829681192889836 ) ) ;
#91810=CARTESIAN_POINT ( 'NONE',  ( 10.66776494137399922, 1424.286284822849893, 206.6302607443430190 ) ) ;
#91822=CARTESIAN_POINT ( 'NONE',  ( 11.36942005508340081, 1422.263558134510049, 203.3812548922369956 ) ) ;
#91824=CARTESIAN_POINT ( 'NONE',  ( -11.01419074117260166, 1462.544645942729858, 208.2905843779830093 ) ) ;
#91825=DIRECTION ( 'NONE',  ( 8.881784197000000007E-16, -1.000000000000000000, 1.836970198721029688E-16 ) ) ;
#91826=CARTESIAN_POINT ( 'NONE',  ( -8.097663848092500061, 1477.149761026620126, 215.6266069428237699 ) ) ;
#91833=CARTESIAN_POINT ( 'NONE',  ( 6.558237873239729510, 1465.446384999080010, 217.0856503752089850 ) ) ;
#91836=B_SPLINE_CURVE_WITH_KNOTS ( 'NONE', 3,
 ( #26984, #61173, #94726, #85213, #102008, #18004, #95288, #25846, #34268, #84663, #52197, #69007, #690, #86326, #110427, #58934, #68450, #93066, #1238, #85771, #60048, #35375, #103111, #25292, #43781 ),
 .UNSPECIFIED., .F., .F.,
 ( 4, 3, 3, 3, 3, 3, 3, 3, 4 ),
 ( -7.276689993590000682, -7.237684796489060268, -6.557067735913999940, -5.837445478237999197, -5.133895891482029405, -5.098374790361580366, -4.440006559831749300, -3.663150781442820136, -2.991101461899999592 ),
 .UNSPECIFIED. ) ;
#91837=DIRECTION ( 'NONE',  ( 0.9066646370135239552, -0.3866611060802799260, -0.1686784664203160033 ) ) ;
#91844=DIRECTION ( 'NONE',  ( -0.2767035999362660315, -0.4514656066772200216, 0.8483006093183480534 ) ) ;
#91850=ORIENTED_EDGE ( 'NONE', *, *, #80218, .T. ) ;
#91857=B_SPLINE_SURFACE_WITH_KNOTS ( 'NONE', 5, 5, ( 
 ( #62568, #96688, #102844, #60327, #51926, #86068 ),
 ( #43528, #983, #35108, #26701, #71525, #55805 ),
 ( #37329, #4286, #3751, #89922, #13196, #81508 ),
 ( #72589, #88830, #64199, #98321, #28930, #46852 ),
 ( #46307, #56338, #30572, #22139, #38414, #37882 ),
 ( #12672, #80980, #21044, #97221, #47386, #29461 ),
 ( #105645, #4810, #21600, #38956, #73705, #63121 ),
 ( #64762, #73135, #5371, #47930, #12115, #80436 ),
 ( #106718, #39530, #72066, #90470, #13746, #30008 ) ),
 .UNSPECIFIED., .F., .F., .F.,
 ( 6, 3, 6 ),
 ( 6, 6 ),
 ( 62.33963421229999824, 67.09990280889999781, 77.98062232429998630 ),
 ( 0.000000000000000000, 1.000000000000000000 ),
 .UNSPECIFIED. ) ;
#91859=CARTESIAN_POINT ( 'NONE',  ( 10.46072157490000087, 1479.162298522890069, 206.0231600751390033 ) ) ;
#91861=CARTESIAN_POINT ( 'NONE',  ( -12.23489726360000063, 1490.237666927790087, 209.6382998835400144 ) ) ;
#91864=CARTESIAN_POINT ( 'NONE',  ( 3.083943351259999854, 1469.624425254990001, 189.3818552890990077 ) ) ;
#91866=CARTESIAN_POINT ( 'NONE',  ( -16.81641964920000021, 1417.207246461349996, 207.8736676468290057 ) ) ;
#91871=CARTESIAN_POINT ( 'NONE',  ( 10.05007022209490053, 1424.553937115210147, 207.8952550960959798 ) ) ;
#91878=CARTESIAN_POINT ( 'NONE',  ( 4.527727924400000603, 1473.939356039790027, 219.1579490833989894 ) ) ;
#91879=CARTESIAN_POINT ( 'NONE',  ( 10.51038035267259829, 1471.685921060520059, 212.2896990852769932 ) ) ;
#91890=CARTESIAN_POINT ( 'NONE',  ( -9.498196251736658269, 1449.159077731892467, 207.4992946632423241 ) ) ;
#91897=EDGE_LOOP ( 'NONE', ( #7022, #83837, #10548, #2981 ) ) ;
#91900=CARTESIAN_POINT ( 'NONE',  ( -2.423738817658458888, 1456.568741658530826, 199.9484635142324578 ) ) ;
#91901=CARTESIAN_POINT ( 'NONE',  ( 11.53251555600000167, 1501.193729600089910, 207.9797876773089911 ) ) ;
#91906=( BOUNDED_CURVE ( )  B_SPLINE_CURVE ( 3, ( #57680, #47604, #48165, #72813 ),
 .UNSPECIFIED., .F., .F. ) 
 B_SPLINE_CURVE_WITH_KNOTS ( ( 4, 4 ),
 ( 4.170645138360129955, 5.254132885623210569 ),
 .UNSPECIFIED. ) 
 CURVE ( )  GEOMETRIC_REPRESENTATION_ITEM ( )  RATIONAL_B_SPLINE_CURVE ( ( 1.000000000000000000, 0.9045405262885497510, 0.9045405262885497510, 1.000000000000000000 ) ) 
 REPRESENTATION_ITEM ( '' )  );
#91909=CARTESIAN_POINT ( 'NONE',  ( 11.26937486967429969, 1478.652699849539886, 205.8601904136019982 ) ) ;
#91910=CARTESIAN_POINT ( 'NONE',  ( 12.61287423918429873, 1500.964026500809950, 210.7122643477439965 ) ) ;
#91926=CARTESIAN_POINT ( 'NONE',  ( 3.028596170552124711, 1468.380354110695180, 218.6645797360170889 ) ) ;
#91943=CARTESIAN_POINT ( 'NONE',  ( 6.177825127070350142, 1429.592228316399996, 216.3189436702849946 ) ) ;
#91944=CARTESIAN_POINT ( 'NONE',  ( -17.12577710671219933, 1420.218837620449904, 204.3128004817139924 ) ) ;
#91948=CARTESIAN_POINT ( 'NONE',  ( 10.81671648281710141, 1470.126838882340053, 207.0136797372550177 ) ) ;
#91953=CARTESIAN_POINT ( 'NONE',  ( 2.487935150835943077, 1508.884207226184117, 213.6131390771874692 ) ) ;
#91971=CARTESIAN_POINT ( 'NONE',  ( -6.879245333380899829, 1439.807514724469911, 203.6160362513539894 ) ) ;
#91973=CARTESIAN_POINT ( 'NONE',  ( 7.805005982189999969, 1501.592229086989846, 206.4628694365890169 ) ) ;
#91977=CARTESIAN_POINT ( 'NONE',  ( -10.06498070994410021, 1481.481372748229887, 205.8729891504069940 ) ) ;
#91986=CARTESIAN_POINT ( 'NONE',  ( 2.837607610297419924, 1454.387933475150021, 218.0768438231829975 ) ) ;
#91989=CARTESIAN_POINT ( 'NONE',  ( -9.447779140010000631, 1460.630169784690224, 214.7547266466890221 ) ) ;
#91993=CARTESIAN_POINT ( 'NONE',  ( -4.261736558349999981, 1515.372048625790057, 210.9648096574089777 ) ) ;
#91994=CARTESIAN_POINT ( 'NONE',  ( -5.411583886059999848, 1438.069580177289936, 208.0725929255889923 ) ) ;
#92007=CARTESIAN_POINT ( 'NONE',  ( -9.771541787747370478, 1462.553260899800080, 206.2413424840439973 ) ) ;
#92020=B_SPLINE_SURFACE_WITH_KNOTS ( 'NONE', 5, 1, ( 
 ( #16572, #102262 ),
 ( #33395, #940 ),
 ( #24988, #103354 ),
 ( #25542, #396 ),
 ( #69246, #50769 ),
 ( #9322, #67590 ) ),
 .UNSPECIFIED., .F., .F., .F.,
 ( 6, 6 ),
 ( 2, 2 ),
 ( 0.000000000000000000, 3.604516979870000082 ),
 ( 0.000000000000000000, 14.00000000000000000 ),
 .UNSPECIFIED. ) ;
#92022=CARTESIAN_POINT ( 'NONE',  ( -19.86527982506180479, 1442.216701827569977, 212.8358345280389869 ) ) ;
#92023=CARTESIAN_POINT ( 'NONE',  ( -13.59015224396020116, 1508.309004612710169, 209.6873486301020080 ) ) ;
#92024=CARTESIAN_POINT ( 'NONE',  ( -18.32377786701850297, 1464.077817828640036, 217.4721512911559955 ) ) ;
#92026=CARTESIAN_POINT ( 'NONE',  ( -2.487935060306839752, 1508.611350403544293, 204.4436907971870312 ) ) ;
#92029=CARTESIAN_POINT ( 'NONE',  ( -8.716383294119999903, 1450.962816624490188, 203.1307156043189934 ) ) ;
#92034=CARTESIAN_POINT ( 'NONE',  ( -21.51775564986490252, 1417.978020122130147, 208.5749635269120006 ) ) ;
#92039=EDGE_LOOP ( 'NONE', ( #11797, #102244, #33418, #20129, #24306 ) ) ;
#92047=CARTESIAN_POINT ( 'NONE',  ( 2.895368129540000002, 1444.422959043590026, 200.6322053094490059 ) ) ;
#92057=ORIENTED_EDGE ( 'NONE', *, *, #29551, .F. ) ;
#92066=CARTESIAN_POINT ( 'NONE',  ( -6.907011062519999633, 1472.523400736590020, 209.7330543039639963 ) ) ;
#92068=CARTESIAN_POINT ( 'NONE',  ( -11.60945018750000024, 1501.942143215190072, 208.6602335187679671 ) ) ;
#92075=CARTESIAN_POINT ( 'NONE',  ( -8.826855412864000883, 1451.573000863549851, 206.2801294249610180 ) ) ;
#92089=CARTESIAN_POINT ( 'NONE',  ( 12.32478205772809865, 1492.212416795640138, 209.6735840658209895 ) ) ;
#92093=CARTESIAN_POINT ( 'NONE',  ( -17.39681893400159041, 1503.136625852793486, 222.8800851632994693 ) ) ;
#92109=DIRECTION ( 'NONE',  ( 1.000000000000000000, 2.249639673992789970E-32, 1.224646799147350002E-16 ) ) ;
#92116=VECTOR ( 'NONE', #1729, 1000.000000000000227 ) ;
#92118=CARTESIAN_POINT ( 'NONE',  ( 10.93592733551849960, 1461.398175533179938, 209.9040846029700162 ) ) ;
#92119=DIRECTION ( 'NONE',  ( -0.1867471702549219348, 2.391457216852619248E-16, 0.9824080081115885710 ) ) ;
#92120=CARTESIAN_POINT ( 'NONE',  ( 4.487574688360000508, 1465.989648107290122, 219.2141235446990208 ) ) ;
#92131=ORIENTED_EDGE ( 'NONE', *, *, #7641, .F. ) ;
#92140=CARTESIAN_POINT ( 'NONE',  ( -9.441857781927620152, 1438.488253401759948, 210.2256333341519792 ) ) ;
#92141=CARTESIAN_POINT ( 'NONE',  ( -3.368596972435520254, 1515.551842520359969, 212.9003872916790101 ) ) ;
#92145=CARTESIAN_POINT ( 'NONE',  ( -5.476857725019999457, 1435.904609370590151, 210.5194640658390028 ) ) ;
#92146=EDGE_CURVE ( 'NONE', #103948, #53297, #67246, .T. ) ;
#92152=ORIENTED_EDGE ( 'NONE', *, *, #18790, .F. ) ;
#92154=CARTESIAN_POINT ( 'NONE',  ( 19.41157449629999832, 1457.417846740989944, 209.1218459616989946 ) ) ;
#92155=CARTESIAN_POINT ( 'NONE',  ( 2.702615377909999950, 1455.790727295790020, 218.5929249907289886 ) ) ;
#92157=CARTESIAN_POINT ( 'NONE',  ( -2.874710529609999732, 1443.868727023889960, 218.3772876226990149 ) ) ;
#92160=CARTESIAN_POINT ( 'NONE',  ( 9.604328208296740499, 1464.024737802830032, 211.1412599434549691 ) ) ;
#92161=CARTESIAN_POINT ( 'NONE',  ( 6.808211076640000137, 1424.384911292389916, 213.4787420407489833 ) ) ;
#92165=B_SPLINE_CURVE_WITH_KNOTS ( 'NONE', 3,
 ( #30787, #72270, #12884, #108041, #91794, #23488, #15070, #89593, #81730, #5038, #82302, #63872, #56561, #4503, #97987, #82844, #21254, #38637, #106945, #90133, #55465, #30230, #73357, #56009, #22916, #64967, #39183, #64420, #90689, #49267, #100203, #38094, #65522, #106404, #5601, #39750, #98542, #21809, #6135, #73913, #31337, #99629, #13416 ),
 .UNSPECIFIED., .F., .F.,
 ( 4, 3, 3, 3, 3, 3, 3, 3, 3, 3, 3, 3, 3, 3, 4 ),
 ( 1.211046054640000118E-15, 1.449501323476880099, 2.863878615477850165, 4.272680454590320309, 5.675359640844769515, 7.071450696628339472, 8.457216201530728839, 9.836649899322781110, 11.20677902970780160, 11.59601058781499994, 12.87235518899669984, 14.20837703717869971, 15.54023549398300119, 16.81434485064450257, 17.59284132270000001 ),
 .UNSPECIFIED. ) ;
#92174=CARTESIAN_POINT ( 'NONE',  ( 13.94277550940000054, 1500.493050397790057, 227.7144758862989988 ) ) ;
#92181=CARTESIAN_POINT ( 'NONE',  ( 18.28301776585879779, 1431.668727188719913, 208.6526615892310019 ) ) ;
#92191=CARTESIAN_POINT ( 'NONE',  ( 7.107370174153629705, 1424.720561740850144, 194.0450910679149956 ) ) ;
#92210=CARTESIAN_POINT ( 'NONE',  ( 3.365542939320150140, 1426.305845304849754, 191.3806609882720124 ) ) ;
#92214=CARTESIAN_POINT ( 'NONE',  ( 6.459044766406664806, 1460.224289355106748, 201.9543198508955584 ) ) ;
#92216=CARTESIAN_POINT ( 'NONE',  ( 5.859507211404899607, 1440.154374017829923, 216.2888686505930025 ) ) ;
#92217=CARTESIAN_POINT ( 'NONE',  ( 3.829620113550000315, 1515.551704408389924, 211.2083941403789993 ) ) ;
#92222=CARTESIAN_POINT ( 'NONE',  ( -10.46967383089999970, 1471.722673347089767, 207.5079226880490069 ) ) ;
#92225=CARTESIAN_POINT ( 'NONE',  ( 7.287315400159999790, 1481.177127506090073, 208.3645142728410065 ) ) ;
#92228=CARTESIAN_POINT ( 'NONE',  ( -17.68146714750000115, 1417.155949729040003, 208.4269447418569996 ) ) ;
#92230=CARTESIAN_POINT ( 'NONE',  ( 4.765390666840000122, 1487.224757102889726, 198.9594462837989965 ) ) ;
#92244=CARTESIAN_POINT ( 'NONE',  ( 0.3242204524379989627, 1473.869303647089964, 219.3860063639990017 ) ) ;
#92247=CARTESIAN_POINT ( 'NONE',  ( -11.19405031572889975, 1471.333863838639900, 206.8852767382200284 ) ) ;
#92248=CARTESIAN_POINT ( 'NONE',  ( -6.390565317395836331, 1508.334948605542195, 219.9846009609073860 ) ) ;
#92250=CARTESIAN_POINT ( 'NONE',  ( 1.665775206630939920, 1456.320421830250098, 198.6701496495810204 ) ) ;
#92254=CARTESIAN_POINT ( 'NONE',  ( -10.52544773458219929, 1471.060235731149987, 210.0669986522439956 ) ) ;
#92255=CARTESIAN_POINT ( 'NONE',  ( 4.327620191588789744, 1515.134623705510194, 208.4650689536229891 ) ) ;
#92256=CARTESIAN_POINT ( 'NONE',  ( -5.100957845159999948, 1482.122785942490054, 228.9672709512990139 ) ) ;
#92260=CARTESIAN_POINT ( 'NONE',  ( -13.59512407998240135, 1507.703338069740084, 209.3532897553030239 ) ) ;
#92261=CARTESIAN_POINT ( 'NONE',  ( 11.50463699793380101, 1502.210269078540250, 211.3057782935299826 ) ) ;
#92262=CARTESIAN_POINT ( 'NONE',  ( 1970.639179128770138, -8387.357407334289746, 416.8689628978009978 ) ) ;
#92266=CARTESIAN_POINT ( 'NONE',  ( -3.829620113550000315, 1515.551704408389924, 207.2788837304390199 ) ) ;
#92271=CARTESIAN_POINT ( 'NONE',  ( 10.84203907937230049, 1491.933390519110162, 211.8638197534569940 ) ) ;
#92272=CARTESIAN_POINT ( 'NONE',  ( 0.2489532241669990265, 1455.106714014390036, 218.5657548107290040 ) ) ;
#92276=CARTESIAN_POINT ( 'NONE',  ( 8.360512069408569502, 1436.611072127150010, 207.0360533130520082 ) ) ;
#92278=VERTEX_POINT ( 'NONE', #77833 ) ;
#92279=CARTESIAN_POINT ( 'NONE',  ( -21.50574124000000253, 1505.376505907290039, 210.1536426368190007 ) ) ;
#92282=CARTESIAN_POINT ( 'NONE',  ( -5.890030312369999521, 1462.819977020890065, 201.3180516141489704 ) ) ;
#92287=CARTESIAN_POINT ( 'NONE',  ( 4.781276783620000081, 1452.020048942890071, 190.5513815401990030 ) ) ;
#92290=CARTESIAN_POINT ( 'NONE',  ( 3.771470575086420141, 1431.990137918330220, 200.6994607577710212 ) ) ;
#92296=DIRECTION ( 'NONE',  ( -1.000000000000000000, 0.000000000000000000, 0.000000000000000000 ) ) ;
#92299=CARTESIAN_POINT ( 'NONE',  ( -0.6907574904219989653, 1475.844123532889853, 198.0538682590990049 ) ) ;
#92304=CARTESIAN_POINT ( 'NONE',  ( 3.787233628934549845, 1428.472671622899952, 216.4667291094249890 ) ) ;
#92305=CARTESIAN_POINT ( 'NONE',  ( -8.046515503210001086, 1425.053020564090048, 207.2502090198989890 ) ) ;
#92309=CARTESIAN_POINT ( 'NONE',  ( 7.335500683392449872, 1425.052454098660064, 212.5855600729070147 ) ) ;
#92324=CARTESIAN_POINT ( 'NONE',  ( 9.835001303689999474, 1462.581801261389955, 210.2517437191489762 ) ) ;
#92342=CARTESIAN_POINT ( 'NONE',  ( 0.03085303418417100277, 1444.874163974749990, 199.0604885470160070 ) ) ;
#92345=CARTESIAN_POINT ( 'NONE',  ( -10.59763471844589944, 1480.490663172710128, 210.4673335203119962 ) ) ;
#92349=CARTESIAN_POINT ( 'NONE',  ( 10.89674973356500054, 1502.604160945439844, 215.7130242589950058 ) ) ;
#92350=CARTESIAN_POINT ( 'NONE',  ( 8.017723747350000707, 1421.540647238610063, 195.9972256206989982 ) ) ;
#92351=CARTESIAN_POINT ( 'NONE',  ( -1.708172839108350161, 1432.537737004170140, 218.4855024170419995 ) ) ;
#92352=CARTESIAN_POINT ( 'NONE',  ( 10.03970810010159909, 1480.319677133890082, 205.9223887158739785 ) ) ;
#92356=CARTESIAN_POINT ( 'NONE',  ( 12.45662817246929954, 1427.088122696140090, 206.6493147128259977 ) ) ;
#92364=CARTESIAN_POINT ( 'NONE',  ( 10.08433468493209872, 1427.583401277489884, 210.6616427254850237 ) ) ;
#92365=CARTESIAN_POINT ( 'NONE',  ( 11.78821558584650120, 1425.864958446819855, 202.8633695863799744 ) ) ;
#92372=CARTESIAN_POINT ( 'NONE',  ( -10.16653193143260125, 1461.891276504430152, 209.1676276534749945 ) ) ;
#92375=CARTESIAN_POINT ( 'NONE',  ( 5.314820689285160604, 1466.895574952380002, 217.5561230666059771 ) ) ;
#92381=CARTESIAN_POINT ( 'NONE',  ( 0.9412110656418017918, 1477.897737442060588, 198.7439859402530828 ) ) ;
#92385=CARTESIAN_POINT ( 'NONE',  ( 2.740701587498710179, 1426.136123854220159, 188.7843822190389744 ) ) ;
#92387=CARTESIAN_POINT ( 'NONE',  ( -15.00704310973959998, 1421.341523247710029, 203.5123511438659705 ) ) ;
#92396=ORIENTED_EDGE ( 'NONE', *, *, #88452, .T. ) ;
#92402=CARTESIAN_POINT ( 'NONE',  ( -1.204685347530000117, 1506.953552699789952, 221.9093730674989899 ) ) ;
#92410=CARTESIAN_POINT ( 'NONE',  ( 11.13275964168929910, 1426.431015207049768, 207.0489135758679993 ) ) ;
#92416=DIRECTION ( 'NONE',  ( -1.000000000000000000, 0.000000000000000000, 0.000000000000000000 ) ) ;
#92424=CARTESIAN_POINT ( 'NONE',  ( 9.103282207110000357, 1450.329653372990151, 206.7256654112989906 ) ) ;
#92427=CARTESIAN_POINT ( 'NONE',  ( 0.01997215604490120214, 1457.681682718290176, 199.5608357732290017 ) ) ;
#92436=CARTESIAN_POINT ( 'NONE',  ( -17.51974517380610052, 1417.750436891259824, 206.7510270525189924 ) ) ;
#92440=CARTESIAN_POINT ( 'NONE',  ( 11.70063000989999935, 1500.556383425389868, 207.1978923261789873 ) ) ;
#92456=CARTESIAN_POINT ( 'NONE',  ( 10.99044244102760004, 1479.494692313550104, 229.8297415043770116 ) ) ;
#92461=CARTESIAN_POINT ( 'NONE',  ( 10.55680192255090155, 1452.714797730689952, 209.8973982115319927 ) ) ;
#92462=CARTESIAN_POINT ( 'NONE',  ( -5.389604961048250154, 1507.858604756060004, 220.8468629847619980 ) ) ;
#92464=CARTESIAN_POINT ( 'NONE',  ( 4.274335294360000148, 1515.341803653790066, 210.5964280301390090 ) ) ;
#92484=CARTESIAN_POINT ( 'NONE',  ( -10.82265089720440088, 1462.846529889819976, 206.8444605232329820 ) ) ;
#92486=CARTESIAN_POINT ( 'NONE',  ( 10.42328684261450178, 1469.828409879329911, 207.1733329790250195 ) ) ;
#92487=CARTESIAN_POINT ( 'NONE',  ( -11.16643438350000039, 1471.372555911289965, 206.7508257855590159 ) ) ;
#92503=CARTESIAN_POINT ( 'NONE',  ( 2.329898844064780317, 1515.219291385429869, 213.4472495150509701 ) ) ;
#92508=CARTESIAN_POINT ( 'NONE',  ( -0.9525667512430020523, 1508.146044033290082, 220.9334930897990148 ) ) ;
#92510=CARTESIAN_POINT ( 'NONE',  ( -2.103463323419999753, 1431.236868155990123, 214.4359102488789972 ) ) ;
#92513=CARTESIAN_POINT ( 'NONE',  ( 8.104834441009998613, 1501.961773108790112, 207.6242399624189829 ) ) ;
#92516=CARTESIAN_POINT ( 'NONE',  ( -10.14004033922460124, 1481.416246290540130, 206.1146705078360242 ) ) ;
#92526=CARTESIAN_POINT ( 'NONE',  ( 1.551945958219810073, 1454.746255304280112, 218.4022335687689917 ) ) ;
#92529=CARTESIAN_POINT ( 'NONE',  ( -15.32028296150000024, 1415.735746099170001, 207.3531220195189917 ) ) ;
#92531=CARTESIAN_POINT ( 'NONE',  ( -3.141117940442379908, 1485.405160230890033, 197.6410428545480045 ) ) ;
#92532=CARTESIAN_POINT ( 'NONE',  ( -8.595910032225260622, 1436.830216193329989, 209.8479140031089969 ) ) ;
#92536=CIRCLE ( 'NONE', #40682, 524.3013518614112627 ) ;
#92538=CARTESIAN_POINT ( 'NONE',  ( -11.15142467606159826, 1508.551704408290107, 209.1655305885859946 ) ) ;
#92548=CARTESIAN_POINT ( 'NONE',  ( 4.226426730290000044, 1515.477082009390188, 208.7508285102820196 ) ) ;
#92551=( BOUNDED_CURVE ( )  B_SPLINE_CURVE ( 3, ( #16219, #65568, #67224, #40890 ),
 .UNSPECIFIED., .F., .T. ) 
 B_SPLINE_CURVE_WITH_KNOTS ( ( 4, 4 ),
 ( 1.005825317590492096, 2.135767310345805026 ),
 .UNSPECIFIED. ) 
 CURVE ( )  GEOMETRIC_REPRESENTATION_ITEM ( )  RATIONAL_B_SPLINE_CURVE ( ( 1.000000000000000000, 0.8964027527108247018, 0.8964027527108247018, 1.000000000000000000 ) ) 
 REPRESENTATION_ITEM ( '' )  );
#92554=ADVANCED_FACE ( 'NONE', ( #76049 ), #13504, .T. ) ;
#92558=CARTESIAN_POINT ( 'NONE',  ( 11.91319089239999940, 1436.492803299989873, 225.5464727294989871 ) ) ;
#92560=CARTESIAN_POINT ( 'NONE',  ( 4.677562605192279399, 1434.889072343160024, 228.7640133632109780 ) ) ;
#92563=B_SPLINE_CURVE_WITH_KNOTS ( 'NONE', 3,
 ( #89056, #12342, #46533, #29700, #4516, #30242, #63884, #55479, #12897, #38649, #21821, #90144, #81742, #57690, #76526, #108614, #51894, #26666, #66091, #26104, #74487, #77098, #17132, #31903, #9333, #100218, #86032, #40304, #51322, #407, #91805, #102272, #49277, #951, #23498, #83406, #110677, #85458, #8757, #35624, #15083, #25552, #8204 ),
 .UNSPECIFIED., .F., .F.,
 ( 4, 3, 3, 3, 3, 3, 3, 3, 3, 3, 3, 3, 3, 3, 4 ),
 ( -27.09462204860000156, -25.77410041705229915, -24.45357878550460029, -23.11321150369849775, -21.76171864759629671, -20.41647214834780044, -19.09105860935400045, -18.89473426365130138, -17.55491631884689951, -16.19268673722569929, -14.82069223479160058, -13.39723677660409962, -12.03725603264010147, -10.69631803245800228, -9.378668589109999232 ),
 .UNSPECIFIED. ) ;
#92565=CARTESIAN_POINT ( 'NONE',  ( 8.446022254560531906, 1449.499043747640144, 203.1286689207940128 ) ) ;
#92569=VECTOR ( 'NONE', #63608, 1000.000000000000114 ) ;
#92580=EDGE_LOOP ( 'NONE', ( #75139, #59800, #78453, #32857 ) ) ;
#92582=EDGE_CURVE ( 'NONE', #35548, #94111, #53489, .T. ) ;
#92584=CARTESIAN_POINT ( 'NONE',  ( 2.801043665294330243, 1515.551704203360032, 205.2926231557239873 ) ) ;
#92585=CARTESIAN_POINT ( 'NONE',  ( -0.3050640126979990430, 1444.736015696789991, 199.0470353275990192 ) ) ;
#92592=CARTESIAN_POINT ( 'NONE',  ( 10.52837420263239920, 1481.199010226290284, 208.2608686310830137 ) ) ;
#92609=CARTESIAN_POINT ( 'NONE',  ( -11.92169980599999946, 1502.281710837490209, 208.9298105593169907 ) ) ;
#92626=CARTESIAN_POINT ( 'NONE',  ( 8.503372964620000474, 1452.005661874290126, 212.9202014103589988 ) ) ;
#92634=CARTESIAN_POINT ( 'NONE',  ( 17.49022258196330171, 1428.660011336650086, 204.2345431054930032 ) ) ;
#92638=CARTESIAN_POINT ( 'NONE',  ( 9.327651199099038948, 1434.415569083649871, 206.2244204008570136 ) ) ;
#92645=CARTESIAN_POINT ( 'NONE',  ( 12.40160258794860049, 1420.584110727309962, 200.5244627772079866 ) ) ;
#92646=CARTESIAN_POINT ( 'NONE',  ( -2.417252593174890940, 1495.142685870479681, 220.0295633172205214 ) ) ;
#92653=CARTESIAN_POINT ( 'NONE',  ( 10.32067503063590053, 1469.846144623479859, 207.1838946627530049 ) ) ;
#92661=CARTESIAN_POINT ( 'NONE',  ( 4.509330006639999944, 1466.131481732889824, 218.7653230973990048 ) ) ;
#92675=EDGE_CURVE ( 'NONE', #73362, #77955, #64712, .T. ) ;
#92680=B_SPLINE_CURVE_WITH_KNOTS ( 'NONE', 3,
 ( #24339, #42259, #15923, #58520, #76406, #70125, #35939, #95831, #19099, #83700 ),
 .UNSPECIFIED., .F., .F.,
 ( 4, 2, 2, 2, 4 ),
 ( 0.000000000000000000, 0.2500000000000384137, 0.3750000000000323075, 0.5000000000000262013, 1.000000000000000000 ),
 .UNSPECIFIED. ) ;
#92682=CARTESIAN_POINT ( 'NONE',  ( -9.139549689176309499, 1438.859193681930265, 208.8000896448019716 ) ) ;
#92699=CARTESIAN_POINT ( 'NONE',  ( -1.073559339189999795, 1444.993510083389992, 218.0402162257890097 ) ) ;
#92704=CARTESIAN_POINT ( 'NONE',  ( 7.664247930350000182, 1423.636725678029961, 212.7912655606789940 ) ) ;
#92710=CARTESIAN_POINT ( 'NONE',  ( -19.97979314536150142, 1483.906058459090218, 214.0067405813460084 ) ) ;
#92716=CARTESIAN_POINT ( 'NONE',  ( -0.06846930289512999368, 1501.841009900990002, 233.2444182323090160 ) ) ;
#92726=CARTESIAN_POINT ( 'NONE',  ( -10.31302053876249936, 1447.618248150379941, 210.0527956824380169 ) ) ;
#92730=ORIENTED_EDGE ( 'NONE', *, *, #52310, .F. ) ;
#92732=ORIENTED_EDGE ( 'NONE', *, *, #80244, .F. ) ;
#92748=CARTESIAN_POINT ( 'NONE',  ( 3.375977085881459949, 1446.395221913229989, 199.5681764770490076 ) ) ;
#92749=CARTESIAN_POINT ( 'NONE',  ( -7.042124254411990414, 1488.841176089370038, 189.4374097027819914 ) ) ;
#92762=CARTESIAN_POINT ( 'NONE',  ( 9.682534244272909874, 1436.279766483590038, 210.8540000661170097 ) ) ;
#92767=ORIENTED_EDGE ( 'NONE', *, *, #7158, .F. ) ;
#92769=CARTESIAN_POINT ( 'NONE',  ( -11.40487640519999957, 1470.866518659589929, 208.6816973537609954 ) ) ;
#92772=CARTESIAN_POINT ( 'NONE',  ( -2.795964621609999590, 1422.864594294989956, 191.4386244948990168 ) ) ;
#92778=CARTESIAN_POINT ( 'NONE',  ( 4.231776932839999894, 1487.020005215089896, 198.7423800976989980 ) ) ;
#92782=CARTESIAN_POINT ( 'NONE',  ( -1.842963219480119985, 1515.064792700640055, 204.7923971808919816 ) ) ;
#92793=CARTESIAN_POINT ( 'NONE',  ( -3.657993755839999750, 1474.872004365689918, 218.7367895275489786 ) ) ;
#92798=CARTESIAN_POINT ( 'NONE',  ( -4.543595434040840431, 1508.194578301092406, 220.5427723295427143 ) ) ;
#92803=CARTESIAN_POINT ( 'NONE',  ( -10.94914411430109880, 1470.861661619450160, 209.5252488941420097 ) ) ;
#92804=LINE ( 'NONE', #16614, #108777 ) ;
#92806=EDGE_LOOP ( 'NONE', ( #14307, #72208, #106463, #41293 ) ) ;
#92807=VERTEX_POINT ( 'NONE', #12016 ) ;
#92809=CARTESIAN_POINT ( 'NONE',  ( -5.159279705950000405, 1438.838331987589982, 207.0068192150190214 ) ) ;
#92811=CARTESIAN_POINT ( 'NONE',  ( 7.793708231120000107, 1423.746790494559946, 195.8019968817989991 ) ) ;
#92812=VECTOR ( 'NONE', #45954, 1000.000000000000114 ) ;
#92814=CARTESIAN_POINT ( 'NONE',  ( 9.753082900275339640, 1422.542729491349974, 212.4417178624250084 ) ) ;
#92819=CARTESIAN_POINT ( 'NONE',  ( 10.94256459999999898, 1470.964391698490090, 209.6240817813279875 ) ) ;
#92820=CARTESIAN_POINT ( 'NONE',  ( 11.01161918054969924, 1492.458987749750122, 212.4071534856509800 ) ) ;
#92821=CARTESIAN_POINT ( 'NONE',  ( -2.909142857259999992, 1456.184073613490000, 218.1442093800189923 ) ) ;
#92827=ORIENTED_EDGE ( 'NONE', *, *, #100468, .T. ) ;
#92830=CARTESIAN_POINT ( 'NONE',  ( -3.269259737218870310, 1476.740802116999930, 199.2818558394819775 ) ) ;
#92832=CARTESIAN_POINT ( 'NONE',  ( 11.68690449393020003, 1479.943320198230140, 210.6621425521760216 ) ) ;
#92834=CARTESIAN_POINT ( 'NONE',  ( 1.956348389710000024, 1444.118055948189976, 203.1454441604489887 ) ) ;
#92837=CARTESIAN_POINT ( 'NONE',  ( -3.494218103360000161, 1450.155609024890055, 190.3271737256989979 ) ) ;
#92844=VERTEX_POINT ( 'NONE', #3646 ) ;
#92853=CARTESIAN_POINT ( 'NONE',  ( 1.002066158240000115, 1476.232001529690251, 198.0640689639990057 ) ) ;
#92858=CARTESIAN_POINT ( 'NONE',  ( 0.7577247913304160365, 1429.693372890590126, 217.4019828439899698 ) ) ;
#92859=CARTESIAN_POINT ( 'NONE',  ( -9.093965512229999604, 1423.880366148619942, 207.4491482849089721 ) ) ;
#92863=CARTESIAN_POINT ( 'NONE',  ( 7.340346552482979625, 1426.363565825339947, 212.7077574225189949 ) ) ;
#92866=VERTEX_POINT ( 'NONE', #71966 ) ;
#92869=CARTESIAN_POINT ( 'NONE',  ( -11.43932180835810186, 1491.557538122099913, 206.8739097152079864 ) ) ;
#92872=CARTESIAN_POINT ( 'NONE',  ( -0.5875326727945574534, 1487.946859735538737, 219.9643640775660458 ) ) ;
#92873=CARTESIAN_POINT ( 'NONE',  ( -16.52604361424539903, 1508.522046710420000, 213.6181396652249873 ) ) ;
#92874=CARTESIAN_POINT ( 'NONE',  ( 7.897123973650000295, 1424.702922360419961, 211.7415114879590021 ) ) ;
#92877=CARTESIAN_POINT ( 'NONE',  ( 18.13864071049999893, 1429.364573343489837, 207.4452956957889853 ) ) ;
#92880=CARTESIAN_POINT ( 'NONE',  ( 0.000000000000000000, 1515.551704408389924, 209.1218459616989946 ) ) ;
#92881=CARTESIAN_POINT ( 'NONE',  ( 9.761911793579997720, 1462.730917074890158, 209.3821448747769978 ) ) ;
#92882=ORIENTED_EDGE ( 'NONE', *, *, #72798, .T. ) ;
#92889=B_SPLINE_SURFACE_WITH_KNOTS ( 'NONE', 5, 5, ( 
 ( #98970, #64306, #80542, #55903, #90573, #31224 ),
 ( #90021, #13298, #47491, #65406, #11675, #37434 ),
 ( #54796, #97328, #105752, #45852, #79984, #63221 ),
 ( #20597, #83282, #33408, #75459, #8210, #15501 ),
 ( #110683, #49699, #41829, #41285, #49150, #23904 ),
 ( #91130, #74360, #100620, #83829, #65958, #6025 ),
 ( #23367, #31771, #74903, #7130, #100083, #108488 ),
 ( #57557, #109594, #67056, #91680, #32865, #48600 ),
 ( #109052, #82734, #42376, #76531, #67603, #58099 ),
 ( #14955, #33974, #32337, #6580, #25005, #50785 ),
 ( #93326, #40729, #66517, #92230, #101162, #24456 ),
 ( #58644, #25558, #84385, #92778, #101713, #16053 ),
 ( #50257, #75984, #68170, #7672, #102277, #110135 ),
 ( #59207, #14407, #16588, #84918, #40179, #1498 ),
 ( #86039, #70379, #10434, #96090, #60299, #19367 ) ),
 .UNSPECIFIED., .F., .F., .F.,
 ( 6, 3, 3, 3, 6 ),
 ( 6, 6 ),
 ( 14.35637078220000085, 25.15719987230000143, 30.14272855600000156, 32.63549289790000074, 35.12825723969999814 ),
 ( 0.000000000000000000, 2.000000000000000000 ),
 .UNSPECIFIED. ) ;
#92892=ORIENTED_EDGE ( 'NONE', *, *, #69299, .F. ) ;
#92903=CARTESIAN_POINT ( 'NONE',  ( -10.78779494798200034, 1480.680906080729983, 211.1296427397590207 ) ) ;
#92906=CARTESIAN_POINT ( 'NONE',  ( -3.545811734980049756, 1508.551704408389924, 213.8736419469829855 ) ) ;
#92908=CARTESIAN_POINT ( 'NONE',  ( 7.823331862799999037, 1421.665691048000099, 195.8606073899989894 ) ) ;
#92911=DIRECTION ( 'NONE',  ( -1.224646799147350002E-16, 1.836970198721029688E-16, 1.000000000000000000 ) ) ;
#92922=CARTESIAN_POINT ( 'NONE',  ( -11.24957740497779923, 1482.901240094499826, 205.2054264539789870 ) ) ;
#92923=B_SPLINE_SURFACE_WITH_KNOTS ( 'NONE', 5, 5, ( 
 ( #82855, #30240, #72822, #64975, #108051, #22929 ),
 ( #65531, #73922, #80665, #106955, #57133, #5047 ),
 ( #48173, #30797, #97462, #47615, #13425, #98550 ),
 ( #89054, #38646, #82311, #39192, #6144, #64434 ),
 ( #4514, #40302, #14540, #89602, #21819, #48729 ),
 ( #22369, #12895, #31347, #39762, #74485, #63882 ),
 ( #63342, #97997, #20731, #47072, #12340, #46531 ),
 ( #55477, #73369, #3979, #38103, #72281, #106413 ),
 ( #21267, #81196, #58771, #101283, #24026, #15081 ),
 ( #58226, #109182, #102407, #76119, #109718, #7799 ),
 ( #43075, #92350, #77235, #41421, #32466, #42506 ),
 ( #85597, #49275, #92908, #41965, #40855, #24578 ),
 ( #31901, #100742, #83404, #16182, #16721, #110815 ),
 ( #15622, #49828, #75586, #67735, #34108, #32993 ),
 ( #50383, #93450, #66641, #25137, #75030, #101844 ),
 ( #84511, #110259, #66088, #59340, #33535, #85052 ),
 ( #50921, #8342, #83958, #8897, #7258, #59884 ),
 ( #67182, #6700, #76666, #68299, #25689, #94009 ),
 ( #17274, #51465, #100215, #23496, #57688, #91803 ),
 ( #52033, #27364, #44744, #94555, #17828, #35772 ),
 ( #36314, #96229, #86169, #9462, #43627, #77775 ) ),
 .UNSPECIFIED., .F., .F., .F.,
 ( 6, 3, 3, 3, 3, 3, 6 ),
 ( 6, 6 ),
 ( 0.000000000000000000, 5.488753621229999879, 8.789679567349999445, 9.802594204569999192, 10.53188235890000080, 11.38341475070000008, 12.02704502919999996 ),
 ( 0.000000000000000000, 0.5000000000000000000 ),
 .UNSPECIFIED. ) ;
#92925=CARTESIAN_POINT ( 'NONE',  ( 9.067461874531819177, 1422.840410830630162, 212.2224494962840140 ) ) ;
#92926=CARTESIAN_POINT ( 'NONE',  ( 12.10217674255069831, 1421.433546240750047, 203.4323860903909917 ) ) ;
#92927=CARTESIAN_POINT ( 'NONE',  ( -11.03055288841810011, 1462.470873763560121, 208.6170698419460052 ) ) ;
#92929=CARTESIAN_POINT ( 'NONE',  ( -9.998385933616845023, 1478.713224390999585, 212.3145837183469666 ) ) ;
#92933=CARTESIAN_POINT ( 'NONE',  ( -9.826755612460519984, 1461.294814416169856, 209.7781363122770131 ) ) ;
#92934=CARTESIAN_POINT ( 'NONE',  ( -16.80096818656820190, 1420.465473985719882, 203.2469209014659839 ) ) ;
#92936=CARTESIAN_POINT ( 'NONE',  ( 11.48582467623369929, 1425.717167183619949, 202.9080862240699901 ) ) ;
#92937=FACE_OUTER_BOUND ( 'NONE', #45700, .T. ) ;
#92942=CARTESIAN_POINT ( 'NONE',  ( -8.118158757799047720, 1425.416527785969265, 208.7218458587759358 ) ) ;
#92946=CARTESIAN_POINT ( 'NONE',  ( 12.69240854808390040, 1426.852967891420121, 205.1934168669720009 ) ) ;
#92947=CARTESIAN_POINT ( 'NONE',  ( -9.299436737415328835, 1446.922292678779968, 190.6945112243980134 ) ) ;
#92948=CARTESIAN_POINT ( 'NONE',  ( -14.47400497512000150, 1421.606899549969967, 203.6042114461530161 ) ) ;
#92962=CARTESIAN_POINT ( 'NONE',  ( -3.273107898713619957, 1432.100754207539921, 216.8813792401940077 ) ) ;
#92970=CARTESIAN_POINT ( 'NONE',  ( 11.80015117941170111, 1427.466181701940059, 208.7971124954779896 ) ) ;
#92974=ORIENTED_EDGE ( 'NONE', *, *, #27677, .T. ) ;
#92975=CARTESIAN_POINT ( 'NONE',  ( 3.610101826099999744, 1473.850871782889953, 219.1404246027990155 ) ) ;
#92976=B_SPLINE_CURVE_WITH_KNOTS ( 'NONE', 5,
 ( #89464, #39040, #22227, #28461, #46391, #63204, #81058, #107364, #30094 ),
 .UNSPECIFIED., .F., .F.,
 ( 6, 3, 6 ),
 ( -13.00939335640000039, -6.504696678220000194, 0.000000000000000000 ),
 .UNSPECIFIED. ) ;
#92979=CARTESIAN_POINT ( 'NONE',  ( -11.77958525670000078, 1491.567240239189914, 205.4571824156389823 ) ) ;
#92984=CARTESIAN_POINT ( 'NONE',  ( 9.279405576849999449, 1450.853110856889771, 207.7367179272790167 ) ) ;
#92993=ORIENTED_EDGE ( 'NONE', *, *, #17104, .T. ) ;
#93002=AXIS2_PLACEMENT_3D ( 'NONE', #99749, #57243, #74580 ) ;
#93012=CARTESIAN_POINT ( 'NONE',  ( 9.738311102098309746, 1493.400122879349965, 188.2659922716460130 ) ) ;
#93017=CARTESIAN_POINT ( 'NONE',  ( 4.464391958920000292, 1426.554722128930052, 191.5974441596989948 ) ) ;
#93018=CARTESIAN_POINT ( 'NONE',  ( 10.45954636811110028, 1453.050608579339951, 210.8472557228290043 ) ) ;
#93020=CARTESIAN_POINT ( 'NONE',  ( -15.31153093854189962, 1508.451225488540103, 209.8004562725960227 ) ) ;
#93021=CIRCLE ( 'NONE', #60932, 11.73460161499999899 ) ;
#93023=CARTESIAN_POINT ( 'NONE',  ( -5.529153398355120430, 1454.733540159410040, 201.5061756946240052 ) ) ;
#93028=B_SPLINE_CURVE_WITH_KNOTS ( 'NONE', 5,
 ( #78965, #3783, #8972, #52102, #44252, #95193 ),
 .UNSPECIFIED., .F., .F.,
 ( 6, 6 ),
 ( 239.4206172199999969, 244.3064142099999856 ),
 .UNSPECIFIED. ) ;
#93038=CARTESIAN_POINT ( 'NONE',  ( 5.610572505957840406, 1429.830968158320047, 216.7704346018900310 ) ) ;
#93040=CARTESIAN_POINT ( 'NONE',  ( -9.833554420730120427, 1461.675800432549977, 208.3780452630800255 ) ) ;
#93042=CARTESIAN_POINT ( 'NONE',  ( 11.13973213087689906, 1470.272412021129867, 206.9146623043149873 ) ) ;
#93048=CARTESIAN_POINT ( 'NONE',  ( -20.69294079850000045, 1505.646924528690079, 209.1300474139309813 ) ) ;
#93049=CARTESIAN_POINT ( 'NONE',  ( 7.978761767491338475, 1468.077760772049942, 201.2729507454290001 ) ) ;
#93051=B_SPLINE_SURFACE_WITH_KNOTS ( 'NONE', 5, 1, ( 
 ( #4494, #83381 ),
 ( #6682, #38626 ),
 ( #13965, #40835 ),
 ( #75012, #64957 ),
 ( #5025, #98532 ),
 ( #63861, #97975 ) ),
 .UNSPECIFIED., .F., .F., .F.,
 ( 6, 6 ),
 ( 2, 2 ),
 ( 0.000000000000000000, 3.962517353580000012 ),
 ( 0.000000000000000000, 14.00000000000000000 ),
 .UNSPECIFIED. ) ;
#93057=CARTESIAN_POINT ( 'NONE',  ( 5.662343758720000508, 1504.894618425089902, 220.5557215505990314 ) ) ;
#93059=CARTESIAN_POINT ( 'NONE',  ( -11.44574129031820142, 1500.980493451109851, 211.1514305463080063 ) ) ;
#93066=CARTESIAN_POINT ( 'NONE',  ( -11.00907965078549999, 1462.196140238690077, 209.7526447668389835 ) ) ;
#93067=CARTESIAN_POINT ( 'NONE',  ( -2.298816259811510054, 1486.462377102800019, 220.8289805423670202 ) ) ;
#93071=CARTESIAN_POINT ( 'NONE',  ( -10.65742070623289983, 1481.357802822280064, 207.9456758233610287 ) ) ;
#93080=ADVANCED_FACE ( 'NONE', ( #58435 ), #12642, .T. ) ;
#93081=CARTESIAN_POINT ( 'NONE',  ( 4.319855718986739923, 1453.935607868970010, 217.4425725348959872 ) ) ;
#93083=VECTOR ( 'NONE', #16723, 999.9999999999998863 ) ;
#93084=CARTESIAN_POINT ( 'NONE',  ( -15.52522232080000109, 1416.123895944519973, 207.8294199178490089 ) ) ;
#93089=CARTESIAN_POINT ( 'NONE',  ( -5.215695451837711438, 1495.379824343749760, 198.7908095108026885 ) ) ;
#93092=CARTESIAN_POINT ( 'NONE',  ( -18.67614678860000055, 1441.800567318090089, 210.9159933499589954 ) ) ;
#93093=CARTESIAN_POINT ( 'NONE',  ( 10.50817522199910137, 1481.942267134329995, 210.4830409274069893 ) ) ;
#93100=CARTESIAN_POINT ( 'NONE',  ( -9.457584820017499894, 1462.148799351590014, 206.2711904065230044 ) ) ;
#93109=CARTESIAN_POINT ( 'NONE',  ( 3.347839154809999940, 1485.651791778389907, 219.4796426812989978 ) ) ;
#93112=CARTESIAN_POINT ( 'NONE',  ( -19.86670360899999821, 1443.974114956090034, 213.2631289620589712 ) ) ;
#93114=EDGE_CURVE ( 'NONE', #53131, #77321, #86934, .T. ) ;
#93116=CARTESIAN_POINT ( 'NONE',  ( -16.58369734668589501, 1417.133262957369880, 208.4557275984209923 ) ) ;
#93118=CARTESIAN_POINT ( 'NONE',  ( -3.665756888430000249, 1509.038615934189920, 204.6345961887290059 ) ) ;
#93119=CARTESIAN_POINT ( 'NONE',  ( -5.292247061280000331, 1391.913060387289988, 203.8075142969990168 ) ) ;
#93122=EDGE_CURVE ( 'NONE', #37425, #90721, #60659, .T. ) ;
#93123=CARTESIAN_POINT ( 'NONE',  ( 10.09177798305169915, 1451.176487112019913, 206.2838416248820010 ) ) ;
#93141=CARTESIAN_POINT ( 'NONE',  ( 4.325403553351909736, 1515.219291385429869, 206.7919471176340096 ) ) ;
#93142=CARTESIAN_POINT ( 'NONE',  ( 1.381522864419999941, 1444.570505314090042, 200.1133580050590126 ) ) ;
#93147=CARTESIAN_POINT ( 'NONE',  ( 2.309941155180000205, 1466.993925648989944, 219.5497868284989806 ) ) ;
#93149=CARTESIAN_POINT ( 'NONE',  ( 10.93008446023089952, 1479.841554277730211, 208.5739487062600119 ) ) ;
#93162=CARTESIAN_POINT ( 'NONE',  ( 11.19148376978288439, 1422.145534526647452, 210.4506217739875353 ) ) ;
#93172=DIRECTION ( 'NONE',  ( -1.913759484722300243E-19, 1.000000000000000000, -1.836968204960139822E-16 ) ) ;
#93175=CARTESIAN_POINT ( 'NONE',  ( 3.657829568870575976, 1442.827323799996748, 217.2295476630547171 ) ) ;
#93177=CARTESIAN_POINT ( 'NONE',  ( 7.892605823620001182, 1452.443926081389918, 214.1248619204189936 ) ) ;
#93183=CARTESIAN_POINT ( 'NONE',  ( -3.132119737639480483, 1428.847266505159951, 200.2946123499760063 ) ) ;
#93194=EDGE_CURVE ( 'NONE', #45310, #36236, #69755, .T. ) ;
#93198=CARTESIAN_POINT ( 'NONE',  ( 11.27257476199999964, 1426.317358070279852, 206.4672093773990014 ) ) ;
#93216=EDGE_CURVE ( 'NONE', #59183, #75973, #94890, .T. ) ;
#93227=CARTESIAN_POINT ( 'NONE',  ( -9.096590249497090497, 1440.282600144749949, 206.1070276416620004 ) ) ;
#93230=FACE_OUTER_BOUND ( 'NONE', #105415, .T. ) ;
#93233=CARTESIAN_POINT ( 'NONE',  ( 11.60235767850000066, 1501.497651028989821, 209.0874959428689976 ) ) ;
#93235=CARTESIAN_POINT ( 'NONE',  ( -9.471890498288960458, 1438.598768578280215, 210.0041281920070162 ) ) ;
#93236=CARTESIAN_POINT ( 'NONE',  ( 1.792279166353169861, 1494.398886770019999, 220.1169078828669967 ) ) ;
#93248=CARTESIAN_POINT ( 'NONE',  ( -12.48995958879999968, 1501.883328876989935, 211.6213070136890053 ) ) ;
#93251=CARTESIAN_POINT ( 'NONE',  ( 2.550590696230000010, 1455.409333296890054, 218.3516928308589797 ) ) ;
#93253=CARTESIAN_POINT ( 'NONE',  ( -8.587559811879998506, 1448.168510073290008, 212.1995923204489998 ) ) ;
#93262=EDGE_CURVE ( 'NONE', #53103, #26024, #97547, .T. ) ;
#93265=CARTESIAN_POINT ( 'NONE',  ( 4.709066435679999607, 1495.147136540189877, 220.5787752062990137 ) ) ;
#93268=CARTESIAN_POINT ( 'NONE',  ( -2.178514691999632991, 1508.356099863727650, 220.7675093205359360 ) ) ;
#93274=CARTESIAN_POINT ( 'NONE',  ( -2.170920964160679922, 1475.243440997999869, 197.8895928898250247 ) ) ;
#93277=CARTESIAN_POINT ( 'NONE',  ( -8.953512711461160123, 1447.964222359199994, 211.4838949693660197 ) ) ;
#93281=CARTESIAN_POINT ( 'NONE',  ( -4.326992699989999913, 1515.158586642790169, 209.1218459619010162 ) ) ;
#93290=CARTESIAN_POINT ( 'NONE',  ( -9.699660872752350116, 1472.030908259890111, 212.1562907213800031 ) ) ;
#93306=CARTESIAN_POINT ( 'NONE',  ( 10.48725263721749990, 1460.097526990779897, 206.1395495003129952 ) ) ;
#93310=VECTOR ( 'NONE', #101466, 1000.000000000000227 ) ;
#93312=DIRECTION ( 'NONE',  ( -1.699538841806929935E-33, 1.000000000000000000, -1.698192320643030073E-16 ) ) ;
#93316=CARTESIAN_POINT ( 'NONE',  ( -10.10810022239999917, 1473.154118535690031, 207.6476596274190172 ) ) ;
#93318=ORIENTED_EDGE ( 'NONE', *, *, #19919, .T. ) ;
#93323=CARTESIAN_POINT ( 'NONE',  ( -9.678642251699999477, 1414.581381510680103, 208.2850554633440083 ) ) ;
#93326=CARTESIAN_POINT ( 'NONE',  ( 4.907342515529999893, 1485.995388969990245, 199.5215206418690173 ) ) ;
#93327=CARTESIAN_POINT ( 'NONE',  ( 1.338019250827790163, 1431.361302059610125, 218.5179660117710227 ) ) ;
#93339=CARTESIAN_POINT ( 'NONE',  ( -21.39706014069999895, 1505.152228921489950, 211.4762334770289840 ) ) ;
#93341=CARTESIAN_POINT ( 'NONE',  ( -4.376990639194925592, 1508.181752870080800, 220.5833432285685944 ) ) ;
#93348=CARTESIAN_POINT ( 'NONE',  ( -10.27997055782769920, 1471.607896215150049, 209.6291398427710249 ) ) ;
#93353=ORIENTED_EDGE ( 'NONE', *, *, #73400, .T. ) ;
#93361=CARTESIAN_POINT ( 'NONE',  ( 2.448877809997429988, 1508.551704408389924, 219.5616561886379827 ) ) ;
#93362=CARTESIAN_POINT ( 'NONE',  ( 5.140094423509999011, 1436.845494339190054, 228.7442485628990028 ) ) ;
#93365=CARTESIAN_POINT ( 'NONE',  ( -5.254554520956747687, 1391.913060387289988, 214.4737135289948071 ) ) ;
#93366=CARTESIAN_POINT ( 'NONE',  ( 12.32717396260830078, 1492.190839752460079, 209.5895836007599939 ) ) ;
#93367=CARTESIAN_POINT ( 'NONE',  ( -1.880000144899999892, 1457.107126484389937, 218.8420116927090078 ) ) ;
#93371=CARTESIAN_POINT ( 'NONE',  ( 8.274166279097638466, 1436.481534978870059, 206.7313558027209695 ) ) ;
#93380=CARTESIAN_POINT ( 'NONE',  ( -6.816032832730000379, 1464.119504676089946, 200.4313534491789994 ) ) ;
#93382=FACE_OUTER_BOUND ( 'NONE', #48086, .T. ) ;
#93384=CARTESIAN_POINT ( 'NONE',  ( -15.31939472967450122, 1508.551704408389924, 214.5736414636859877 ) ) ;
#93388=CARTESIAN_POINT ( 'NONE',  ( 5.538490023541649876, 1434.582427083100129, 202.4776097773300023 ) ) ;
#93390=AXIS2_PLACEMENT_3D ( 'NONE', #46410, #29037, #71633 ) ;
#93394=CARTESIAN_POINT ( 'NONE',  ( 4.912821653402110300, 1470.978916084819957, 187.7503311908630224 ) ) ;
#93395=CARTESIAN_POINT ( 'NONE',  ( -9.828024340748898524, 1446.801136768030119, 212.2328356403849909 ) ) ;
#93397=CARTESIAN_POINT ( 'NONE',  ( -14.48519483975229960, 1416.181292564900104, 203.8595933512790168 ) ) ;
#93404=CARTESIAN_POINT ( 'NONE',  ( -1.804012654820000172, 1476.275330878590012, 198.7886378605990103 ) ) ;
#93409=CARTESIAN_POINT ( 'NONE',  ( 2.151199513684490139, 1429.150501611710069, 217.1299383594469816 ) ) ;
#93410=CARTESIAN_POINT ( 'NONE',  ( -7.824467775549998727, 1425.791227067999898, 206.8230464701690039 ) ) ;
#93415=CARTESIAN_POINT ( 'NONE',  ( 7.225592507856469560, 1426.518265663189823, 212.9482508202709994 ) ) ;
#93419=CARTESIAN_POINT ( 'NONE',  ( -10.94209231895430179, 1492.979988125699947, 207.3926202358989883 ) ) ;
#93422=CARTESIAN_POINT ( 'NONE',  ( -4.261736552472808803, 1515.372048948340080, 207.2788837468951613 ) ) ;
#93423=CARTESIAN_POINT ( 'NONE',  ( 10.54065430160000005, 1425.980116282510153, 194.3020730708990129 ) ) ;
#93430=ORIENTED_EDGE ( 'NONE', *, *, #77426, .T. ) ;
#93436=CARTESIAN_POINT ( 'NONE',  ( 4.246473540454690720, 1508.879013859839915, 212.8696703459879984 ) ) ;
#93439=CARTESIAN_POINT ( 'NONE',  ( -5.706316465129999571, 1427.594387386090148, 202.5140759953890210 ) ) ;
#93443=CARTESIAN_POINT ( 'NONE',  ( 0.3220128118225270009, 1444.991323582689802, 199.0632997620110132 ) ) ;
#93445=EDGE_LOOP ( 'NONE', ( #6265, #82525, #7411, #81550 ) ) ;
#93446=CARTESIAN_POINT ( 'NONE',  ( -10.88526200584609960, 1480.877704328530172, 210.6248047774270162 ) ) ;
#93447=CARTESIAN_POINT ( 'NONE',  ( 5.382848799108077564, 1434.543798359927450, 202.5092580921534307 ) ) ;
#93448=CARTESIAN_POINT ( 'NONE',  ( -4.604592056941269718, 1508.551704408389924, 212.9405302482509796 ) ) ;
#93450=CARTESIAN_POINT ( 'NONE',  ( 7.496491729189999731, 1422.157925818930153, 195.6730238920989962 ) ) ;
#93451=CARTESIAN_POINT ( 'NONE',  ( -2.012497635052489908, 1432.674193821990002, 218.4327187538029875 ) ) ;
#93452=CARTESIAN_POINT ( 'NONE',  ( -4.474843316269999427, 1495.214972003490175, 197.6335801705990036 ) ) ;
#93455=DIRECTION ( 'NONE',  ( 0.9824080081115887930, -2.243614313870717968E-31, 0.1867471702549210744 ) ) ;
#93459=EDGE_LOOP ( 'NONE', ( #63084, #35465, #90793 ) ) ;
#93467=ADVANCED_FACE ( 'NONE', ( #8983 ), #48445, .T. ) ;
#93473=B_SPLINE_CURVE_WITH_KNOTS ( 'NONE', 3,
 ( #29441, #3731, #107257, #5352, #12654, #91001, #22671, #106164, #81490, #56872, #89360, #30552, #4791, #65281, #80961, #80417 ),
 .UNSPECIFIED., .F., .F.,
 ( 4, 3, 3, 3, 3, 4 ),
 ( -7.430926500750000052, -7.205864747455129837, -6.166310293502959894, -5.126937956299970622, -4.087228192414619876, -3.046684027040000409 ),
 .UNSPECIFIED. ) ;
#93474=CARTESIAN_POINT ( 'NONE',  ( -10.99082249780570031, 1462.122377081429931, 210.0450475653020135 ) ) ;
#93475=CARTESIAN_POINT ( 'NONE',  ( -16.76078030769999927, 1420.494757909599912, 203.1294657649889928 ) ) ;
#93476=CARTESIAN_POINT ( 'NONE',  ( 12.80027819501479946, 1420.728244072559846, 201.6266405663580201 ) ) ;
#93477=CARTESIAN_POINT ( 'NONE',  ( 6.653879410529840221, 1466.704669164200141, 216.5527109682910236 ) ) ;
#93485=CARTESIAN_POINT ( 'NONE',  ( 3.727343958979999705, 1478.549430577389785, 229.1364021244989715 ) ) ;
#93488=CARTESIAN_POINT ( 'NONE',  ( -5.292247061280000331, 1391.913060387289988, 203.8075142969990168 ) ) ;
#93489=CARTESIAN_POINT ( 'NONE',  ( 20.56230379148770027, 1477.111289846620139, 217.7195331044080149 ) ) ;
#93491=CARTESIAN_POINT ( 'NONE',  ( -13.58779897810510029, 1422.057029525010194, 203.7652383086400221 ) ) ;
#93500=VERTEX_POINT ( 'NONE', #54331 ) ;
#93503=CARTESIAN_POINT ( 'NONE',  ( 7.273621552740451968, 1447.419844749426829, 203.6721120216986662 ) ) ;
#93505=CARTESIAN_POINT ( 'NONE',  ( -7.878925220306069122, 1435.199465323840059, 212.6510895369020204 ) ) ;
#93507=CARTESIAN_POINT ( 'NONE',  ( -17.80192030199999920, 1421.535218730880160, 207.7056227470090164 ) ) ;
#93513=CARTESIAN_POINT ( 'NONE',  ( 12.25515206146219960, 1421.728505657969890, 208.1409196252290030 ) ) ;
#93519=CARTESIAN_POINT ( 'NONE',  ( 2.771411902819999717, 1474.602400374589934, 220.2115235061990006 ) ) ;
#93522=CARTESIAN_POINT ( 'NONE',  ( 19.13035349170000288, 1454.816283974190128, 206.3418420143889875 ) ) ;
#93524=CARTESIAN_POINT ( 'NONE',  ( -7.515867157249999764, 1494.783219423989976, 200.6183447482190161 ) ) ;
#93528=CARTESIAN_POINT ( 'NONE',  ( 9079.130222195200986, 5181.793945261120825, 1985.491949542980137 ) ) ;
#93536=CARTESIAN_POINT ( 'NONE',  ( -2.443866463060000438, 1496.089559380390028, 197.4171228521990145 ) ) ;
#93538=VERTEX_POINT ( 'NONE', #28551 ) ;
#93550=CARTESIAN_POINT ( 'NONE',  ( 12.57213386914980013, 1501.053060317580048, 211.0179505362860084 ) ) ;
#93552=CARTESIAN_POINT ( 'NONE',  ( 3.586875048626919860, 1508.551704408389924, 213.8556843534749987 ) ) ;
#93556=CARTESIAN_POINT ( 'NONE',  ( 9.249044665192510450, 1461.483507358830138, 206.1780078038019894 ) ) ;
#93558=EDGE_LOOP ( 'NONE', ( #57947, #65786, #63641, #57935 ) ) ;
#93563=CARTESIAN_POINT ( 'NONE',  ( -14.16968073959050045, 1507.983981868130059, 209.4049785662649867 ) ) ;
#93564=CARTESIAN_POINT ( 'NONE',  ( 4.015749066599999750, 1515.588778490289997, 209.8749815410619988 ) ) ;
#93568=CARTESIAN_POINT ( 'NONE',  ( 9.657865277128729886, 1451.546502117730142, 208.2092904370149995 ) ) ;
#93579=CARTESIAN_POINT ( 'NONE',  ( 5.215161240205300253, 1429.990180876930253, 217.0496817771059739 ) ) ;
#93581=CARTESIAN_POINT ( 'NONE',  ( -7.675557469593909943, 1490.010120624091769, 216.9302191894742293 ) ) ;
#93585=CARTESIAN_POINT ( 'NONE',  ( 5.755589866880000294, 1494.343251907090007, 219.1208360334990175 ) ) ;
#93590=CARTESIAN_POINT ( 'NONE',  ( 6.502040414733439633, 1467.454815019450052, 200.0748247799739943 ) ) ;
#93597=CARTESIAN_POINT ( 'NONE',  ( -14.15287909329999927, 1415.677402202029953, 214.2967794726189936 ) ) ;
#93598=CARTESIAN_POINT ( 'NONE',  ( -11.26962181946710118, 1500.379234792439775, 210.9259952136519871 ) ) ;
#93601=CARTESIAN_POINT ( 'NONE',  ( -2.152267782280000041, 1508.551704408389924, 220.2796779675990138 ) ) ;
#93604=CARTESIAN_POINT ( 'NONE',  ( 3.150079082345019987, 1446.276749673359973, 199.4986788256669854 ) ) ;
#93606=DIRECTION ( 'NONE',  ( -9.341989762165448955E-47, 1.000000000000000000, -1.836970198721029688E-16 ) ) ;
#93609=CARTESIAN_POINT ( 'NONE',  ( -11.82004774745709952, 1482.260572698100077, 207.7363177859789971 ) ) ;
#93610=CARTESIAN_POINT ( 'NONE',  ( -18.18664760840000127, 1466.015845117190111, 218.0276224371390015 ) ) ;
#93621=CARTESIAN_POINT ( 'NONE',  ( -15.00614681839999953, 1416.220781585230043, 205.5855558466790001 ) ) ;
#93625=CARTESIAN_POINT ( 'NONE',  ( -16.41393203050009220, 1419.676706660666696, 209.5083631726842839 ) ) ;
#93627=ORIENTED_EDGE ( 'NONE', *, *, #2824, .F. ) ;
#93630=FACE_OUTER_BOUND ( 'NONE', #72796, .T. ) ;
#93644=CARTESIAN_POINT ( 'NONE',  ( 3.848901911860000080, 1484.746040934790017, 219.9081948904990043 ) ) ;
#93645=CARTESIAN_POINT ( 'NONE',  ( 4.009460067780000081, 1422.110854443290009, 194.2227175196989890 ) ) ;
#93647=CARTESIAN_POINT ( 'NONE',  ( -8.468273497790530513, 1438.274789257269958, 228.4488543761889900 ) ) ;
#93649=CARTESIAN_POINT ( 'NONE',  ( -21.26810766748090131, 1485.919195119950018, 201.7808564924430073 ) ) ;
#93656=CARTESIAN_POINT ( 'NONE',  ( 7.801285059986189374, 1449.017548237110077, 202.3630618800679883 ) ) ;
#93664=CARTESIAN_POINT ( 'NONE',  ( 10.16310853745439857, 1503.066809769739848, 217.0134810410080206 ) ) ;
#93672=CARTESIAN_POINT ( 'NONE',  ( -12.71559489689999900, 1467.455103516190093, 192.9444858715990279 ) ) ;
#93674=CARTESIAN_POINT ( 'NONE',  ( 4.077241479695380200, 1515.224507089990084, 205.5390440451549807 ) ) ;
#93682=B_SPLINE_SURFACE_WITH_KNOTS ( 'NONE', 5, 1, ( 
 ( #24090, #58278 ),
 ( #84012, #41478 ),
 ( #109776, #58824 ),
 ( #33593, #79496 ),
 ( #54311, #96850 ),
 ( #43679, #63268 ),
 ( #88438, #103573 ),
 ( #62728, #87335 ),
 ( #77830, #104129 ) ),
 .UNSPECIFIED., .F., .F., .F.,
 ( 6, 3, 6 ),
 ( 2, 2 ),
 ( -8.704553073772529568E-10, 8.290775826610000010, 16.58943550237049891 ),
 ( 0.000000000000000000, 14.00000211182629961 ),
 .UNSPECIFIED. ) ;
#93683=CARTESIAN_POINT ( 'NONE',  ( 5.579983761340000292, 1439.143574310590111, 210.6739328916289935 ) ) ;
#93686=FACE_OUTER_BOUND ( 'NONE', #68647, .T. ) ;
#93689=ORIENTED_EDGE ( 'NONE', *, *, #308, .F. ) ;
#93693=CARTESIAN_POINT ( 'NONE',  ( -7.030811903863808610, 1475.320784634834354, 201.5754146800807689 ) ) ;
#93697=( GEOMETRIC_REPRESENTATION_CONTEXT ( 3 ) GLOBAL_UNCERTAINTY_ASSIGNED_CONTEXT ( ( #95011 ) ) GLOBAL_UNIT_ASSIGNED_CONTEXT ( ( #5435, #16014, #35464 ) ) REPRESENTATION_CONTEXT ( 'NONE', 'WORKASPACE' ) );
#93713=CARTESIAN_POINT ( 'NONE',  ( -14.60203837859040021, 1508.551704408389924, 210.3568941631429823 ) ) ;
#93715=CARTESIAN_POINT ( 'NONE',  ( 8.723134474349999223, 1451.781317889190177, 212.2855316608589931 ) ) ;
#93717=B_SPLINE_SURFACE_WITH_KNOTS ( 'NONE', 5, 1, ( 
 ( #6365, #7463 ),
 ( #5825, #67399 ),
 ( #83610, #108271 ),
 ( #24252, #90915 ),
 ( #107722, #14199 ),
 ( #23704, #58432 ),
 ( #108822, #47820 ),
 ( #32668, #75241 ),
 ( #65734, #41625 ),
 ( #92560, #15830 ),
 ( #100421, #66846 ),
 ( #22025, #56777 ),
 ( #39415, #31557 ),
 ( #39964, #66303 ),
 ( #50034, #41064 ),
 ( #100956, #48942 ),
 ( #5262, #40512 ),
 ( #56223, #99299 ),
 ( #109391, #74140 ),
 ( #48386, #81955 ),
 ( #57888, #84162 ),
 ( #82528, #23148 ),
 ( #22573, #65187 ),
 ( #75779, #109932 ),
 ( #92024, #90354 ),
 ( #33210, #49487 ),
 ( #83073, #73592 ),
 ( #99853, #31007 ),
 ( #57351, #91476 ),
 ( #32118, #15295 ),
 ( #43290, #10221 ),
 ( #86377, #1855 ),
 ( #16932, #86930 ),
 ( #26460, #738 ),
 ( #34321, #27035 ),
 ( #85825, #94213 ),
 ( #35990, #25899 ),
 ( #84710, #94779 ),
 ( #93649, #77980 ),
 ( #43835, #8557 ),
 ( #44399, #77438 ),
 ( #9663, #1288 ),
 ( #101497, #9123 ),
 ( #78541, #34870 ),
 ( #35427, #17488 ),
 ( #58987, #103159 ),
 ( #69058, #51686 ),
 ( #103736, #24785 ),
 ( #51134, #60655 ),
 ( #18056, #197 ),
 ( #69614, #59537 ) ),
 .UNSPECIFIED., .F., .F., .F.,
 ( 6, 3, 3, 3, 3, 3, 3, 3, 3, 3, 3, 3, 3, 3, 3, 3, 6 ),
 ( 2, 2 ),
 ( 0.000000000000000000, 28.69702819429999963, 61.04778752440000034, 93.62768910810000023, 123.7336603250000024, 156.1762685979999787, 187.3272846180000215, 220.4669312460000015, 237.3878297990000021, 254.2938300590000154, 289.2398204710000300, 325.3030936050000150, 360.8626869010000178, 395.8828220460000011, 432.6128460950000090, 468.8934854820000169, 502.1482307969999965 ),
 ( -1.158612088544819935E-09, 2.001768489946770035 ),
 .UNSPECIFIED. ) ;
#93719=CARTESIAN_POINT ( 'NONE',  ( -2.800144927338689804, 1429.031935871130145, 200.1802602962729907 ) ) ;
#93723=CARTESIAN_POINT ( 'NONE',  ( -11.87328627558470018, 1482.014094172719979, 208.6022272904490080 ) ) ;
#93726=ORIENTED_EDGE ( 'NONE', *, *, #46392, .F. ) ;
#93729=CARTESIAN_POINT ( 'NONE',  ( 10.92886027419739925, 1490.469936390880093, 210.0530976118369892 ) ) ;
#93746=LINE ( 'NONE', #75341, #10896 ) ;
#93754=CARTESIAN_POINT ( 'NONE',  ( 5.544571539851137487, 1465.562015094885737, 218.7011515308894047 ) ) ;
#93757=VERTEX_POINT ( 'NONE', #110212 ) ;
#93761=CARTESIAN_POINT ( 'NONE',  ( 0.000000000000000000, 1515.551704408389924, 209.1218459616989946 ) ) ;
#93763=CARTESIAN_POINT ( 'NONE',  ( 12.02501080200000061, 1501.456225530590018, 211.6043546659689980 ) ) ;
#93766=CARTESIAN_POINT ( 'NONE',  ( 7.465427998170000023, 1423.561403314650079, 212.9273434364789921 ) ) ;
#93768=CARTESIAN_POINT ( 'NONE',  ( -11.51163193560000053, 1413.913060387330006, 206.7812028963490150 ) ) ;
#93780=CARTESIAN_POINT ( 'NONE',  ( 3.044773427654349440, 1435.191935258749936, 227.3099679716739843 ) ) ;
#93790=CARTESIAN_POINT ( 'NONE',  ( 7.717520428720000325, 1424.057070268800089, 212.3256381827789880 ) ) ;
#93791=CARTESIAN_POINT ( 'NONE',  ( -17.11733429290000075, 1420.830776148560062, 201.6585816624789800 ) ) ;
#93792=LINE ( 'NONE', #87075, #74860 ) ;
#93794=B_SPLINE_SURFACE_WITH_KNOTS ( 'NONE', 5, 5, ( 
 ( #74769, #32201, #100502, #23781, #57969, #15381 ),
 ( #49570, #83698, #6994, #24337, #15921, #81852 ),
 ( #12458, #14092, #107067, #5155, #46640, #72389 ),
 ( #38206, #89167, #21924, #48281, #47721, #64543 ),
 ( #20844, #12991, #20295, #37663, #47174, #30352 ),
 ( #3540, #21380, #106518, #13535, #80774, #55589 ),
 ( #29261, #80222, #63995, #97572, #39864, #30902 ),
 ( #29807, #73483, #56119, #98661, #11914, #81302 ),
 ( #90253, #39312, #107619, #89713, #65080, #99195 ) ),
 .UNSPECIFIED., .F., .F., .F.,
 ( 6, 3, 6 ),
 ( 6, 6 ),
 ( -0.0001215403142825610000, 11.59601121190000050, 17.59296286301430001 ),
 ( -0.0001215403143104999955, 2.000000000000000000 ),
 .UNSPECIFIED. ) ;
#93798=ORIENTED_EDGE ( 'NONE', *, *, #11217, .F. ) ;
#93806=CARTESIAN_POINT ( 'NONE',  ( -3.021909043552730267, 1474.995172108610177, 198.0928472765529875 ) ) ;
#93810=CARTESIAN_POINT ( 'NONE',  ( -8.587344795677900322, 1448.168822778199910, 212.1998721081249926 ) ) ;
#93816=B_SPLINE_SURFACE_WITH_KNOTS ( 'NONE', 5, 5, ( 
 ( #80852, #10895, #28797, #68200, #102303, #85494 ),
 ( #8793, #37198, #104394, #27690, #71393, #105507 ),
 ( #20370, #74666, #108800, #57327, #106594, #22552 ),
 ( #21459, #73568, #23681, #98741, #49461, #99276 ),
 ( #81934, #83583, #81374, #38828, #39392, #5237 ),
 ( #38281, #48361, #91993, #72464, #47248, #56755 ) ),
 .UNSPECIFIED., .F., .F., .F.,
 ( 6, 6 ),
 ( 6, 6 ),
 ( 4.991132198159999867, 7.657648704650000582 ),
 ( 0.000000000000000000, 0.5000000000000000000 ),
 .UNSPECIFIED. ) ;
#93817=AXIS2_PLACEMENT_3D ( 'NONE', #96082, #45714, #88246 ) ;
#93826=B_SPLINE_SURFACE_WITH_KNOTS ( 'NONE', 5, 1, ( 
 ( #59409, #94633 ),
 ( #17907, #34180 ),
 ( #26890, #1155 ),
 ( #69470, #93522 ),
 ( #86790, #77303 ),
 ( #78397, #51541 ) ),
 .UNSPECIFIED., .F., .F., .F.,
 ( 6, 6 ),
 ( 2, 2 ),
 ( 0.000000000000000000, 3.563599656280000083 ),
 ( 0.000000000000000000, 14.00000000000000000 ),
 .UNSPECIFIED. ) ;
#93830=ADVANCED_FACE ( 'NONE', ( #20548 ), #80558, .T. ) ;
#93831=EDGE_CURVE ( 'NONE', #61245, #11716, #30921, .T. ) ;
#93833=B_SPLINE_CURVE_WITH_KNOTS ( 'NONE', 5,
 ( #14018, #67633, #90738, #76559, #48208, #101189, #51358, #82347, #50815 ),
 .UNSPECIFIED., .F., .F.,
 ( 6, 3, 6 ),
 ( 0.000000000000000000, 0.2400526034259363450, 1.000000000000000000 ),
 .UNSPECIFIED. ) ;
#93848=CARTESIAN_POINT ( 'NONE',  ( -10.78800202809769893, 1480.681112002840109, 211.1294777255430120 ) ) ;
#93864=CARTESIAN_POINT ( 'NONE',  ( -3.899052081260000246, 1430.170681384590125, 201.7535711888990022 ) ) ;
#93873=CARTESIAN_POINT ( 'NONE',  ( 2.764297497180530083, 1430.881855750599925, 218.1996282248960028 ) ) ;
#93881=CARTESIAN_POINT ( 'NONE',  ( -16.83891731359999966, 1420.416781728159776, 203.6059137768390030 ) ) ;
#93885=CARTESIAN_POINT ( 'NONE',  ( 1.859895826240000050, 1474.627878585689814, 219.9708148048989926 ) ) ;
#93886=CARTESIAN_POINT ( 'NONE',  ( 0.000000000000000000, 1515.551704408389924, 209.1218459616989946 ) ) ;
#93890=CARTESIAN_POINT ( 'NONE',  ( -6.649360560760902317, 1508.353256394122127, 219.8944077188511130 ) ) ;
#93896=CARTESIAN_POINT ( 'NONE',  ( -8.459381271141269920, 1419.310188839569946, 195.9551710783830174 ) ) ;
#93897=CARTESIAN_POINT ( 'NONE',  ( 4.326992699990039881, 1515.158586642889986, 209.0578234245899978 ) ) ;
#93900=VERTEX_POINT ( 'NONE', #109543 ) ;
#93903=CARTESIAN_POINT ( 'NONE',  ( 8.883832781222039898, 1425.079104944299843, 195.6883722520829849 ) ) ;
#93904=CARTESIAN_POINT ( 'NONE',  ( -10.38946316992339902, 1479.436785722010200, 210.5481016495319864 ) ) ;
#93907=CARTESIAN_POINT ( 'NONE',  ( -4.642542606699569419, 1378.262313272806523, 203.6938890911571320 ) ) ;
#93914=CARTESIAN_POINT ( 'NONE',  ( 10.49159676556239873, 1452.005212983920046, 208.0898620772609888 ) ) ;
#93918=CARTESIAN_POINT ( 'NONE',  ( 8.535515121215828671, 1436.958083742609915, 207.8253345400139835 ) ) ;
#93926=CARTESIAN_POINT ( 'NONE',  ( 11.77725420934070044, 1479.493139331419798, 209.1772973198850138 ) ) ;
#93933=CARTESIAN_POINT ( 'NONE',  ( 0.8856752070958160417, 1486.352519237200113, 197.2385176272069884 ) ) ;
#93941=CARTESIAN_POINT ( 'NONE',  ( 20.60747693140000081, 1477.505856213189873, 217.6602180427189808 ) ) ;
#93947=CARTESIAN_POINT ( 'NONE',  ( 2.330134126090000368, 1515.551704408389924, 212.9514660752490158 ) ) ;
#93948=CARTESIAN_POINT ( 'NONE',  ( 9.990309780743139356, 1460.215770112410155, 206.0069743695009947 ) ) ;
#93949=CARTESIAN_POINT ( 'NONE',  ( -1.986418230135969853, 1420.852199177890043, 193.8262422174969970 ) ) ;
#93951=CARTESIAN_POINT ( 'NONE',  ( -2.234267340169999727, 1476.147103045889935, 198.8785287704990026 ) ) ;
#93953=VECTOR ( 'NONE', #97591, 1000.000000000000114 ) ;
#93955=B_SPLINE_CURVE_WITH_KNOTS ( 'NONE', 3,
 ( #68561, #102660, #85890, #85319, #8614, #49549, #93713, #101015, #32728, #75844, #25960, #42791, #9192, #94276, #24314, #58496, #51754, #33270, #103219, #51190, #43354, #77502, #16990, #60155, #260, #802, #34931, #59597, #69118, #76951, #26527 ),
 .UNSPECIFIED., .F., .F.,
 ( 4, 3, 3, 3, 3, 3, 3, 3, 3, 3, 4 ),
 ( -117.7436746770000013, -117.2149955653400042, -116.2593090969979954, -115.4891864406449997, -114.8126480616819975, -114.1739245078169915, -113.5701753798730067, -112.8587766767369942, -112.0199461915819938, -111.3181123378909945, -110.7231579952140095 ),
 .UNSPECIFIED. ) ;
#93964=B_SPLINE_SURFACE_WITH_KNOTS ( 'NONE', 5, 1, ( 
 ( #58983, #50579 ),
 ( #9120, #85256 ),
 ( #84707, #25340 ),
 ( #60094, #17485 ),
 ( #51683, #45515 ),
 ( #97541, #27575 ) ),
 .UNSPECIFIED., .F., .F., .F.,
 ( 6, 6 ),
 ( 2, 2 ),
 ( -2.269822869709659820E-05, 16.31242598182869941 ),
 ( 0.000000000000000000, 14.00002269822869927 ),
 .UNSPECIFIED. ) ;
#93966=CARTESIAN_POINT ( 'NONE',  ( 7.533869295375639652, 1425.775636318390070, 212.2138369296450264 ) ) ;
#93970=CARTESIAN_POINT ( 'NONE',  ( -10.99258910100319930, 1492.354469455359776, 207.1887574598779906 ) ) ;
#93974=CARTESIAN_POINT ( 'NONE',  ( -16.59142030353789821, 1508.492718974290028, 213.6717301258460111 ) ) ;
#93975=DIRECTION ( 'NONE',  ( -1.000000000000000000, 0.000000000000000000, 0.000000000000000000 ) ) ;
#93977=CARTESIAN_POINT ( 'NONE',  ( 4.559613763440699685, 1467.726731048589954, 217.9977195186110066 ) ) ;
#93989=CARTESIAN_POINT ( 'NONE',  ( -18.22824482168599758, 1443.229620491730202, 204.5519806992609801 ) ) ;
#94002=CARTESIAN_POINT ( 'NONE',  ( -1.278600148798100022, 1444.381613973289859, 199.1499497165799824 ) ) ;
#94009=CARTESIAN_POINT ( 'NONE',  ( 7.348570800660000124, 1422.803073198840139, 195.5677875354990078 ) ) ;
#94012=CARTESIAN_POINT ( 'NONE',  ( -3.938370151530000474, 1495.868122056089987, 198.2201402197989921 ) ) ;
#94026=CARTESIAN_POINT ( 'NONE',  ( 8.561386400597299939, 1423.835855477939958, 211.2535102716829840 ) ) ;
#94027=CARTESIAN_POINT ( 'NONE',  ( 3.975726521872664510, 1422.097627045033278, 194.1803425279607040 ) ) ;
#94028=CARTESIAN_POINT ( 'NONE',  ( -10.91387039267799963, 1462.739297843610075, 207.3784283796969987 ) ) ;
#94035=CARTESIAN_POINT ( 'NONE',  ( -9.104779855139769396, 1421.478964305890031, 192.1853055963059660 ) ) ;
#94036=CARTESIAN_POINT ( 'NONE',  ( 12.49065589463330106, 1426.226283141350223, 200.9747314135889837 ) ) ;
#94044=CARTESIAN_POINT ( 'NONE',  ( 3.155009993958097336, 1508.551704391360545, 219.5005843085808692 ) ) ;
#94046=CARTESIAN_POINT ( 'NONE',  ( 10.75631870973100135, 1451.138109356459836, 190.3409054002840151 ) ) ;
#94048=CARTESIAN_POINT ( 'NONE',  ( -15.77321957905520122, 1420.788161934480058, 204.8879566011889892 ) ) ;
#94050=CARTESIAN_POINT ( 'NONE',  ( 5.170971366870000807, 1436.537220372990078, 207.3761814019889869 ) ) ;
#94056=CARTESIAN_POINT ( 'NONE',  ( -7.470275378713659542, 1508.551704408439946, 219.0703384621789951 ) ) ;
#94058=CARTESIAN_POINT ( 'NONE',  ( -10.19384471300000072, 1472.681895133989883, 209.3325899942670105 ) ) ;
#94062=CARTESIAN_POINT ( 'NONE',  ( 2.484221813290000025, 1505.974367507990110, 221.6747987149990138 ) ) ;
#94063=FACE_OUTER_BOUND ( 'NONE', #12255, .T. ) ;
#94070=CARTESIAN_POINT ( 'NONE',  ( 10.41307521078920040, 1422.727929710979879, 209.2808407624430060 ) ) ;
#94076=CARTESIAN_POINT ( 'NONE',  ( -18.35817859039589806, 1441.385501788960028, 212.7641934202129903 ) ) ;
#94078=FACE_OUTER_BOUND ( 'NONE', #80683, .T. ) ;
#94083=CARTESIAN_POINT ( 'NONE',  ( 5.235182724180000413, 1445.859873156990034, 201.6914249771490120 ) ) ;
#94086=CARTESIAN_POINT ( 'NONE',  ( -2.436662679049999891, 1455.201177966789828, 199.6236828809589952 ) ) ;
#94090=DIRECTION ( 'NONE',  ( 0.9352732527595466472, 0.3048504653312879564, 0.1798058298828889567 ) ) ;
#94092=CARTESIAN_POINT ( 'NONE',  ( 1.901527550710000014, 1494.834316974189960, 220.2474433046989759 ) ) ;
#94109=CARTESIAN_POINT ( 'NONE',  ( 4.038129178976070044, 1508.551704408389924, 213.5713170429240222 ) ) ;
#94111=VERTEX_POINT ( 'NONE', #22831 ) ;
#94113=CARTESIAN_POINT ( 'NONE',  ( 9.990133414916458676, 1460.215732121300107, 206.0067476231430135 ) ) ;
#94114=EDGE_CURVE ( 'NONE', #18354, #79507, #8243, .T. ) ;
#94120=EDGE_CURVE ( 'NONE', #2979, #22353, #16139, .T. ) ;
#94121=CARTESIAN_POINT ( 'NONE',  ( -7.274316450086129926, 1508.306618212879812, 219.8289394896960118 ) ) ;
#94122=CARTESIAN_POINT ( 'NONE',  ( -11.07029335559397509, 1417.884409290571966, 198.4126321785992388 ) ) ;
#94128=CARTESIAN_POINT ( 'NONE',  ( 9.407380373042538935, 1451.375700834039890, 208.8070606591070089 ) ) ;
#94131=ORIENTED_EDGE ( 'NONE', *, *, #49160, .F. ) ;
#94144=CARTESIAN_POINT ( 'NONE',  ( -10.13245345400000019, 1472.295918207390059, 207.1576006814689777 ) ) ;
#94149=CARTESIAN_POINT ( 'NONE',  ( 8.721463030380689929, 1468.435740110270217, 202.0638425475829933 ) ) ;
#94152=CARTESIAN_POINT ( 'NONE',  ( -8.123539286424179551, 1500.423757730580064, 210.2681710058099895 ) ) ;
#94159=CARTESIAN_POINT ( 'NONE',  ( -14.20591846559999993, 1415.677402202029953, 213.6695356306190092 ) ) ;
#94160=CARTESIAN_POINT ( 'NONE',  ( 0.3770322116046740391, 1515.150283736280016, 204.7946358424930224 ) ) ;
#94168=CARTESIAN_POINT ( 'NONE',  ( -4.868096759910030435, 1427.828191610080012, 201.1376980637430165 ) ) ;
#94171=FACE_OUTER_BOUND ( 'NONE', #10487, .T. ) ;
#94172=CARTESIAN_POINT ( 'NONE',  ( -11.87328667094049983, 1482.014090395339963, 208.6022402748390050 ) ) ;
#94185=CARTESIAN_POINT ( 'NONE',  ( -14.24607136059999846, 1416.872397861769969, 203.2551075799290174 ) ) ;
#94187=CARTESIAN_POINT ( 'NONE',  ( -4.664452821781310377, 1485.067080777090041, 198.1685467601409982 ) ) ;
#94188=CARTESIAN_POINT ( 'NONE',  ( 17.68711869539999881, 1428.828027849089949, 204.9896315466789929 ) ) ;
#94191=CARTESIAN_POINT ( 'NONE',  ( -1.805659813559999938, 1477.256586422089867, 201.7144240183190220 ) ) ;
#94193=CARTESIAN_POINT ( 'NONE',  ( -12.38301933211369921, 1507.638490190219954, 208.9814132950569956 ) ) ;
#94194=CARTESIAN_POINT ( 'NONE',  ( -15.23237985030026564, 1418.498831278173157, 202.0311994841594867 ) ) ;
#94211=CARTESIAN_POINT ( 'NONE',  ( 11.35868560929959870, 1433.949220014620096, 225.7806587185430089 ) ) ;
#94213=CARTESIAN_POINT ( 'NONE',  ( -4.354845126375000319, 1481.954762872750052, 231.1149980757659819 ) ) ;
#94217=CARTESIAN_POINT ( 'NONE',  ( 9.811585304708989597, 1435.742264125679867, 209.6664975758049820 ) ) ;
#94218=CARTESIAN_POINT ( 'NONE',  ( -11.04520924769999901, 1490.920650304590026, 210.5690864859589908 ) ) ;
#94220=CARTESIAN_POINT ( 'NONE',  ( 6.177122345705179818, 1447.962585782399856, 200.9448045309679856 ) ) ;
#94227=CARTESIAN_POINT ( 'NONE',  ( 6.347281094337080098, 1505.438767865790169, 219.0712605421129808 ) ) ;
#94228=CARTESIAN_POINT ( 'NONE',  ( -14.35646903299999799, 1420.584115152450067, 213.7701001417389932 ) ) ;
#94231=EDGE_LOOP ( 'NONE', ( #92892, #87516, #105797, #108869, #79488, #67545, #29945, #103588, #98417, #98975, #72048, #85401, #6929, #55803 ) ) ;
#94243=CARTESIAN_POINT ( 'NONE',  ( 5.826428076080000906, 1473.811884028689974, 218.9454251420289950 ) ) ;
#94247=CARTESIAN_POINT ( 'NONE',  ( 5.532282644110000369, 1438.101548174390018, 209.4569669639380152 ) ) ;
#94257=CARTESIAN_POINT ( 'NONE',  ( -4.958564224928870168, 1476.141795758730041, 200.0452580833139962 ) ) ;
#94260=CARTESIAN_POINT ( 'NONE',  ( -19.84400731930000106, 1467.319027288089956, 208.1478232803480068 ) ) ;
#94261=CARTESIAN_POINT ( 'NONE',  ( 11.89841253197050008, 1421.888142385570063, 209.0481693330570181 ) ) ;
#94273=CARTESIAN_POINT ( 'NONE',  ( -3.732259305638550018, 1433.538075186169863, 217.9425128220690056 ) ) ;
#94276=CARTESIAN_POINT ( 'NONE',  ( -15.74454477997780089, 1508.551704408389924, 210.3741846618140130 ) ) ;
#94277=CARTESIAN_POINT ( 'NONE',  ( 5.662343758720000508, 1504.894618425089902, 220.5557215505990314 ) ) ;
#94282=CARTESIAN_POINT ( 'NONE',  ( -3.241666583938100032, 1428.785741415590110, 200.3354813264270149 ) ) ;
#94297=VECTOR ( 'NONE', #92109, 1000.000000000000000 ) ;
#94308=DIRECTION ( 'NONE',  ( 0.9824080081115912355, 0.000000000000000000, 0.1867471702549089174 ) ) ;
#94309=CARTESIAN_POINT ( 'NONE',  ( 3.554051323329999956, 1466.352086058089981, 219.5854740514990056 ) ) ;
#94310=CARTESIAN_POINT ( 'NONE',  ( 2.167844020415154560, 1468.694760366214268, 218.9020797896687327 ) ) ;
#94314=CARTESIAN_POINT ( 'NONE',  ( -1.848575068539999977, 1431.426229023689984, 200.9261770996690188 ) ) ;
#94315=CARTESIAN_POINT ( 'NONE',  ( 10.52417073115330126, 1481.313718111980052, 210.1442249564590270 ) ) ;
#94318=CARTESIAN_POINT ( 'NONE',  ( -2.086548178679999754, 1515.551704408389924, 212.9514660752490158 ) ) ;
#94322=CARTESIAN_POINT ( 'NONE',  ( 11.39903530061180170, 1471.112746094619979, 209.6182361319149834 ) ) ;
#94325=CARTESIAN_POINT ( 'NONE',  ( 12.17208542549999883, 1501.180003388690011, 210.7301006051390004 ) ) ;
#94326=CARTESIAN_POINT ( 'NONE',  ( -6.919353105000337401, 1470.289799349278837, 190.2359701780528383 ) ) ;
#94328=CARTESIAN_POINT ( 'NONE',  ( 8.625843005480000159, 1428.332922249990133, 213.2805166664589933 ) ) ;
#94332=CARTESIAN_POINT ( 'NONE',  ( -7.288035249400000026, 1483.352442713390019, 201.0303113485389872 ) ) ;
#94338=VERTEX_POINT ( 'NONE', #104532 ) ;
#94340=CARTESIAN_POINT ( 'NONE',  ( 0.2132038637309990048, 1494.307031516189909, 217.5014853844989773 ) ) ;
#94343=CARTESIAN_POINT ( 'NONE',  ( -1.171005540028109859, 1457.331745760810236, 219.6985076373949823 ) ) ;
#94348=CARTESIAN_POINT ( 'NONE',  ( 18.99431323780000014, 1459.501207708489801, 220.3864241394989847 ) ) ;
#94352=CARTESIAN_POINT ( 'NONE',  ( 3.076465250140000052, 1495.499561967389809, 221.1031209306989638 ) ) ;
#94356=B_SPLINE_CURVE_WITH_KNOTS ( 'NONE', 5,
 ( #87259, #44725, #96212, #19487, #106799, #31199 ),
 .UNSPECIFIED., .F., .F.,
 ( 6, 6 ),
 ( 363.0445097500000315, 368.0632323040000529 ),
 .UNSPECIFIED. ) ;
#94357=CARTESIAN_POINT ( 'NONE',  ( -21.62191568639999772, 1508.114882721290087, 209.5578768717909668 ) ) ;
#94359=CARTESIAN_POINT ( 'NONE',  ( 9.088475950640962253, 1500.760587046248929, 202.1887800772891808 ) ) ;
#94362=CARTESIAN_POINT ( 'NONE',  ( 0.3658621740327940297, 1475.868828734210183, 197.6638016826259729 ) ) ;
#94375=AXIS2_PLACEMENT_3D ( 'NONE', #3333, #98452, #4416 ) ;
#94384=CIRCLE ( 'NONE', #55113, 0.4999999999999449329 ) ;
#94397=CARTESIAN_POINT ( 'NONE',  ( -10.37617513879240150, 1479.403831811299824, 210.6295454707710064 ) ) ;
#94406=ORIENTED_EDGE ( 'NONE', *, *, #69502, .T. ) ;
#94412=CARTESIAN_POINT ( 'NONE',  ( -3.802211600920000212, 1430.235143476489839, 201.6995583931590090 ) ) ;
#94416=B_SPLINE_CURVE_WITH_KNOTS ( 'NONE', 3,
 ( #54830, #30139, #11171, #46978, #38011, #81102, #45331, #79470, #72192, #106311, #54288, #88411, #57033, #40757, #99544, #14985, #82201, #41318, #32364, #108514, #92261, #4945, #101192, #73831, #6607, #83311, #49181, #91160, #13881, #15532, #39663, #14435, #40207, #58128 ),
 .UNSPECIFIED., .F., .F.,
 ( 4, 3, 3, 3, 3, 3, 3, 3, 3, 3, 3, 4 ),
 ( -1.999999997816839903, -1.865374217096350096, -1.681834405945489941, -1.496047443713429903, -1.309079570038079954, -1.120656966309940161, -0.9318186706558500010, -0.7430292649658170046, -0.5547479918945381616, -0.3681582181805309606, -0.1831547726995599312, 0.000000000000000000 ),
 .UNSPECIFIED. ) ;
#94419=CARTESIAN_POINT ( 'NONE',  ( 3.427508779931670357, 1430.651858238479917, 217.9719317096229929 ) ) ;
#94431=CARTESIAN_POINT ( 'NONE',  ( -12.61766350599999953, 1502.778797914289953, 208.5850585992880042 ) ) ;
#94433=CARTESIAN_POINT ( 'NONE',  ( 2.901791247649999850, 1441.419505434789926, 218.6084270491589905 ) ) ;
#94438=CARTESIAN_POINT ( 'NONE',  ( 8.787489738345170665, 1459.851268306849988, 204.0738034033330166 ) ) ;
#94441=CARTESIAN_POINT ( 'NONE',  ( -8.867713673612659164, 1420.193669887999931, 195.6881175697860158 ) ) ;
#94443=DIRECTION ( 'NONE',  ( 0.000000000000000000, 1.000000000000000000, 0.000000000000000000 ) ) ;
#94447=CARTESIAN_POINT ( 'NONE',  ( -4.329448776040000446, 1515.064792882589927, 207.2788837304390199 ) ) ;
#94450=CARTESIAN_POINT ( 'NONE',  ( -10.50924080488429979, 1480.092739868610124, 208.7673280485799978 ) ) ;
#94461=CARTESIAN_POINT ( 'NONE',  ( -8.590718235127866365, 1437.541524225612193, 210.2462751636549569 ) ) ;
#94471=VERTEX_POINT ( 'NONE', #81515 ) ;
#94472=EDGE_LOOP ( 'NONE', ( #7864, #19577, #59515, #84182 ) ) ;
#94478=CARTESIAN_POINT ( 'NONE',  ( 8.663291285446870660, 1437.708809294000048, 209.4154668070010246 ) ) ;
#94484=CARTESIAN_POINT ( 'NONE',  ( 0.1984908215090459838, 1486.169885337769983, 197.2145582505330026 ) ) ;
#94486=CARTESIAN_POINT ( 'NONE',  ( -9.163589329508671000, 1449.727551480139937, 209.8107205256980023 ) ) ;
#94491=CARTESIAN_POINT ( 'NONE',  ( -4.410745166166390341, 1508.610338516509955, 212.9873992348109937 ) ) ;
#94492=CARTESIAN_POINT ( 'NONE',  ( 11.06889095329999861, 1479.888754528190020, 229.8106084604989974 ) ) ;
#94495=PLANE ( 'NONE',  #12288 ) ;
#94497=CARTESIAN_POINT ( 'NONE',  ( -16.86523139679999872, 1468.641458686789974, 198.2210143100990081 ) ) ;
#94508=CARTESIAN_POINT ( 'NONE',  ( -8.097513007330000789, 1424.669315053030004, 209.4052413237879762 ) ) ;
#94510=ORIENTED_EDGE ( 'NONE', *, *, #8261, .T. ) ;
#94513=CARTESIAN_POINT ( 'NONE',  ( -9.385572798718857968, 1471.838051314206268, 213.1320772043752072 ) ) ;
#94514=CARTESIAN_POINT ( 'NONE',  ( 7.510429961322310888, 1425.933150149150151, 212.2881029679170126 ) ) ;
#94523=CARTESIAN_POINT ( 'NONE',  ( -4.772433264290000032, 1461.586210710390105, 228.1254610687989839 ) ) ;
#94537=AXIS2_PLACEMENT_3D ( 'NONE', #76605, #95068, #43567 ) ;
#94541=VECTOR ( 'NONE', #110271, 1000.000000000000114 ) ;
#94553=CARTESIAN_POINT ( 'NONE',  ( -4.948068031382700127, 1508.551704408389924, 212.0494981076920169 ) ) ;
#94555=CARTESIAN_POINT ( 'NONE',  ( 7.463794710130000176, 1422.976950754710060, 195.6323374253989869 ) ) ;
#94566=ADVANCED_FACE ( 'NONE', ( #20502 ), #63663, .T. ) ;
#94568=ORIENTED_EDGE ( 'NONE', *, *, #44686, .T. ) ;
#94573=CARTESIAN_POINT ( 'NONE',  ( -0.1602782174031799067, 1421.018467852183903, 193.7178847131137047 ) ) ;
#94581=CARTESIAN_POINT ( 'NONE',  ( -16.89200104021849924, 1419.273703591249841, 201.3369295748360059 ) ) ;
#94588=CARTESIAN_POINT ( 'NONE',  ( -8.040086649609909486, 1425.809972356560820, 207.7969723859449687 ) ) ;
#94590=CARTESIAN_POINT ( 'NONE',  ( -0.6463351481710662982, 1477.515498289491234, 198.7392143834898661 ) ) ;
#94592=CARTESIAN_POINT ( 'NONE',  ( 3.406450987864870328, 1507.508084575899829, 220.3277226881679951 ) ) ;
#94593=ADVANCED_FACE ( 'NONE', ( #35095 ), #59766, .T. ) ;
#94594=CARTESIAN_POINT ( 'NONE',  ( -4.705736713569160123, 1479.984769566100113, 230.9466532730550057 ) ) ;
#94596=CARTESIAN_POINT ( 'NONE',  ( -10.59625218578830008, 1423.662071466640100, 204.3772360533070014 ) ) ;
#94599=CARTESIAN_POINT ( 'NONE',  ( 5.365832140090000202, 1437.051389308390071, 208.1168906416689879 ) ) ;
#94604=FACE_OUTER_BOUND ( 'NONE', #61466, .T. ) ;
#94607=CARTESIAN_POINT ( 'NONE',  ( 4.677526816337639559, 1434.888920963079954, 228.7640148925319750 ) ) ;
#94609=B_SPLINE_SURFACE_WITH_KNOTS ( 'NONE', 5, 1, ( 
 ( #31956, #73430 ),
 ( #106467, #90197 ),
 ( #66149, #91864 ),
 ( #38700, #23552 ),
 ( #31403, #89657 ),
 ( #57743, #15137 ),
 ( #107564, #12943 ),
 ( #80721, #4029 ),
 ( #99144, #98053 ) ),
 .UNSPECIFIED., .F., .F., .F.,
 ( 6, 3, 6 ),
 ( 2, 2 ),
 ( 0.000000000000000000, 3.695647608739999868, 7.374251186729999574 ),
 ( 0.000000000000000000, 14.00000000000000000 ),
 .UNSPECIFIED. ) ;
#94612=CARTESIAN_POINT ( 'NONE',  ( 9.046284717930422659, 1449.608882353234549, 207.3630802585645938 ) ) ;
#94613=CARTESIAN_POINT ( 'NONE',  ( -3.313501335607589748, 1397.551704408390151, 203.0565224509919915 ) ) ;
#94614=CARTESIAN_POINT ( 'NONE',  ( -4.881632653818110512, 1434.082703436370139, 217.0349096382250025 ) ) ;
#94618=CARTESIAN_POINT ( 'NONE',  ( -16.26800630319999641, 1422.453322322420036, 210.2998271891489992 ) ) ;
#94624=CARTESIAN_POINT ( 'NONE',  ( 10.62762824711120224, 1422.391620394080064, 210.1053338132739725 ) ) ;
#94630=CARTESIAN_POINT ( 'NONE',  ( 6.970868710793260092, 1466.504179844829878, 216.1871911102630008 ) ) ;
#94633=CARTESIAN_POINT ( 'NONE',  ( 19.32263322520000060, 1455.378559704889767, 209.1218459616989946 ) ) ;
#94635=CARTESIAN_POINT ( 'NONE',  ( -11.37447413379999972, 1491.756880625089934, 205.6190363507990071 ) ) ;
#94639=CARTESIAN_POINT ( 'NONE',  ( -9108.204429824800172, -2340.220200558880151, -1569.808522337019895 ) ) ;
#94645=CARTESIAN_POINT ( 'NONE',  ( 1.779428958460000265, 1456.357349049189907, 198.6855221643990035 ) ) ;
#94650=B_SPLINE_SURFACE_WITH_KNOTS ( 'NONE', 5, 1, ( 
 ( #34603, #58167 ),
 ( #41907, #77719 ),
 ( #68789, #102350 ),
 ( #16664, #94497 ),
 ( #76607, #50861 ),
 ( #32937, #26186 ),
 ( #60376, #17768 ),
 ( #51972, #9407 ),
 ( #37374, #45243 ) ),
 .UNSPECIFIED., .F., .F., .F.,
 ( 6, 3, 6 ),
 ( 2, 2 ),
 ( 0.000000000000000000, 8.334083717689999560, 16.69887895509999964 ),
 ( 0.000000000000000000, 14.00000000000000000 ),
 .UNSPECIFIED. ) ;
#94652=CARTESIAN_POINT ( 'NONE',  ( -3.370189795129999943, 1496.076862149890076, 198.0269955820990049 ) ) ;
#94653=CARTESIAN_POINT ( 'NONE',  ( -2.231199251659999661, 1495.993596543689819, 220.2514328137989992 ) ) ;
#94669=CARTESIAN_POINT ( 'NONE',  ( -5.076113882490000506, 1391.871667423589997, 214.6636951175890147 ) ) ;
#94673=CARTESIAN_POINT ( 'NONE',  ( -19.52647806210000070, 1464.795176723290069, 212.0690861509589809 ) ) ;
#94681=CARTESIAN_POINT ( 'NONE',  ( -9.765242783855931918, 1418.346146421839194, 197.2107663835972176 ) ) ;
#94684=DIRECTION ( 'NONE',  ( 0.9824080081115912355, 0.000000000000000000, 0.1867471702549089174 ) ) ;
#94686=CARTESIAN_POINT ( 'NONE',  ( 9.194133702223101778, 1450.204357222580029, 208.5217520979160213 ) ) ;
#94689=VERTEX_POINT ( 'NONE', #60884 ) ;
#94699=CARTESIAN_POINT ( 'NONE',  ( -9.816650044347928983, 1461.735905517830133, 208.1390970106120051 ) ) ;
#94703=CARTESIAN_POINT ( 'NONE',  ( 4.487357219410602838, 1509.034509700537683, 206.0057024814164777 ) ) ;
#94704=CARTESIAN_POINT ( 'NONE',  ( -6.479645409570000680, 1473.991665852890037, 200.1438768917790014 ) ) ;
#94707=CARTESIAN_POINT ( 'NONE',  ( -4.503834590931400150, 1496.999185789959938, 198.8010291948349959 ) ) ;
#94714=AXIS2_PLACEMENT_3D ( 'NONE', #13306, #81625, #91140 ) ;
#94716=DIRECTION ( 'NONE',  ( -1.000000000000000000, 0.000000000000000000, 0.000000000000000000 ) ) ;
#94719=CARTESIAN_POINT ( 'NONE',  ( 0.5750010241369649666, 1515.139742041519867, 204.7943597985580197 ) ) ;
#94722=CARTESIAN_POINT ( 'NONE',  ( -2.163895355619999794, 1508.493132411889974, 220.4958316090989854 ) ) ;
#94726=CARTESIAN_POINT ( 'NONE',  ( -10.76971639860709828, 1461.755917255409940, 211.3234507930380062 ) ) ;
#94727=CARTESIAN_POINT ( 'NONE',  ( -4.993214560040000194, 1391.653934889589891, 203.5347113830289913 ) ) ;
#94732=CARTESIAN_POINT ( 'NONE',  ( -11.31630330039999954, 1480.636685083989732, 212.6825498069390221 ) ) ;
#94748=CARTESIAN_POINT ( 'NONE',  ( -3.703568358935259930, 1497.311626042180023, 220.9591690318370070 ) ) ;
#94749=CARTESIAN_POINT ( 'NONE',  ( 18.20044471017449794, 1429.674601861270048, 208.8920640582719841 ) ) ;
#94752=EDGE_CURVE ( 'NONE', #106368, #27485, #17534, .T. ) ;
#94756=CARTESIAN_POINT ( 'NONE',  ( -11.62069880129860167, 1507.830664569160263, 207.5518378911060040 ) ) ;
#94766=EDGE_CURVE ( 'NONE', #41878, #42556, #10835, .T. ) ;
#94772=CARTESIAN_POINT ( 'NONE',  ( 3.645289263010000003, 1485.122998769089918, 219.6252413598990074 ) ) ;
#94774=CARTESIAN_POINT ( 'NONE',  ( 10.63291962098290000, 1480.187357847879866, 208.2421106722409831 ) ) ;
#94775=B_SPLINE_SURFACE_WITH_KNOTS ( 'NONE', 5, 5, ( 
 ( #107454, #93810, #81690, #106901, #7620, #59697 ),
 ( #98502, #33363, #13378, #30187, #30749, #42331 ),
 ( #41778, #84330, #48122, #4997, #16002, #73317 ),
 ( #17089, #55971, #93277, #82261, #64930, #50731 ),
 ( #73876, #67004, #21770, #110635, #51281, #99043 ),
 ( #67556, #64380, #32817, #90095, #22321, #76483 ),
 ( #56523, #39712, #90650, #101114, #5561, #84864 ),
 ( #108004, #24410, #101659, #50205, #58595, #92726 ),
 ( #75933, #8162, #33920, #68115, #4465, #102228 ) ),
 .UNSPECIFIED., .F., .F., .F.,
 ( 6, 3, 6 ),
 ( 6, 6 ),
 ( 2.932875705070239647, 5.043863234400000728, 7.154850763719760032 ),
 ( -0.0004325517097626320083, 2.000000000000000000 ),
 .UNSPECIFIED. ) ;
#94777=CARTESIAN_POINT ( 'NONE',  ( -3.250062279909999852, 1451.275148989389891, 188.5377248918989892 ) ) ;
#94778=CARTESIAN_POINT ( 'NONE',  ( -4.019735481675231092, 1515.589562461625064, 209.7439076584321356 ) ) ;
#94779=CARTESIAN_POINT ( 'NONE',  ( -22.15968219182800070, 1485.573411980050196, 217.2083784210080069 ) ) ;
#94785=CARTESIAN_POINT ( 'NONE',  ( -10.81369826949999968, 1491.706306174490010, 211.2949660241190202 ) ) ;
#94792=CARTESIAN_POINT ( 'NONE',  ( 16.68551868298740004, 1431.393131126370008, 216.7641592467800251 ) ) ;
#94794=EDGE_CURVE ( 'NONE', #108598, #62493, #93746, .T. ) ;
#94797=CARTESIAN_POINT ( 'NONE',  ( -11.36959371680000075, 1503.847165134090119, 207.0750569533189775 ) ) ;
#94805=CARTESIAN_POINT ( 'NONE',  ( -10.36148874078660143, 1447.909434907649938, 209.3402815508519836 ) ) ;
#94806=CARTESIAN_POINT ( 'NONE',  ( 4.138326087764579775, 1515.492270357739926, 206.7919250688289878 ) ) ;
#94807=CARTESIAN_POINT ( 'NONE',  ( -0.6816155568609990612, 1444.074492657990049, 199.8235773416689938 ) ) ;
#94808=EDGE_CURVE ( 'NONE', #54763, #2539, #91571, .T. ) ;
#94811=CARTESIAN_POINT ( 'NONE',  ( 2.035491882000000086, 1468.277065364090276, 218.9268452469790134 ) ) ;
#94815=CARTESIAN_POINT ( 'NONE',  ( -7.469914488626709925, 1425.609915395969892, 205.2032434723799952 ) ) ;
#94825=CARTESIAN_POINT ( 'NONE',  ( -8.332436002999379809, 1474.689645896253978, 203.1022837292814245 ) ) ;
#94827=CARTESIAN_POINT ( 'NONE',  ( 1.483134297318269956, 1465.770756053359946, 198.2023842196989847 ) ) ;
#94828=B_SPLINE_CURVE_WITH_KNOTS ( 'NONE', 3,
 ( #30564, #73127, #30000, #21592, #56882, #14302, #91013, #64191, #32221, #38406, #98313, #31661, #65841, #90461, #108379, #31112, #100521, #66402, #72582, #40069, #22683, #74790, #15401 ),
 .UNSPECIFIED., .F., .F.,
 ( 4, 2, 2, 2, 1, 1, 1, 1, 1, 2, 2, 2, 2, 4 ),
 ( 0.000000000000000000, 0.2499999999977853271, 0.3749999999966871500, 0.4374999999961360908, 0.4687499999958624763, 0.4843749999957339125, 0.4921874999956594166, 0.4960937499956221131, 0.4980468749956012409, 0.4990234374955930807, 0.4999999999955848651, 0.7499999999977895460, 0.8749999999988947730, 1.000000000000000000 ),
 .UNSPECIFIED. ) ;
#94829=CARTESIAN_POINT ( 'NONE',  ( 12.06000798031920063, 1421.818391337039884, 208.6542734367120033 ) ) ;
#94831=CARTESIAN_POINT ( 'NONE',  ( 2.402586825280000227, 1466.023001228489875, 198.3390201041990224 ) ) ;
#94835=ORIENTED_EDGE ( 'NONE', *, *, #9898, .F. ) ;
#94843=CARTESIAN_POINT ( 'NONE',  ( 3.900198121993049938, 1423.884075158320002, 192.9473687097540164 ) ) ;
#94851=B_SPLINE_CURVE_WITH_KNOTS ( 'NONE', 3,
 ( #103735, #85824, #94778, #9122, #52250, #33754 ),
 .UNSPECIFIED., .F., .F.,
 ( 4, 2, 4 ),
 ( 0.000000000000000000, 0.5000000000000000000, 1.000000000000000000 ),
 .UNSPECIFIED. ) ;
#94861=ORIENTED_EDGE ( 'NONE', *, *, #78909, .T. ) ;
#94868=B_SPLINE_CURVE_WITH_KNOTS ( 'NONE', 3,
 ( #40775, #93918, #67104, #26161, #34576, #102864, #92276, #7178, #93371, #49745, #14998, #76034, #7717 ),
 .UNSPECIFIED., .F., .F.,
 ( 4, 3, 3, 3, 4 ),
 ( -6.749361107549999517, -5.746593412767809994, -4.743825717985610702, -3.763266661680000347, -2.767901846390000031 ),
 .UNSPECIFIED. ) ;
#94871=CARTESIAN_POINT ( 'NONE',  ( -10.33297333698109988, 1447.717229192940067, 209.8087386623969905 ) ) ;
#94877=CARTESIAN_POINT ( 'NONE',  ( 10.78159844869479933, 1461.896569297480028, 211.1674770051990038 ) ) ;
#94879=DIRECTION ( 'NONE',  ( 0.000000000000000000, 1.000000000000000000, 0.000000000000000000 ) ) ;
#94880=CARTESIAN_POINT ( 'NONE',  ( 2.175409717514719593E-31, 1397.551704408390151, 209.1218459616989946 ) ) ;
#94881=CARTESIAN_POINT ( 'NONE',  ( 3.578848130929999982, 1466.803391000889860, 218.7998462970390108 ) ) ;
#94882=CARTESIAN_POINT ( 'NONE',  ( 3.919629339340000573, 1445.919245566989957, 204.1216026806789898 ) ) ;
#94889=CARTESIAN_POINT ( 'NONE',  ( 1.011935686670000001, 1508.279717064390070, 220.8600042037990079 ) ) ;
#94890=CIRCLE ( 'NONE', #105853, 11.23850026409999892 ) ;
#94895=CARTESIAN_POINT ( 'NONE',  ( 2.759147620390000277, 1485.169339790590129, 198.7305754187989919 ) ) ;
#94899=CARTESIAN_POINT ( 'NONE',  ( 12.08289755050000025, 1501.361268123389891, 211.3149880542889889 ) ) ;
#94902=CARTESIAN_POINT ( 'NONE',  ( 9.067034957830001574, 1422.697473312089869, 213.1748827745390145 ) ) ;
#94907=CARTESIAN_POINT ( 'NONE',  ( -8.160121199729999830, 1484.191520557689955, 200.3086294344790019 ) ) ;
#94916=CARTESIAN_POINT ( 'NONE',  ( -12.16304787920000052, 1501.912848009289746, 211.0099873911190116 ) ) ;
#94917=CARTESIAN_POINT ( 'NONE',  ( -14.59132467482771212, 1416.165632769844024, 204.1513725631303942 ) ) ;
#94919=CARTESIAN_POINT ( 'NONE',  ( -9.792917003243150731, 1438.431876507500192, 210.7357112484050106 ) ) ;
#94920=CARTESIAN_POINT ( 'NONE',  ( 2.963633255220000429, 1451.607057905790043, 190.1601877849990103 ) ) ;
#94923=CARTESIAN_POINT ( 'NONE',  ( 7.490423649669999406, 1425.310147181990033, 212.2658099247589973 ) ) ;
#94924=CARTESIAN_POINT ( 'NONE',  ( 18.28863238269999769, 1430.119121229389975, 201.0315571599689974 ) ) ;
#94927=EDGE_CURVE ( 'NONE', #34771, #77131, #43099, .T. ) ;
#94929=CARTESIAN_POINT ( 'NONE',  ( 5.456719627610000067, 1455.595244131089885, 218.2350948550090095 ) ) ;
#94930=VERTEX_POINT ( 'NONE', #17587 ) ;
#94933=CARTESIAN_POINT ( 'NONE',  ( -21.53008337650500081, 1505.945960034420068, 209.1889141163210013 ) ) ;
#94937=EDGE_CURVE ( 'NONE', #18354, #103670, #32216, .T. ) ;
#94953=CARTESIAN_POINT ( 'NONE',  ( -3.179033943583710276, 1457.997354099609993, 219.3203918230290128 ) ) ;
#94970=CARTESIAN_POINT ( 'NONE',  ( -10.55952072472410030, 1471.180150025179955, 209.5617685359960092 ) ) ;
#94975=CARTESIAN_POINT ( 'NONE',  ( -6.711262841758562914, 1442.278122625611786, 201.5834799348254194 ) ) ;
#95004=ORIENTED_EDGE ( 'NONE', *, *, #108164, .T. ) ;
#95011=UNCERTAINTY_MEASURE_WITH_UNIT (LENGTH_MEASURE( 1.000000000000000082E-05 ), #5435, 'distance_accuracy_value', 'NONE');
#95012=CARTESIAN_POINT ( 'NONE',  ( 3.314835131729999773, 1443.023294147790011, 217.3780381071989893 ) ) ;
#95017=CARTESIAN_POINT ( 'NONE',  ( -4.772204876747930591, 1456.966521863563912, 217.3851231261082262 ) ) ;
#95019=FACE_OUTER_BOUND ( 'NONE', #109694, .T. ) ;
#95021=DIRECTION ( 'NONE',  ( 1.224646799147353207E-16, -1.836970198721029688E-16, -1.000000000000000000 ) ) ;
#95031=CARTESIAN_POINT ( 'NONE',  ( -4.635215035006506668, 1377.957596388888533, 204.0719524705168624 ) ) ;
#95032=CARTESIAN_POINT ( 'NONE',  ( -17.11733429290000075, 1420.830776148560062, 201.6585816624789800 ) ) ;
#95039=CARTESIAN_POINT ( 'NONE',  ( 10.57019798174319902, 1452.578602367869962, 209.5296950901719981 ) ) ;
#95043=CARTESIAN_POINT ( 'NONE',  ( -14.68737671657240007, 1419.645626571690173, 213.7540033288840107 ) ) ;
#95052=CARTESIAN_POINT ( 'NONE',  ( 9.782549294074950552, 1435.950597167319984, 210.1455436486230042 ) ) ;
#95055=FACE_OUTER_BOUND ( 'NONE', #17092, .T. ) ;
#95058=CARTESIAN_POINT ( 'NONE',  ( 2.502839789385249869, 1486.822988642699784, 197.4474283702710125 ) ) ;
#95060=CARTESIAN_POINT ( 'NONE',  ( -9.188196878108460197, 1450.454516124349993, 208.3425459881050017 ) ) ;
#95061=CARTESIAN_POINT ( 'NONE',  ( -11.61130078636250040, 1423.105448014539888, 204.1619613308869816 ) ) ;
#95064=ORIENTED_EDGE ( 'NONE', *, *, #24232, .F. ) ;
#95065=CARTESIAN_POINT ( 'NONE',  ( -4.303235405216489617, 1508.728291632010041, 212.9102526658959960 ) ) ;
#95066=CARTESIAN_POINT ( 'NONE',  ( 18.43405782060979803, 1472.181634805399881, 195.1578483246480005 ) ) ;
#95068=DIRECTION ( 'NONE',  ( -1.699538841806929935E-33, 1.000000000000000000, -1.698192320643030073E-16 ) ) ;
#95081=CARTESIAN_POINT ( 'NONE',  ( -8.759598966840000500, 1423.140078425670026, 210.5148996192390030 ) ) ;
#95085=CARTESIAN_POINT ( 'NONE',  ( 7.538438372221369477, 1425.706950029929885, 212.1947421841360040 ) ) ;
#95092=CARTESIAN_POINT ( 'NONE',  ( -0.4827268496605868764, 1487.916102923474682, 219.9679759818499747 ) ) ;
#95095=CARTESIAN_POINT ( 'NONE',  ( -9.084504854676080043, 1439.262540927600185, 207.9197032644189846 ) ) ;
#95107=CARTESIAN_POINT ( 'NONE',  ( 12.18695065166680358, 1473.011202655907937, 192.8237078935919158 ) ) ;
#95121=CARTESIAN_POINT ( 'NONE',  ( 4.410745166166449849, 1508.610338516509955, 205.2562926885780143 ) ) ;
#95122=ADVANCED_FACE ( 'NONE', ( #18701 ), #61030, .T. ) ;
#95125=CARTESIAN_POINT ( 'NONE',  ( -4.980141907650089905, 1508.551704408389924, 211.7958595151590089 ) ) ;
#95140=CARTESIAN_POINT ( 'NONE',  ( -7.611722247467775482, 1464.044227469945326, 227.3821205927781364 ) ) ;
#95144=CARTESIAN_POINT ( 'NONE',  ( -1.920602012799999869, 1420.567466289690174, 193.8392733480989989 ) ) ;
#95145=CARTESIAN_POINT ( 'NONE',  ( -4.327495487222860149, 1515.139385973079925, 208.5392436879629940 ) ) ;
#95151=CARTESIAN_POINT ( 'NONE',  ( -10.38333126256229910, 1461.681020311170187, 210.9775042442759911 ) ) ;
#95153=CARTESIAN_POINT ( 'NONE',  ( 14.20069603096709976, 1428.565903384720059, 195.1302447813920082 ) ) ;
#95154=CARTESIAN_POINT ( 'NONE',  ( 10.72410096480519925, 1421.781422562299895, 200.2028139908449873 ) ) ;
#95162=CARTESIAN_POINT ( 'NONE',  ( -16.80221138011627957, 1420.025806103657942, 208.0932244396257715 ) ) ;
#95164=CARTESIAN_POINT ( 'NONE',  ( -0.7442430207490000615, 1515.589102391990082, 205.1050341093590248 ) ) ;
#95166=CARTESIAN_POINT ( 'NONE',  ( 7.755379628513099810, 1459.738852961230123, 228.9106028297960052 ) ) ;
#95168=CARTESIAN_POINT ( 'NONE',  ( 1.326713953160000070, 1454.806608698389937, 218.4390644836289823 ) ) ;
#95170=CARTESIAN_POINT ( 'NONE',  ( 3.554603345999999942, 1442.390756379090135, 217.2531437058290180 ) ) ;
#95177=CARTESIAN_POINT ( 'NONE',  ( -5.000754081882999635, 1508.551704408389924, 219.6714415651769912 ) ) ;
#95182=CARTESIAN_POINT ( 'NONE',  ( 0.007371176946978959775, 1430.919077003989969, 217.6339654454789923 ) ) ;
#95183=CARTESIAN_POINT ( 'NONE',  ( -14.65245970860000035, 1420.119839379899986, 213.8659343334090011 ) ) ;
#95190=CARTESIAN_POINT ( 'NONE',  ( 10.85576822019209864, 1490.211973181020085, 207.6231814341079769 ) ) ;
#95191=CARTESIAN_POINT ( 'NONE',  ( -0.6259040480903699244, 1438.020704032760023, 227.6802023094499816 ) ) ;
#95192=ORIENTED_EDGE ( 'NONE', *, *, #7744, .T. ) ;
#95193=CARTESIAN_POINT ( 'NONE',  ( -19.27355791249999939, 1467.813399981289876, 204.3088842694490097 ) ) ;
#95197=CARTESIAN_POINT ( 'NONE',  ( -6.855565616159999820, 1494.715409694790196, 199.7515626485690063 ) ) ;
#95199=CARTESIAN_POINT ( 'NONE',  ( 11.45021740003180000, 1427.604960870419973, 209.5607445365500325 ) ) ;
#95202=CARTESIAN_POINT ( 'NONE',  ( 3.329658494789999867, 1445.620183534490025, 200.6158397099989941 ) ) ;
#95203=CARTESIAN_POINT ( 'NONE',  ( -8.655671105859999770, 1512.830360918489987, 210.0583268009119990 ) ) ;
#95205=CARTESIAN_POINT ( 'NONE',  ( -8.444049741005709819, 1488.605066998670054, 190.0484225089540189 ) ) ;
#95206=CARTESIAN_POINT ( 'NONE',  ( 1.676160982570000124, 1456.565164728689979, 199.0597759751990168 ) ) ;
#95213=CARTESIAN_POINT ( 'NONE',  ( 0.8661595920449980390, 1495.979405726489858, 221.4595168884989960 ) ) ;
#95227=CARTESIAN_POINT ( 'NONE',  ( -5.028437303939999659, 1391.796862042790053, 214.5333048971589847 ) ) ;
#95231=CARTESIAN_POINT ( 'NONE',  ( 9.475842709078071024, 1461.102026927640054, 206.4900463968490101 ) ) ;
#95233=ORIENTED_EDGE ( 'NONE', *, *, #31658, .T. ) ;
#95236=CARTESIAN_POINT ( 'NONE',  ( -1.748905610829809998, 1488.269106374019884, 219.8524659745219765 ) ) ;
#95240=EDGE_CURVE ( 'NONE', #105229, #25916, #53693, .T. ) ;
#95253=B_SPLINE_CURVE_WITH_KNOTS ( 'NONE', 3,
 ( #43002, #100136, #53630, #27849, #87203, #70435, #104554, #35689, #103994, #19429, #60355, #36801, #62030 ),
 .UNSPECIFIED., .F., .F.,
 ( 4, 3, 3, 3, 4 ),
 ( -25.27124713432710124, -24.90871837163620128, -23.58501801755940264, -23.26424315256220154, -21.89878892990000026 ),
 .UNSPECIFIED. ) ;
#95257=CARTESIAN_POINT ( 'NONE',  ( -7.701846892468879879, 1508.539045597550057, 219.2228727215799893 ) ) ;
#95260=CARTESIAN_POINT ( 'NONE',  ( -9.658472698806898293, 1461.210338549909920, 208.2934798919299908 ) ) ;
#95264=CARTESIAN_POINT ( 'NONE',  ( -12.78210459472699867, 1502.593308907019946, 209.4105061602950002 ) ) ;
#95265=CARTESIAN_POINT ( 'NONE',  ( -2.334596864402660010, 1422.040517539739994, 193.1911830680820117 ) ) ;
#95266=CARTESIAN_POINT ( 'NONE',  ( 14.91143818900724405, 1415.677402202029953, 209.1063111766177940 ) ) ;
#95267=CARTESIAN_POINT ( 'NONE',  ( 7.653195889217795589, 1423.477952156526044, 195.7103289535878332 ) ) ;
#95269=CARTESIAN_POINT ( 'NONE',  ( -21.58396545289999935, 1505.929462060390051, 209.1867379206110229 ) ) ;
#95276=EDGE_CURVE ( 'NONE', #53118, #21613, #76263, .T. ) ;
#95280=CARTESIAN_POINT ( 'NONE',  ( -14.58197489760000032, 1416.181292664740113, 214.1195166561190035 ) ) ;
#95281=EDGE_CURVE ( 'NONE', #24288, #72135, #97642, .T. ) ;
#95282=CARTESIAN_POINT ( 'NONE',  ( -0.7597457875130829708, 1515.127202858759802, 204.7940314484660007 ) ) ;
#95286=CARTESIAN_POINT ( 'NONE',  ( -16.32138437919999774, 1416.733793783010015, 208.9008268797709889 ) ) ;
#95288=CARTESIAN_POINT ( 'NONE',  ( -10.85709873899809885, 1461.880737148149819, 210.9081126214580024 ) ) ;
#95289=EDGE_CURVE ( 'NONE', #1678, #55998, #104426, .T. ) ;
#95295=CARTESIAN_POINT ( 'NONE',  ( -8.432300450239999634, 1478.613105400289896, 216.7664695459189943 ) ) ;
#95307=CARTESIAN_POINT ( 'NONE',  ( -15.42042112429999889, 1415.259230628689920, 208.9538274143839942 ) ) ;
#95310=CARTESIAN_POINT ( 'NONE',  ( 18.04903976654019715, 1429.245179625179844, 206.8954713348119867 ) ) ;
#95328=FACE_OUTER_BOUND ( 'NONE', #63584, .T. ) ;
#95331=EDGE_CURVE ( 'NONE', #102504, #34771, #56688, .T. ) ;
#95333=CARTESIAN_POINT ( 'NONE',  ( 3.513937425589999997, 1485.582095535989993, 219.4230302830989672 ) ) ;
#95334=CARTESIAN_POINT ( 'NONE',  ( 4.997209437610000471, 1423.732853852190146, 194.0938684716990110 ) ) ;
#95336=CARTESIAN_POINT ( 'NONE',  ( 0.6387483492823400333, 1461.179315971390224, 230.4375156181200168 ) ) ;
#95343=CARTESIAN_POINT ( 'NONE',  ( -10.55591960359999959, 1490.955095264389911, 212.1910566715390019 ) ) ;
#95346=EDGE_CURVE ( 'NONE', #2466, #51946, #28057, .T. ) ;
#95352=CARTESIAN_POINT ( 'NONE',  ( 9.444504587474009227, 1504.434930463329920, 216.0229134707260243 ) ) ;
#95361=CARTESIAN_POINT ( 'NONE',  ( -10.35873372929360059, 1448.228887144569853, 208.5914340594589760 ) ) ;
#95363=CARTESIAN_POINT ( 'NONE',  ( -1.208150493920000068, 1443.877570131390030, 199.8977866975789937 ) ) ;
#95368=CARTESIAN_POINT ( 'NONE',  ( 1.871223699670000018, 1467.140817989690049, 219.6429414212990139 ) ) ;
#95372=CARTESIAN_POINT ( 'NONE',  ( -9.238451120100068081, 1424.071832880570128, 206.1097894639889887 ) ) ;
#95377=CARTESIAN_POINT ( 'NONE',  ( -15.55153481088430034, 1441.783360245790163, 219.6938892586900067 ) ) ;
#95378=ORIENTED_EDGE ( 'NONE', *, *, #44686, .F. ) ;
#95384=CARTESIAN_POINT ( 'NONE',  ( -4.487249770485409961, 1509.038615931769982, 206.6339108289169815 ) ) ;
#95385=CARTESIAN_POINT ( 'NONE',  ( -1.773373219119749766, 1465.043355074880083, 198.2607089762770158 ) ) ;
#95411=CARTESIAN_POINT ( 'NONE',  ( -3.395951246300449977, 1428.698596373810233, 200.3955505136949853 ) ) ;
#95415=B_SPLINE_CURVE_WITH_KNOTS ( 'NONE', 5,
 ( #100492, #23773, #57960, #92093, #15371, #75853 ),
 .UNSPECIFIED., .F., .F.,
 ( 6, 6 ),
 ( 0.000000000000000000, 1.000000000000000000 ),
 .UNSPECIFIED. ) ;
#95416=CARTESIAN_POINT ( 'NONE',  ( -11.78939996719659966, 1482.318781070740215, 207.5200076686040234 ) ) ;
#95424=EDGE_CURVE ( 'NONE', #108761, #75688, #41350, .T. ) ;
#95425=B_SPLINE_CURVE_WITH_KNOTS ( 'NONE', 5,
 ( #91734, #99569, #72746, #91186, #106336, #56498, #100139, #29622, #98477 ),
 .UNSPECIFIED., .F., .F.,
 ( 6, 3, 6 ),
 ( -2.813093253849999975, -1.406546626929999988, 0.000000000000000000 ),
 .UNSPECIFIED. ) ;
#95429=CARTESIAN_POINT ( 'NONE',  ( -9.231300103966539439, 1449.703421660030017, 207.7615902039960076 ) ) ;
#95433=CARTESIAN_POINT ( 'NONE',  ( -12.15118411454099956, 1508.442498811720043, 217.6820456900339877 ) ) ;
#95443=CARTESIAN_POINT ( 'NONE',  ( 0.8927505473990010598, 1432.232264963090074, 200.7285312053789994 ) ) ;
#95444=CARTESIAN_POINT ( 'NONE',  ( 10.50094040442339960, 1481.402766154620167, 210.3929528566290230 ) ) ;
#95445=CARTESIAN_POINT ( 'NONE',  ( -1.137508020020000066, 1507.161920010990116, 221.5186969393989784 ) ) ;
#95446=LINE ( 'NONE', #94318, #106510 ) ;
#95451=CARTESIAN_POINT ( 'NONE',  ( 5.842913806858009984, 1467.176569223159959, 199.5123709362070201 ) ) ;
#95453=CARTESIAN_POINT ( 'NONE',  ( 11.85459483029999994, 1500.917689607990042, 208.6046481015860081 ) ) ;
#95455=CARTESIAN_POINT ( 'NONE',  ( 8.481741098329999673, 1422.818662954220144, 213.7027547429590015 ) ) ;
#95468=CARTESIAN_POINT ( 'NONE',  ( -11.39360664099999987, 1501.071473199189995, 211.1722694495890096 ) ) ;
#95470=CARTESIAN_POINT ( 'NONE',  ( 1.660747496199999951, 1456.055585494690149, 218.8271600400589989 ) ) ;
#95471=CARTESIAN_POINT ( 'NONE',  ( -2.107860014578959884, 1457.626357230750273, 219.5693110658939986 ) ) ;
#95472=CARTESIAN_POINT ( 'NONE',  ( -4.390466737189999691, 1449.947854720489886, 190.5483265708990075 ) ) ;
#95475=CARTESIAN_POINT ( 'NONE',  ( 7.754157970519999665, 1425.611232019499994, 211.7686771286390126 ) ) ;
#95476=CARTESIAN_POINT ( 'NONE',  ( 14.43085696089999992, 1426.807557149800004, 195.4949581795989957 ) ) ;
#95482=ORIENTED_EDGE ( 'NONE', *, *, #10056, .F. ) ;
#95489=CARTESIAN_POINT ( 'NONE',  ( 0.8761538346837720592, 1475.978191697550074, 197.6843414950239719 ) ) ;
#95501=CARTESIAN_POINT ( 'NONE',  ( -3.786971751329999858, 1455.326410022090158, 200.4755219205989931 ) ) ;
#95505=ORIENTED_EDGE ( 'NONE', *, *, #99444, .F. ) ;
#95523=CARTESIAN_POINT ( 'NONE',  ( -7.332236864109274777, 1441.976884069165862, 202.1892200067096041 ) ) ;
#95529=CARTESIAN_POINT ( 'NONE',  ( -5.292247061280000331, 1391.913060387289988, 214.4361776263990009 ) ) ;
#95538=CARTESIAN_POINT ( 'NONE',  ( -3.471770239069999597, 1428.655773691090189, 200.4250886094789905 ) ) ;
#95560=CARTESIAN_POINT ( 'NONE',  ( 3.125212102749999943, 1443.129716313290146, 217.4566555861789823 ) ) ;
#95561=CARTESIAN_POINT ( 'NONE',  ( 3.829619994797929916, 1515.551704292389786, 207.2788821832570250 ) ) ;
#95569=CARTESIAN_POINT ( 'NONE',  ( -5.085989740509197610, 1391.850992569807204, 203.6120040231442658 ) ) ;
#95574=CARTESIAN_POINT ( 'NONE',  ( -18.43525369369999822, 1507.707328976990084, 209.4281662339789705 ) ) ;
#95577=B_SPLINE_SURFACE_WITH_KNOTS ( 'NONE', 5, 5, ( 
 ( #68821, #50361, #60411, #44158, #67709, #77752 ),
 ( #101818, #102922, #59316, #16697, #50897, #85027 ),
 ( #8320, #76638, #110790, #68276, #45824, #27897 ),
 ( #96206, #46381, #70484, #19481, #11113, #62645 ),
 ( #81047, #78870, #28451, #21117, #104604, #4361 ),
 ( #44718, #2176, #96766, #36291, #63729, #38490 ),
 ( #53683, #62080, #29007, #29542, #71603, #72667 ),
 ( #87825, #3830, #53116, #3274, #106793, #45274 ),
 ( #64277, #37958, #80513, #105159, #10544, #55322 ) ),
 .UNSPECIFIED., .F., .F., .F.,
 ( 6, 3, 6 ),
 ( 6, 6 ),
 ( 2.767471764330379891, 4.758631476969999774, 6.749791190855430223 ),
 ( -0.0004300833054265790429, 2.000000000000000000 ),
 .UNSPECIFIED. ) ;
#95579=CARTESIAN_POINT ( 'NONE',  ( -10.93162295028230169, 1470.132889486390013, 212.2376398131100075 ) ) ;
#95580=CARTESIAN_POINT ( 'NONE',  ( -4.769978619596870750, 1487.672230412279987, 219.3630103478849946 ) ) ;
#95582=CARTESIAN_POINT ( 'NONE',  ( -9.771923492860000948, 1448.872168905890021, 190.8346797514990101 ) ) ;
#95588=EDGE_LOOP ( 'NONE', ( #98210, #107183, #91058, #23507 ) ) ;
#95600=CARTESIAN_POINT ( 'NONE',  ( 8.635265467701518816, 1437.313984394470026, 208.5984011097850157 ) ) ;
#95609=CARTESIAN_POINT ( 'NONE',  ( -15.98649555842510139, 1420.860515612879908, 203.3512188490260257 ) ) ;
#95613=ORIENTED_EDGE ( 'NONE', *, *, #82141, .F. ) ;
#95614=CARTESIAN_POINT ( 'NONE',  ( -3.117394561335489644, 1508.880976916049804, 213.6144879082389991 ) ) ;
#95615=CARTESIAN_POINT ( 'NONE',  ( 20.63006355019999916, 1477.703139823589936, 217.6305604476790165 ) ) ;
#95625=CARTESIAN_POINT ( 'NONE',  ( -7.672540978279999813, 1458.367780384589878, 214.9746805944489836 ) ) ;
#95629=ORIENTED_EDGE ( 'NONE', *, *, #11777, .F. ) ;
#95630=CARTESIAN_POINT ( 'NONE',  ( -8.813634211109999228, 1423.275147988690151, 209.8404090638680088 ) ) ;
#95637=ORIENTED_EDGE ( 'NONE', *, *, #36330, .T. ) ;
#95642=CARTESIAN_POINT ( 'NONE',  ( -0.4375840930677259988, 1487.902785764265445, 219.9692466604490448 ) ) ;
#95643=CARTESIAN_POINT ( 'NONE',  ( -18.74955383543489873, 1508.522973533499908, 210.3303428506329738 ) ) ;
#95644=CARTESIAN_POINT ( 'NONE',  ( -0.8775825618903728698, 1398.755125754900064, 209.6012715003031985 ) ) ;
#95645=CARTESIAN_POINT ( 'NONE',  ( -8.447729234144269128, 1439.539276948720044, 206.3527110188499876 ) ) ;
#95659=B_SPLINE_SURFACE_WITH_KNOTS ( 'NONE', 5, 5, ( 
 ( #27628, #35474, #45010, #105446, #62940, #11932 ),
 ( #9717, #61815, #104890, #95938, #69105, #19771 ),
 ( #80242, #103206, #19198, #28181, #26511, #94831 ),
 ( #96491, #4099, #108177, #81872, #4632, #13551 ),
 ( #48858, #98123, #82983, #47192, #38223, #48300 ),
 ( #71888, #64012, #5739, #37683, #46660, #107637 ),
 ( #90268, #106003, #106536, #20863, #21940, #22490 ),
 ( #30920, #29279, #21398, #73503, #5173, #39881 ),
 ( #55058, #30371, #63472, #29825, #13006, #99766 ) ),
 .UNSPECIFIED., .F., .F., .F.,
 ( 6, 3, 6 ),
 ( 6, 6 ),
 ( 3.948767879310000062, 7.805279617920000135, 12.92009085129999946 ),
 ( 0.000000000000000000, 2.000000000000000000 ),
 .UNSPECIFIED. ) ;
#95662=EDGE_CURVE ( 'NONE', #44452, #102315, #14764, .T. ) ;
#95667=VERTEX_POINT ( 'NONE', #82895 ) ;
#95668=CARTESIAN_POINT ( 'NONE',  ( 1.751672294820000086, 1443.909066847590111, 215.1365789184590085 ) ) ;
#95672=CARTESIAN_POINT ( 'NONE',  ( 3.137381254594810542, 1508.729448404669938, 204.5649390561709993 ) ) ;
#95674=EDGE_CURVE ( 'NONE', #58146, #72871, #84175, .T. ) ;
#95690=ORIENTED_EDGE ( 'NONE', *, *, #56468, .T. ) ;
#95694=CARTESIAN_POINT ( 'NONE',  ( -20.46845896326908587, 1507.979024348134317, 209.5470984320012917 ) ) ;
#95695=CARTESIAN_POINT ( 'NONE',  ( -0.2472255341746696089, 1420.996142865428283, 193.7190874371098346 ) ) ;
#95701=B_SPLINE_SURFACE_WITH_KNOTS ( 'NONE', 5, 5, ( 
 ( #7466, #99440, #22717, #56918, #91048, #93119 ),
 ( #18060, #104293, #11891, #61227, #63428, #87503 ),
 ( #43838, #104845, #35993, #2966, #28132, #46063 ),
 ( #103738, #77984, #35430, #88609, #61765, #44402 ),
 ( #10224, #69617, #79662, #96448, #19151, #78544 ),
 ( #9666, #88063, #11348, #1858, #79111, #27039 ) ),
 .UNSPECIFIED., .F., .F., .F.,
 ( 6, 6 ),
 ( 6, 6 ),
 ( 2.088384708059999983, 2.452169171380000012 ),
 ( 0.000000000000000000, 0.2999999999999999889 ),
 .UNSPECIFIED. ) ;
#95703=CARTESIAN_POINT ( 'NONE',  ( 14.04725111459999987, 1429.738167031290004, 194.8870957077990340 ) ) ;
#95705=CARTESIAN_POINT ( 'NONE',  ( 10.71266894638830003, 1462.053231644700190, 211.5459097712770244 ) ) ;
#95710=CARTESIAN_POINT ( 'NONE',  ( -15.60279201232230406, 1420.350159234621287, 210.5032511881165931 ) ) ;
#95714=CARTESIAN_POINT ( 'NONE',  ( 20.75865324819899982, 1455.056399446189971, 207.3304374463790225 ) ) ;
#95716=CARTESIAN_POINT ( 'NONE',  ( -4.038582018629999659, 1515.598601288590089, 209.1218459616989946 ) ) ;
#95718=CARTESIAN_POINT ( 'NONE',  ( 3.616466670889999957, 1441.209878957790124, 217.9421667894289953 ) ) ;
#95719=ORIENTED_EDGE ( 'NONE', *, *, #53684, .F. ) ;
#95722=CARTESIAN_POINT ( 'NONE',  ( -4.519117204389999642, 1475.824012005989971, 199.8305589088090244 ) ) ;
#95725=CARTESIAN_POINT ( 'NONE',  ( -6.857441324633220425, 1508.551704407529996, 219.2237596246229714 ) ) ;
#95727=CIRCLE ( 'NONE', #81394, 1.000006598386372847 ) ;
#95732=CARTESIAN_POINT ( 'NONE',  ( 0.8465099650069989323, 1430.128328917089902, 217.4134727424889775 ) ) ;
#95738=CARTESIAN_POINT ( 'NONE',  ( 11.19141260661350046, 1422.145557588919928, 210.4507437126630123 ) ) ;
#95742=EDGE_LOOP ( 'NONE', ( #80978, #53021, #95744, #11024 ) ) ;
#95744=ORIENTED_EDGE ( 'NONE', *, *, #48902, .F. ) ;
#95745=CARTESIAN_POINT ( 'NONE',  ( 1.842962215208693078, 1515.492058412108918, 204.9833025688982104 ) ) ;
#95756=CARTESIAN_POINT ( 'NONE',  ( 1.145290941939999918, 1458.110488011190000, 199.6352770980190030 ) ) ;
#95761=CARTESIAN_POINT ( 'NONE',  ( -3.584843346320000013, 1496.864215273689979, 220.1846651968990045 ) ) ;
#95775=CARTESIAN_POINT ( 'NONE',  ( 3.892100939925419834, 1508.551704408389924, 213.6765049832410170 ) ) ;
#95779=CARTESIAN_POINT ( 'NONE',  ( 10.21143262099270110, 1460.458462329770100, 206.7445078786060151 ) ) ;
#95783=CARTESIAN_POINT ( 'NONE',  ( 8.916180505392530264, 1451.556357916370189, 211.6695736768569986 ) ) ;
#95784=CARTESIAN_POINT ( 'NONE',  ( 8.766925616880000049, 1424.448725112169996, 196.2368360184990195 ) ) ;
#95792=CARTESIAN_POINT ( 'NONE',  ( 3.586339042944246103, 1515.071394417499278, 213.2045494097142182 ) ) ;
#95805=CARTESIAN_POINT ( 'NONE',  ( -6.232811146862309748, 1469.026420360470183, 218.0650955369210067 ) ) ;
#95810=CARTESIAN_POINT ( 'NONE',  ( 10.13319077529999923, 1492.435480105489887, 213.9998358472890061 ) ) ;
#95814=CARTESIAN_POINT ( 'NONE',  ( 9.322115572355668789, 1468.760034264159913, 202.8348514626249823 ) ) ;
#95822=CARTESIAN_POINT ( 'NONE',  ( 3.753799318440000032, 1506.440767537289958, 220.3044440926989864 ) ) ;
#95825=CARTESIAN_POINT ( 'NONE',  ( -1.324264359524509826, 1515.084669001950033, 204.7929176606560304 ) ) ;
#95827=CARTESIAN_POINT ( 'NONE',  ( -16.88834672024129802, 1418.279337056010036, 203.8013833312560052 ) ) ;
#95828=FACE_OUTER_BOUND ( 'NONE', #72833, .T. ) ;
#95829=CARTESIAN_POINT ( 'NONE',  ( -16.53913957400000001, 1417.008824413999946, 208.4907982911209956 ) ) ;
#95830=CARTESIAN_POINT ( 'NONE',  ( -0.02536948887749890247, 1430.362855603430035, 199.7013224701310037 ) ) ;
#95831=CARTESIAN_POINT ( 'NONE',  ( 2.000821305087136182, 1443.721900349954467, 217.8590849949153210 ) ) ;
#95833=CARTESIAN_POINT ( 'NONE',  ( -4.992349871978174924, 1391.620913784733830, 203.7130789026546154 ) ) ;
#95834=DIRECTION ( 'NONE',  ( 1.000000000000000000, 0.000000000000000000, 0.000000000000000000 ) ) ;
#95853=CARTESIAN_POINT ( 'NONE',  ( -15.41862096090000200, 1414.824310420299980, 208.6539393912370031 ) ) ;
#95856=CARTESIAN_POINT ( 'NONE',  ( 17.85886714360680116, 1428.995146824200219, 205.7472297062370217 ) ) ;
#95857=CARTESIAN_POINT ( 'NONE',  ( 9.682511080499990541, 1436.279831232390052, 210.8541354582289955 ) ) ;
#95858=ORIENTED_EDGE ( 'NONE', *, *, #125, .F. ) ;
#95864=CARTESIAN_POINT ( 'NONE',  ( -11.64243205524850033, 1481.168562452440028, 211.2324576138770169 ) ) ;
#95874=CARTESIAN_POINT ( 'NONE',  ( 4.201107383170000098, 1515.456955069890228, 208.0103411306490102 ) ) ;
#95882=CARTESIAN_POINT ( 'NONE',  ( 11.76015609417409991, 1479.338828819800028, 208.6267683045179808 ) ) ;
#95886=EDGE_CURVE ( 'NONE', #46147, #52400, #47110, .T. ) ;
#95887=CARTESIAN_POINT ( 'NONE',  ( 18.87014351247420052, 1458.714671120490038, 220.5051382869739882 ) ) ;
#95893=CARTESIAN_POINT ( 'NONE',  ( -10.97860730640000071, 1492.014415902390056, 210.2726032398089728 ) ) ;
#95900=CARTESIAN_POINT ( 'NONE',  ( 10.92782285068519954, 1503.815843204259863, 213.0813150825409821 ) ) ;
#95904=VERTEX_POINT ( 'NONE', #79340 ) ;
#95907=ORIENTED_EDGE ( 'NONE', *, *, #43312, .F. ) ;
#95908=CARTESIAN_POINT ( 'NONE',  ( -0.05883584365174199943, 1457.642074517544415, 199.5869934370919054 ) ) ;
#95909=FACE_OUTER_BOUND ( 'NONE', #15564, .T. ) ;
#95918=EDGE_CURVE ( 'NONE', #14236, #18748, #70971, .T. ) ;
#95920=CARTESIAN_POINT ( 'NONE',  ( -4.949448334325509791, 1426.816921726720011, 207.3013729964370100 ) ) ;
#95921=CARTESIAN_POINT ( 'NONE',  ( -6.918225063430000432, 1481.313522505289939, 206.5729028383990169 ) ) ;
#95922=ORIENTED_EDGE ( 'NONE', *, *, #9660, .F. ) ;
#95924=CARTESIAN_POINT ( 'NONE',  ( -17.21523805317120193, 1442.518106596560074, 216.7674110779969965 ) ) ;
#95933=CARTESIAN_POINT ( 'NONE',  ( 10.12978361029999874, 1461.480643167490143, 208.6898772595120306 ) ) ;
#95936=CARTESIAN_POINT ( 'NONE',  ( -18.40088546307429951, 1508.551704408389924, 210.4144978082819648 ) ) ;
#95938=CARTESIAN_POINT ( 'NONE',  ( 2.745476835439999874, 1465.706481184990025, 199.2183696094690220 ) ) ;
#95940=ORIENTED_EDGE ( 'NONE', *, *, #57775, .T. ) ;
#95944=CARTESIAN_POINT ( 'NONE',  ( 11.47796531776959839, 1478.826507664550036, 206.6271712911859879 ) ) ;
#95950=CARTESIAN_POINT ( 'NONE',  ( -1.127400696442319994, 1422.674730469140059, 192.5292151802170224 ) ) ;
#95954=CARTESIAN_POINT ( 'NONE',  ( -5.482980402289999944, 1508.348588800990001, 220.2461224233989867 ) ) ;
#95959=AXIS2_PLACEMENT_3D ( 'NONE', #40943, #15171, #90794 ) ;
#95981=CARTESIAN_POINT ( 'NONE',  ( 4.545982227442832979, 1508.783371655767723, 211.6097810847320204 ) ) ;
#95989=CARTESIAN_POINT ( 'NONE',  ( -0.5525097125479990767, 1430.369002146489947, 200.0800212161890101 ) ) ;
#95996=CARTESIAN_POINT ( 'NONE',  ( 3.168149218889090069, 1465.479944987909903, 199.6312225713100190 ) ) ;
#95998=CARTESIAN_POINT ( 'NONE',  ( 7.271691885010000078, 1501.094707673489893, 204.7367163811290141 ) ) ;
#96002=VECTOR ( 'NONE', #90324, 1000.000000000000114 ) ;
#96004=CARTESIAN_POINT ( 'NONE',  ( 15.58948595390000058, 1452.698291846990060, 196.7507890572990163 ) ) ;
#96010=CARTESIAN_POINT ( 'NONE',  ( -18.97541190666909827, 1485.183224067069887, 218.3497724515069933 ) ) ;
#96012=CARTESIAN_POINT ( 'NONE',  ( -6.569077902550000125, 1472.000453826989997, 211.3893757803390088 ) ) ;
#96016=CARTESIAN_POINT ( 'NONE',  ( -9.898687722262419442, 1438.737011691519911, 210.1098268883750109 ) ) ;
#96021=CARTESIAN_POINT ( 'NONE',  ( 7.880635186530000169, 1425.932163105479958, 211.6468907411690168 ) ) ;
#96023=CARTESIAN_POINT ( 'NONE',  ( 0.5708672984259970384, 1460.784242392889837, 230.4191149236990270 ) ) ;
#96029=CARTESIAN_POINT ( 'NONE',  ( 5.853197488659999337, 1455.236944383789933, 217.5027156205790106 ) ) ;
#96038=CARTESIAN_POINT ( 'NONE',  ( -2.711955045610519921, 1463.961042537189996, 199.5488283424340068 ) ) ;
#96051=EDGE_CURVE ( 'NONE', #12135, #104137, #21277, .T. ) ;
#96056=EDGE_CURVE ( 'NONE', #13254, #89963, #38766, .T. ) ;
#96060=CARTESIAN_POINT ( 'NONE',  ( 8.377020731070000892, 1427.910351821989934, 212.6460221678989910 ) ) ;
#96064=CARTESIAN_POINT ( 'NONE',  ( 10.51054176719999944, 1491.593345921790160, 212.4262175969289785 ) ) ;
#96082=CARTESIAN_POINT ( 'NONE',  ( 0.000000000000000000, 1508.551704408389924, 209.1218459616989946 ) ) ;
#96086=CARTESIAN_POINT ( 'NONE',  ( -10.61669498371649922, 1508.551704408389924, 207.6874897006059939 ) ) ;
#96087=CARTESIAN_POINT ( 'NONE',  ( -2.942964642939999820, 1430.286447874990245, 201.3134892009489931 ) ) ;
#96090=CARTESIAN_POINT ( 'NONE',  ( 3.415183242699999955, 1486.712733892290089, 198.4695611698990092 ) ) ;
#96091=CARTESIAN_POINT ( 'NONE',  ( 11.20716745179999840, 1422.288374914430278, 203.3912787612890156 ) ) ;
#96100=CARTESIAN_POINT ( 'NONE',  ( 5.161034791280000533, 1485.814572579490005, 218.5690567784690188 ) ) ;
#96101=CARTESIAN_POINT ( 'NONE',  ( 8.214063898797519414, 1423.929538348540291, 211.6355982495960006 ) ) ;
#96110=CARTESIAN_POINT ( 'NONE',  ( 295.4396770967078965, -8387.357407334289746, 2232.807573057129957 ) ) ;
#96111=EDGE_CURVE ( 'NONE', #75452, #14195, #78849, .T. ) ;
#96115=CARTESIAN_POINT ( 'NONE',  ( -4.391428885256890347, 1464.583814225909919, 199.0196702316530093 ) ) ;
#96118=CARTESIAN_POINT ( 'NONE',  ( -5.093685840561368749, 1391.856767254725355, 203.6189120034268853 ) ) ;
#96125=CARTESIAN_POINT ( 'NONE',  ( -4.542064733420000167, 1483.636937311689962, 199.4558309895289767 ) ) ;
#96130=CARTESIAN_POINT ( 'NONE',  ( -11.39064650766950137, 1470.655863615889984, 209.6027845347450125 ) ) ;
#96131=CARTESIAN_POINT ( 'NONE',  ( -4.592827604961299492, 1488.079576444790064, 219.1748425648949876 ) ) ;
#96132=CARTESIAN_POINT ( 'NONE',  ( 18.99431323780000014, 1459.501207708489801, 220.3864241394989847 ) ) ;
#96135=CARTESIAN_POINT ( 'NONE',  ( -5.108150090387360009, 1391.866415515492235, 214.6117004621733599 ) ) ;
#96142=CARTESIAN_POINT ( 'NONE',  ( -14.93718008229999938, 1416.181292664740113, 212.9156384192889959 ) ) ;
#96143=ORIENTED_EDGE ( 'NONE', *, *, #2736, .F. ) ;
#96151=CARTESIAN_POINT ( 'NONE',  ( 8.610988768402860316, 1436.778401557170127, 208.5600591984729988 ) ) ;
#96155=CARTESIAN_POINT ( 'NONE',  ( 0.9431357159449988981, 1487.666359187690205, 217.1994056721289894 ) ) ;
#96161=CARTESIAN_POINT ( 'NONE',  ( -14.41439834266500064, 1421.637802249239940, 203.6166032916469817 ) ) ;
#96169=CARTESIAN_POINT ( 'NONE',  ( -17.89922477309999849, 1489.399004187290075, 195.2216578317990070 ) ) ;
#96172=( BOUNDED_CURVE ( )  B_SPLINE_CURVE ( 3, ( #38059, #3379, #13938, #63293 ),
 .UNSPECIFIED., .F., .F. ) 
 B_SPLINE_CURVE_WITH_KNOTS ( ( 4, 4 ),
 ( 4.168090934964655325, 5.256687371692810196 ),
 .UNSPECIFIED. ) 
 CURVE ( )  GEOMETRIC_REPRESENTATION_ITEM ( )  RATIONAL_B_SPLINE_CURVE ( ( 1.000000000000000000, 0.9036605976482073865, 0.9036605976482073865, 1.000000000000000000 ) ) 
 REPRESENTATION_ITEM ( '' )  );
#96175=CARTESIAN_POINT ( 'NONE',  ( 4.329271545279290478, 1515.071561052290008, 210.6721986880200177 ) ) ;
#96184=CARTESIAN_POINT ( 'NONE',  ( -9.205204419190000209, 1422.968094939250022, 210.4274292779389839 ) ) ;
#96187=CARTESIAN_POINT ( 'NONE',  ( -9.754833734307490900, 1446.835976941670197, 212.2157276707299900 ) ) ;
#96192=CARTESIAN_POINT ( 'NONE',  ( -0.9609375957247829891, 1496.458315686089918, 221.4414273593889959 ) ) ;
#96198=CARTESIAN_POINT ( 'NONE',  ( -0.1535940140686828936, 1487.818612005767591, 219.9756013004578676 ) ) ;
#96199=CARTESIAN_POINT ( 'NONE',  ( -18.30804477475249925, 1508.522800635979820, 211.1085587802360237 ) ) ;
#96200=FACE_OUTER_BOUND ( 'NONE', #73841, .T. ) ;
#96201=CARTESIAN_POINT ( 'NONE',  ( -8.630929624523329124, 1438.255171044090048, 208.1083491479620022 ) ) ;
#96206=CARTESIAN_POINT ( 'NONE',  ( 8.257535438202340927, 1436.457248292470013, 206.6719407321619997 ) ) ;
#96209=VERTEX_POINT ( 'NONE', #6889 ) ;
#96211=CARTESIAN_POINT ( 'NONE',  ( -2.130922739038390024, 1467.954349360780043, 220.0452206896550251 ) ) ;
#96212=CARTESIAN_POINT ( 'NONE',  ( -20.49321649319999850, 1486.267955954489935, 212.0899509670090026 ) ) ;
#96222=FACE_OUTER_BOUND ( 'NONE', #33375, .T. ) ;
#96225=CARTESIAN_POINT ( 'NONE',  ( 3.176056732109850067, 1508.610720109290014, 204.4420549359030019 ) ) ;
#96229=CARTESIAN_POINT ( 'NONE',  ( 7.550314398180000275, 1423.033197812850176, 195.6993106477989954 ) ) ;
#96243=B_SPLINE_SURFACE_WITH_KNOTS ( 'NONE', 5, 1, ( 
 ( #43417, #54050 ),
 ( #52926, #68627 ),
 ( #9258, #51818 ),
 ( #10914, #18187 ),
 ( #52383, #96010 ),
 ( #19280, #61346 ) ),
 .UNSPECIFIED., .F., .F., .F.,
 ( 6, 6 ),
 ( 2, 2 ),
 ( -8.513468052107540614E-05, 17.21697013008050092 ),
 ( 0.000000000000000000, 14.00008513468049998 ),
 .UNSPECIFIED. ) ;
#96249=CARTESIAN_POINT ( 'NONE',  ( -4.327045307008839714, 1515.156577661799929, 208.9300209000519999 ) ) ;
#96256=CARTESIAN_POINT ( 'NONE',  ( -17.72527547369999823, 1420.469651944000134, 207.4580708041989965 ) ) ;
#96268=CARTESIAN_POINT ( 'NONE',  ( -3.788228201615989832, 1508.728292637470076, 204.8186040600340050 ) ) ;
#96272=CARTESIAN_POINT ( 'NONE',  ( 18.28406076839999983, 1431.588999307289896, 208.2780601718820037 ) ) ;
#96277=CARTESIAN_POINT ( 'NONE',  ( -3.950036120199999612, 1475.164021116390131, 199.1854335113090144 ) ) ;
#96280=CARTESIAN_POINT ( 'NONE',  ( -3.200625999729659554, 1508.551704408389924, 219.9719447069430203 ) ) ;
#96283=CARTESIAN_POINT ( 'NONE',  ( -2.869809977300000092, 1489.506021206889955, 188.4705320259990060 ) ) ;
#96286=CARTESIAN_POINT ( 'NONE',  ( -1.324219039799999997, 1431.506123345290007, 217.5609468189390157 ) ) ;
#96287=CARTESIAN_POINT ( 'NONE',  ( -15.61813151019999957, 1420.484314087570056, 211.1660300703989890 ) ) ;
#96289=FACE_OUTER_BOUND ( 'NONE', #8498, .T. ) ;
#96294=CARTESIAN_POINT ( 'NONE',  ( 10.96709298812059963, 1490.204820260260021, 209.1517527257469737 ) ) ;
#96315=CIRCLE ( 'NONE', #17629, 8.104319688360000384 ) ;
#96316=CARTESIAN_POINT ( 'NONE',  ( -3.703568382519999869, 1497.311625982490114, 220.9591690777990038 ) ) ;
#96328=CARTESIAN_POINT ( 'NONE',  ( 3.153551286829999967, 1486.681966494889821, 219.4644408646990144 ) ) ;
#96337=ORIENTED_EDGE ( 'NONE', *, *, #54901, .F. ) ;
#96344=FACE_OUTER_BOUND ( 'NONE', #81999, .T. ) ;
#96349=CARTESIAN_POINT ( 'NONE',  ( 6.277696993560000216, 1462.172825430389821, 207.2400390766889871 ) ) ;
#96359=CARTESIAN_POINT ( 'NONE',  ( -7.026031763481809911, 1508.551704408389924, 219.1713198989909870 ) ) ;
#96360=CARTESIAN_POINT ( 'NONE',  ( -17.02584102842030234, 1420.296749622020116, 203.9584675048969871 ) ) ;
#96361=CARTESIAN_POINT ( 'NONE',  ( -9.762135819850678686, 1470.449700743350149, 213.1189514009770107 ) ) ;
#96365=CARTESIAN_POINT ( 'NONE',  ( -5.062209827260000239, 1474.342206524190033, 198.8731686433990262 ) ) ;
#96366=CARTESIAN_POINT ( 'NONE',  ( -2.472546487080370170, 1422.360492482099744, 192.6709265187130029 ) ) ;
#96368=CARTESIAN_POINT ( 'NONE',  ( 7.539561783740881040, 1423.272083796969127, 195.6671181022157100 ) ) ;
#96369=CARTESIAN_POINT ( 'NONE',  ( -17.60187515309999995, 1504.668623956589954, 208.9385782990950133 ) ) ;
#96370=CARTESIAN_POINT ( 'NONE',  ( 10.94478922204540083, 1470.010321155669772, 206.1681359757739926 ) ) ;
#96374=ORIENTED_EDGE ( 'NONE', *, *, #75587, .T. ) ;
#96380=CARTESIAN_POINT ( 'NONE',  ( 1.338019250827790163, 1431.361302059610125, 218.5179660117710227 ) ) ;
#96381=CARTESIAN_POINT ( 'NONE',  ( 5.137469271169999629, 1505.238374756890153, 220.3656813046989953 ) ) ;
#96382=CARTESIAN_POINT ( 'NONE',  ( -14.93717996069999998, 1416.181292681839977, 212.9156383665589942 ) ) ;
#96383=CARTESIAN_POINT ( 'NONE',  ( -1.554992009257179841, 1515.071272245639875, 204.7925668544159805 ) ) ;
#96385=B_SPLINE_CURVE_WITH_KNOTS ( 'NONE', 3,
 ( #45095, #85964, #94919, #104419, #1988, #36123, #61899, #70862, #96016, #28262, #26029, #2544, #19287, #53488, #87632, #880, #79235, #18193, #52389, #9804, #104973, #35004, #62456, #96579, #51257 ),
 .UNSPECIFIED., .F., .F.,
 ( 4, 3, 3, 3, 3, 3, 3, 3, 4 ),
 ( -7.174290254210000661, -7.054144120975740506, -6.393701831169590122, -5.726089240763790222, -5.061843816283770003, -4.939077517077059554, -4.323976577597050230, -3.586109338910330013, -2.949396961920000670 ),
 .UNSPECIFIED. ) ;
#96386=CARTESIAN_POINT ( 'NONE',  ( -15.71805126636130545, 1415.757702161196903, 209.6739713832304233 ) ) ;
#96390=CARTESIAN_POINT ( 'NONE',  ( -0.4909561157465350267, 1430.166341371809949, 199.7248743074169965 ) ) ;
#96394=B_SPLINE_CURVE_WITH_KNOTS ( 'NONE', 3,
 ( #40973, #25253, #14109, #48299, #104192, #42635 ),
 .UNSPECIFIED., .F., .F.,
 ( 4, 2, 4 ),
 ( 0.000000000000000000, 0.5000000000000000000, 1.000000000000000000 ),
 .UNSPECIFIED. ) ;
#96398=CARTESIAN_POINT ( 'NONE',  ( -6.343596359860000256, 1477.040213282090008, 217.6105473213789878 ) ) ;
#96417=CARTESIAN_POINT ( 'NONE',  ( 8.959051896893781120, 1436.612241212953904, 210.6498963299843012 ) ) ;
#96418=VERTEX_POINT ( 'NONE', #10204 ) ;
#96437=CARTESIAN_POINT ( 'NONE',  ( 3.281831459213320201, 1466.303209658950209, 198.5678429405679992 ) ) ;
#96444=CARTESIAN_POINT ( 'NONE',  ( 18.95586338705119900, 1455.565549131589933, 200.3905214973929958 ) ) ;
#96448=CARTESIAN_POINT ( 'NONE',  ( -5.081549580979999980, 1391.866816822089959, 203.6256639786390110 ) ) ;
#96450=CARTESIAN_POINT ( 'NONE',  ( -10.99273643789999966, 1491.630725559690063, 209.8916748351909973 ) ) ;
#96451=CARTESIAN_POINT ( 'NONE',  ( 7.146147325059948763, 1378.399971913189802, 209.1218459616989946 ) ) ;
#96454=CARTESIAN_POINT ( 'NONE',  ( -6.799851167021637721, 1423.999032497903045, 192.0811406717795080 ) ) ;
#96456=CARTESIAN_POINT ( 'NONE',  ( -8.742754168010000271, 1424.489613839150024, 206.0336725849989818 ) ) ;
#96460=ORIENTED_EDGE ( 'NONE', *, *, #66461, .T. ) ;
#96465=CARTESIAN_POINT ( 'NONE',  ( 11.44321141689999877, 1500.298942533189802, 206.0875178983189926 ) ) ;
#96475=CARTESIAN_POINT ( 'NONE',  ( -7.175751430708140255, 1425.273472374989979, 206.5995256342289963 ) ) ;
#96478=CARTESIAN_POINT ( 'NONE',  ( -3.076366055149999834, 1424.853903601579987, 191.3970713258989917 ) ) ;
#96479=CARTESIAN_POINT ( 'NONE',  ( 0.6340598045975409658, 1432.588596709849980, 200.7036721141990085 ) ) ;
#96486=DIRECTION ( 'NONE',  ( -1.000000000000000000, 0.000000000000000000, 0.000000000000000000 ) ) ;
#96487=CARTESIAN_POINT ( 'NONE',  ( 2.183557716942239768, 1465.964082040959738, 198.3088933049640161 ) ) ;
#96491=CARTESIAN_POINT ( 'NONE',  ( 2.128647007970000171, 1464.204386043490103, 199.5196855943389949 ) ) ;
#96494=ORIENTED_EDGE ( 'NONE', *, *, #99292, .F. ) ;
#96498=CARTESIAN_POINT ( 'NONE',  ( 11.75720880967569926, 1479.323378685179932, 208.5706975412350062 ) ) ;
#96509=CARTESIAN_POINT ( 'NONE',  ( -5.303775421610000151, 1508.737782198590139, 220.0395200587989848 ) ) ;
#96514=CARTESIAN_POINT ( 'NONE',  ( 0.8923934389429990510, 1469.297510594290088, 216.3874288503389778 ) ) ;
#96519=EDGE_CURVE ( 'NONE', #2979, #73174, #13354, .T. ) ;
#96520=CARTESIAN_POINT ( 'NONE',  ( 4.329448802989709577, 1515.064791341159889, 211.4517443316900085 ) ) ;
#96521=CARTESIAN_POINT ( 'NONE',  ( -4.978441812830840085, 1483.044991982689908, 199.7126697438380063 ) ) ;
#96528=CARTESIAN_POINT ( 'NONE',  ( -11.52225187220090774, 1489.339478244986822, 213.1483457362718070 ) ) ;
#96529=CARTESIAN_POINT ( 'NONE',  ( -14.21441912100000060, 1415.677402202029953, 204.5785383627490148 ) ) ;
#96535=CARTESIAN_POINT ( 'NONE',  ( -9.077189760424749565, 1449.419093657679923, 210.4763515235329976 ) ) ;
#96540=CARTESIAN_POINT ( 'NONE',  ( -0.008286608719400527859, 1515.284302758789863, 213.4455463337289984 ) ) ;
#96543=EDGE_CURVE ( 'NONE', #72135, #82048, #70739, .T. ) ;
#96567=CARTESIAN_POINT ( 'NONE',  ( -9.383290498310000061, 1483.074069049089985, 203.0916503736390268 ) ) ;
#96575=CARTESIAN_POINT ( 'NONE',  ( -19.23853081770000273, 1466.576780668189940, 213.8528554934590034 ) ) ;
#96576=CARTESIAN_POINT ( 'NONE',  ( -15.77825334036446492, 1415.905193579931620, 209.0522866884972188 ) ) ;
#96577=CARTESIAN_POINT ( 'NONE',  ( -4.987275435840000881, 1510.323409146890071, 216.8373829782190114 ) ) ;
#96579=CARTESIAN_POINT ( 'NONE',  ( -9.972556032338060206, 1439.430100340180161, 208.5509081778830023 ) ) ;
#96580=DIRECTION ( 'NONE',  ( 1.000000000000000000, 0.000000000000000000, 0.000000000000000000 ) ) ;
#96584=CARTESIAN_POINT ( 'NONE',  ( 7.603387035110000802, 1425.782375950509959, 212.0439570241190097 ) ) ;
#96602=CARTESIAN_POINT ( 'NONE',  ( 11.41288121311350068, 1427.618783885739958, 209.6357582931089780 ) ) ;
#96615=CARTESIAN_POINT ( 'NONE',  ( -3.720950966109999758, 1454.058771263989911, 199.3235536337890039 ) ) ;
#96626=CARTESIAN_POINT ( 'NONE',  ( -12.23218726772509868, 1490.223478903719979, 209.6887218936990109 ) ) ;
#96637=CARTESIAN_POINT ( 'NONE',  ( 16.27172383310000114, 1476.104910058290216, 222.3698031616989965 ) ) ;
#96644=CARTESIAN_POINT ( 'NONE',  ( 9.305981717835429379, 1425.677315260519890, 193.6786577638000040 ) ) ;
#96663=CARTESIAN_POINT ( 'NONE',  ( -3.889576884872586682, 1455.763526873609408, 200.4986044836267922 ) ) ;
#96665=CARTESIAN_POINT ( 'NONE',  ( 10.04074129076350097, 1469.832169069019983, 209.8604891245049942 ) ) ;
#96671=ADVANCED_FACE ( 'NONE', ( #23554 ), #35797, .F. ) ;
#96674=CARTESIAN_POINT ( 'NONE',  ( 3.074701863640000088, 1441.333177043090018, 218.5515105840890158 ) ) ;
#96681=CARTESIAN_POINT ( 'NONE',  ( -4.139067334555820210, 1464.629524841519924, 198.9111649813920053 ) ) ;
#96688=CARTESIAN_POINT ( 'NONE',  ( -7.737321863080000028, 1508.477796734990079, 219.4085941960990169 ) ) ;
#96692=CARTESIAN_POINT ( 'NONE',  ( -1.637262557069999902, 1483.893433194890122, 198.5669152071990027 ) ) ;
#96697=CARTESIAN_POINT ( 'NONE',  ( -11.32770374180210027, 1470.496536099929926, 210.3424180843229863 ) ) ;
#96699=CARTESIAN_POINT ( 'NONE',  ( -9.247716023661459062, 1489.608888726200121, 215.3272058384319791 ) ) ;
#96700=CARTESIAN_POINT ( 'NONE',  ( -18.92739421348260009, 1503.346059615760169, 222.1981729787850099 ) ) ;
#96703=CARTESIAN_POINT ( 'NONE',  ( -5.114744891480448530, 1391.870385291815182, 214.6056989427710562 ) ) ;
#96704=CARTESIAN_POINT ( 'NONE',  ( 4.271857500090000315, 1429.250640823790036, 216.3852677031590019 ) ) ;
#96712=CARTESIAN_POINT ( 'NONE',  ( -7.835191567469999896, 1492.420539004689999, 209.1441751587790066 ) ) ;
#96717=CARTESIAN_POINT ( 'NONE',  ( 9.022884344052069849, 1436.030640010990055, 209.0591187573379841 ) ) ;
#96722=CARTESIAN_POINT ( 'NONE',  ( -1.403832662453629920, 1515.079617817460075, 213.4509065325290180 ) ) ;
#96733=CARTESIAN_POINT ( 'NONE',  ( -22.14393498469999955, 1486.559014183590079, 217.4067828909289801 ) ) ;
#96742=CARTESIAN_POINT ( 'NONE',  ( -9.442727158709999458, 1460.560438940789709, 211.9848800811889760 ) ) ;
#96745=ORIENTED_EDGE ( 'NONE', *, *, #18526, .F. ) ;
#96749=EDGE_CURVE ( 'NONE', #86208, #234, #90710, .T. ) ;
#96751=CARTESIAN_POINT ( 'NONE',  ( -9.593461995991589220, 1446.925636462349985, 212.1822515110659992 ) ) ;
#96760=CARTESIAN_POINT ( 'NONE',  ( 9.585967232940001637, 1472.264498658589901, 214.5747525333089811 ) ) ;
#96766=CARTESIAN_POINT ( 'NONE',  ( 8.616327664749301007, 1435.881562212750168, 207.7018527875740119 ) ) ;
#96767=EDGE_CURVE ( 'NONE', #53387, #69529, #10606, .T. ) ;
#96769=ORIENTED_EDGE ( 'NONE', *, *, #6359, .T. ) ;
#96772=CARTESIAN_POINT ( 'NONE',  ( 3.114565223550959772, 1466.517051284160061, 219.7262097583810032 ) ) ;
#96774=CARTESIAN_POINT ( 'NONE',  ( 4.967684365510000255, 1469.890599266690060, 189.7939106698990201 ) ) ;
#96783=CARTESIAN_POINT ( 'NONE',  ( 2.564080367290000328, 1443.257105434990081, 214.7475390850690076 ) ) ;
#96806=CARTESIAN_POINT ( 'NONE',  ( -19.32547173205315971, 1508.392602783547318, 209.8687894484399408 ) ) ;
#96809=CARTESIAN_POINT ( 'NONE',  ( -4.328546746085120134, 1515.099240016830208, 207.9973207389659819 ) ) ;
#96816=CARTESIAN_POINT ( 'NONE',  ( 9.378915144369848633, 1500.841300073399907, 202.4402467813089856 ) ) ;
#96818=ADVANCED_FACE ( 'NONE', ( #64910 ), #79656, .T. ) ;
#96819=B_SPLINE_CURVE_WITH_KNOTS ( 'NONE', 5,
 ( #85541, #93948, #25635, #25080, #51410, #50333 ),
 .UNSPECIFIED., .F., .F.,
 ( 6, 6 ),
 ( -1.999999605764219979, -2.592271335366547191E-07 ),
 .UNSPECIFIED. ) ;
#96821=CARTESIAN_POINT ( 'NONE',  ( 9.885290350402808457, 1462.702877345079969, 211.5948837706700090 ) ) ;
#96824=CARTESIAN_POINT ( 'NONE',  ( -1.430538850779999871, 1444.328264147990012, 199.1703828715889983 ) ) ;
#96828=CARTESIAN_POINT ( 'NONE',  ( -15.97653678204605221, 1420.243090095628986, 209.7114017956471343 ) ) ;
#96835=CARTESIAN_POINT ( 'NONE',  ( -2.330134126678749418, 1515.492058413688255, 204.9833025705414116 ) ) ;
#96839=CIRCLE ( 'NONE', #37847, 12.73448142120000171 ) ;
#96841=CARTESIAN_POINT ( 'NONE',  ( -4.735819760670000100, 1474.606130560490101, 199.1616167749889712 ) ) ;
#96844=CARTESIAN_POINT ( 'NONE',  ( -5.950684562925319554, 1508.551704408389924, 219.4535821075459978 ) ) ;
#96850=CARTESIAN_POINT ( 'NONE',  ( 14.46805569519750101, 1471.430981385289897, 194.8600923975780006 ) ) ;
#96851=CARTESIAN_POINT ( 'NONE',  ( -1.452023954020000174, 1431.108953371590133, 217.3997850383090054 ) ) ;
#96875=CARTESIAN_POINT ( 'NONE',  ( -4.869779319875719992, 1491.215858047409938, 188.8099518120989728 ) ) ;
#96884=CARTESIAN_POINT ( 'NONE',  ( 3.018304369310000013, 1486.259445700090055, 219.4861415874989916 ) ) ;
#96885=CARTESIAN_POINT ( 'NONE',  ( -5.106893094720000192, 1391.877272790489997, 214.4361776263990009 ) ) ;
#96890=CARTESIAN_POINT ( 'NONE',  ( -4.086314366678965193, 1515.499673595108106, 206.7917118397523666 ) ) ;
#96893=CARTESIAN_POINT ( 'NONE',  ( 9.133139594464850575, 1451.141730094770082, 210.6182008139099935 ) ) ;
#96895=B_SPLINE_CURVE_WITH_KNOTS ( 'NONE', 3,
 ( #53439, #1937, #87585, #29859, #20896, #63510, #20349, #10874, #11966, #4134 ),
 .UNSPECIFIED., .F., .F.,
 ( 4, 2, 2, 2, 4 ),
 ( 0.000000000000000000, 0.2500000000000000000, 0.5000000000000000000, 0.7500000000000000000, 1.000000000000000000 ),
 .UNSPECIFIED. ) ;
#96915=ORIENTED_EDGE ( 'NONE', *, *, #108907, .F. ) ;
#96918=CARTESIAN_POINT ( 'NONE',  ( -7.656877098949100180, 1508.551704408389924, 219.0266944425760016 ) ) ;
#96920=CARTESIAN_POINT ( 'NONE',  ( -3.622938608617219725, 1468.835452661259978, 218.9451918032920048 ) ) ;
#96923=CARTESIAN_POINT ( 'NONE',  ( 9.225032543388721251, 1450.630799636350048, 209.4288614389280099 ) ) ;
#96924=CARTESIAN_POINT ( 'NONE',  ( -6.281153590029999734, 1475.159552144489908, 200.8925845212189927 ) ) ;
#96925=CARTESIAN_POINT ( 'NONE',  ( 8.502412689479999841, 1494.223831056089921, 218.1490364173589853 ) ) ;
#96928=CARTESIAN_POINT ( 'NONE',  ( -20.17395953629999994, 1505.644431352489846, 209.1238650338669913 ) ) ;
#96930=CARTESIAN_POINT ( 'NONE',  ( 12.32667913303630058, 1421.670227258269961, 207.4634014051960094 ) ) ;
#96931=CARTESIAN_POINT ( 'NONE',  ( -9.914173110146720092, 1439.743127349719998, 207.7929445919720024 ) ) ;
#96940=CARTESIAN_POINT ( 'NONE',  ( 5.057785354339999984, 1505.946855220289990, 219.7575345696990041 ) ) ;
#96941=DIRECTION ( 'NONE',  ( -0.9081805863301267712, -0.3859282978888783910, 0.1620721182118019799 ) ) ;
#96947=CARTESIAN_POINT ( 'NONE',  ( -16.00209757519999698, 1416.197507335639784, 209.0643480693830156 ) ) ;
#96952=CARTESIAN_POINT ( 'NONE',  ( 2.835689136585590298, 1456.955521931160092, 199.2250932076429990 ) ) ;
#96955=CARTESIAN_POINT ( 'NONE',  ( -7.980349849529399187, 1424.821740665096513, 210.5240757545262511 ) ) ;
#96966=CARTESIAN_POINT ( 'NONE',  ( -14.85956138398720050, 1417.764634060990147, 203.2214948970120361 ) ) ;
#96968=EDGE_CURVE ( 'NONE', #46415, #18694, #54657, .T. ) ;
#96973=CARTESIAN_POINT ( 'NONE',  ( 3.002126187839210480, 1456.245863093199887, 219.3132837443019980 ) ) ;
#96974=CARTESIAN_POINT ( 'NONE',  ( 17.92652493019800275, 1429.078765382750134, 206.1304143520609955 ) ) ;
#96978=CARTESIAN_POINT ( 'NONE',  ( 4.387476684030000129, 1477.221828185889990, 199.1648530448690053 ) ) ;
#96981=CARTESIAN_POINT ( 'NONE',  ( 17.78284146230000218, 1432.724246433989947, 213.5810953123289835 ) ) ;
#96992=B_SPLINE_CURVE_WITH_KNOTS ( 'NONE', 3,
 ( #23637, #16312, #75167, #84637, #7934, #76251, #91944, #70641, #96360, #85742 ),
 .UNSPECIFIED., .F., .F.,
 ( 4, 2, 2, 2, 4 ),
 ( -0.2944084045147770112, -0.1489376058949150039, -0.07511920350920017753, -0.03772615716977101297, 0.000000000000000000 ),
 .UNSPECIFIED. ) ;
#96994=CARTESIAN_POINT ( 'NONE',  ( 3.970093244310000102, 1515.569676282289947, 207.9973965014289945 ) ) ;
#97000=CARTESIAN_POINT ( 'NONE',  ( -1.191029124920000015, 1421.235635819999970, 193.7391320501990322 ) ) ;
#97003=CARTESIAN_POINT ( 'NONE',  ( 10.30424762810000061, 1453.480958077889909, 189.9461784470989869 ) ) ;
#97009=CARTESIAN_POINT ( 'NONE',  ( -12.23489737639999930, 1490.237667550689821, 209.6383003343199789 ) ) ;
#97010=CARTESIAN_POINT ( 'NONE',  ( -11.60387546109999946, 1481.105535807389970, 211.4044418313389997 ) ) ;
#97016=AXIS2_PLACEMENT_3D ( 'NONE', #36320, #12779, #70517 ) ;
#97017=CARTESIAN_POINT ( 'NONE',  ( -9.205204419190000209, 1422.968094939250022, 210.4274292779389839 ) ) ;
#97018=CARTESIAN_POINT ( 'NONE',  ( -15.57808073540140015, 1420.358152465259991, 210.5578313205389804 ) ) ;
#97024=CARTESIAN_POINT ( 'NONE',  ( -1.973026181207146124, 1456.791506541725994, 199.8306417962847092 ) ) ;
#97032=CARTESIAN_POINT ( 'NONE',  ( 12.48512064311860037, 1501.209728726249978, 211.5369004838399860 ) ) ;
#97036=FACE_OUTER_BOUND ( 'NONE', #109291, .T. ) ;
#97039=CARTESIAN_POINT ( 'NONE',  ( -2.425229330588690058, 1431.099637562449971, 201.1035349865409785 ) ) ;
#97040=B_SPLINE_CURVE_WITH_KNOTS ( 'NONE', 3,
 ( #53484, #10916, #106071, #104969, #97667, #79231, #36119, #29896, #2540, #80325, #63016, #36664, #88728, #105529, #54594, #87061, #70858, #28258, #62451, #87628, #72481, #80872, #3641, #44520, #12561, #19847, #12011, #3090, #38301, #21479, #45645, #55144, #70303 ),
 .UNSPECIFIED., .F., .F.,
 ( 4, 1, 1, 2, 2, 1, 1, 2, 2, 2, 1, 1, 1, 2, 2, 2, 1, 1, 2, 2, 4 ),
 ( 0.000000000000000000, 0.06250000000018264557, 0.09375000000028335667, 0.1093750000003022582, 0.1250000000003211598, 0.1875000000005473677, 0.2187500000006051826, 0.2343750000006341039, 0.2500000000006630252, 0.3750000000007583378, 0.4375000000008123502, 0.4687500000008393286, 0.4843750000007667200, 0.4921875000007259193, 0.5000000000006850076, 0.6250000000008451018, 0.6875000000009251488, 0.7187500000009674483, 0.7343750000008923973, 0.7500000000008173462, 1.000000000000000000 ),
 .UNSPECIFIED. ) ;
#97042=ORIENTED_EDGE ( 'NONE', *, *, #24725, .F. ) ;
#97048=CARTESIAN_POINT ( 'NONE',  ( -0.1084292933363149997, 1465.381382752510035, 198.1171392823189876 ) ) ;
#97055=ORIENTED_EDGE ( 'NONE', *, *, #9842, .F. ) ;
#97064=CARTESIAN_POINT ( 'NONE',  ( -4.823731843395559160, 1434.139159376030193, 217.4489446990200179 ) ) ;
#97068=CARTESIAN_POINT ( 'NONE',  ( -2.469737752589999946, 1507.227429050490173, 221.7265311398990093 ) ) ;
#97074=EDGE_CURVE ( 'NONE', #53387, #110093, #24514, .T. ) ;
#97077=CARTESIAN_POINT ( 'NONE',  ( 4.261662194147191052, 1515.372228416590133, 211.4517523138519834 ) ) ;
#97078=CARTESIAN_POINT ( 'NONE',  ( 4.781276783620000081, 1452.020048942890071, 190.5513815401990030 ) ) ;
#97079=CARTESIAN_POINT ( 'NONE',  ( -3.076366055149999834, 1424.853903601579987, 191.3970713258989917 ) ) ;
#97085=CARTESIAN_POINT ( 'NONE',  ( -1.993187091982024040, 1485.308211440273226, 198.1316096946227390 ) ) ;
#97095=CARTESIAN_POINT ( 'NONE',  ( 1.105873109660000075, 1515.456834174690130, 213.3233725384289983 ) ) ;
#97103=CARTESIAN_POINT ( 'NONE',  ( 2.154904617470000172, 1507.931312947989909, 220.6735988848989791 ) ) ;
#97115=CARTESIAN_POINT ( 'NONE',  ( 4.760896992130000172, 1449.971761959190189, 190.6385172635989704 ) ) ;
#97118=CARTESIAN_POINT ( 'NONE',  ( -2.740438610378060247, 1508.551704408389924, 204.1475582648899945 ) ) ;
#97121=ORIENTED_EDGE ( 'NONE', *, *, #108302, .F. ) ;
#97122=CARTESIAN_POINT ( 'NONE',  ( -1.418378755168210104, 1436.146031861469964, 227.5501453695390239 ) ) ;
#97130=CARTESIAN_POINT ( 'NONE',  ( 7.814950425870000217, 1425.209952447059777, 211.6921920394489973 ) ) ;
#97131=CARTESIAN_POINT ( 'NONE',  ( -0.3862240863000029889, 1500.063269133189806, 233.1571802061990013 ) ) ;
#97138=EDGE_LOOP ( 'NONE', ( #41114, #89420, #91355, #89446, #47968 ) ) ;
#97154=VERTEX_POINT ( 'NONE', #104557 ) ;
#97161=B_SPLINE_SURFACE_WITH_KNOTS ( 'NONE', 5, 1, ( 
 ( #80087, #58075 ),
 ( #15480, #49675 ),
 ( #7106, #63322 ),
 ( #20708, #16565 ),
 ( #43477, #69238 ),
 ( #933, #84895 ) ),
 .UNSPECIFIED., .F., .F., .F.,
 ( 6, 6 ),
 ( 2, 2 ),
 ( 0.000000000000000000, 3.596547541650000124 ),
 ( 0.000000000000000000, 14.00000000000000000 ),
 .UNSPECIFIED. ) ;
#97175=CARTESIAN_POINT ( 'NONE',  ( -5.303285988883490454, 1442.879254652209966, 200.5943008362860098 ) ) ;
#97180=CARTESIAN_POINT ( 'NONE',  ( 13.00946304068309978, 1426.713679829950024, 196.5727733038569909 ) ) ;
#97181=CARTESIAN_POINT ( 'NONE',  ( -17.55006637065400099, 1487.029424903359995, 194.9701071948420008 ) ) ;
#97189=CARTESIAN_POINT ( 'NONE',  ( -2.435720662160000050, 1429.409294711090070, 200.4602889503590006 ) ) ;
#97196=CARTESIAN_POINT ( 'NONE',  ( -16.28895431073521749, 1416.654488107960333, 208.3339384829398853 ) ) ;
#97198=CARTESIAN_POINT ( 'NONE',  ( 10.21694293408019938, 1469.929603999700021, 208.6439139955809878 ) ) ;
#97208=CARTESIAN_POINT ( 'NONE',  ( 1.786066050100000080, 1443.335463714089883, 217.8608858550190064 ) ) ;
#97211=CARTESIAN_POINT ( 'NONE',  ( 7.066689964004210012, 1470.190416163020245, 190.3198042189900150 ) ) ;
#97214=CARTESIAN_POINT ( 'NONE',  ( -19.41733818020000157, 1465.673979701889948, 205.2701344044189966 ) ) ;
#97221=CARTESIAN_POINT ( 'NONE',  ( -13.17280652390000029, 1508.540907300989829, 216.8072460398490193 ) ) ;
#97222=B_SPLINE_CURVE_WITH_KNOTS ( 'NONE', 5,
 ( #42761, #67432, #93149, #33242, #34356, #92592 ),
 .UNSPECIFIED., .F., .F.,
 ( 6, 6 ),
 ( -1.999999979519569981, 0.000000000000000000 ),
 .UNSPECIFIED. ) ;
#97226=CARTESIAN_POINT ( 'NONE',  ( -2.710273452790000093, 1484.982664535189770, 198.3319090041989909 ) ) ;
#97231=CARTESIAN_POINT ( 'NONE',  ( 5.989314528585920172, 1494.629792490379941, 219.4239423612390283 ) ) ;
#97232=CARTESIAN_POINT ( 'NONE',  ( -9.853265956016100446, 1488.872806762260097, 215.5614415617639850 ) ) ;
#97233=CARTESIAN_POINT ( 'NONE',  ( -13.32684181309999971, 1469.522592936189994, 191.9925905970989959 ) ) ;
#97252=CARTESIAN_POINT ( 'NONE',  ( -7.499365986679999985, 1445.290603318090007, 216.2717625584189989 ) ) ;
#97254=CARTESIAN_POINT ( 'NONE',  ( 0.2432117948283340214, 1515.155210303460080, 213.4489270742160159 ) ) ;
#97258=CARTESIAN_POINT ( 'NONE',  ( 1.396945595908719806, 1473.097535771269804, 219.2356281669150064 ) ) ;
#97264=CARTESIAN_POINT ( 'NONE',  ( 16.46134999639999563, 1495.070035120589864, 192.9350266946989905 ) ) ;
#97275=CARTESIAN_POINT ( 'NONE',  ( -8.977785982439998591, 1459.740360813789948, 212.8396695563389756 ) ) ;
#97291=CARTESIAN_POINT ( 'NONE',  ( 4.046802277660000335, 1505.460036802790000, 221.2327940266990254 ) ) ;
#97294=CARTESIAN_POINT ( 'NONE',  ( 5.133103592700000384, 1472.975266187489979, 218.0948351415289892 ) ) ;
#97296=CARTESIAN_POINT ( 'NONE',  ( 17.88377006740000397, 1429.006865431090091, 205.7968609931990045 ) ) ;
#97297=ORIENTED_EDGE ( 'NONE', *, *, #20601, .F. ) ;
#97303=EDGE_LOOP ( 'NONE', ( #10073, #99484, #62947, #3845 ) ) ;
#97304=EDGE_CURVE ( 'NONE', #86829, #2979, #46430, .T. ) ;
#97306=CARTESIAN_POINT ( 'NONE',  ( -0.8168899812832949303, 1467.671549419570056, 220.1953764921350114 ) ) ;
#97309=ADVANCED_FACE ( 'NONE', ( #50037 ), #95701, .F. ) ;
#97322=CARTESIAN_POINT ( 'NONE',  ( -4.987078442593329441, 1508.551704408389924, 211.6097810465890063 ) ) ;
#97328=CARTESIAN_POINT ( 'NONE',  ( 10.17747861530000009, 1489.224014057989962, 204.9037901253090013 ) ) ;
#97333=ORIENTED_EDGE ( 'NONE', *, *, #92582, .T. ) ;
#97346=CARTESIAN_POINT ( 'NONE',  ( -9.559981065551120594, 1460.552225690790237, 210.5447656127829816 ) ) ;
#97348=CARTESIAN_POINT ( 'NONE',  ( 10.03746411003220018, 1501.098977471080161, 203.4535166149570102 ) ) ;
#97362=CARTESIAN_POINT ( 'NONE',  ( -14.45258105951289807, 1415.677402202029953, 212.7925583759839867 ) ) ;
#97364=CARTESIAN_POINT ( 'NONE',  ( 9.395113974487038888, 1451.852228830569857, 209.9056078797769942 ) ) ;
#97366=B_SPLINE_CURVE_WITH_KNOTS ( 'NONE', 5,
 ( #75716, #58914, #16318, #58363, #110405, #7940 ),
 .UNSPECIFIED., .F., .F.,
 ( 6, 6 ),
 ( -2.000000000000000000, 0.000000000000000000 ),
 .UNSPECIFIED. ) ;
#97373=CARTESIAN_POINT ( 'NONE',  ( -12.04604675982380080, 1481.197891243110007, 227.9689080549119922 ) ) ;
#97378=ADVANCED_FACE ( 'NONE', ( #98632 ), #4587, .T. ) ;
#97380=CARTESIAN_POINT ( 'NONE',  ( -14.73654635989563033, 1420.116477539524567, 213.6061976603614596 ) ) ;
#97389=CARTESIAN_POINT ( 'NONE',  ( 10.83489300642449926, 1489.711129298920014, 207.6370862455599990 ) ) ;
#97391=ORIENTED_EDGE ( 'NONE', *, *, #73078, .T. ) ;
#97396=CARTESIAN_POINT ( 'NONE',  ( -3.190252885392550475, 1495.655215145649890, 197.2101252161220089 ) ) ;
#97397=EDGE_CURVE ( 'NONE', #43603, #86830, #83478, .T. ) ;
#97414=ADVANCED_FACE ( 'NONE', ( #16258 ), #78717, .T. ) ;
#97422=FACE_OUTER_BOUND ( 'NONE', #30680, .T. ) ;
#97425=CARTESIAN_POINT ( 'NONE',  ( 1.209344357960000282, 1487.394827286090049, 219.9223287670990032 ) ) ;
#97433=VERTEX_POINT ( 'NONE', #53789 ) ;
#97434=B_SPLINE_CURVE_WITH_KNOTS ( 'NONE', 3,
 ( #43214, #101984, #7935, #69536, #77363, #664, #17974, #93581, #34795, #51609, #17412, #33135, #67874, #59471, #16857, #33680, #18521, #102530, #67323, #25822, #10145, #51061, #34245, #84638, #85191, #42105, #85743, #24712, #60023, #52170 ),
 .UNSPECIFIED., .F., .F.,
 ( 4, 2, 2, 2, 1, 1, 1, 1, 2, 2, 2, 2, 1, 2, 2, 1, 2, 4 ),
 ( 0.000000000000000000, 0.2499999999997336020, 0.3749999999995978217, 0.4374999999995382582, 0.4687499999995027311, 0.4843749999994849675, 0.4921874999994722000, 0.4960937499994640953, 0.4980468749994599875, 0.4999999999994559352, 0.7499999999995180522, 0.8124999999995377031, 0.8281249999995426991, 0.8320312499995468070, 0.8359374999995510258, 0.8437499999995592415, 0.8749999999996469491, 1.000000000000000000 ),
 .UNSPECIFIED. ) ;
#97436=CARTESIAN_POINT ( 'NONE',  ( 9.200833838318960289, 1451.501850391510061, 210.2568363721279923 ) ) ;
#97437=CARTESIAN_POINT ( 'NONE',  ( 5.639791218109999171, 1424.329486380210028, 193.4460986586989861 ) ) ;
#97440=CARTESIAN_POINT ( 'NONE',  ( -5.815894185941668404, 1419.536499247897382, 194.8620236102833871 ) ) ;
#97450=ORIENTED_EDGE ( 'NONE', *, *, #105493, .F. ) ;
#97457=FACE_OUTER_BOUND ( 'NONE', #82617, .T. ) ;
#97459=CARTESIAN_POINT ( 'NONE',  ( 3.714835820328249660, 1497.588999516199920, 197.6014933246789838 ) ) ;
#97460=CARTESIAN_POINT ( 'NONE',  ( -8.267101759600800293, 1469.515716270360144, 216.2369933283739840 ) ) ;
#97462=CARTESIAN_POINT ( 'NONE',  ( 11.73531390670000008, 1420.449078066779975, 199.2341047989489766 ) ) ;
#97463=CARTESIAN_POINT ( 'NONE',  ( -2.391424667983720109, 1476.089688646680088, 220.3288384573359906 ) ) ;
#97465=LINE ( 'NONE', #13989, #12614 ) ;
#97467=CARTESIAN_POINT ( 'NONE',  ( -16.36114452500000027, 1503.966594772790131, 208.9878484538460270 ) ) ;
#97482=ORIENTED_EDGE ( 'NONE', *, *, #33518, .T. ) ;
#97486=CARTESIAN_POINT ( 'NONE',  ( 7.097349803439506388, 1439.093602098585052, 216.1529730758497010 ) ) ;
#97491=CARTESIAN_POINT ( 'NONE',  ( 8.522139007390389764, 1459.194399288350041, 203.0278343432409827 ) ) ;
#97494=CARTESIAN_POINT ( 'NONE',  ( -5.430946523250000268, 1476.595381090889987, 218.1965627062390354 ) ) ;
#97503=CARTESIAN_POINT ( 'NONE',  ( -14.28499805876190010, 1416.808594522969770, 203.2225434410350147 ) ) ;
#97507=CARTESIAN_POINT ( 'NONE',  ( 8.546316978770940764, 1428.346933653820088, 213.3379775298699883 ) ) ;
#97508=CARTESIAN_POINT ( 'NONE',  ( -3.984081752360000284, 1515.551704408389924, 207.2788837304390199 ) ) ;
#97511=CARTESIAN_POINT ( 'NONE',  ( 4.345191827429070841, 1455.903930675749962, 218.8175630227480042 ) ) ;
#97513=DIRECTION ( 'NONE',  ( -0.9625294240555893888, 6.236250047180620319E-07, -0.2711772627393869706 ) ) ;
#97526=CARTESIAN_POINT ( 'NONE',  ( -12.21562307281700122, 1490.700173189130055, 208.0633276266580083 ) ) ;
#97540=B_SPLINE_SURFACE_WITH_KNOTS ( 'NONE', 5, 5, ( 
 ( #16231, #52084, #59941, #42563, #33589, #67783 ),
 ( #101894, #25187, #28, #34161, #68347, #102453 ),
 ( #94058, #25740, #582, #17326, #51520, #68900 ),
 ( #103002, #24995, #67595, #108478, #101702, #92769 ),
 ( #39625, #24448, #6015, #100611, #14397, #75975 ),
 ( #110127, #40719, #32855, #48591, #65397, #31761 ),
 ( #23895, #91121, #49691, #92222, #41819, #7120 ),
 ( #93316, #16045, #73793, #100072, #33400, #56990 ),
 ( #5464, #107920, #59198, #82725, #58089, #50246 ) ),
 .UNSPECIFIED., .F., .F., .F.,
 ( 6, 3, 6 ),
 ( 6, 6 ),
 ( 3.064599166390000295, 5.269658684210000388, 7.474718202020000035 ),
 ( 0.000000000000000000, 2.000000000000000000 ),
 .UNSPECIFIED. ) ;
#97541=CARTESIAN_POINT ( 'NONE',  ( -2.777747345173310123, 1456.209076296149988, 202.9659044564290014 ) ) ;
#97542=CARTESIAN_POINT ( 'NONE',  ( -18.75153682899999907, 1469.211784502090040, 201.1821593617290205 ) ) ;
#97547=LINE ( 'NONE', #62898, #69904 ) ;
#97549=DIRECTION ( 'NONE',  ( 0.000000000000000000, -1.000000000000000000, 0.000000000000000000 ) ) ;
#97555=CARTESIAN_POINT ( 'NONE',  ( -8.952944454599998991, 1424.162919053179849, 206.7489373822789673 ) ) ;
#97562=ORIENTED_EDGE ( 'NONE', *, *, #55698, .F. ) ;
#97564=VECTOR ( 'NONE', #100642, 1000.000000000000000 ) ;
#97570=CARTESIAN_POINT ( 'NONE',  ( -0.8848931312460019960, 1467.694904068390088, 220.2161335405990314 ) ) ;
#97572=CARTESIAN_POINT ( 'NONE',  ( 10.47412083013409934, 1481.229225394920149, 212.5602164828920024 ) ) ;
#97575=AXIS2_PLACEMENT_3D ( 'NONE', #51295, #25524, #110101 ) ;
#97576=CARTESIAN_POINT ( 'NONE',  ( -20.02799630220000182, 1485.574563381989947, 204.1280247810589970 ) ) ;
#97578=CARTESIAN_POINT ( 'NONE',  ( 7.755379691499999062, 1459.738853293389866, 228.9106028235989925 ) ) ;
#97579=CARTESIAN_POINT ( 'NONE',  ( 7.560886196111736623, 1492.428349930449258, 217.3049961171652740 ) ) ;
#97582=ORIENTED_EDGE ( 'NONE', *, *, #27798, .F. ) ;
#97587=CARTESIAN_POINT ( 'NONE',  ( 10.78159632189999861, 1461.896570031590045, 211.1674760275290055 ) ) ;
#97591=DIRECTION ( 'NONE',  ( -0.04170409655914577435, 0.9849797009429184236, 0.1675582199135109140 ) ) ;
#97600=B_SPLINE_CURVE_WITH_KNOTS ( 'NONE', 3,
 ( #4367, #37963, #37409, #28456, #62650, #20042, #72144, #106262, #54237, #88363, #45829, #29548, #63734, #46934, #81052, #38496, #64282, #72673, #106798 ),
 .UNSPECIFIED., .F., .F.,
 ( 4, 3, 3, 3, 3, 3, 4 ),
 ( -7.611835603415659790, -7.445832134393750579, -6.293638100938689917, -5.367142758962240023, -4.666606357331840371, -3.867104339607819963, -3.122448789919999967 ),
 .UNSPECIFIED. ) ;
#97601=CARTESIAN_POINT ( 'NONE',  ( 11.43893751517350132, 1478.788528365839966, 206.4651667696550135 ) ) ;
#97608=CARTESIAN_POINT ( 'NONE',  ( -8.140676920415208073, 1436.358399980439799, 214.5433328127169830 ) ) ;
#97612=CARTESIAN_POINT ( 'NONE',  ( -4.632636518429999128, 1507.809020188690056, 221.0048302704990135 ) ) ;
#97614=CARTESIAN_POINT ( 'NONE',  ( 1.914156610164409855, 1431.087920293139859, 199.8421651263110164 ) ) ;
#97629=CARTESIAN_POINT ( 'NONE',  ( -15.62922400629999942, 1415.754093022550023, 208.9578334822819841 ) ) ;
#97634=CARTESIAN_POINT ( 'NONE',  ( 6.602631447940000342, 1463.509733493989870, 209.4768623231300069 ) ) ;
#97639=CARTESIAN_POINT ( 'NONE',  ( -0.7576697578790009269, 1515.544658147190148, 213.2443391230790155 ) ) ;
#97642=LINE ( 'NONE', #98733, #96002 ) ;
#97643=CARTESIAN_POINT ( 'NONE',  ( 19.45791513090297542, 1498.411990192014628, 218.7312280957626456 ) ) ;
#97645=B_SPLINE_CURVE_WITH_KNOTS ( 'NONE', 5,
 ( #72542, #44583, #106673, #29963, #64155, #18794 ),
 .UNSPECIFIED., .F., .F.,
 ( 6, 6 ),
 ( -2.000000000000000000, 0.000000000000000000 ),
 .UNSPECIFIED. ) ;
#97647=CARTESIAN_POINT ( 'NONE',  ( 10.62756433831671288, 1462.208184687777020, 211.9187829460415742 ) ) ;
#97653=CARTESIAN_POINT ( 'NONE',  ( 6.582297905418769801, 1467.177907444709945, 200.9815396461360137 ) ) ;
#97667=CARTESIAN_POINT ( 'NONE',  ( -11.39741020242381175, 1501.140956553491606, 208.2051223886542459 ) ) ;
#97668=CARTESIAN_POINT ( 'NONE',  ( -15.59833272758146094, 1415.960467561331143, 208.0431140678893485 ) ) ;
#97672=CARTESIAN_POINT ( 'NONE',  ( -5.376254996749998888E-14, 1377.913060387289988, 209.1218459616989946 ) ) ;
#97674=CARTESIAN_POINT ( 'NONE',  ( -4.646147325060000277, 1378.399971913189802, 203.6922293430689876 ) ) ;
#97675=CARTESIAN_POINT ( 'NONE',  ( 8.045781271640001009, 1426.290936267859934, 211.5934327219790134 ) ) ;
#97676=CARTESIAN_POINT ( 'NONE',  ( 10.59813991459999905, 1477.524080022390081, 229.9254213492990004 ) ) ;
#97683=ORIENTED_EDGE ( 'NONE', *, *, #69410, .T. ) ;
#97684=ADVANCED_FACE ( 'NONE', ( #7446 ), #90407, .T. ) ;
#97692=CARTESIAN_POINT ( 'NONE',  ( 8.454790733525280544, 1428.363638633589972, 213.4109935021670026 ) ) ;
#97694=FACE_OUTER_BOUND ( 'NONE', #81309, .T. ) ;
#97700=LINE ( 'NONE', #19877, #103701 ) ;
#97704=ORIENTED_EDGE ( 'NONE', *, *, #86035, .F. ) ;
#97706=CARTESIAN_POINT ( 'NONE',  ( -4.987793514269999839, 1425.174461588439954, 209.2447519049540006 ) ) ;
#97718=CARTESIAN_POINT ( 'NONE',  ( -11.93029924615809989, 1489.674051635599881, 211.7541755384660007 ) ) ;
#97734=CARTESIAN_POINT ( 'NONE',  ( 15.21359001291670054, 1427.479649557399853, 199.3000641055990059 ) ) ;
#97746=CARTESIAN_POINT ( 'NONE',  ( 11.13557732129999955, 1425.386704443429835, 204.8117771081390117 ) ) ;
#97749=CARTESIAN_POINT ( 'NONE',  ( -16.45607496635827616, 1416.877115859795595, 207.9322112222681938 ) ) ;
#97751=CARTESIAN_POINT ( 'NONE',  ( 10.17376127383159989, 1469.762723852360068, 208.1640156044039998 ) ) ;
#97755=VERTEX_POINT ( 'NONE', #80724 ) ;
#97756=CARTESIAN_POINT ( 'NONE',  ( 13.63295136444099853, 1492.115748128389896, 192.2627295947740151 ) ) ;
#97759=CARTESIAN_POINT ( 'NONE',  ( 8.059493427214674099, 1423.943097687976206, 195.8566467428261433 ) ) ;
#97760=CARTESIAN_POINT ( 'NONE',  ( 2.178538215579999715, 1442.258130819589951, 218.0918924510989996 ) ) ;
#97767=CARTESIAN_POINT ( 'NONE',  ( -15.62861691365340100, 1418.244675075289933, 203.0179649770489902 ) ) ;
#97769=CARTESIAN_POINT ( 'NONE',  ( -10.10912477582879987, 1472.430577810449904, 210.3411266470020280 ) ) ;
#97773=CARTESIAN_POINT ( 'NONE',  ( 11.31210319729820135, 1470.591574153610054, 207.8732379879190262 ) ) ;
#97774=FACE_OUTER_BOUND ( 'NONE', #99216, .T. ) ;
#97775=CARTESIAN_POINT ( 'NONE',  ( -16.59172940107149330, 1417.375819201424747, 206.4523686363734498 ) ) ;
#97779=CARTESIAN_POINT ( 'NONE',  ( 10.59812402283390043, 1477.524000194940072, 229.9254252251899970 ) ) ;
#97780=CARTESIAN_POINT ( 'NONE',  ( -15.34230038387189943, 1415.677402202110216, 209.0149701286740083 ) ) ;
#97782=( BOUNDED_CURVE ( )  B_SPLINE_CURVE ( 3, ( #40956, #24135, #48280, #91372 ),
 .UNSPECIFIED., .F., .F. ) 
 B_SPLINE_CURVE_WITH_KNOTS ( ( 4, 4 ),
 ( 2.356485377174994955, 3.926596519726254897 ),
 .UNSPECIFIED. ) 
 CURVE ( )  GEOMETRIC_REPRESENTATION_ITEM ( )  RATIONAL_B_SPLINE_CURVE ( ( 1.000000000000000000, 0.8048993259319946469, 0.8048993259319946469, 1.000000000000000000 ) ) 
 REPRESENTATION_ITEM ( '' )  );
#97783=CARTESIAN_POINT ( 'NONE',  ( 5.455371915589999787, 1427.707280442089768, 215.3790498620489871 ) ) ;
#97784=CARTESIAN_POINT ( 'NONE',  ( -18.44599904095050036, 1443.433905668329999, 212.7798859627189927 ) ) ;
#97789=ORIENTED_EDGE ( 'NONE', *, *, #23261, .T. ) ;
#97790=CARTESIAN_POINT ( 'NONE',  ( -20.35107102299999937, 1487.435604149590063, 205.0880641165789768 ) ) ;
#97803=CARTESIAN_POINT ( 'NONE',  ( 1.480922050692270009, 1515.075000927530027, 213.4510274295309955 ) ) ;
#97804=CARTESIAN_POINT ( 'NONE',  ( -9.973184873930010852, 1479.579336554859992, 215.2613112899330190 ) ) ;
#97809=CARTESIAN_POINT ( 'NONE',  ( -12.75669765699999836, 1503.496733507889985, 208.6968453557029761 ) ) ;
#97810=CARTESIAN_POINT ( 'NONE',  ( -22.14708463899999913, 1486.361880417990051, 217.3670993146189971 ) ) ;
#97815=CARTESIAN_POINT ( 'NONE',  ( 4.327148319165510237, 1515.152643786259887, 209.4426799714850347 ) ) ;
#97817=CIRCLE ( 'NONE', #1285, 3.750000000000000000 ) ;
#97827=CARTESIAN_POINT ( 'NONE',  ( -9.244110535254980832, 1447.194003664420052, 212.1343190185759795 ) ) ;
#97841=ORIENTED_EDGE ( 'NONE', *, *, #6256, .F. ) ;
#97846=CARTESIAN_POINT ( 'NONE',  ( -0.6623177435430670501, 1467.634584622510147, 220.2019122221780094 ) ) ;
#97847=CARTESIAN_POINT ( 'NONE',  ( -8.316672828268760753, 1425.055149638239982, 204.9623390585310005 ) ) ;
#97857=CARTESIAN_POINT ( 'NONE',  ( -7.604289863101939773, 1426.735970264149955, 206.0920986175900111 ) ) ;
#97861=CARTESIAN_POINT ( 'NONE',  ( -6.025152189795589308, 1484.743689720570046, 198.8560543189699956 ) ) ;
#97863=CARTESIAN_POINT ( 'NONE',  ( -9.175147725320000447, 1415.658347088709888, 205.8467875627789851 ) ) ;
#97875=CARTESIAN_POINT ( 'NONE',  ( -3.544886644340000448, 1474.831256732490147, 198.2487847239990231 ) ) ;
#97876=EDGE_CURVE ( 'NONE', #100109, #58839, #45252, .T. ) ;
#97891=ORIENTED_EDGE ( 'NONE', *, *, #44859, .F. ) ;
#97892=CARTESIAN_POINT ( 'NONE',  ( -2.487935123034410001, 1509.038615930399828, 213.6090957347729784 ) ) ;
#97895=CARTESIAN_POINT ( 'NONE',  ( -1.144427402640000091, 1442.540072109689845, 200.3174140758290207 ) ) ;
#97901=CARTESIAN_POINT ( 'NONE',  ( -2.480175250669919951, 1429.207669930499833, 200.0830571243679969 ) ) ;
#97903=CARTESIAN_POINT ( 'NONE',  ( -11.53021216923110082, 1501.524780145790146, 208.7332286060340039 ) ) ;
#97909=CARTESIAN_POINT ( 'NONE',  ( -3.411708654729999513, 1475.348535422589975, 198.9840501600990024 ) ) ;
#97912=CARTESIAN_POINT ( 'NONE',  ( -18.29179247696389865, 1466.060385685149868, 217.7541634367629797 ) ) ;
#97915=( BOUNDED_CURVE ( )  B_SPLINE_CURVE ( 3, ( #4066, #108701, #15708, #48266 ),
 .UNSPECIFIED., .F., .F. ) 
 B_SPLINE_CURVE_WITH_KNOTS ( ( 4, 4 ),
 ( 1.009833105023860034, 2.131759800080520240 ),
 .UNSPECIFIED. ) 
 CURVE ( )  GEOMETRIC_REPRESENTATION_ITEM ( )  RATIONAL_B_SPLINE_CURVE ( ( 1.000000000000000000, 0.8978286673593871559, 0.8978286673593871559, 1.000000000000000000 ) ) 
 REPRESENTATION_ITEM ( '' )  );
#97921=CARTESIAN_POINT ( 'NONE',  ( 10.29420224292342745, 1504.334860404003166, 214.4873101959476003 ) ) ;
#97922=CARTESIAN_POINT ( 'NONE',  ( 4.329448776274299249, 1515.064792882709980, 211.4519800890089982 ) ) ;
#97923=CARTESIAN_POINT ( 'NONE',  ( 20.41258333560000082, 1494.156730172889866, 204.1224707391089908 ) ) ;
#97935=CARTESIAN_POINT ( 'NONE',  ( -1.680260975536200130, 1496.115540335259993, 196.8918274691459942 ) ) ;
#97950=CARTESIAN_POINT ( 'NONE',  ( -0.7967037284469989933, 1496.366648252889945, 196.7585635602989953 ) ) ;
#97951=CARTESIAN_POINT ( 'NONE',  ( -4.461124787584389573, 1496.650352879389857, 201.9768976816139912 ) ) ;
#97960=CARTESIAN_POINT ( 'NONE',  ( 0.01339502592799870009, 1487.310215832789936, 219.9787594541990075 ) ) ;
#97970=CARTESIAN_POINT ( 'NONE',  ( 9.218373049180989653, 1451.410758823449896, 210.0413447373219924 ) ) ;
#97971=CARTESIAN_POINT ( 'NONE',  ( 5.057110678409999949, 1424.030137221399855, 193.7146012876989971 ) ) ;
#97975=CARTESIAN_POINT ( 'NONE',  ( 21.04904418909999819, 1494.916427559390058, 209.1218459616989946 ) ) ;
#97980=VERTEX_POINT ( 'NONE', #100134 ) ;
#97987=CARTESIAN_POINT ( 'NONE',  ( 8.437259666070110242, 1482.594120399739950, 217.4026692653139889 ) ) ;
#97992=CARTESIAN_POINT ( 'NONE',  ( -10.48469270268349796, 1480.274672445829992, 208.2228694171070345 ) ) ;
#97994=CARTESIAN_POINT ( 'NONE',  ( 2.371290244962170224, 1497.318959729730068, 197.3528097553119949 ) ) ;
#97995=CARTESIAN_POINT ( 'NONE',  ( -3.786808085590160022, 1468.516302267170204, 219.2555408501270051 ) ) ;
#97997=CARTESIAN_POINT ( 'NONE',  ( 9.220875156419999996, 1420.949518439220128, 196.8516559346990107 ) ) ;
#97998=CARTESIAN_POINT ( 'NONE',  ( -1.656993444572020024, 1475.839453786890090, 220.4462510233660169 ) ) ;
#98002=CARTESIAN_POINT ( 'NONE',  ( -16.23266583089999671, 1504.391494419190167, 208.8786546347319870 ) ) ;
#98005=AXIS2_PLACEMENT_3D ( 'NONE', #4975, #107434, #30729 ) ;
#98013=CARTESIAN_POINT ( 'NONE',  ( 4.114445074009999814, 1505.903523102289910, 220.4261431997990144 ) ) ;
#98014=CARTESIAN_POINT ( 'NONE',  ( -15.30092036139999934, 1415.735729274460027, 210.9263093465289955 ) ) ;
#98015=CARTESIAN_POINT ( 'NONE',  ( -16.35827608089219964, 1420.124075138139915, 209.1664405693819901 ) ) ;
#98016=VERTEX_POINT ( 'NONE', #92830 ) ;
#98018=CARTESIAN_POINT ( 'NONE',  ( 4.440855653409998993, 1430.031384578290044, 217.0414287054690021 ) ) ;
#98020=DIRECTION ( 'NONE',  ( 1.000000000000000000, 0.000000000000000000, 0.000000000000000000 ) ) ;
#98021=CARTESIAN_POINT ( 'NONE',  ( -0.9085210321814130019, 1429.982231419140135, 199.7651695299570065 ) ) ;
#98024=CARTESIAN_POINT ( 'NONE',  ( 1.548969699112269893, 1456.873934020939942, 199.3713766746409988 ) ) ;
#98043=CARTESIAN_POINT ( 'NONE',  ( -3.970164549730000214, 1515.569681836989957, 207.9977555470689765 ) ) ;
#98044=CARTESIAN_POINT ( 'NONE',  ( -0.7042569225233946684, 1484.127373294593099, 198.4525884679282512 ) ) ;
#98049=CARTESIAN_POINT ( 'NONE',  ( 1.847634023740000186, 1478.089546284990092, 198.8590795994990117 ) ) ;
#98051=CARTESIAN_POINT ( 'NONE',  ( -10.94025997009999962, 1492.428993089990172, 207.5139326340290040 ) ) ;
#98053=CARTESIAN_POINT ( 'NONE',  ( -4.602356253840000022, 1468.583955076089978, 189.7619545879989857 ) ) ;
#98062=B_SPLINE_SURFACE_WITH_KNOTS ( 'NONE', 5, 5, ( 
 ( #21289, #90722, #48751, #46550, #47634, #6167 ),
 ( #99111, #14006, #90163, #48193, #98018, #13444 ),
 ( #72303, #55496, #5066, #4533, #38667, #39213 ),
 ( #82331, #98569, #5631, #21838, #80684, #108072 ),
 ( #65550, #39782, #56036, #81763, #73391, #107526 ),
 ( #30816, #64993, #3996, #73941, #99659, #22950 ),
 ( #57155, #38121, #91280, #14560, #82874, #40321 ),
 ( #74503, #108632, #76136, #101301, #83421, #32485 ),
 ( #67202, #100759, #43093, #34128, #76683, #33556 ) ),
 .UNSPECIFIED., .F., .F., .F.,
 ( 6, 3, 6 ),
 ( 6, 6 ),
 ( 0.000000000000000000, 3.560296025780000040, 7.120592051560000080 ),
 ( 0.000000000000000000, 2.000000000000000000 ),
 .UNSPECIFIED. ) ;
#98065=CARTESIAN_POINT ( 'NONE',  ( -4.986724123564950872, 1508.551704408389924, 206.5918190285340188 ) ) ;
#98079=CARTESIAN_POINT ( 'NONE',  ( -13.21674774426140075, 1468.729004077370064, 191.9552650913620084 ) ) ;
#98085=CARTESIAN_POINT ( 'NONE',  ( -1966.823930461590180, 11221.53578756869865, -25.46789276350280318 ) ) ;
#98086=CARTESIAN_POINT ( 'NONE',  ( -20.64498752849999974, 1505.794066315190094, 209.1536330714710061 ) ) ;
#98091=CARTESIAN_POINT ( 'NONE',  ( -12.14581532088685201, 1421.748045606286951, 210.6453319782864071 ) ) ;
#98093=ORIENTED_EDGE ( 'NONE', *, *, #72193, .T. ) ;
#98109=CARTESIAN_POINT ( 'NONE',  ( -7.023365448820000800, 1481.189736218790131, 206.9209398003490037 ) ) ;
#98111=CARTESIAN_POINT ( 'NONE',  ( 2.740689650046610026, 1426.136172726640098, 188.7843778714569964 ) ) ;
#98112=CARTESIAN_POINT ( 'NONE',  ( -1.515897882684319908, 1431.595581664609881, 200.8620100226909813 ) ) ;
#98123=CARTESIAN_POINT ( 'NONE',  ( 1.055290578150000158, 1464.343017313090058, 199.3193465885090063 ) ) ;
#98139=CARTESIAN_POINT ( 'NONE',  ( -5.033671048615249610, 1434.259900860620064, 217.3302329488490159 ) ) ;
#98157=CARTESIAN_POINT ( 'NONE',  ( 5.745121365829383819, 1452.240402759911149, 190.7895842241696300 ) ) ;
#98164=CARTESIAN_POINT ( 'NONE',  ( -14.48519478120000059, 1416.181292573540304, 203.8595931902989946 ) ) ;
#98166=ADVANCED_FACE ( 'NONE', ( #108407 ), #62692, .F. ) ;
#98184=CARTESIAN_POINT ( 'NONE',  ( -5.208772481359999595, 1458.757019672090109, 218.5248626948989852 ) ) ;
#98210=ORIENTED_EDGE ( 'NONE', *, *, #46003, .T. ) ;
#98211=CARTESIAN_POINT ( 'NONE',  ( -4.066802226674130161, 1436.717946482039906, 227.1798391186449919 ) ) ;
#98217=CARTESIAN_POINT ( 'NONE',  ( -9.972208786350000409, 1449.536236232390138, 205.8362451147190200 ) ) ;
#98219=CARTESIAN_POINT ( 'NONE',  ( 7.445779770949999765, 1426.630704572389732, 212.5192353855690044 ) ) ;
#98222=LINE ( 'NONE', #12023, #18529 ) ;
#98237=B_SPLINE_CURVE_WITH_KNOTS ( 'NONE', 3,
 ( #77230, #11133, #34656, #26244, #69951, #27358 ),
 .UNSPECIFIED., .F., .F.,
 ( 4, 2, 4 ),
 ( 0.000000000000000000, 0.5000000000000000000, 1.000000000000000000 ),
 .UNSPECIFIED. ) ;
#98239=CARTESIAN_POINT ( 'NONE',  ( -1.954513284677499962, 1463.646611191549937, 199.5155506679120094 ) ) ;
#98246=EDGE_LOOP ( 'NONE', ( #22729, #13522, #36114, #30570 ) ) ;
#98258=ORIENTED_EDGE ( 'NONE', *, *, #13834, .F. ) ;
#98266=CARTESIAN_POINT ( 'NONE',  ( -12.03651488328679875, 1489.799716091139999, 211.2608063207809721 ) ) ;
#98280=CARTESIAN_POINT ( 'NONE',  ( 11.24070573841260057, 1426.193493941640099, 194.9955581729190044 ) ) ;
#98290=CARTESIAN_POINT ( 'NONE',  ( -4.987078426973329925, 1508.551704408389924, 206.6339106789369851 ) ) ;
#98293=CARTESIAN_POINT ( 'NONE',  ( 4.554962005479513465, 1508.731359867455467, 206.6339108206555295 ) ) ;
#98294=CARTESIAN_POINT ( 'NONE',  ( 3.767362825309999774, 1499.438298220989964, 230.0641493129989783 ) ) ;
#98295=CARTESIAN_POINT ( 'NONE',  ( 12.75748638139999969, 1426.660728386520077, 203.9418282069190127 ) ) ;
#98296=CARTESIAN_POINT ( 'NONE',  ( -1.872941326106300597, 1497.922954902849369, 197.9834655647225929 ) ) ;
#98298=CARTESIAN_POINT ( 'NONE',  ( -15.91787331746375500, 1416.014249173312919, 209.3106600495536611 ) ) ;
#98300=CARTESIAN_POINT ( 'NONE',  ( 10.95547293380590048, 1470.846847384059856, 209.2244093452740117 ) ) ;
#98308=CARTESIAN_POINT ( 'NONE',  ( 8.997154110830200224, 1425.027132644833046, 195.6828247586980183 ) ) ;
#98309=CARTESIAN_POINT ( 'NONE',  ( 0.7065304258729989684, 1442.384625720290160, 219.0605242788890052 ) ) ;
#98313=CARTESIAN_POINT ( 'NONE',  ( 8.267083892837330694, 1487.528308034231713, 202.1104332054804047 ) ) ;
#98321=CARTESIAN_POINT ( 'NONE',  ( -9.454311864350000150, 1508.539839826989919, 218.7120270370789967 ) ) ;
#98323=CARTESIAN_POINT ( 'NONE',  ( 10.30449505059999815, 1426.851415982049957, 209.1702054645420219 ) ) ;
#98330=EDGE_CURVE ( 'NONE', #65500, #105896, #51774, .T. ) ;
#98332=CARTESIAN_POINT ( 'NONE',  ( 19.12714383624729919, 1496.834757293069970, 222.0421909404099949 ) ) ;
#98333=CARTESIAN_POINT ( 'NONE',  ( -15.46337563405010052, 1415.677402202039957, 209.5778891453549875 ) ) ;
#98335=CARTESIAN_POINT ( 'NONE',  ( -9.631607308150519131, 1460.301351192619904, 209.7569760522880244 ) ) ;
#98336=CARTESIAN_POINT ( 'NONE',  ( 6.697438882680000205, 1428.609913361190138, 214.7541855357489737 ) ) ;
#98353=CARTESIAN_POINT ( 'NONE',  ( 20.45347777980000004, 1495.695647834889996, 214.2365953844490036 ) ) ;
#98355=CARTESIAN_POINT ( 'NONE',  ( 5.829580275110519239, 1467.124413742679963, 217.1880984370909857 ) ) ;
#98357=CARTESIAN_POINT ( 'NONE',  ( -0.5750010241229840391, 1515.139742041519867, 213.4493321248399980 ) ) ;
#98366=CARTESIAN_POINT ( 'NONE',  ( 16.47697133779999845, 1494.872252754689953, 192.9650186975990209 ) ) ;
#98373=CARTESIAN_POINT ( 'NONE',  ( 3.545373040442179935, 1484.694412436259881, 220.4261202662389962 ) ) ;
#98375=CARTESIAN_POINT ( 'NONE',  ( -5.540249615179999587, 1457.790387395490143, 216.9137936155790101 ) ) ;
#98382=ORIENTED_EDGE ( 'NONE', *, *, #95424, .F. ) ;
#98384=CARTESIAN_POINT ( 'NONE',  ( -8.908008619578920317, 1447.595509318989798, 212.1355612019459898 ) ) ;
#98386=SURFACE_SIDE_STYLE ('',( #65367 ) ) ;
#98393=CARTESIAN_POINT ( 'NONE',  ( 10.10526316670000035, 1471.402127257289976, 212.2219417807989998 ) ) ;
#98401=B_SPLINE_CURVE_WITH_KNOTS ( 'NONE', 3,
 ( #33333, #25477, #59670, #93780, #26593, #60222, #17618, #67528, #35000, #101628, #69180, #24917, #85961, #59127, #71415, #97122, #79785, #106611, #78666, #89265, #45091, #4171, #98211, #11470, #20939 ),
 .UNSPECIFIED., .F., .F.,
 ( 4, 3, 3, 3, 3, 3, 3, 3, 4 ),
 ( -3.448512466139999955, -2.538571452078679958, -1.628606578387550075, -0.7191125574035575063, -0.01266682060199997295, 0.9054669040022687021, 1.822853446759360008, 2.738681977611620244, 3.448512466139999955 ),
 .UNSPECIFIED. ) ;
#98403=CARTESIAN_POINT ( 'NONE',  ( -2.695307629501230373, 1424.941390411620205, 191.3270642277350078 ) ) ;
#98417=ORIENTED_EDGE ( 'NONE', *, *, #26966, .T. ) ;
#98422=CARTESIAN_POINT ( 'NONE',  ( -14.43714569989999852, 1417.316660727240105, 204.8390003888189881 ) ) ;
#98427=DIRECTION ( 'NONE',  ( -1.000000000000000000, 0.000000000000000000, 0.000000000000000000 ) ) ;
#98431=EDGE_LOOP ( 'NONE', ( #110825, #35564, #69515, #95690, #68308 ) ) ;
#98443=CARTESIAN_POINT ( 'NONE',  ( 0.8123333382153080651, 1456.028120524400038, 198.5934206245379983 ) ) ;
#98449=CARTESIAN_POINT ( 'NONE',  ( 8.165692104976699284, 1498.965027995250011, 200.4303008461249931 ) ) ;
#98451=CARTESIAN_POINT ( 'NONE',  ( 10.65095720820150049, 1480.263004433129936, 208.4908651385430005 ) ) ;
#98452=DIRECTION ( 'NONE',  ( 2.368020459168575969E-05, 1.033907832572708405E-06, -0.9999999997190894829 ) ) ;
#98453=CARTESIAN_POINT ( 'NONE',  ( -4.222176722049999498, 1443.314582379889771, 199.9747765569790090 ) ) ;
#98459=CARTESIAN_POINT ( 'NONE',  ( -2.472546487080370170, 1422.360492482099744, 192.6709265187130029 ) ) ;
#98463=CARTESIAN_POINT ( 'NONE',  ( 10.56407631929999980, 1452.658139941989930, 209.7432180256290053 ) ) ;
#98467=CARTESIAN_POINT ( 'NONE',  ( -3.501244980050000066, 1476.186593646489882, 199.3843432763690089 ) ) ;
#98470=CARTESIAN_POINT ( 'NONE',  ( 18.99432649145670027, 1459.501291662010090, 220.3864114681610147 ) ) ;
#98474=CARTESIAN_POINT ( 'NONE',  ( -0.5750466322259990548, 1484.101157922590119, 201.2237824415789760 ) ) ;
#98475=CARTESIAN_POINT ( 'NONE',  ( -10.32785587848439945, 1461.601613029019973, 211.2212836788939967 ) ) ;
#98477=CARTESIAN_POINT ( 'NONE',  ( 4.789673499540000101, 1465.867933640490037, 219.0700355186390027 ) ) ;
#98478=AXIS2_PLACEMENT_3D ( 'NONE', #30685, #63764, #55359 ) ;
#98485=CARTESIAN_POINT ( 'NONE',  ( 1.332267629549999902E-15, 1413.913060387330006, 209.1218459616989946 ) ) ;
#98486=ORIENTED_EDGE ( 'NONE', *, *, #89234, .T. ) ;
#98502=CARTESIAN_POINT ( 'NONE',  ( -8.634542021964680458, 1448.697323880249996, 212.1401996392050080 ) ) ;
#98507=CARTESIAN_POINT ( 'NONE',  ( 7.146076167249690414, 1424.928856607450143, 212.9496858538670097 ) ) ;
#98508=CARTESIAN_POINT ( 'NONE',  ( -5.175842961363289696, 1496.203461988439813, 202.5536918307219878 ) ) ;
#98517=CARTESIAN_POINT ( 'NONE',  ( -0.3150667361910010067, 1485.959260498290178, 221.0364148184989688 ) ) ;
#98520=CARTESIAN_POINT ( 'NONE',  ( -5.188151218920000751, 1391.908650948090099, 214.4790552262790015 ) ) ;
#98522=ORIENTED_EDGE ( 'NONE', *, *, #69186, .F. ) ;
#98525=CARTESIAN_POINT ( 'NONE',  ( 2.175409717514719593E-31, 1397.551704408390151, 209.1218459616989946 ) ) ;
#98526=ORIENTED_EDGE ( 'NONE', *, *, #15165, .T. ) ;
#98529=CARTESIAN_POINT ( 'NONE',  ( 6.440198200940000284, 1422.794610071979832, 195.1019709172990133 ) ) ;
#98532=CARTESIAN_POINT ( 'NONE',  ( 21.05584956750000103, 1495.071772848290038, 210.1533086104089989 ) ) ;
#98542=CARTESIAN_POINT ( 'NONE',  ( 11.23602576897910055, 1480.655328786240034, 212.7100351049870142 ) ) ;
#98543=CARTESIAN_POINT ( 'NONE',  ( 9.720077016953126758, 1480.309013615846879, 204.9736173252133540 ) ) ;
#98544=VERTEX_POINT ( 'NONE', #28691 ) ;
#98546=CARTESIAN_POINT ( 'NONE',  ( -3.163365581163430029, 1508.551704140590118, 220.1905023666739964 ) ) ;
#98547=CARTESIAN_POINT ( 'NONE',  ( 3.563478199850190098, 1497.907656018719990, 197.9170815786390278 ) ) ;
#98550=CARTESIAN_POINT ( 'NONE',  ( 11.78588353789999843, 1420.143588805510035, 199.1665921514089916 ) ) ;
#98557=CARTESIAN_POINT ( 'NONE',  ( 11.17902487211149953, 1422.624457870070046, 207.0208317409139909 ) ) ;
#98558=VECTOR ( 'NONE', #33314, 1000.000000000000114 ) ;
#98567=CARTESIAN_POINT ( 'NONE',  ( -17.35671359422410021, 1419.675078620990007, 207.6719667936040139 ) ) ;
#98569=CARTESIAN_POINT ( 'NONE',  ( 3.170476667209999988, 1429.217760481790037, 216.7986323648590030 ) ) ;
#98577=CONICAL_SURFACE ( 'NONE', #64644, 0.9999999999999962252, 1.047197551199999799 ) ;
#98578=( BOUNDED_CURVE ( )  B_SPLINE_CURVE ( 3, ( #21930, #90259, #47727, #66204 ),
 .UNSPECIFIED., .F., .T. ) 
 B_SPLINE_CURVE_WITH_KNOTS ( ( 4, 4 ),
 ( 4.168168146778059580, 5.256609830765320623 ),
 .UNSPECIFIED. ) 
 CURVE ( )  GEOMETRIC_REPRESENTATION_ITEM ( )  RATIONAL_B_SPLINE_CURVE ( ( 1.000000000000000000, 0.9036873071847475458, 0.9036873071847475458, 1.000000000000000000 ) ) 
 REPRESENTATION_ITEM ( '' )  );
#98579=CARTESIAN_POINT ( 'NONE',  ( 6.454732559708139306, 1459.182081823159933, 201.6346944821260081 ) ) ;
#98590=CARTESIAN_POINT ( 'NONE',  ( 0.008738962267850510293, 1515.558522550590169, 204.9671006875190074 ) ) ;
#98597=CARTESIAN_POINT ( 'NONE',  ( -4.274335294360000148, 1515.341803653790066, 207.6472638932690131 ) ) ;
#98603=CARTESIAN_POINT ( 'NONE',  ( 1.267691646300000086, 1484.678796645290049, 198.4480578130989841 ) ) ;
#98604=CARTESIAN_POINT ( 'NONE',  ( 6.999275391030000293, 1479.249878728790009, 201.1196786008089816 ) ) ;
#98606=CARTESIAN_POINT ( 'NONE',  ( -10.97260161140000001, 1492.335061974789824, 207.7727722944690072 ) ) ;
#98615=CARTESIAN_POINT ( 'NONE',  ( -8.117475352257454091, 1423.842526962705506, 210.5481715165687149 ) ) ;
#98622=CARTESIAN_POINT ( 'NONE',  ( 10.65764281875889985, 1471.555037556759771, 211.7634253889970068 ) ) ;
#98628=CARTESIAN_POINT ( 'NONE',  ( -18.71468957869999983, 1468.814975980689951, 201.1421764933589884 ) ) ;
#98632=FACE_OUTER_BOUND ( 'NONE', #29137, .T. ) ;
#98634=CARTESIAN_POINT ( 'NONE',  ( 1732.234191736389675, 11221.53578756870047, 2410.535515148488230 ) ) ;
#98641=CARTESIAN_POINT ( 'NONE',  ( -4.183240852922301301, 1454.059675636378415, 200.2646904393691614 ) ) ;
#98645=ORIENTED_EDGE ( 'NONE', *, *, #88592, .T. ) ;
#98648=CARTESIAN_POINT ( 'NONE',  ( -0.2453275326669540068, 1485.933059197169996, 221.0102401867029869 ) ) ;
#98653=EDGE_CURVE ( 'NONE', #26067, #63638, #19149, .T. ) ;
#98661=CARTESIAN_POINT ( 'NONE',  ( 10.65123798173899949, 1480.972066468270214, 211.8901002702700112 ) ) ;
#98663=EDGE_CURVE ( 'NONE', #86013, #37425, #39657, .T. ) ;
#98674=CARTESIAN_POINT ( 'NONE',  ( 12.46317070049899911, 1499.977136260429916, 206.8116722807479846 ) ) ;
#98675=CARTESIAN_POINT ( 'NONE',  ( -19.38790225612389762, 1508.451864247089816, 209.8663014701650127 ) ) ;
#98686=CARTESIAN_POINT ( 'NONE',  ( 9.436719802170449256, 1462.190294945330152, 206.7292107723660024 ) ) ;
#98694=CARTESIAN_POINT ( 'NONE',  ( -17.63263719517827255, 1508.456413885124675, 212.4308869866120517 ) ) ;
#98696=CARTESIAN_POINT ( 'NONE',  ( -9.580270985622490798, 1460.853522025070106, 207.7412804523160048 ) ) ;
#98700=ADVANCED_FACE ( 'NONE', ( #84584 ), #40761, .F. ) ;
#98707=CARTESIAN_POINT ( 'NONE',  ( -9.467068884459999722, 1450.246902653889947, 204.4311477998990085 ) ) ;
#98708=CARTESIAN_POINT ( 'NONE',  ( -10.35499315259030517, 1480.611330010711526, 207.1660253079129177 ) ) ;
#98711=CARTESIAN_POINT ( 'NONE',  ( 3.644352556201880144, 1515.551704204679936, 212.3939927026280259 ) ) ;
#98713=CARTESIAN_POINT ( 'NONE',  ( -5.007763590949999788, 1426.931744156050172, 207.4587325135290143 ) ) ;
#98718=CARTESIAN_POINT ( 'NONE',  ( -20.31208665306889927, 1487.462847046120032, 204.9267914088850091 ) ) ;
#98719=CARTESIAN_POINT ( 'NONE',  ( -6.031237335843999681, 1442.578951278860131, 201.0497613954999849 ) ) ;
#98729=CARTESIAN_POINT ( 'NONE',  ( 10.95851507883410036, 1490.212960435480227, 209.1823932077190022 ) ) ;
#98730=ADVANCED_FACE ( 'NONE', ( #68371 ), #88001, .F. ) ;
#98733=CARTESIAN_POINT ( 'NONE',  ( -3.523962701577560086, 1476.511731529740018, 220.0526012636759958 ) ) ;
#98736=CARTESIAN_POINT ( 'NONE',  ( -10.07052356819160188, 1447.097068999800058, 211.4090694554620029 ) ) ;
#98741=CARTESIAN_POINT ( 'NONE',  ( -4.201107383170000098, 1515.456955069990045, 210.2333507927889968 ) ) ;
#98754=CARTESIAN_POINT ( 'NONE',  ( 12.16396381444949881, 1491.556051155780096, 207.3115473875270141 ) ) ;
#98765=CARTESIAN_POINT ( 'NONE',  ( -16.23751604409000038, 1416.676673989810070, 209.1091032500480082 ) ) ;
#98769=CARTESIAN_POINT ( 'NONE',  ( -6.964608808889999558, 1453.224209856889956, 202.7117130979790147 ) ) ;
#98771=CARTESIAN_POINT ( 'NONE',  ( 7.909027525009999948, 1426.208968979389965, 211.6952151749889879 ) ) ;
#98772=CARTESIAN_POINT ( 'NONE',  ( -13.67845557849999949, 1504.250295190390034, 227.6838176112990197 ) ) ;
#98774=CARTESIAN_POINT ( 'NONE',  ( -21.16165221186960110, 1418.123385324889796, 208.6155873984789935 ) ) ;
#98777=CARTESIAN_POINT ( 'NONE',  ( 8.850386993630001697, 1454.013591409390074, 214.2286051505190017 ) ) ;
#98779=VERTEX_POINT ( 'NONE', #91750 ) ;
#98788=CARTESIAN_POINT ( 'NONE',  ( -21.53565904410000087, 1506.077647802389947, 209.2113159668039941 ) ) ;
#98791=CARTESIAN_POINT ( 'NONE',  ( -4.467442984997470390, 1464.039775823070158, 199.9285363783119749 ) ) ;
#98799=FACE_OUTER_BOUND ( 'NONE', #33778, .T. ) ;
#98803=CARTESIAN_POINT ( 'NONE',  ( -5.010776572990000233, 1425.617167130440066, 208.7696333329660092 ) ) ;
#98811=CARTESIAN_POINT ( 'NONE',  ( -18.59685951017700134, 1508.551704410880120, 210.2475276029339852 ) ) ;
#98818=CARTESIAN_POINT ( 'NONE',  ( -9.154585039681560232, 1450.683066379740012, 207.9130041143549761 ) ) ;
#98823=ADVANCED_FACE ( 'NONE', ( #39988 ), #10787, .T. ) ;
#98826=B_SPLINE_CURVE_WITH_KNOTS ( 'NONE', 5,
 ( #45411, #3958, #86835, #44862, #79552, #71169 ),
 .UNSPECIFIED., .F., .F.,
 ( 6, 6 ),
 ( -2.000000000000000000, 0.000000000000000000 ),
 .UNSPECIFIED. ) ;
#98847=CARTESIAN_POINT ( 'NONE',  ( 11.41335056429999995, 1426.197677042169971, 205.8024195469589870 ) ) ;
#98853=ORIENTED_EDGE ( 'NONE', *, *, #31658, .F. ) ;
#98859=CARTESIAN_POINT ( 'NONE',  ( 10.79317411587489950, 1461.870335762409923, 211.1042069659010281 ) ) ;
#98860=CARTESIAN_POINT ( 'NONE',  ( 9.226840260308872388, 1425.198049312735975, 195.6167264984963765 ) ) ;
#98861=CARTESIAN_POINT ( 'NONE',  ( 2.232433900040000196, 1443.114183221789972, 217.7415636394590024 ) ) ;
#98863=CARTESIAN_POINT ( 'NONE',  ( 9.093901123017769095, 1470.494570018200193, 191.1297851741429952 ) ) ;
#98865=CARTESIAN_POINT ( 'NONE',  ( -20.26467651240000123, 1485.408278981489957, 205.1073287502989899 ) ) ;
#98870=CARTESIAN_POINT ( 'NONE',  ( -9.856202761009180691, 1472.140734045829959, 211.6206523853309704 ) ) ;
#98875=CARTESIAN_POINT ( 'NONE',  ( 11.38728035538260208, 1470.834447203169930, 208.6597894033529883 ) ) ;
#98881=CARTESIAN_POINT ( 'NONE',  ( 4.164418577872849525, 1494.305047636430118, 219.6348937993929837 ) ) ;
#98885=CARTESIAN_POINT ( 'NONE',  ( 7.605961836409999677, 1428.548125308290082, 214.1230708307590191 ) ) ;
#98886=CARTESIAN_POINT ( 'NONE',  ( -18.78579970166540036, 1443.967530420280127, 210.3883505492739801 ) ) ;
#98892=CARTESIAN_POINT ( 'NONE',  ( -11.42085373749999988, 1500.664288093890036, 209.5050427136080202 ) ) ;
#98899=CARTESIAN_POINT ( 'NONE',  ( 0.000000000000000000, 1512.051704408390151, 209.1218459616989946 ) ) ;
#98901=CARTESIAN_POINT ( 'NONE',  ( 9.207476614228639278, 1464.697200489039915, 212.6097977664159941 ) ) ;
#98903=CARTESIAN_POINT ( 'NONE',  ( 1.251490820293549966, 1515.089511802750167, 213.4506474497650004 ) ) ;
#98905=CARTESIAN_POINT ( 'NONE',  ( -7.933021179928469557, 1478.422619274720091, 217.6197839746220097 ) ) ;
#98911=CARTESIAN_POINT ( 'NONE',  ( -11.56701740770000164, 1505.460402719889998, 207.8473594444390073 ) ) ;
#98912=CARTESIAN_POINT ( 'NONE',  ( -21.46116573947509920, 1504.834610015079988, 215.7390694031070097 ) ) ;
#98920=CARTESIAN_POINT ( 'NONE',  ( 3.394586470828380165, 1484.752177860970050, 220.4731790445629827 ) ) ;
#98922=CARTESIAN_POINT ( 'NONE',  ( -5.729479221760000129, 1458.872054288590107, 217.7597387405890288 ) ) ;
#98941=CARTESIAN_POINT ( 'NONE',  ( -6.338192872240000497, 1481.865655818189907, 205.0401094726289841 ) ) ;
#98945=ORIENTED_EDGE ( 'NONE', *, *, #52190, .T. ) ;
#98948=CARTESIAN_POINT ( 'NONE',  ( 2.976200793056689609, 1426.218032820240069, 191.3194850719970077 ) ) ;
#98953=CARTESIAN_POINT ( 'NONE',  ( 9.146299198640271300, 1461.861878385089767, 205.8341600298289791 ) ) ;
#98955=CARTESIAN_POINT ( 'NONE',  ( 6.624757470297610418, 1440.385568604370064, 215.0349520669070102 ) ) ;
#98967=CARTESIAN_POINT ( 'NONE',  ( -16.53125420670000167, 1418.541487540729804, 202.7561987471289910 ) ) ;
#98970=CARTESIAN_POINT ( 'NONE',  ( 10.79528401680000016, 1489.628194867089860, 207.4012257089289903 ) ) ;
#98975=ORIENTED_EDGE ( 'NONE', *, *, #95240, .T. ) ;
#98980=CARTESIAN_POINT ( 'NONE',  ( -2.990731931200000471, 1475.888290570790105, 219.4132863883990296 ) ) ;
#98991=CARTESIAN_POINT ( 'NONE',  ( 10.68058308266429890, 1480.421846638939996, 209.0069263140630085 ) ) ;
#98993=CARTESIAN_POINT ( 'NONE',  ( -2.705330512559999789, 1443.650354199390222, 199.8402550512289793 ) ) ;
#98996=DIRECTION ( 'NONE',  ( 0.9532327469067780612, 0.2978772346122090520, -0.05115157206129060385 ) ) ;
#98997=CARTESIAN_POINT ( 'NONE',  ( 2.154110967345579830, 1508.551704408389924, 219.6365568787950338 ) ) ;
#99001=CARTESIAN_POINT ( 'NONE',  ( -11.58641202078170096, 1501.658531164619944, 208.7684197680320040 ) ) ;
#99003=B_SPLINE_CURVE_WITH_KNOTS ( 'NONE', 3,
 ( #57640, #92304, #25644, #42459, #67690, #33488, #32947, #23981, #59292, #58175, #40805, #93409, #74984, #8297, #16674, #8846, #41918, #15574, #43029, #83907, #67137, #92858, #41371, #34060, #58723 ),
 .UNSPECIFIED., .F., .F.,
 ( 4, 3, 3, 3, 3, 3, 3, 3, 4 ),
 ( 0.000000000000000000, 1.234047661610760072, 2.425972046132570448, 3.560296027315850154, 4.348419011639929721, 5.612354531546630554, 6.366473291553310432, 7.034225416716780366, 7.120592051560000080 ),
 .UNSPECIFIED. ) ;
#99005=ORIENTED_EDGE ( 'NONE', *, *, #39902, .F. ) ;
#99008=CARTESIAN_POINT ( 'NONE',  ( 4.604592056516840337, 1508.551704408389924, 205.3031616744609948 ) ) ;
#99011=CARTESIAN_POINT ( 'NONE',  ( 20.56231333760889868, 1477.111373227550075, 217.7195205697740050 ) ) ;
#99012=ORIENTED_EDGE ( 'NONE', *, *, #54901, .T. ) ;
#99014=CARTESIAN_POINT ( 'NONE',  ( -2.958097658349249759, 1515.068899390480283, 204.7924306805940091 ) ) ;
#99029=ORIENTED_EDGE ( 'NONE', *, *, #2899, .F. ) ;
#99034=CARTESIAN_POINT ( 'NONE',  ( 12.73828631345009832, 1420.788157922979963, 202.0023175873409969 ) ) ;
#99043=CARTESIAN_POINT ( 'NONE',  ( -10.16501911979129957, 1447.237709317130111, 211.0287244977210150 ) ) ;
#99048=CARTESIAN_POINT ( 'NONE',  ( 7.216878188901039159, 1424.962458274039818, 212.8178266198389963 ) ) ;
#99053=CARTESIAN_POINT ( 'NONE',  ( -11.65129296574880158, 1491.369970010279985, 206.7844079078949733 ) ) ;
#99067=CARTESIAN_POINT ( 'NONE',  ( 9.695032739815491851, 1452.327451679549995, 210.0352081693090156 ) ) ;
#99068=CARTESIAN_POINT ( 'NONE',  ( 6.577796586379999866, 1424.576947660639917, 193.8008614473990008 ) ) ;
#99071=LINE ( 'NONE', #90124, #15163 ) ;
#99077=CARTESIAN_POINT ( 'NONE',  ( -7.973546373919998764, 1425.245985973290090, 205.1887633420689667 ) ) ;
#99084=EDGE_LOOP ( 'NONE', ( #41466, #8470, #99005, #3497 ) ) ;
#99086=CARTESIAN_POINT ( 'NONE',  ( 2.911802205207963734, 1507.562757914708527, 220.4805861716940001 ) ) ;
#99098=CARTESIAN_POINT ( 'NONE',  ( 10.67506506432800073, 1424.493056960179956, 206.5997893278160120 ) ) ;
#99101=ORIENTED_EDGE ( 'NONE', *, *, #37770, .F. ) ;
#99108=CARTESIAN_POINT ( 'NONE',  ( 10.17360721298319959, 1426.903618366670116, 209.4281458372120142 ) ) ;
#99109=CARTESIAN_POINT ( 'NONE',  ( -15.83960918336639878, 1420.111814593369900, 210.7068784591650115 ) ) ;
#99111=CARTESIAN_POINT ( 'NONE',  ( 3.661554943190000078, 1428.528251320389927, 216.5381528549790175 ) ) ;
#99117=CARTESIAN_POINT ( 'NONE',  ( 1.779422250252779891, 1456.357346840630044, 198.6855212002049882 ) ) ;
#99118=CARTESIAN_POINT ( 'NONE',  ( 7.479166282266099586, 1423.852740058520112, 195.4333272129960051 ) ) ;
#99128=LINE ( 'NONE', #82896, #52776 ) ;
#99130=TOROIDAL_SURFACE ( 'NONE', #79510, 12.73448142120000171, 1.000000000000000000 ) ;
#99132=B_SPLINE_CURVE_WITH_KNOTS ( 'NONE', 3,
 ( #101684, #59721, #61396, #50226 ),
 .UNSPECIFIED., .F., .F.,
 ( 4, 4 ),
 ( 0.000000000000000000, 1.000000000000000000 ),
 .UNSPECIFIED. ) ;
#99144=CARTESIAN_POINT ( 'NONE',  ( -0.8597107442289990686, 1463.363299246390170, 202.2013017290789776 ) ) ;
#99151=CARTESIAN_POINT ( 'NONE',  ( -12.25211328800230071, 1490.425571931200011, 208.9817620660529940 ) ) ;
#99158=CARTESIAN_POINT ( 'NONE',  ( 9.861354742171270615, 1470.940182288200049, 211.9688742596949851 ) ) ;
#99165=CARTESIAN_POINT ( 'NONE',  ( -16.59693199761399995, 1464.025901459640181, 220.5208652158270013 ) ) ;
#99167=CARTESIAN_POINT ( 'NONE',  ( 3.862828020359158732, 1497.382717227735611, 197.2227926766582300 ) ) ;
#99173=AXIS2_PLACEMENT_3D ( 'NONE', #78175, #61968, #70929 ) ;
#99184=ORIENTED_EDGE ( 'NONE', *, *, #74895, .F. ) ;
#99187=CARTESIAN_POINT ( 'NONE',  ( -1.583985751884120052, 1486.289433825739934, 220.9322661043319727 ) ) ;
#99188=CARTESIAN_POINT ( 'NONE',  ( 11.51819234920000135, 1500.360414606190034, 206.3631727204690094 ) ) ;
#99194=CARTESIAN_POINT ( 'NONE',  ( 3.556995324409999881, 1476.475065048189890, 198.0947962222990100 ) ) ;
#99195=CARTESIAN_POINT ( 'NONE',  ( 11.55223054067229960, 1480.217571523739934, 211.4788428327300380 ) ) ;
#99200=CARTESIAN_POINT ( 'NONE',  ( -17.55008888309999904, 1487.029577685089862, 194.9701234138989889 ) ) ;
#99201=CARTESIAN_POINT ( 'NONE',  ( -1.955843867788469970, 1431.363043548789847, 200.9645343544800085 ) ) ;
#99202=ORIENTED_EDGE ( 'NONE', *, *, #20631, .F. ) ;
#99211=CARTESIAN_POINT ( 'NONE',  ( -5.100957845159999948, 1482.122785942490054, 228.9672709512990139 ) ) ;
#99216=EDGE_LOOP ( 'NONE', ( #68551, #55468, #26930, #57145 ) ) ;
#99226=CARTESIAN_POINT ( 'NONE',  ( -16.99050533527280038, 1420.323706995179919, 203.8408272025779979 ) ) ;
#99227=CARTESIAN_POINT ( 'NONE',  ( -8.672201264859550562, 1436.845892416930155, 213.7190775223999992 ) ) ;
#99228=DIRECTION ( 'NONE',  ( 0.6205445805634681733, -0.7071067811868638753, -0.3390050494208928233 ) ) ;
#99243=CARTESIAN_POINT ( 'NONE',  ( 4.259777688362279768, 1515.374151772610048, 212.0586625277509825 ) ) ;
#99244=CARTESIAN_POINT ( 'NONE',  ( -2.171184902437989894, 1483.765132005870100, 198.6683033559409921 ) ) ;
#99248=CARTESIAN_POINT ( 'NONE',  ( 1.909107468240000216, 1507.666028269690059, 220.7249166300989884 ) ) ;
#99250=CARTESIAN_POINT ( 'NONE',  ( 4.208240993269999564, 1434.939300248989866, 227.0651965576989824 ) ) ;
#99251=B_SPLINE_CURVE_WITH_KNOTS ( 'NONE', 5,
 ( #31432, #81829, #39289, #82404, #73463, #74008, #56655, #25082, #33482, #98086, #107594, #108139 ),
 .UNSPECIFIED., .F., .F.,
 ( 6, 3, 3, 6 ),
 ( -18.25602225929999989, -13.68355489660000046, -9.538385084389998880, -6.066676742310001202 ),
 .UNSPECIFIED. ) ;
#99252=CARTESIAN_POINT ( 'NONE',  ( -8.519718778234439682, 1440.842058268650135, 204.6679085666960134 ) ) ;
#99255=CARTESIAN_POINT ( 'NONE',  ( -9.119413322219999785, 1439.059527644790023, 208.3668177869740248 ) ) ;
#99257=CARTESIAN_POINT ( 'NONE',  ( -21.10083498417930059, 1505.340688622180096, 209.5899059317720230 ) ) ;
#99271=CARTESIAN_POINT ( 'NONE',  ( -7.211414364699999524, 1427.415731310709816, 205.0259060341190320 ) ) ;
#99275=CARTESIAN_POINT ( 'NONE',  ( -1.951848414609999915, 1509.046756045790062, 220.7383877411990056 ) ) ;
#99276=CARTESIAN_POINT ( 'NONE',  ( -3.970093244310000102, 1515.569676282289947, 210.2462954219890037 ) ) ;
#99286=CARTESIAN_POINT ( 'NONE',  ( -21.13622131300000007, 1506.830164498290060, 213.5433617895989755 ) ) ;
#99292=EDGE_CURVE ( 'NONE', #508, #8596, #67631, .T. ) ;
#99296=CARTESIAN_POINT ( 'NONE',  ( -6.821020807950000098, 1472.286670839089766, 210.4001276167389847 ) ) ;
#99299=CARTESIAN_POINT ( 'NONE',  ( 18.94655734006379788, 1455.761339616339910, 200.3458083268320138 ) ) ;
#99306=CARTESIAN_POINT ( 'NONE',  ( 7.792129069010000464, 1426.255977840449987, 211.8493891909589877 ) ) ;
#99314=CARTESIAN_POINT ( 'NONE',  ( 9.480877448319999345, 1453.580774491189914, 212.8767779103989994 ) ) ;
#99315=ORIENTED_EDGE ( 'NONE', *, *, #94120, .T. ) ;
#99316=EDGE_LOOP ( 'NONE', ( #4607, #87387, #80599 ) ) ;
#99322=CARTESIAN_POINT ( 'NONE',  ( 2.958096254149829907, 1515.068899375750107, 204.7924306969019881 ) ) ;
#99323=CARTESIAN_POINT ( 'NONE',  ( 3.297786611580000304, 1446.227577985589960, 199.9593576464789919 ) ) ;
#99326=CARTESIAN_POINT ( 'NONE',  ( -4.151903202082950273, 1464.101420083999983, 199.7805968759980146 ) ) ;
#99335=ORIENTED_EDGE ( 'NONE', *, *, #95331, .T. ) ;
#99344=CARTESIAN_POINT ( 'NONE',  ( -11.65393960900000003, 1502.937255890489951, 208.0196683168489926 ) ) ;
#99362=EDGE_CURVE ( 'NONE', #100441, #19417, #19275, .T. ) ;
#99385=CARTESIAN_POINT ( 'NONE',  ( 11.13078225340000138, 1425.146663512289933, 203.3901361119889941 ) ) ;
#99386=CARTESIAN_POINT ( 'NONE',  ( -1.116803387759635502, 1498.149304908504519, 197.8710347455017313 ) ) ;
#99390=CARTESIAN_POINT ( 'NONE',  ( -0.6219649468940665615, 1515.589553500699594, 205.1020666507063481 ) ) ;
#99400=CARTESIAN_POINT ( 'NONE',  ( 2.106115005279999952, 1442.705724707790068, 217.8803785435890177 ) ) ;
#99413=CARTESIAN_POINT ( 'NONE',  ( 9.912692182420000719, 1426.220680563049882, 209.0669814966779825 ) ) ;
#99423=CARTESIAN_POINT ( 'NONE',  ( -15.84432591830269743, 1419.853212859319910, 210.7451195136700051 ) ) ;
#99431=ORIENTED_EDGE ( 'NONE', *, *, #85906, .T. ) ;
#99432=CARTESIAN_POINT ( 'NONE',  ( -11.41402577200000223, 1500.969831348989828, 208.5831151415709996 ) ) ;
#99434=CARTESIAN_POINT ( 'NONE',  ( 2.358876809229999871, 1455.879957205790106, 218.6867517008690243 ) ) ;
#99436=CARTESIAN_POINT ( 'NONE',  ( 8.927028317280980119, 1436.767930426870180, 210.5805728413830025 ) ) ;
#99440=CARTESIAN_POINT ( 'NONE',  ( -4.994775864380000208, 1391.713558696990049, 203.8075142969990168 ) ) ;
#99441=CARTESIAN_POINT ( 'NONE',  ( 9.581777264995830379, 1464.075427050579947, 211.2528481700169891 ) ) ;
#99443=CARTESIAN_POINT ( 'NONE',  ( 1.407451548163070054, 1515.079400017670196, 213.4509122356359967 ) ) ;
#99444=EDGE_CURVE ( 'NONE', #100441, #82285, #78322, .T. ) ;
#99445=CARTESIAN_POINT ( 'NONE',  ( -4.102794113347690619, 1453.855854241320003, 199.4852768663029963 ) ) ;
#99454=CARTESIAN_POINT ( 'NONE',  ( 24.13249860440000205, 1497.226937179990045, 206.7234963521489988 ) ) ;
#99461=CARTESIAN_POINT ( 'NONE',  ( 9.986161364699151832, 1468.785215375359940, 208.2634456866570076 ) ) ;
#99462=CARTESIAN_POINT ( 'NONE',  ( -2.330134126090000368, 1515.064792882589927, 204.7923971856590128 ) ) ;
#99473=CARTESIAN_POINT ( 'NONE',  ( -17.64860873675443287, 1419.496838671263504, 207.1709281612535563 ) ) ;
#99478=CARTESIAN_POINT ( 'NONE',  ( 9.788141037149998169, 1471.003676308989952, 212.2094846091489728 ) ) ;
#99484=ORIENTED_EDGE ( 'NONE', *, *, #69870, .T. ) ;
#99489=ADVANCED_FACE ( 'NONE', ( #35536 ), #7920, .T. ) ;
#99495=CARTESIAN_POINT ( 'NONE',  ( 0.9598037665343115421, 1421.307034539813685, 193.7451072252824247 ) ) ;
#99496=CARTESIAN_POINT ( 'NONE',  ( 5.819172478703739770, 1440.531633204680020, 216.0087162162849665 ) ) ;
#99509=DIRECTION ( 'NONE',  ( 1.224646799147350002E-16, -1.836970198721029688E-16, -1.000000000000000000 ) ) ;
#99522=TOROIDAL_SURFACE ( 'NONE', #95959, 10.10241613150000006, 2.000000000000000000 ) ;
#99523=B_SPLINE_CURVE_WITH_KNOTS ( 'NONE', 3,
 ( #53072, #70441, #36808, #70999, #28409, #62607, #96722, #54188, #56371, #5402, #39561, #105681, #4318, #55835, #55284, #91052, #107312, #56922, #46886, #37362, #98357, #20531, #28965, #63690, #38449, #21080, #90502, #89414, #80470, #47420, #12702, #81011, #13780, #72621, #97254, #29497, #106753, #54736, #30042, #63155, #64794, #38990, #64234, #81543, #31147, #107858, #47961, #82104, #73735, #65335, #98903, #21629, #106215, #46341, #99443, #97803, #3786, #22720, #45786, #88865, #79921 ),
 .UNSPECIFIED., .F., .F.,
 ( 4, 3, 3, 3, 3, 3, 3, 3, 3, 3, 3, 3, 3, 3, 3, 3, 3, 3, 3, 3, 4 ),
 ( 2.324858856890000158, 2.629298819987540003, 2.933834190021629595, 3.016888080810000261, 3.323211181039090079, 3.630193766034540026, 3.937176351030000188, 4.233214320285879850, 4.526002641956389461, 4.813615658896620353, 4.970096098099999971, 5.257590953083679963, 5.548112191535929938, 5.843468099036670083, 6.019659498159999345, 6.321166958453420470, 6.626011430626180143, 6.935803168058399137, 7.053491825919998348, 7.364378125606098280, 7.657659707949999728 ),
 .UNSPECIFIED. ) ;
#99525=CARTESIAN_POINT ( 'NONE',  ( 1.326883316820000269, 1474.953498172789978, 220.4794457010989959 ) ) ;
#99530=CARTESIAN_POINT ( 'NONE',  ( 0.6680169871064080001, 1455.976695232599923, 198.5860125881739862 ) ) ;
#99531=EDGE_CURVE ( 'NONE', #103262, #5409, #29967, .T. ) ;
#99534=CARTESIAN_POINT ( 'NONE',  ( -10.49702031989500028, 1471.002758439979971, 210.3192899704120293 ) ) ;
#99535=CARTESIAN_POINT ( 'NONE',  ( -3.441085789689999785, 1476.342819426989990, 219.6507253252989926 ) ) ;
#99536=CARTESIAN_POINT ( 'NONE',  ( 0.7998021860399979754, 1481.092795404789968, 229.6971392698989973 ) ) ;
#99538=ADVANCED_FACE ( 'NONE', ( #64075 ), #49661, .T. ) ;
#99539=ORIENTED_EDGE ( 'NONE', *, *, #42452, .F. ) ;
#99540=CARTESIAN_POINT ( 'NONE',  ( -2.487935123034410001, 1508.783371655767951, 213.6678281891418578 ) ) ;
#99541=ADVANCED_FACE ( 'NONE', ( #70291 ), #24880, .T. ) ;
#99543=CARTESIAN_POINT ( 'NONE',  ( -4.014584143420000473, 1443.145720380289958, 200.3327953268290287 ) ) ;
#99544=CARTESIAN_POINT ( 'NONE',  ( 11.72073075646250118, 1501.840823038659892, 211.4460601384429879 ) ) ;
#99553=B_SPLINE_CURVE_WITH_KNOTS ( 'NONE', 5,
 ( #32092, #101471, #93089, #83582, #110450, #50005 ),
 .UNSPECIFIED., .F., .F.,
 ( 6, 6 ),
 ( 0.000000000000000000, 1.000000000000000000 ),
 .UNSPECIFIED. ) ;
#99556=CARTESIAN_POINT ( 'NONE',  ( -3.094819227209999912, 1457.827881835389917, 218.9172905669589966 ) ) ;
#99560=CARTESIAN_POINT ( 'NONE',  ( -3.592139376770000059, 1475.286963719890082, 199.0484973181989972 ) ) ;
#99564=FACE_OUTER_BOUND ( 'NONE', #17528, .T. ) ;
#99566=CARTESIAN_POINT ( 'NONE',  ( -1.073240929390329958E-18, 1414.661898229710005, 209.1218459616989946 ) ) ;
#99569=CARTESIAN_POINT ( 'NONE',  ( 3.395043742270000386, 1466.412111213989874, 219.6384586637989855 ) ) ;
#99582=DIRECTION ( 'NONE',  ( -1.000000000000000000, 0.000000000000000000, 0.000000000000000000 ) ) ;
#99586=CARTESIAN_POINT ( 'NONE',  ( -14.65245208429999835, 1420.119839420520066, 213.8659312793989784 ) ) ;
#99598=CARTESIAN_POINT ( 'NONE',  ( 7.462159244181010287, 1425.241657824579988, 212.3244533792270090 ) ) ;
#99601=CARTESIAN_POINT ( 'NONE',  ( -7.500000000000000888, 1392.213060387289943, 209.1218459616989946 ) ) ;
#99613=CARTESIAN_POINT ( 'NONE',  ( 10.94062157769999999, 1501.627468090889806, 205.7261589474190373 ) ) ;
#99621=FACE_OUTER_BOUND ( 'NONE', #47406, .T. ) ;
#99626=CARTESIAN_POINT ( 'NONE',  ( -7.753833341240000898, 1425.741319864559955, 203.8098606200590268 ) ) ;
#99629=CARTESIAN_POINT ( 'NONE',  ( 11.52063869959389919, 1480.272724040029971, 211.6366542486999833 ) ) ;
#99630=CARTESIAN_POINT ( 'NONE',  ( 20.05746556670000302, 1473.529709444389937, 207.1912480031890027 ) ) ;
#99634=CARTESIAN_POINT ( 'NONE',  ( 2.413234528062761619, 1507.615208040094103, 220.6132374451732971 ) ) ;
#99636=CARTESIAN_POINT ( 'NONE',  ( -10.93170597650880005, 1470.132936137649949, 212.2373671120849963 ) ) ;
#99637=CARTESIAN_POINT ( 'NONE',  ( 9.464504535678571528, 1503.363322680939973, 217.6559705080630067 ) ) ;
#99639=CARTESIAN_POINT ( 'NONE',  ( -2.993158061556190130, 1476.307674819270005, 220.1965791242180046 ) ) ;
#99641=CARTESIAN_POINT ( 'NONE',  ( 10.02421119480000122, 1480.534221758890226, 205.8829018067289951 ) ) ;
#99646=CARTESIAN_POINT ( 'NONE',  ( 10.72411309857909778, 1423.704347997469995, 206.7356728586999850 ) ) ;
#99647=B_SPLINE_CURVE_WITH_KNOTS ( 'NONE', 3,
 ( #52073, #86762, #69998, #10051, #45341, #18982, #43664, #19548, #54295, #86206, #79481, #53179, #9498, #2788, #36908, #1125 ),
 .UNSPECIFIED., .F., .F.,
 ( 4, 3, 3, 3, 3, 4 ),
 ( -7.332849288699999413, -7.184230839218289866, -6.152654883699300470, -5.122512162619800691, -4.092878776982500355, -3.012888606410000669 ),
 .UNSPECIFIED. ) ;
#99656=CARTESIAN_POINT ( 'NONE',  ( 11.26956004432950031, 1427.671205884309984, 209.9218968568520154 ) ) ;
#99657=CARTESIAN_POINT ( 'NONE',  ( 12.00882698043040087, 1426.066405874380052, 202.8181785508519965 ) ) ;
#99659=CARTESIAN_POINT ( 'NONE',  ( 2.354338606519999821, 1430.802573520589931, 217.9074022094590077 ) ) ;
#99666=CARTESIAN_POINT ( 'NONE',  ( -16.82407893874610139, 1420.448463740390025, 203.3157013238160289 ) ) ;
#99667=CARTESIAN_POINT ( 'NONE',  ( -5.812333085687390266, 1457.439411062993941, 216.6809223546719068 ) ) ;
#99673=CARTESIAN_POINT ( 'NONE',  ( -7.571527303769999939, 1491.603552466590145, 211.0272147816089898 ) ) ;
#99674=CARTESIAN_POINT ( 'NONE',  ( 18.81609481059999922, 1456.479165729590022, 204.5196734937790097 ) ) ;
#99677=CARTESIAN_POINT ( 'NONE',  ( -0.7331377667929990238, 1515.470556211590065, 204.9034494321989825 ) ) ;
#99678=CARTESIAN_POINT ( 'NONE',  ( 12.71887460719259977, 1426.545466713459973, 203.1631513952430055 ) ) ;
#99694=CARTESIAN_POINT ( 'NONE',  ( -11.43172008590000033, 1490.909894833790077, 209.1362624142179811 ) ) ;
#99703=CARTESIAN_POINT ( 'NONE',  ( -12.06665071716309967, 1491.071228040269943, 206.9060804303800012 ) ) ;
#99711=CARTESIAN_POINT ( 'NONE',  ( 10.40693933779219904, 1471.062888143880173, 210.9539924980650198 ) ) ;
#99713=CARTESIAN_POINT ( 'NONE',  ( 17.77217598520769926, 1430.610759356409972, 213.2442890844889973 ) ) ;
#99719=CARTESIAN_POINT ( 'NONE',  ( -16.56403879315699967, 1464.818678847870160, 220.6315892174129942 ) ) ;
#99723=CARTESIAN_POINT ( 'NONE',  ( 20.21728935790000037, 1475.862786327189951, 209.1218459616989946 ) ) ;
#99741=CARTESIAN_POINT ( 'NONE',  ( -2.037005282023119701, 1486.400766935479851, 220.8722278604369933 ) ) ;
#99742=CARTESIAN_POINT ( 'NONE',  ( 11.43369621480000120, 1502.212434881789932, 208.0469179695890034 ) ) ;
#99746=( BOUNDED_CURVE ( )  B_SPLINE_CURVE ( 3, ( #68268, #41933, #76089, #25658 ),
 .UNSPECIFIED., .F., .T. ) 
 B_SPLINE_CURVE_WITH_KNOTS ( ( 4, 4 ),
 ( 4.149749351278939180, 5.275028794336680704 ),
 .UNSPECIFIED. ) 
 CURVE ( )  GEOMETRIC_REPRESENTATION_ITEM ( )  RATIONAL_B_SPLINE_CURVE ( ( 1.000000000000000000, 0.8972333180728662150, 0.8972333180728662150, 1.000000000000000000 ) ) 
 REPRESENTATION_ITEM ( '' )  );
#99749=CARTESIAN_POINT ( 'NONE',  ( 3.552713678799999608E-15, 1507.551704408389924, 209.1218459616989946 ) ) ;
#99754=CARTESIAN_POINT ( 'NONE',  ( -21.47380076839990082, 1487.892778387440103, 202.0847333328300124 ) ) ;
#99762=CARTESIAN_POINT ( 'NONE',  ( -21.11937805367519871, 1508.452816383899972, 209.9028812253390015 ) ) ;
#99766=CARTESIAN_POINT ( 'NONE',  ( -2.031883754679999932, 1464.998375783689880, 198.3053765207990011 ) ) ;
#99781=CARTESIAN_POINT ( 'NONE',  ( -10.92255993703960115, 1462.741395054350278, 207.3771677357329963 ) ) ;
#99785=B_SPLINE_CURVE_WITH_KNOTS ( 'NONE', 5,
 ( #2232, #36900, #28506, #62705, #2780, #47519, #29063, #36348, #63248 ),
 .UNSPECIFIED., .F., .F.,
 ( 6, 3, 6 ),
 ( 0.000000000000000000, 0.9874393323384224042, 1.000000000000000000 ),
 .UNSPECIFIED. ) ;
#99799=CARTESIAN_POINT ( 'NONE',  ( -2.022453434156979757, 1483.801003577689926, 198.6380168107399982 ) ) ;
#99805=CARTESIAN_POINT ( 'NONE',  ( -0.4895834631420010186, 1430.089577145089834, 214.7663758875890210 ) ) ;
#99806=CARTESIAN_POINT ( 'NONE',  ( -4.360112039636049985, 1441.644505157019921, 201.4346413363180091 ) ) ;
#99810=CARTESIAN_POINT ( 'NONE',  ( -8.588225070092541102, 1439.751992671629978, 226.1486124413150094 ) ) ;
#99812=CARTESIAN_POINT ( 'NONE',  ( -10.64685008816380041, 1482.274716053820157, 206.1670479490190360 ) ) ;
#99813=CARTESIAN_POINT ( 'NONE',  ( 19.26216268010000121, 1457.979299265790132, 211.9620131672190269 ) ) ;
#99826=CARTESIAN_POINT ( 'NONE',  ( -6.574341282982393508, 1439.975808622007889, 203.3270148206125612 ) ) ;
#99832=CARTESIAN_POINT ( 'NONE',  ( -10.94721987830000032, 1499.473939016889972, 212.6801052600889932 ) ) ;
#99839=CARTESIAN_POINT ( 'NONE',  ( 8.723134474349999223, 1451.781317889190177, 212.2855316608589931 ) ) ;
#99842=CARTESIAN_POINT ( 'NONE',  ( -10.61999372029469946, 1462.990852176999852, 206.0510140530389833 ) ) ;
#99848=CARTESIAN_POINT ( 'NONE',  ( -4.633397096295920115, 1377.913060387289988, 213.8868415672910146 ) ) ;
#99851=CARTESIAN_POINT ( 'NONE',  ( -6.872280032289999063, 1472.400811630890075, 210.0671059703809931 ) ) ;
#99853=CARTESIAN_POINT ( 'NONE',  ( -18.47518245109339929, 1466.235720590640085, 200.8822878488529966 ) ) ;
#99860=CARTESIAN_POINT ( 'NONE',  ( 7.586419159530000123, 1426.023150451340143, 212.1170382088889994 ) ) ;
#99863=CARTESIAN_POINT ( 'NONE',  ( -15.80819117724120026, 1420.947422077100100, 203.3790723405460028 ) ) ;
#99878=CARTESIAN_POINT ( 'NONE',  ( -4.669740627984789505, 1464.328320229509927, 199.6059302412689931 ) ) ;
#99879=CARTESIAN_POINT ( 'NONE',  ( -17.13142892129999950, 1417.632139391989995, 207.5091448026290095 ) ) ;
#99888=CARTESIAN_POINT ( 'NONE',  ( 0.000000000000000000, 1391.913060387289988, 209.1218459616989946 ) ) ;
#99890=ORIENTED_EDGE ( 'NONE', *, *, #16453, .F. ) ;
#99899=CARTESIAN_POINT ( 'NONE',  ( -12.50356189400000062, 1503.103369310989819, 208.6063100965829733 ) ) ;
#99924=CARTESIAN_POINT ( 'NONE',  ( -3.467940587273969921, 1495.562067866610050, 197.2905559816869925 ) ) ;
#99940=CARTESIAN_POINT ( 'NONE',  ( 12.54060419009999983, 1427.026833031130082, 206.2830509747190035 ) ) ;
#99941=CARTESIAN_POINT ( 'NONE',  ( -1.637258856660000150, 1483.893433971690001, 198.5669146070989939 ) ) ;
#99944=CARTESIAN_POINT ( 'NONE',  ( 8.884590929279953642, 1458.997830320633511, 202.8087306969714518 ) ) ;
#99946=ORIENTED_EDGE ( 'NONE', *, *, #35723, .T. ) ;
#99952=CARTESIAN_POINT ( 'NONE',  ( 10.92804747355420147, 1461.442164761259846, 210.0201248578009938 ) ) ;
#99954=CARTESIAN_POINT ( 'NONE',  ( -0.9256615464240010027, 1443.221293306289908, 218.6972998774490122 ) ) ;
#99960=CARTESIAN_POINT ( 'NONE',  ( -20.60448988230000111, 1484.737042837089803, 209.1218459616989946 ) ) ;
#99966=ORIENTED_EDGE ( 'NONE', *, *, #22687, .T. ) ;
#99975=CARTESIAN_POINT ( 'NONE',  ( -3.465081665767479890, 1515.493283046529996, 213.0346231893849733 ) ) ;
#99978=CARTESIAN_POINT ( 'NONE',  ( -14.98124668174299856, 1415.677402202029953, 207.3353217124920036 ) ) ;
#99979=CIRCLE ( 'NONE', #21310, 3.750000000000000000 ) ;
#99981=CARTESIAN_POINT ( 'NONE',  ( -12.17813008270000097, 1438.571549855089870, 224.0393728361989929 ) ) ;
#99991=CARTESIAN_POINT ( 'NONE',  ( 3.209129091579999926, 1455.228273979189908, 218.1432107165790057 ) ) ;
#99994=CARTESIAN_POINT ( 'NONE',  ( -3.026951662149999667, 1443.662240191790033, 218.7413276925990147 ) ) ;
#99996=ADVANCED_FACE ( 'NONE', ( #103115 ), #74379, .T. ) ;
#99997=CARTESIAN_POINT ( 'NONE',  ( 4.208240993269999564, 1434.939300248989866, 227.0651965576989824 ) ) ;
#99998=AXIS2_PLACEMENT_3D ( 'NONE', #33960, #93312, #35613 ) ;
#100004=CARTESIAN_POINT ( 'NONE',  ( -11.60387536552270049, 1481.105535834539978, 211.4044418330699955 ) ) ;
#100011=CARTESIAN_POINT ( 'NONE',  ( 13.91046082419999941, 1500.295402486089870, 227.7266705026989939 ) ) ;
#100013=CARTESIAN_POINT ( 'NONE',  ( 0.1263686949653684832, 1473.473085869263741, 219.3472977631268463 ) ) ;
#100018=B_SPLINE_CURVE_WITH_KNOTS ( 'NONE', 3,
 ( #17695, #84386, #85464, #103369, #75461, #101714, #50258, #59208, #94419, #83830, #86040, #101163, #93873, #43500, #24457, #58645, #102278, #60871, #16054, #77644, #7674, #93327 ),
 .UNSPECIFIED., .F., .F.,
 ( 4, 3, 3, 3, 3, 3, 3, 4 ),
 ( 0.000000000000000000, 1.239833439119680136, 2.490079122229909903, 3.560295889715780149, 4.472241803407629668, 5.624444489460710628, 6.402815887447280474, 7.120592051560000080 ),
 .UNSPECIFIED. ) ;
#100019=CARTESIAN_POINT ( 'NONE',  ( 9.967358615308720360, 1468.722972651999953, 208.0937358601780147 ) ) ;
#100020=CARTESIAN_POINT ( 'NONE',  ( -4.882000055239999803, 1457.939062349089909, 217.4853468547690056 ) ) ;
#100024=CARTESIAN_POINT ( 'NONE',  ( -4.329200639848730603, 1515.074268821609849, 210.6179437698939978 ) ) ;
#100027=VERTEX_POINT ( 'NONE', #84666 ) ;
#100045=CARTESIAN_POINT ( 'NONE',  ( 9.549000335789999738, 1470.075890097690035, 212.3436668229989834 ) ) ;
#100048=CARTESIAN_POINT ( 'NONE',  ( -6.918225190410000280, 1481.313522052990038, 206.5729027308990169 ) ) ;
#100057=CARTESIAN_POINT ( 'NONE',  ( -0.3900471094334390099, 1425.462776352800120, 191.1056874147849953 ) ) ;
#100062=EDGE_CURVE ( 'NONE', #103670, #63089, #35414, .T. ) ;
#100068=( BOUNDED_CURVE ( )  B_SPLINE_CURVE ( 3, ( #86729, #17837, #6842, #60445 ),
 .UNSPECIFIED., .F., .T. ) 
 B_SPLINE_CURVE_WITH_KNOTS ( ( 4, 4 ),
 ( 0.9240765055798439986, 2.217571029433250018 ),
 .UNSPECIFIED. ) 
 CURVE ( )  GEOMETRIC_REPRESENTATION_ITEM ( )  RATIONAL_B_SPLINE_CURVE ( ( 1.000000000000000000, 0.8653653976934794212, 0.8653653976934794212, 1.000000000000000000 ) ) 
 REPRESENTATION_ITEM ( '' )  );
#100072=CARTESIAN_POINT ( 'NONE',  ( -10.42886454120000117, 1471.797594669490081, 207.2580361199489687 ) ) ;
#100083=CARTESIAN_POINT ( 'NONE',  ( 7.174675627540000100, 1488.418531450889986, 199.9219973391489873 ) ) ;
#100092=CARTESIAN_POINT ( 'NONE',  ( -17.57477352489999944, 1417.955521924099912, 206.8173651875889902 ) ) ;
#100094=ADVANCED_FACE ( 'NONE', ( #92937 ), #41901, .F. ) ;
#100096=CARTESIAN_POINT ( 'NONE',  ( -16.68447695228019967, 1508.551704408389924, 212.9946650234450090 ) ) ;
#100098=CARTESIAN_POINT ( 'NONE',  ( -2.182683425780000075, 1475.185842043989851, 219.3315818484989848 ) ) ;
#100101=CARTESIAN_POINT ( 'NONE',  ( -3.751676929405963978, 1508.135276464469143, 220.7189868887600142 ) ) ;
#100106=CARTESIAN_POINT ( 'NONE',  ( -10.00567527226339948, 1472.275973908610013, 211.0029054612709842 ) ) ;
#100109=VERTEX_POINT ( 'NONE', #10602 ) ;
#100111=CARTESIAN_POINT ( 'NONE',  ( 4.253777714910000007, 1442.471859903390168, 216.9083338397390150 ) ) ;
#100115=CARTESIAN_POINT ( 'NONE',  ( 11.19147557906589974, 1422.145537183640045, 210.4506353095700035 ) ) ;
#100122=CARTESIAN_POINT ( 'NONE',  ( -12.73491014300939916, 1502.691142067039891, 209.0150589030249932 ) ) ;
#100123=CARTESIAN_POINT ( 'NONE',  ( 10.46256578778500135, 1491.122137232039904, 212.5076585947759895 ) ) ;
#100124=CARTESIAN_POINT ( 'NONE',  ( 0.7870490817069989431, 1454.950702146390086, 218.5222641204089769 ) ) ;
#100129=CARTESIAN_POINT ( 'NONE',  ( 2.564245648567370139, 1508.551704408389924, 204.1347675678190114 ) ) ;
#100130=ORIENTED_EDGE ( 'NONE', *, *, #2859, .T. ) ;
#100133=CARTESIAN_POINT ( 'NONE',  ( -2.329920892870120053, 1515.492270357739926, 204.9835198739350233 ) ) ;
#100134=CARTESIAN_POINT ( 'NONE',  ( -14.93718008229999938, 1416.181292664740113, 212.9156384192889959 ) ) ;
#100136=CARTESIAN_POINT ( 'NONE',  ( -3.541011004710050258, 1495.537215548379891, 197.3123223667620323 ) ) ;
#100139=CARTESIAN_POINT ( 'NONE',  ( 4.487574688360000508, 1465.989648107290122, 219.2141235446990208 ) ) ;
#100140=CARTESIAN_POINT ( 'NONE',  ( -12.19041342026659969, 1508.551704408389924, 217.1207088137099959 ) ) ;
#100144=CARTESIAN_POINT ( 'NONE',  ( 4.462819848452499905, 1432.645271588519790, 201.4082248412790079 ) ) ;
#100148=EDGE_LOOP ( 'NONE', ( #94510, #80834, #52075, #34946 ) ) ;
#100155=CARTESIAN_POINT ( 'NONE',  ( -15.68596832889999959, 1420.312328904400147, 210.6114427239490112 ) ) ;
#100167=B_SPLINE_SURFACE_WITH_KNOTS ( 'NONE', 5, 1, ( 
 ( #96783, #19499 ),
 ( #53701, #11664 ),
 ( #52577, #86712 ),
 ( #95668, #20054 ),
 ( #10004, #45840 ),
 ( #3291, #37423 ),
 ( #71620, #105740 ),
 ( #53132, #87269 ),
 ( #78312, #29024 ) ),
 .UNSPECIFIED., .F., .F., .F.,
 ( 6, 3, 6 ),
 ( 2, 2 ),
 ( 0.000000000000000000, 3.503639760140000003, 6.986073851990000527 ),
 ( 0.000000000000000000, 14.00000000000000000 ),
 .UNSPECIFIED. ) ;
#100168=CARTESIAN_POINT ( 'NONE',  ( 3.586377583332121866, 1515.071394844002270, 205.0391410476011913 ) ) ;
#100169=CARTESIAN_POINT ( 'NONE',  ( 7.495056103950230586, 1425.330532392250007, 212.2567483120330110 ) ) ;
#100178=CARTESIAN_POINT ( 'NONE',  ( -4.635184277964138566, 1377.964720639146435, 214.2196526210096579 ) ) ;
#100202=ORIENTED_EDGE ( 'NONE', *, *, #81477, .F. ) ;
#100203=CARTESIAN_POINT ( 'NONE',  ( 10.63195896838979948, 1481.229057553459825, 214.2444091096009799 ) ) ;
#100208=CARTESIAN_POINT ( 'NONE',  ( -10.50709737680259970, 1479.857933738049951, 209.4405100821019801 ) ) ;
#100209=B_SPLINE_CURVE_WITH_KNOTS ( 'NONE', 3,
 ( #89088, #12375, #14428, #48625, #53308, #79064, #87450, #31244, #19673, #29187, #10744, #2369, #71225, #53879, #82756, #4006 ),
 .UNSPECIFIED., .F., .F.,
 ( 4, 3, 3, 3, 3, 4 ),
 ( -7.611835606329999671, -7.348446743584259977, -6.291169182585940156, -5.234779306343579464, -4.178565810992130203, -3.122448789919999967 ),
 .UNSPECIFIED. ) ;
#100210=CARTESIAN_POINT ( 'NONE',  ( 5.989683923130864507, 1434.842958979083505, 203.0326939871309548 ) ) ;
#100211=B_SPLINE_SURFACE_WITH_KNOTS ( 'NONE', 5, 5, ( 
 ( #103635, #62213, #53254, #43734, #26932, #77886 ),
 ( #44858, #61121, #95784, #18500, #85170, #52696 ),
 ( #19051, #1752, #68407, #35890, #36423, #8456 ),
 ( #70073, #104736, #27469, #28025, #61658, #102511 ),
 ( #87394, #10689, #79010, #3954, #63317, #71734 ),
 ( #98529, #13403, #2850, #55997, #29130, #99068 ),
 ( #64954, #54362, #80084, #55452, #11776, #87956 ),
 ( #80640, #89027, #21796, #5022, #71166, #97437 ),
 ( #3402, #45945, #36974, #105851, #97971, #53819 ) ),
 .UNSPECIFIED., .F., .F., .F.,
 ( 6, 3, 6 ),
 ( 6, 6 ),
 ( 25.28925225189999892, 28.57063311849999820, 31.85201398510000104 ),
 ( 0.000000000000000000, 2.000000000000000000 ),
 .UNSPECIFIED. ) ;
#100215=CARTESIAN_POINT ( 'NONE',  ( 7.457597788700000230, 1422.876260087079800, 195.6364883457989947 ) ) ;
#100218=CARTESIAN_POINT ( 'NONE',  ( -10.14960351718960041, 1492.786034375650161, 202.1826628221230067 ) ) ;
#100219=CARTESIAN_POINT ( 'NONE',  ( 10.87765004282280046, 1478.880950294009835, 205.9430073526910121 ) ) ;
#100223=CARTESIAN_POINT ( 'NONE',  ( 11.36690311099069994, 1426.240274596359995, 206.5033745847870250 ) ) ;
#100225=EDGE_CURVE ( 'NONE', #100706, #11098, #64858, .T. ) ;
#100227=ORIENTED_EDGE ( 'NONE', *, *, #38524, .F. ) ;
#100233=CARTESIAN_POINT ( 'NONE',  ( 9.228811086073759995, 1424.916317554060015, 209.5472453667709942 ) ) ;
#100234=CARTESIAN_POINT ( 'NONE',  ( 11.22642611442629956, 1422.531523140060017, 203.3570491252529848 ) ) ;
#100243=CARTESIAN_POINT ( 'NONE',  ( -16.99050533527280038, 1420.323706995179919, 203.8408272025779979 ) ) ;
#100245=DIRECTION ( 'NONE',  ( 1.000000000000000000, 0.000000000000000000, 0.000000000000000000 ) ) ;
#100248=CARTESIAN_POINT ( 'NONE',  ( 3.096410888356740276, 1474.521509624629743, 220.1161525996240016 ) ) ;
#100251=CARTESIAN_POINT ( 'NONE',  ( -2.157956873969999911, 1474.488379276790056, 216.3412529684890160 ) ) ;
#100253=CARTESIAN_POINT ( 'NONE',  ( 1.842962231260000028, 1515.372048949689997, 204.8601094097890041 ) ) ;
#100254=CARTESIAN_POINT ( 'NONE',  ( 12.73074594762250022, 1426.578829893890088, 203.3886192763110330 ) ) ;
#100255=CARTESIAN_POINT ( 'NONE',  ( 14.43085700395960025, 1426.807556820840091, 195.4949582478319883 ) ) ;
#100261=CONICAL_SURFACE ( 'NONE', #91305, 6.911399307709998219, 0.04363323129990067523 ) ;
#100269=FACE_OUTER_BOUND ( 'NONE', #93459, .T. ) ;
#100271=CARTESIAN_POINT ( 'NONE',  ( -11.24222018449999894, 1491.652723530989988, 206.9322330278289712 ) ) ;
#100279=CARTESIAN_POINT ( 'NONE',  ( 11.05034677255730102, 1426.485892148770290, 207.3310236586839892 ) ) ;
#100284=ORIENTED_EDGE ( 'NONE', *, *, #27065, .F. ) ;
#100285=CARTESIAN_POINT ( 'NONE',  ( 4.551482758439999721, 1472.189735705889916, 218.2242021444390048 ) ) ;
#100287=CARTESIAN_POINT ( 'NONE',  ( 18.02736213689669853, 1430.307743537649912, 211.8462674276539985 ) ) ;
#100294=CARTESIAN_POINT ( 'NONE',  ( 7.590404545110000178, 1448.844191051889993, 202.5505402568389854 ) ) ;
#100297=CARTESIAN_POINT ( 'NONE',  ( -0.04684193791649880062, 1455.943453576789807, 198.9381708170990066 ) ) ;
#100300=ORIENTED_EDGE ( 'NONE', *, *, #17506, .T. ) ;
#100301=CARTESIAN_POINT ( 'NONE',  ( -1.861669630580974566, 1464.694416944532804, 199.0202437191204581 ) ) ;
#100302=CARTESIAN_POINT ( 'NONE',  ( 9.327651199099038948, 1434.415569083649871, 206.2244204008570136 ) ) ;
#100308=CARTESIAN_POINT ( 'NONE',  ( -3.218646267206591638, 1456.153438597946661, 200.2079057308925485 ) ) ;
#100317=ADVANCED_FACE ( 'NONE', ( #38542 ), #101782, .T. ) ;
#100322=CARTESIAN_POINT ( 'NONE',  ( 16.50821004073419829, 1494.476738410949793, 193.0249950623970108 ) ) ;
#100326=CARTESIAN_POINT ( 'NONE',  ( 0.1517714129250010147, 1432.859101342389977, 203.3442573752690237 ) ) ;
#100327=CARTESIAN_POINT ( 'NONE',  ( 10.43262181653840059, 1453.107031927230082, 211.0136350519360064 ) ) ;
#100332=CARTESIAN_POINT ( 'NONE',  ( -4.678976733710140223, 1508.551704408389924, 213.1801812299080154 ) ) ;
#100335=CARTESIAN_POINT ( 'NONE',  ( -19.84369564248747864, 1485.788751164898940, 214.8618253020684392 ) ) ;
#100349=CARTESIAN_POINT ( 'NONE',  ( -17.33260530524039211, 1508.455897782298734, 212.8473335983153731 ) ) ;
#100352=CARTESIAN_POINT ( 'NONE',  ( 10.03483494456899905, 1469.241669691499965, 207.4251379534379964 ) ) ;
#100353=CARTESIAN_POINT ( 'NONE',  ( -8.374556587419998976, 1473.433882946689891, 202.3872411742389943 ) ) ;
#100359=EDGE_CURVE ( 'NONE', #87290, #61133, #16800, .T. ) ;
#100361=ORIENTED_EDGE ( 'NONE', *, *, #18756, .F. ) ;
#100371=ORIENTED_EDGE ( 'NONE', *, *, #30388, .F. ) ;
#100373=CARTESIAN_POINT ( 'NONE',  ( 2.645105003909999919, 1508.551704408389924, 219.5149751571990180 ) ) ;
#100375=CARTESIAN_POINT ( 'NONE',  ( 0.06577164741639930645, 1429.775327166390070, 214.7293411062190103 ) ) ;
#100376=CARTESIAN_POINT ( 'NONE',  ( -5.051788235653639880, 1442.712519720660111, 200.9272651379969830 ) ) ;
#100379=CARTESIAN_POINT ( 'NONE',  ( -4.682239257119849896, 1438.893378829450057, 227.1256970199729892 ) ) ;
#100381=CARTESIAN_POINT ( 'NONE',  ( -13.54690246880000082, 1502.950168964990098, 209.0732237156209976 ) ) ;
#100383=ORIENTED_EDGE ( 'NONE', *, *, #61791, .F. ) ;
#100387=CARTESIAN_POINT ( 'NONE',  ( 10.81257864043729988, 1489.663435189140046, 207.4999579193730028 ) ) ;
#100393=CARTESIAN_POINT ( 'NONE',  ( -15.72388564909999964, 1416.853542096379897, 206.7724104149789923 ) ) ;
#100397=CARTESIAN_POINT ( 'NONE',  ( -11.25637333110000071, 1500.624827943590162, 211.0037259975690063 ) ) ;
#100415=AXIS2_PLACEMENT_3D ( 'NONE', #24869, #31087, #6992 ) ;
#100416=CARTESIAN_POINT ( 'NONE',  ( 5.145309177750649887, 1422.426130283250131, 194.5914460530619863 ) ) ;
#100417=CARTESIAN_POINT ( 'NONE',  ( 11.26929293258100095, 1478.652642090589779, 205.8599246912870058 ) ) ;
#100421=CARTESIAN_POINT ( 'NONE',  ( -8.627754864100788623, 1437.492696373060198, 228.3379673427390060 ) ) ;
#100425=FACE_OUTER_BOUND ( 'NONE', #98431, .T. ) ;
#100426=CARTESIAN_POINT ( 'NONE',  ( -8.405631201569999433, 1451.156562209089998, 203.4069089233589978 ) ) ;
#100431=CARTESIAN_POINT ( 'NONE',  ( -19.79017267473430053, 1418.757295473250224, 207.3023242580109979 ) ) ;
#100433=VECTOR ( 'NONE', #56306, 1000.000000000000227 ) ;
#100441=VERTEX_POINT ( 'NONE', #32361 ) ;
#100445=CARTESIAN_POINT ( 'NONE',  ( 0.6279484944370010702, 1443.757946321590225, 200.1921173854589995 ) ) ;
#100449=CARTESIAN_POINT ( 'NONE',  ( -17.44368141866249999, 1417.861416191989974, 207.0172452560950092 ) ) ;
#100457=ORIENTED_EDGE ( 'NONE', *, *, #4861, .T. ) ;
#100464=VERTEX_POINT ( 'NONE', #100645 ) ;
#100465=CARTESIAN_POINT ( 'NONE',  ( -11.46285876299999984, 1503.757027581689954, 207.6153421870490092 ) ) ;
#100468=EDGE_CURVE ( 'NONE', #98544, #105125, #51550, .T. ) ;
#100474=EDGE_CURVE ( 'NONE', #36031, #65500, #14035, .T. ) ;
#100478=ORIENTED_EDGE ( 'NONE', *, *, #24780, .T. ) ;
#100487=CARTESIAN_POINT ( 'NONE',  ( -5.100957845159999948, 1482.122785942490054, 228.9672709512990139 ) ) ;
#100488=CARTESIAN_POINT ( 'NONE',  ( 17.59477483717979851, 1428.744049018530177, 204.6105714838779761 ) ) ;
#100492=CARTESIAN_POINT ( 'NONE',  ( -5.311724842150000292, 1500.891271500089942, 229.7588813323989996 ) ) ;
#100501=CARTESIAN_POINT ( 'NONE',  ( -0.1651761191785623695, 1494.443534717202510, 220.2719660499762995 ) ) ;
#100502=CARTESIAN_POINT ( 'NONE',  ( 4.955161316548390538, 1484.956798682839917, 218.7828042351830220 ) ) ;
#100504=CARTESIAN_POINT ( 'NONE',  ( -2.072561274125446218, 1497.860486493681265, 198.0224543596587807 ) ) ;
#100507=CARTESIAN_POINT ( 'NONE',  ( 5.291552342926635788, 1457.527819839196582, 199.7187649193072332 ) ) ;
#100512=CONICAL_SURFACE ( 'NONE', #97016, 6.911399307709998219, 0.04363323129990067523 ) ;
#100515=CARTESIAN_POINT ( 'NONE',  ( 10.91194618042609932, 1461.517685402190182, 210.2175723062259749 ) ) ;
#100516=CARTESIAN_POINT ( 'NONE',  ( -5.516138227071085254, 1462.433753707725145, 201.0655331976316802 ) ) ;
#100517=CARTESIAN_POINT ( 'NONE',  ( -1.259107554299999876, 1443.335980107890009, 218.6644318344589806 ) ) ;
#100521=CARTESIAN_POINT ( 'NONE',  ( 8.784378609766859469, 1487.811415144687999, 202.7137191972914536 ) ) ;
#100530=CARTESIAN_POINT ( 'NONE',  ( -4.871322248929999432, 1483.548475176390184, 199.6254626716689984 ) ) ;
#100533=CARTESIAN_POINT ( 'NONE',  ( -8.590080337109450070, 1437.218647809359709, 210.0977144842290159 ) ) ;
#100534=CARTESIAN_POINT ( 'NONE',  ( 3.076459279043819883, 1495.499563246870139, 221.1031227505570200 ) ) ;
#100537=CARTESIAN_POINT ( 'NONE',  ( -9.615660731045778675, 1460.249980679099963, 209.9216382747220280 ) ) ;
#100541=B_SPLINE_CURVE_WITH_KNOTS ( 'NONE', 5,
 ( #30162, #98475, #5530, #38032, #64353, #108536 ),
 .UNSPECIFIED., .F., .F.,
 ( 6, 6 ),
 ( -2.000000000000000000, -4.054528290886594277E-08 ),
 .UNSPECIFIED. ) ;
#100548=CARTESIAN_POINT ( 'NONE',  ( 3.380344682699999659, 1455.610420236290111, 218.3745015725090184 ) ) ;
#100550=CARTESIAN_POINT ( 'NONE',  ( -7.825150488850000308, 1446.296144498489866, 214.7080216625790001 ) ) ;
#100559=CARTESIAN_POINT ( 'NONE',  ( -7.243611849145669801, 1479.647692371829862, 210.0496540924740145 ) ) ;
#100560=CARTESIAN_POINT ( 'NONE',  ( 4.989246313819999834, 1471.909539260290103, 189.7082128665990126 ) ) ;
#100564=CARTESIAN_POINT ( 'NONE',  ( 24.13933143269999704, 1497.424724656589888, 206.6888131984590018 ) ) ;
#100572=CARTESIAN_POINT ( 'NONE',  ( -3.703897191089999819, 1458.190786016390120, 219.1639864912989992 ) ) ;
#100581=CARTESIAN_POINT ( 'NONE',  ( 5.161277877375379575, 1424.205378946189967, 193.2953230041809718 ) ) ;
#100583=CARTESIAN_POINT ( 'NONE',  ( -17.64670096713561165, 1419.583565028061230, 207.1176534675684877 ) ) ;
#100585=VECTOR ( 'NONE', #58118, 1000.000000000000114 ) ;
#100586=CARTESIAN_POINT ( 'NONE',  ( -10.12195197648249945, 1470.644448988779914, 212.0626821655110348 ) ) ;
#100607=CARTESIAN_POINT ( 'NONE',  ( 8.530448452174001162, 1437.926137415760195, 210.8253904255420252 ) ) ;
#100611=CARTESIAN_POINT ( 'NONE',  ( -10.55526070360000013, 1471.506691870590203, 208.2730915841879948 ) ) ;
#100620=CARTESIAN_POINT ( 'NONE',  ( 7.346915560640000287, 1487.962896346489970, 200.9143651426790029 ) ) ;
#100621=CARTESIAN_POINT ( 'NONE',  ( -4.623067421070000016, 1470.601194648889987, 189.6761541078989808 ) ) ;
#100630=CARTESIAN_POINT ( 'NONE',  ( -18.05232962988900169, 1508.551704408389924, 211.0109356106890175 ) ) ;
#100631=CARTESIAN_POINT ( 'NONE',  ( 0.01429292403579860045, 1475.129915452889918, 220.1645601639990275 ) ) ;
#100633=CARTESIAN_POINT ( 'NONE',  ( -11.30252681748399901, 1471.157032186200013, 207.5285798585680084 ) ) ;
#100634=CARTESIAN_POINT ( 'NONE',  ( -4.717896399877197666, 1508.208081382373848, 220.4986227734547128 ) ) ;
#100636=CARTESIAN_POINT ( 'NONE',  ( -2.812687921020009973, 1454.522389872590111, 199.0175643825760119 ) ) ;
#100637=CARTESIAN_POINT ( 'NONE',  ( -4.326079385514251641, 1515.193466644350337, 210.9648093357023697 ) ) ;
#100639=B_SPLINE_CURVE_WITH_KNOTS ( 'NONE', 3,
 ( #42183, #26466, #52257, #745, #59544, #16938, #33761, #51140, #77444, #85266, #76895, #102604, #9130, #94220, #25351, #204, #67405, #8563, #18063, #51692, #109938, #50042, #93656, #86383, #34876, #58437, #60103, #92565, #84169, #103165, #17494, #42735, #34327, #25905, #85833, #43296, #60661, #9669, #43841, #7469, #77987, #93123, #35433, #24257, #41631, #75785 ),
 .UNSPECIFIED., .F., .F.,
 ( 4, 3, 3, 3, 3, 3, 3, 3, 3, 3, 3, 3, 3, 3, 3, 4 ),
 ( -33.33692105922289528, -32.30496137087640562, -30.87533264016670032, -29.45119221417040123, -28.03232753619460027, -26.62582012346450000, -25.22895400231270102, -23.84265630345680265, -23.19230641462139886, -21.81245709143689737, -20.43032364105260257, -19.04908065426700148, -17.67389872415650132, -16.30563378985170075, -14.94618987489860018, -13.59708442930000061 ),
 .UNSPECIFIED. ) ;
#100640=CARTESIAN_POINT ( 'NONE',  ( -10.24327470438359988, 1471.488599568509926, 210.1179836163729817 ) ) ;
#100642=DIRECTION ( 'NONE',  ( 0.9127217750004207319, -0.3840007055116108625, -0.1395794383376949832 ) ) ;
#100645=CARTESIAN_POINT ( 'NONE',  ( 11.41287573240554032, 1427.618782186570115, 209.6357587079445182 ) ) ;
#100647=CARTESIAN_POINT ( 'NONE',  ( -3.395799912579999802, 1442.082743038290118, 200.9143888862090250 ) ) ;
#100649=CARTESIAN_POINT ( 'NONE',  ( 2178.386296064867111, -8387.357407334289746, -1553.770216230970163 ) ) ;
#100651=CARTESIAN_POINT ( 'NONE',  ( -2.140641997699999965, 1508.551704408389924, 220.0635241299990241 ) ) ;
#100659=CARTESIAN_POINT ( 'NONE',  ( 11.32936712494479892, 1492.131809937580101, 211.0328881183560270 ) ) ;
#100661=CARTESIAN_POINT ( 'NONE',  ( -2.019856026379999836, 1456.316848387589971, 218.3948360566789972 ) ) ;
#100665=EDGE_CURVE ( 'NONE', #73174, #3165, #23121, .T. ) ;
#100667=ORIENTED_EDGE ( 'NONE', *, *, #53238, .T. ) ;
#100668=ORIENTED_EDGE ( 'NONE', *, *, #60562, .F. ) ;
#100670=CARTESIAN_POINT ( 'NONE',  ( -8.169799973510000868, 1501.392344667289990, 208.3166649180830063 ) ) ;
#100671=CARTESIAN_POINT ( 'NONE',  ( -4.077242828485170278, 1515.224507406410112, 205.5390080823180199 ) ) ;
#100674=CARTESIAN_POINT ( 'NONE',  ( 11.64374231457060027, 1480.041980269009855, 210.9631198931459721 ) ) ;
#100678=CARTESIAN_POINT ( 'NONE',  ( -8.804153820836120303, 1508.551704408389924, 218.7132714456290046 ) ) ;
#100681=CARTESIAN_POINT ( 'NONE',  ( 18.79226589730000185, 1456.307606824690083, 213.7887498653890077 ) ) ;
#100682=CARTESIAN_POINT ( 'NONE',  ( 1.372916587609890104, 1432.414705139630087, 200.7998117957879742 ) ) ;
#100699=CARTESIAN_POINT ( 'NONE',  ( -8.259628006849998982, 1424.858822388950102, 205.8688264180890144 ) ) ;
#100700=EDGE_CURVE ( 'NONE', #54152, #2493, #10132, .T. ) ;
#100704=CARTESIAN_POINT ( 'NONE',  ( 6.937981266933950231, 1424.879596851670158, 213.3109209129980002 ) ) ;
#100705=EDGE_CURVE ( 'NONE', #57731, #35548, #28748, .T. ) ;
#100706=VERTEX_POINT ( 'NONE', #43801 ) ;
#100713=CARTESIAN_POINT ( 'NONE',  ( -1.748905560439999896, 1488.269106391890091, 219.8524659834990018 ) ) ;
#100718=CARTESIAN_POINT ( 'NONE',  ( 10.47517306970000028, 1461.766207292889931, 210.2934874650690062 ) ) ;
#100735=CARTESIAN_POINT ( 'NONE',  ( -1.034405465910470001, 1444.468934022600024, 199.1208377739500008 ) ) ;
#100736=CARTESIAN_POINT ( 'NONE',  ( 0.06577166592579929139, 1429.775327338489888, 214.7293410279390002 ) ) ;
#100737=ORIENTED_EDGE ( 'NONE', *, *, #54943, .T. ) ;
#100738=CARTESIAN_POINT ( 'NONE',  ( 4.491284101707059939, 1508.884228866460035, 206.6339218519869974 ) ) ;
#100741=CARTESIAN_POINT ( 'NONE',  ( 7.703548237945829769, 1504.124514085119927, 219.2853995089439820 ) ) ;
#100742=CARTESIAN_POINT ( 'NONE',  ( 7.767274028600000157, 1421.765204529709990, 195.8385879648990056 ) ) ;
#100743=CARTESIAN_POINT ( 'NONE',  ( -0.05601447201598130227, 1431.857486804389964, 218.6169334100210051 ) ) ;
#100744=CARTESIAN_POINT ( 'NONE',  ( -4.922543830899999584, 1496.353864017489968, 199.0299218828990035 ) ) ;
#100748=CARTESIAN_POINT ( 'NONE',  ( 11.13262782095319814, 1425.908268888629891, 206.4954163449100122 ) ) ;
#100757=CARTESIAN_POINT ( 'NONE',  ( 20.22418986319999590, 1476.021096013189890, 210.1149224964580071 ) ) ;
#100758=CARTESIAN_POINT ( 'NONE',  ( 11.72053595058989828, 1425.791693304140153, 202.8787723380090142 ) ) ;
#100759=CARTESIAN_POINT ( 'NONE',  ( 0.8465175048109989664, 1430.128326741589945, 217.4134717798089866 ) ) ;
#100762=B_SPLINE_CURVE_WITH_KNOTS ( 'NONE', 3,
 ( #61424, #26114, #87721, #8767 ),
 .UNSPECIFIED., .F., .F.,
 ( 4, 4 ),
 ( 0.9643540914522175100, 1.000000000000000000 ),
 .UNSPECIFIED. ) ;
#100776=CARTESIAN_POINT ( 'NONE',  ( -0.3672702989670010298, 1473.612351522490144, 216.6187257883390203 ) ) ;
#100781=CARTESIAN_POINT ( 'NONE',  ( 14.17511961927979947, 1428.761297916650165, 195.0897163562519836 ) ) ;
#100795=CARTESIAN_POINT ( 'NONE',  ( -1.436398804920000050, 1485.575541285890040, 197.7087229570989848 ) ) ;
#100800=CARTESIAN_POINT ( 'NONE',  ( -3.430356047799270058, 1431.707894944020154, 216.7924308075639885 ) ) ;
#100804=CARTESIAN_POINT ( 'NONE',  ( 3.984081755090749688, 1515.551704407335137, 210.9648081771169643 ) ) ;
#100808=CARTESIAN_POINT ( 'NONE',  ( 11.26800005207859812, 1422.300764229830065, 207.0940410118970192 ) ) ;
#100812=CARTESIAN_POINT ( 'NONE',  ( 1.100421420896519953, 1437.654385139740043, 227.6420619421519973 ) ) ;
#100813=ORIENTED_EDGE ( 'NONE', *, *, #27283, .F. ) ;
#100814=CARTESIAN_POINT ( 'NONE',  ( 3.171904416549999883, 1474.503316444290022, 220.1039004212989880 ) ) ;
#100815=CARTESIAN_POINT ( 'NONE',  ( 10.94247266901300186, 1470.964281316320239, 209.6238199810090066 ) ) ;
#100823=CARTESIAN_POINT ( 'NONE',  ( 8.746374439269999357, 1448.961682185689824, 206.1466908165390066 ) ) ;
#100826=FACE_OUTER_BOUND ( 'NONE', #11615, .T. ) ;
#100835=CARTESIAN_POINT ( 'NONE',  ( -17.53940096235950108, 1417.889611524100246, 206.8563643866829977 ) ) ;
#100836=ORIENTED_EDGE ( 'NONE', *, *, #74895, .T. ) ;
#100838=CARTESIAN_POINT ( 'NONE',  ( 11.09014987159999954, 1501.265658831390056, 206.2946274632390100 ) ) ;
#100846=CARTESIAN_POINT ( 'NONE',  ( 4.987078393879730065, 1508.551704408389924, 211.6860916102569661 ) ) ;
#100848=B_SPLINE_CURVE_WITH_KNOTS ( 'NONE', 3,
 ( #22734, #64805, #83226, #40669, #32809, #22186, #66994, #56384, #100013, #23303, #82115, #5969, #5414, #49638, #65348, #14349, #101104, #58588, #66453, #40114, #57498, #91623, #14899, #23847 ),
 .UNSPECIFIED., .F., .F.,
 ( 4, 2, 1, 1, 2, 2, 2, 2, 2, 1, 1, 2, 2, 4 ),
 ( 0.000000000000000000, 0.1249999999997721822, 0.1874999999996589395, 0.2187499999995849431, 0.2343749999995655697, 0.2499999999995461963, 0.3749999999995765609, 0.4999999999996068700, 0.6249999999996371791, 0.6874999999996733724, 0.7187499999997116751, 0.7343749999997076783, 0.7499999999997037925, 1.000000000000000000 ),
 .UNSPECIFIED. ) ;
#100851=CARTESIAN_POINT ( 'NONE',  ( -17.84104287039070158, 1489.004150074129939, 195.1797407690729926 ) ) ;
#100854=ORIENTED_EDGE ( 'NONE', *, *, #20778, .F. ) ;
#100857=CARTESIAN_POINT ( 'NONE',  ( -6.752164255999639764, 1508.178364352339941, 220.1479925240329862 ) ) ;
#100858=CARTESIAN_POINT ( 'NONE',  ( -18.43222347473149725, 1508.250680623890048, 209.6150243477850097 ) ) ;
#100859=CARTESIAN_POINT ( 'NONE',  ( 4.325405441710000076, 1515.219201591190085, 210.9648081929590262 ) ) ;
#100873=ORIENTED_EDGE ( 'NONE', *, *, #85906, .F. ) ;
#100875=CARTESIAN_POINT ( 'NONE',  ( 7.370119641675869637, 1429.027654456439905, 215.0938587317789938 ) ) ;
#100877=CARTESIAN_POINT ( 'NONE',  ( -9.416464707496981390, 1461.065390459309810, 206.8423381932979908 ) ) ;
#100879=CARTESIAN_POINT ( 'NONE',  ( 10.32832267219609967, 1469.723099828480144, 207.2225980447589961 ) ) ;
#100880=CARTESIAN_POINT ( 'NONE',  ( -10.07154918490000028, 1473.228065907190057, 207.4129428866989997 ) ) ;
#100881=CARTESIAN_POINT ( 'NONE',  ( 7.793403662019999345, 1494.414358568890066, 218.7662867540790046 ) ) ;
#100893=CARTESIAN_POINT ( 'NONE',  ( 4.329415264797519924, 1515.068899375750107, 212.0799422158490017 ) ) ;
#100894=CARTESIAN_POINT ( 'NONE',  ( 3.829620113550000315, 1515.551704408389924, 206.7917118356089929 ) ) ;
#100895=CARTESIAN_POINT ( 'NONE',  ( -12.44369114979409829, 1501.867506418240055, 211.6083604211140141 ) ) ;
#100897=CARTESIAN_POINT ( 'NONE',  ( -15.57383198649972478, 1415.691259407821008, 209.6195876535002185 ) ) ;
#100902=CARTESIAN_POINT ( 'NONE',  ( -6.402186394137180159, 1442.114340014330082, 201.8762545916499960 ) ) ;
#100904=CARTESIAN_POINT ( 'NONE',  ( -7.738175793921410417, 1425.683019801390174, 203.9398901317029811 ) ) ;
#100905=CARTESIAN_POINT ( 'NONE',  ( 5.524836877539999414, 1479.546334898089981, 203.7511963579289898 ) ) ;
#100907=CARTESIAN_POINT ( 'NONE',  ( -10.32767976395509990, 1481.876697752989912, 206.1677484232849906 ) ) ;
#100916=CARTESIAN_POINT ( 'NONE',  ( 3.597520269628190270, 1454.162627168660038, 217.7902427506969900 ) ) ;
#100919=CARTESIAN_POINT ( 'NONE',  ( -15.31079571090000080, 1415.244376457269937, 207.2352505607890123 ) ) ;
#100921=EDGE_CURVE ( 'NONE', #32575, #10141, #48784, .T. ) ;
#100923=CARTESIAN_POINT ( 'NONE',  ( -16.20543174878743287, 1419.737581145931244, 209.9462470130569329 ) ) ;
#100924=CARTESIAN_POINT ( 'NONE',  ( -9.202596930160000355, 1498.966442822989848, 216.3590987745790244 ) ) ;
#100926=CARTESIAN_POINT ( 'NONE',  ( 4.046562303720000031, 1471.775282961290031, 189.4720092632990145 ) ) ;
#100929=CARTESIAN_POINT ( 'NONE',  ( 10.54606093473799966, 1481.256042122329973, 208.4465981898469806 ) ) ;
#100930=EDGE_CURVE ( 'NONE', #35462, #103755, #43424, .T. ) ;
#100936=AXIS2_PLACEMENT_3D ( 'NONE', #54278, #80559, #10037 ) ;
#100945=CARTESIAN_POINT ( 'NONE',  ( 4.324092179320000007, 1515.269353058490196, 208.7600910743320242 ) ) ;
#100947=CARTESIAN_POINT ( 'NONE',  ( 3.350944662710000355, 1464.628126271390101, 199.8699733667390035 ) ) ;
#100950=CARTESIAN_POINT ( 'NONE',  ( 10.60846801522230010, 1479.281623091750134, 206.5255074603050218 ) ) ;
#100954=CARTESIAN_POINT ( 'NONE',  ( -9.582919297036148976, 1448.092179236340144, 190.7786095242630040 ) ) ;
#100955=CARTESIAN_POINT ( 'NONE',  ( -13.59348226018689942, 1508.032052514259931, 209.4636025531580117 ) ) ;
#100956=CARTESIAN_POINT ( 'NONE',  ( -2.515613294096589847, 1448.349718810959985, 188.5842421507169888 ) ) ;
#100967=CARTESIAN_POINT ( 'NONE',  ( -17.11220264658090073, 1420.169995509359978, 204.6828454769579935 ) ) ;
#100976=ORIENTED_EDGE ( 'NONE', *, *, #100921, .F. ) ;
#100978=CIRCLE ( 'NONE', #2713, 15.40132948099999943 ) ;
#100980=CARTESIAN_POINT ( 'NONE',  ( 4.261662193653270592, 1515.372228416479857, 206.7919396051269985 ) ) ;
#100981=CARTESIAN_POINT ( 'NONE',  ( 2.544801979510000312, 1445.822494309589956, 199.7339677725889828 ) ) ;
#100985=CARTESIAN_POINT ( 'NONE',  ( -3.858501607638550102, 1463.264545322189861, 200.1250934300819893 ) ) ;
#100992=EDGE_LOOP ( 'NONE', ( #95922, #51748, #67971, #55943, #110392, #21120, #14841, #7888, #43850, #95004, #6017, #45488, #82709, #89562, #28333, #84452, #59126, #48335, #55654, #4227, #80496, #57103, #96915, #54297, #10003, #28996 ) ) ;
#100994=ORIENTED_EDGE ( 'NONE', *, *, #5122, .F. ) ;
#101002=CARTESIAN_POINT ( 'NONE',  ( -12.66333039259999893, 1503.375086606289869, 208.6466812236969872 ) ) ;
#101009=CARTESIAN_POINT ( 'NONE',  ( -8.754256066850169660, 1451.698950522699988, 206.0561735730059922 ) ) ;
#101015=CARTESIAN_POINT ( 'NONE',  ( -14.77864689549059918, 1508.551704408389924, 210.3595489859820020 ) ) ;
#101024=CARTESIAN_POINT ( 'NONE',  ( 12.29645462760879937, 1492.351698860680017, 210.2246036700939840 ) ) ;
#101033=B_SPLINE_SURFACE_WITH_KNOTS ( 'NONE', 5, 5, ( 
 ( #73397, #63910, #56042, #98024, #56595, #99117 ),
 ( #55503, #5072, #30824, #11834, #96952, #89630 ),
 ( #47097, #108079, #4539, #64999, #73948, #64462 ),
 ( #22395, #38129, #20218, #38673, #72848, #14012 ),
 ( #30270, #54417, #98579, #5639, #80136, #37583 ),
 ( #4003, #71786, #105905, #63375, #97491, #20759 ),
 ( #89084, #12371, #46557, #94438, #78208, #35101 ),
 ( #51351, #69283, #76551, #57165, #82883, #103388 ),
 ( #50807, #16610, #68190, #26694, #102837, #110706 ) ),
 .UNSPECIFIED., .F., .F., .F.,
 ( 6, 3, 6 ),
 ( 6, 6 ),
 ( 13.54778530316779950, 23.82275646639999778, 33.29595707573220409 ),
 ( -1.147433219344110065E-05, 2.000000000000000000 ),
 .UNSPECIFIED. ) ;
#101036=CARTESIAN_POINT ( 'NONE',  ( 1.253776719794245986, 1494.066817944285049, 220.1788260179384054 ) ) ;
#101052=FACE_OUTER_BOUND ( 'NONE', #34366, .T. ) ;
#101061=CARTESIAN_POINT ( 'NONE',  ( 4.190103204352849886, 1507.220947887740067, 220.0490538541789931 ) ) ;
#101065=CARTESIAN_POINT ( 'NONE',  ( -8.355888189921600429, 1440.379141069660136, 205.2277604852559705 ) ) ;
#101070=B_SPLINE_SURFACE_WITH_KNOTS ( 'NONE', 5, 5, ( 
 ( #66231, #74615, #40439, #40989, #108195, #48873 ),
 ( #109318, #6829, #49411, #108750, #32601, #32042 ),
 ( #23638, #56705, #22504, #75168, #81886, #90841 ),
 ( #100877, #23073, #64577, #24170, #58359, #92484 ),
 ( #90285, #82999, #65664, #15754, #49955, #99781 ),
 ( #98696, #13566, #21955, #5189, #14126, #48316 ),
 ( #82457, #76252, #94699, #8477, #110400, #25270 ),
 ( #121, #95260, #93040, #42651, #35349, #1214 ),
 ( #60579, #68428, #16314, #76805, #50515, #77908 ) ),
 .UNSPECIFIED., .F., .F., .F.,
 ( 6, 3, 6 ),
 ( 6, 6 ),
 ( 3.019990725210560001, 5.187276425779999478, 7.354562126349439843 ),
 ( -0.0004187671794352290015, 2.000000000000000000 ),
 .UNSPECIFIED. ) ;
#101071=CARTESIAN_POINT ( 'NONE',  ( -3.644351594698530317, 1515.551704204689941, 212.3939699354600066 ) ) ;
#101084=CARTESIAN_POINT ( 'NONE',  ( -12.33321116790000005, 1502.561054230289983, 208.9929969191140060 ) ) ;
#101088=CARTESIAN_POINT ( 'NONE',  ( -6.429626910120000538, 1446.645710171090059, 215.7201002026189940 ) ) ;
#101091=CARTESIAN_POINT ( 'NONE',  ( 9.363526459378379130, 1464.473567072740025, 212.1249062944089872 ) ) ;
#101100=VERTEX_POINT ( 'NONE', #8389 ) ;
#101102=CARTESIAN_POINT ( 'NONE',  ( 24.04366839390669952, 1494.655600297209958, 207.1743948306419725 ) ) ;
#101104=CARTESIAN_POINT ( 'NONE',  ( -2.080714710711137450, 1474.229611947080684, 219.1688284120783692 ) ) ;
#101106=ADVANCED_FACE ( 'NONE', ( #94604 ), #8621, .T. ) ;
#101111=CARTESIAN_POINT ( 'NONE',  ( 10.01496071350510064, 1468.907470368469831, 208.6044946494789940 ) ) ;
#101114=CARTESIAN_POINT ( 'NONE',  ( -9.471334638087320457, 1448.015926047950188, 210.3227975281659781 ) ) ;
#101118=CARTESIAN_POINT ( 'NONE',  ( -4.329448791022380227, 1515.064792310580060, 210.8975365261770207 ) ) ;
#101122=CARTESIAN_POINT ( 'NONE',  ( 9.117609068447830367, 1425.283679751730006, 195.1398618588590068 ) ) ;
#101126=B_SPLINE_CURVE_WITH_KNOTS ( 'NONE', 5,
 ( #43764, #51068, #17983, #52179, #77371, #7943, #8485, #86310, #94707, #26392, #76259, #33688 ),
 .UNSPECIFIED., .F., .F.,
 ( 6, 3, 3, 6 ),
 ( -25.27124713539999945, -25.02147540209999832, -24.77170366879999719, -21.89878894926970077 ),
 .UNSPECIFIED. ) ;
#101130=CIRCLE ( 'NONE', #88700, 6.646318662569999702 ) ;
#101147=CARTESIAN_POINT ( 'NONE',  ( 9.722207004026980570, 1428.114070666289763, 212.2005352792010058 ) ) ;
#101148=FACE_OUTER_BOUND ( 'NONE', #62820, .T. ) ;
#101149=CARTESIAN_POINT ( 'NONE',  ( 5.994585642347090904, 1439.856461454209921, 216.6194481787469783 ) ) ;
#101152=ORIENTED_EDGE ( 'NONE', *, *, #16459, .T. ) ;
#101154=CARTESIAN_POINT ( 'NONE',  ( -9.534250030377648955, 1439.230267954009832, 208.6524524575060013 ) ) ;
#101160=CARTESIAN_POINT ( 'NONE',  ( -4.317409491140000277, 1412.932174402340024, 207.9150182743289861 ) ) ;
#101162=CARTESIAN_POINT ( 'NONE',  ( 4.851218532629999913, 1487.503864385689894, 198.5929753848990060 ) ) ;
#101163=CARTESIAN_POINT ( 'NONE',  ( 2.924955189797899813, 1430.826773540479962, 218.1505144264980061 ) ) ;
#101171=CARTESIAN_POINT ( 'NONE',  ( -16.68788013329999842, 1420.510568510920166, 203.3707636713990041 ) ) ;
#101175=CARTESIAN_POINT ( 'NONE',  ( 0.05161184595879859949, 1475.303443633190000, 220.5712324161989955 ) ) ;
#101177=CARTESIAN_POINT ( 'NONE',  ( -21.50400446119279962, 1505.467562055609960, 209.6175409707290100 ) ) ;
#101178=CARTESIAN_POINT ( 'NONE',  ( -11.23655883251920073, 1471.270429263729966, 207.1105222724550003 ) ) ;
#101179=CARTESIAN_POINT ( 'NONE',  ( -5.195342543991931628, 1508.245210224850780, 220.3666772047745610 ) ) ;
#101184=CARTESIAN_POINT ( 'NONE',  ( -14.24607374332530085, 1416.872377924300054, 203.2551249638830200 ) ) ;
#101189=CARTESIAN_POINT ( 'NONE',  ( -9.930122423809999432, 1499.782504084789934, 217.2571562510489969 ) ) ;
#101192=CARTESIAN_POINT ( 'NONE',  ( 11.45283955604839932, 1502.343333994649811, 211.2592759328639715 ) ) ;
#101193=CARTESIAN_POINT ( 'NONE',  ( -10.07154918488590134, 1473.228065907060000, 207.4129428866500007 ) ) ;
#101195=CARTESIAN_POINT ( 'NONE',  ( -3.608621357268490204, 1488.296475687800012, 219.4393136407599911 ) ) ;
#101197=CARTESIAN_POINT ( 'NONE',  ( -4.123250153539999907, 1515.545045452190152, 208.3730692491820093 ) ) ;
#101200=CARTESIAN_POINT ( 'NONE',  ( 11.39903530061180170, 1471.112746094619979, 209.6182361319149834 ) ) ;
#101201=CARTESIAN_POINT ( 'NONE',  ( 12.30197900188439952, 1492.344385971049860, 210.1930000934870009 ) ) ;
#101202=CARTESIAN_POINT ( 'NONE',  ( -1.929956593220000016, 1456.736549107989958, 218.5607043152189704 ) ) ;
#101213=CARTESIAN_POINT ( 'NONE',  ( -9.160644070140000039, 1462.341874057690120, 205.2627832839989992 ) ) ;
#101216=CARTESIAN_POINT ( 'NONE',  ( -7.939942809495481590, 1508.551704408389924, 218.9616636473319886 ) ) ;
#101219=CARTESIAN_POINT ( 'NONE',  ( 3.396568279634440302, 1487.113085923700055, 197.6558524979510025 ) ) ;
#101228=CARTESIAN_POINT ( 'NONE',  ( -12.99430343120000053, 1503.123593417290067, 208.6821788852620045 ) ) ;
#101229=CARTESIAN_POINT ( 'NONE',  ( -2.021349652797419960, 1420.993378913349943, 193.8016399264820109 ) ) ;
#101230=CARTESIAN_POINT ( 'NONE',  ( 2.224758126099999789, 1476.466451453390164, 198.2506516800989971 ) ) ;
#101236=CARTESIAN_POINT ( 'NONE',  ( -8.375043687299998041, 1424.685418102950052, 206.2101447219289696 ) ) ;
#101240=CARTESIAN_POINT ( 'NONE',  ( 7.380481980853459412, 1426.294419419770065, 212.6173424388080093 ) ) ;
#101241=CARTESIAN_POINT ( 'NONE',  ( 8.842788026528301870, 1423.233140882379985, 211.5963855810900043 ) ) ;
#101247=CARTESIAN_POINT ( 'NONE',  ( -1.312249485446211450, 1488.152622635656144, 219.9118893847204390 ) ) ;
#101251=CARTESIAN_POINT ( 'NONE',  ( 4.904030442849999893, 1425.409506399530073, 209.9084226658820000 ) ) ;
#101255=CARTESIAN_POINT ( 'NONE',  ( 10.94747859850000005, 1461.374937641390034, 209.8474444777559995 ) ) ;
#101274=CARTESIAN_POINT ( 'NONE',  ( 1.194678736856909840, 1445.356568564189956, 199.1147239880469897 ) ) ;
#101275=FACE_OUTER_BOUND ( 'NONE', #13691, .T. ) ;
#101277=CARTESIAN_POINT ( 'NONE',  ( -10.92262152852349999, 1480.972147131519705, 210.3691105597789885 ) ) ;
#101279=CARTESIAN_POINT ( 'NONE',  ( 6.357608626507394334, 1435.035992033701632, 203.3974798508943422 ) ) ;
#101281=CARTESIAN_POINT ( 'NONE',  ( 2.487935123020000194, 1508.551704408389924, 204.1347675455010062 ) ) ;
#101282=CARTESIAN_POINT ( 'NONE',  ( 12.01380273547430022, 1501.779913421650008, 213.3188837843350143 ) ) ;
#101283=CARTESIAN_POINT ( 'NONE',  ( 8.286012754340001507, 1421.269451573359902, 196.1401172957990013 ) ) ;
#101285=CARTESIAN_POINT ( 'NONE',  ( 10.13999722834100048, 1479.891769232120168, 205.9780649761750055 ) ) ;
#101292=EDGE_LOOP ( 'NONE', ( #109493, #108116, #26514, #21102, #35088 ) ) ;
#101298=CARTESIAN_POINT ( 'NONE',  ( 10.54753901010710138, 1427.432118304579944, 209.9055955873279800 ) ) ;
#101300=CARTESIAN_POINT ( 'NONE',  ( 12.43362777651829987, 1421.210458342309948, 203.4350632585469896 ) ) ;
#101301=CARTESIAN_POINT ( 'NONE',  ( 1.483741821009999962, 1430.780200044390085, 217.7366157072389967 ) ) ;
#101306=CARTESIAN_POINT ( 'NONE',  ( -9.843047294206771269, 1461.614624003160088, 208.6138576386200043 ) ) ;
#101308=FACE_OUTER_BOUND ( 'NONE', #100992, .T. ) ;
#101309=CARTESIAN_POINT ( 'NONE',  ( 11.00511108145959938, 1420.479169930370063, 198.1891849291089898 ) ) ;
#101311=CARTESIAN_POINT ( 'NONE',  ( 9.297172576236979680, 1464.629289270589879, 212.4694656482230073 ) ) ;
#101318=CARTESIAN_POINT ( 'NONE',  ( 0.7430128073871236083, 1477.852875664036219, 198.7306773389195484 ) ) ;
#101320=CARTESIAN_POINT ( 'NONE',  ( -1.118758552070000079, 1515.569725561690120, 205.1507450494889895 ) ) ;
#101322=CARTESIAN_POINT ( 'NONE',  ( -17.66147425336259857, 1440.150478482380095, 218.7822780451419931 ) ) ;
#101323=CARTESIAN_POINT ( 'NONE',  ( -19.27023455780000205, 1418.866878321930017, 210.2656499040089670 ) ) ;
#101328=CARTESIAN_POINT ( 'NONE',  ( -4.367937192439999450, 1447.898255911189835, 190.6350925615990093 ) ) ;
#101332=EDGE_LOOP ( 'NONE', ( #92730, #100854 ) ) ;
#101337=CARTESIAN_POINT ( 'NONE',  ( 3.063200971469999701, 1505.793422128889915, 221.5342279770990217 ) ) ;
#101342=CARTESIAN_POINT ( 'NONE',  ( 4.329448776040000446, 1515.064792882589927, 210.9648081929590262 ) ) ;
#101345=CARTESIAN_POINT ( 'NONE',  ( 11.19645453711150118, 1427.175649664649882, 208.5743989061170112 ) ) ;
#101351=CARTESIAN_POINT ( 'NONE',  ( 4.321260515560000570, 1472.734096669689961, 218.3662689135690016 ) ) ;
#101352=( BOUNDED_CURVE ( )  B_SPLINE_CURVE ( 3, ( #91229, #14509, #377, #73337 ),
 .UNSPECIFIED., .F., .F. ) 
 B_SPLINE_CURVE_WITH_KNOTS ( ( 4, 4 ),
 ( 4.154228272801879562, 5.270549769551020169 ),
 .UNSPECIFIED. ) 
 CURVE ( )  GEOMETRIC_REPRESENTATION_ITEM ( )  RATIONAL_B_SPLINE_CURVE ( ( 1.000000000000000000, 0.8988204416492726612, 0.8988204416492726612, 1.000000000000000000 ) ) 
 REPRESENTATION_ITEM ( '' )  );
#101360=CARTESIAN_POINT ( 'NONE',  ( 9.923042113430000200, 1451.489751075389904, 207.3834753964790139 ) ) ;
#101361=CARTESIAN_POINT ( 'NONE',  ( -8.190304658720000575, 1512.060957475689975, 212.0841603825689958 ) ) ;
#101364=EDGE_CURVE ( 'NONE', #108882, #109440, #96315, .T. ) ;
#101374=VERTEX_POINT ( 'NONE', #17614 ) ;
#101384=CARTESIAN_POINT ( 'NONE',  ( 12.65743788132100178, 1500.841905234319711, 210.2807706420859972 ) ) ;
#101386=CARTESIAN_POINT ( 'NONE',  ( 4.956729644103719856, 1508.551704408389924, 212.0071758648730054 ) ) ;
#101388=EDGE_LOOP ( 'NONE', ( #105609, #4086, #53776, #80304 ) ) ;
#101389=CARTESIAN_POINT ( 'NONE',  ( -16.53114349369899827, 1465.611506726459993, 220.7423202708849885 ) ) ;
#101391=VERTEX_POINT ( 'NONE', #77298 ) ;
#101394=CARTESIAN_POINT ( 'NONE',  ( -1.985912070879999991, 1431.344737485190308, 203.7584604878390167 ) ) ;
#101396=CARTESIAN_POINT ( 'NONE',  ( -7.604021728224319432, 1508.390716753870265, 219.6025803338619937 ) ) ;
#101397=CARTESIAN_POINT ( 'NONE',  ( -14.74338484529040016, 1507.984222099330054, 209.4136964162090067 ) ) ;
#101401=VECTOR ( 'NONE', #24110, 1000.000000000000000 ) ;
#101415=B_SPLINE_CURVE_WITH_KNOTS ( 'NONE', 3,
 ( #93281, #16544, #68120, #67560, #101663, #74310, #7624, #75408, #23317, #59161, #66467, #109548, #102232, #74853, #6529, #50735, #25510, #108439, #24952, #31720, #65906, #32821, #100024, #57509, #91634, #67008, #101118, #49101 ),
 .UNSPECIFIED., .F., .F.,
 ( 4, 3, 3, 3, 3, 3, 3, 3, 3, 4 ),
 ( 4.991132198461049718, 5.278154230359260346, 5.575591039645609648, 5.870273492830619944, 6.165162712813499368, 6.464350792820829916, 6.767514390815449588, 7.076365246473460324, 7.382407343323190041, 7.657648704650000582 ),
 .UNSPECIFIED. ) ;
#101420=CARTESIAN_POINT ( 'NONE',  ( -4.853522982481027093, 1432.607957074035767, 216.0726889064482918 ) ) ;
#101421=CARTESIAN_POINT ( 'NONE',  ( -1.921445414331789836, 1468.480943170730143, 219.3341389517340190 ) ) ;
#101424=CARTESIAN_POINT ( 'NONE',  ( -9.558504124660036183, 1469.579538799191596, 215.2844292078696071 ) ) ;
#101428=ADVANCED_FACE ( 'NONE', ( #54319 ), #84742, .T. ) ;
#101429=CARTESIAN_POINT ( 'NONE',  ( -21.68513540049999833, 1505.549217140589917, 209.4741210534890001 ) ) ;
#101430=CARTESIAN_POINT ( 'NONE',  ( 6.277214161762089795, 1467.366245655900002, 199.9216203958389997 ) ) ;
#101431=CYLINDRICAL_SURFACE ( 'NONE', #43774, 2.458500000000005237 ) ;
#101432=AXIS2_PLACEMENT_3D ( 'NONE', #91449, #31528, #73002 ) ;
#101434=ORIENTED_EDGE ( 'NONE', *, *, #74822, .F. ) ;
#101439=CARTESIAN_POINT ( 'NONE',  ( 5.430432121089999953, 1505.407861808090047, 219.8354485799989959 ) ) ;
#101454=FACE_OUTER_BOUND ( 'NONE', #37382, .T. ) ;
#101466=DIRECTION ( 'NONE',  ( -0.9364122222710381527, 0.3043600949234490649, -0.1746341392729520714 ) ) ;
#101468=CARTESIAN_POINT ( 'NONE',  ( -15.35210835959999898, 1415.142250310439749, 207.5991997658489936 ) ) ;
#101471=CARTESIAN_POINT ( 'NONE',  ( -5.301601239306844349, 1495.069293905918585, 198.4488062458674733 ) ) ;
#101476=CARTESIAN_POINT ( 'NONE',  ( -11.77227379640609861, 1507.876490232319838, 208.2428952626790135 ) ) ;
#101477=CARTESIAN_POINT ( 'NONE',  ( -9.417897711209606726, 1420.662740822867818, 195.0156077546988627 ) ) ;
#101483=CARTESIAN_POINT ( 'NONE',  ( -9.276942849846040673, 1461.680302431059999, 206.2489141960740255 ) ) ;
#101487=CARTESIAN_POINT ( 'NONE',  ( 6.033702791082116157, 1471.717643617360409, 217.3099286337410092 ) ) ;
#101489=VECTOR ( 'NONE', #37245, 1000.000000000000114 ) ;
#101493=CARTESIAN_POINT ( 'NONE',  ( 10.02412832500950124, 1480.534670654839829, 205.8825814297850059 ) ) ;
#101495=CARTESIAN_POINT ( 'NONE',  ( -17.45557808899999941, 1442.885315458190007, 219.4073627859989699 ) ) ;
#101497=CARTESIAN_POINT ( 'NONE',  ( 16.66442743449040265, 1492.498864362939912, 193.3249227321730075 ) ) ;
#101501=CARTESIAN_POINT ( 'NONE',  ( 8.177817319380210392, 1422.878296244719877, 213.9391555383760135 ) ) ;
#101503=CARTESIAN_POINT ( 'NONE',  ( -14.43458679349279983, 1420.584116066620027, 213.5288221046679666 ) ) ;
#101522=CARTESIAN_POINT ( 'NONE',  ( 3.983717799080809474, 1515.551844914359890, 206.7919068468160049 ) ) ;
#101523=CARTESIAN_POINT ( 'NONE',  ( 3.252451448209999985, 1444.627347679690047, 200.7572266927390103 ) ) ;
#101542=CARTESIAN_POINT ( 'NONE',  ( -9.038752695348167165, 1474.281940146342549, 204.2026377629549927 ) ) ;
#101556=EDGE_CURVE ( 'NONE', #5409, #103262, #58750, .T. ) ;
#101562=CARTESIAN_POINT ( 'NONE',  ( 5.383599734016756955, 1505.915176669089760, 219.4473941718215144 ) ) ;
#101569=CARTESIAN_POINT ( 'NONE',  ( -2.594792379150919981, 1429.144945495409956, 200.1164755763740004 ) ) ;
#101585=CARTESIAN_POINT ( 'NONE',  ( -8.796782887879999180, 1468.013265501289879, 190.7844261045989640 ) ) ;
#101589=CARTESIAN_POINT ( 'NONE',  ( -9.571128596670011035, 1448.740117217580064, 208.7132155754160010 ) ) ;
#101592=ORIENTED_EDGE ( 'NONE', *, *, #108401, .T. ) ;
#101599=CARTESIAN_POINT ( 'NONE',  ( -7.818293364874802975, 1461.813659484448408, 203.3506159379348048 ) ) ;
#101600=CARTESIAN_POINT ( 'NONE',  ( 4.105220072099999840, 1467.927057061790038, 218.2260594483290106 ) ) ;
#101607=CARTESIAN_POINT ( 'NONE',  ( 3.876688749703430137, 1507.337224526469981, 220.1660795228299889 ) ) ;
#101610=CARTESIAN_POINT ( 'NONE',  ( 9.805118623159389202, 1463.039694706869113, 208.9028931574285934 ) ) ;
#101614=CARTESIAN_POINT ( 'NONE',  ( 11.87050035490000077, 1500.995002434390017, 208.8930718320189897 ) ) ;
#101617=CARTESIAN_POINT ( 'NONE',  ( -2.801043665293740048, 1515.551704203360032, 212.9510687676740019 ) ) ;
#101618=DIRECTION ( 'NONE',  ( 0.000000000000000000, -1.836970198721029688E-16, -1.000000000000000000 ) ) ;
#101622=CARTESIAN_POINT ( 'NONE',  ( -5.157094080490000287, 1434.836961744490054, 211.6805039011290148 ) ) ;
#101628=CARTESIAN_POINT ( 'NONE',  ( 0.6898828221520181270, 1435.696354552260118, 227.5721478921569769 ) ) ;
#101629=CARTESIAN_POINT ( 'NONE',  ( -15.30505509804103070, 1416.034713203068122, 206.6286703179388553 ) ) ;
#101630=CARTESIAN_POINT ( 'NONE',  ( 2.140393166329999985, 1456.253627881090097, 219.1100769117989842 ) ) ;
#101632=CARTESIAN_POINT ( 'NONE',  ( -8.557074290199999211, 1446.797689270289993, 213.4441513527789880 ) ) ;
#101637=CARTESIAN_POINT ( 'NONE',  ( 7.451350174509999924, 1424.542899935769810, 212.3981519012789931 ) ) ;
#101639=CARTESIAN_POINT ( 'NONE',  ( -3.296219135334409689, 1454.279253091320015, 199.1722461497759866 ) ) ;
#101644=CARTESIAN_POINT ( 'NONE',  ( 5.485824899879999883, 1494.971430001190129, 220.2122618358989712 ) ) ;
#101659=CARTESIAN_POINT ( 'NONE',  ( -9.220308107448930812, 1448.515117430399869, 210.2021542620989862 ) ) ;
#101663=CARTESIAN_POINT ( 'NONE',  ( -4.327091944037070093, 1515.154796665630101, 209.3803870859530036 ) ) ;
#101666=ORIENTED_EDGE ( 'NONE', *, *, #2868, .F. ) ;
#101668=CARTESIAN_POINT ( 'NONE',  ( 5.314610460026229610, 1424.245163613919885, 193.3438872810020257 ) ) ;
#101684=CARTESIAN_POINT ( 'NONE',  ( -8.588755447433969792, 1437.818850531529961, 207.9413692731380081 ) ) ;
#101687=CARTESIAN_POINT ( 'NONE',  ( 3.925166330978474338, 1441.144975113518058, 217.4787537044992121 ) ) ;
#101690=CARTESIAN_POINT ( 'NONE',  ( 10.56340574544989863, 1460.179522302520127, 206.3975810254339933 ) ) ;
#101702=CARTESIAN_POINT ( 'NONE',  ( -10.96160898770000180, 1471.053908682290057, 208.7203235810210060 ) ) ;
#101711=CARTESIAN_POINT ( 'NONE',  ( 15.32773529925650102, 1420.119835273649869, 210.6256678854140034 ) ) ;
#101713=CARTESIAN_POINT ( 'NONE',  ( 4.297657077759999389, 1487.299056241089829, 198.3739788318989952 ) ) ;
#101714=CARTESIAN_POINT ( 'NONE',  ( 4.002785782343220689, 1430.446709099730015, 217.7271167850740028 ) ) ;
#101717=CARTESIAN_POINT ( 'NONE',  ( -11.25901873334290038, 1500.172003390719965, 210.8567363214919794 ) ) ;
#101724=EDGE_CURVE ( 'NONE', #18362, #4497, #63575, .T. ) ;
#101725=CARTESIAN_POINT ( 'NONE',  ( -17.20794664139999952, 1420.221446635479879, 203.8085880389089937 ) ) ;
#101728=CARTESIAN_POINT ( 'NONE',  ( -16.80827233337889837, 1508.551704408389924, 212.8354810807049944 ) ) ;
#101730=CARTESIAN_POINT ( 'NONE',  ( 1.742416831430000146, 1474.343050638090062, 219.6228428829990094 ) ) ;
#101737=CARTESIAN_POINT ( 'NONE',  ( 5.312679136500000787, 1493.059131431590231, 218.8466398904690209 ) ) ;
#101741=CARTESIAN_POINT ( 'NONE',  ( -11.19185250109059915, 1418.956138653949893, 197.9931542539910083 ) ) ;
#101744=ORIENTED_EDGE ( 'NONE', *, *, #95276, .T. ) ;
#101753=CARTESIAN_POINT ( 'NONE',  ( 20.75865085201310123, 1455.056320380349916, 207.3304550445770076 ) ) ;
#101757=CARTESIAN_POINT ( 'NONE',  ( 11.00856587417569976, 1491.731810436480146, 211.0639928105959768 ) ) ;
#101758=CARTESIAN_POINT ( 'NONE',  ( -0.9024754025550010272, 1457.070408835690159, 219.3409596864989908 ) ) ;
#101759=EDGE_LOOP ( 'NONE', ( #33093, #88092, #74893, #19003 ) ) ;
#101766=CARTESIAN_POINT ( 'NONE',  ( -21.11353872800000175, 1504.854732156090222, 213.2197078311189955 ) ) ;
#101769=CARTESIAN_POINT ( 'NONE',  ( -7.203791267549999766, 1462.997894367589879, 202.2063197434089830 ) ) ;
#101772=CARTESIAN_POINT ( 'NONE',  ( -20.87069991009999725, 1506.658021081189872, 214.5368842940590071 ) ) ;
#101773=CARTESIAN_POINT ( 'NONE',  ( -16.03202129173239854, 1508.551704408389924, 213.7937094156460205 ) ) ;
#101782=B_SPLINE_SURFACE_WITH_KNOTS ( 'NONE', 5, 5, ( 
 ( #81638, #88949, #98451, #90600, #56467, #21165 ),
 ( #4415, #48629, #55373, #82760, #72720, #21720 ),
 ( #6052, #39084, #98991, #71658, #73263, #107402 ),
 ( #30698, #22266, #91708, #43939, #1387, #60764 ),
 ( #76995, #14982, #43393, #69722, #26568, #51229 ),
 ( #34972, #94315, #77543, #847, #42834, #301 ),
 ( #65989, #95444, #9774, #34428, #18708, #17594 ),
 ( #35528, #68601, #52361, #78083, #103840, #60196 ),
 ( #66540, #69155, #49178, #85933, #18164, #85362 ) ),
 .UNSPECIFIED., .F., .F., .F.,
 ( 6, 3, 6 ),
 ( 6, 6 ),
 ( 3.153842328722349819, 5.422189802880000187, 7.690534356440440256 ),
 ( -0.0004137068776518209689, 2.000000000000000000 ),
 .UNSPECIFIED. ) ;
#101783=CARTESIAN_POINT ( 'NONE',  ( -3.189845314219999395, 1471.643321501789842, 187.3778031497989787 ) ) ;
#101790=CARTESIAN_POINT ( 'NONE',  ( -13.19474177440000062, 1503.345007237690197, 208.6791437603130248 ) ) ;
#101791=CARTESIAN_POINT ( 'NONE',  ( -2.093884640795049545, 1421.271540113659967, 193.7238421870019636 ) ) ;
#101793=CARTESIAN_POINT ( 'NONE',  ( -2.624961820489999820, 1475.614191382290073, 198.7376068992990099 ) ) ;
#101799=CARTESIAN_POINT ( 'NONE',  ( -8.571317710789999822, 1424.360885749340014, 206.8919365348089912 ) ) ;
#101802=CARTESIAN_POINT ( 'NONE',  ( -6.672894824142502124, 1470.955718715978492, 216.7252699277640602 ) ) ;
#101803=CARTESIAN_POINT ( 'NONE',  ( 7.454189929035849538, 1426.129717880560065, 212.4394750011670112 ) ) ;
#101808=CARTESIAN_POINT ( 'NONE',  ( -11.08420618087970055, 1492.086055949669799, 207.0911962512699915 ) ) ;
#101812=CARTESIAN_POINT ( 'NONE',  ( 7.893069735660001029, 1424.490648431219824, 211.8460496558390105 ) ) ;
#101814=CARTESIAN_POINT ( 'NONE',  ( 18.20258715539999983, 1429.723789929190161, 209.1218459616989946 ) ) ;
#101818=CARTESIAN_POINT ( 'NONE',  ( 8.132247801209091520, 1436.307234911819933, 206.3069409763359943 ) ) ;
#101820=ORIENTED_EDGE ( 'NONE', *, *, #41416, .F. ) ;
#101827=CARTESIAN_POINT ( 'NONE',  ( 3.116136652999580203, 1509.034536824670113, 213.6092057033540073 ) ) ;
#101836=CARTESIAN_POINT ( 'NONE',  ( 15.48933771679000060, 1431.961443115730162, 219.1762183192749944 ) ) ;
#101837=ORIENTED_EDGE ( 'NONE', *, *, #108164, .F. ) ;
#101838=CARTESIAN_POINT ( 'NONE',  ( 4.678144232538230085, 1508.611354625609920, 206.6339229097249870 ) ) ;
#101840=CARTESIAN_POINT ( 'NONE',  ( 6.600633841864996576, 1435.170991571107834, 203.6679139044261717 ) ) ;
#101842=CARTESIAN_POINT ( 'NONE',  ( -4.504070374734999938, 1508.551704408389924, 213.0883275018930192 ) ) ;
#101843=CARTESIAN_POINT ( 'NONE',  ( -1.842962231260000028, 1515.551704408389924, 212.9514660752490158 ) ) ;
#101844=CARTESIAN_POINT ( 'NONE',  ( 7.398264911990000137, 1422.106259636749883, 195.6015909957990289 ) ) ;
#101845=CARTESIAN_POINT ( 'NONE',  ( -2.672909466071800466, 1432.986942304690047, 218.2820170679659952 ) ) ;
#101846=CARTESIAN_POINT ( 'NONE',  ( -4.678725631789999895, 1495.985945357489982, 198.7901154368990149 ) ) ;
#101849=DIRECTION ( 'NONE',  ( 4.465978680329379737E-17, 1.000000000000000000, -2.349386720892264891E-16 ) ) ;
#101855=CARTESIAN_POINT ( 'NONE',  ( 5.170554601400000116, 1484.055082523290139, 219.7711189574989703 ) ) ;
#101859=CARTESIAN_POINT ( 'NONE',  ( 9.398642880860540672, 1427.777155254299942, 211.5857661256089841 ) ) ;
#101860=CARTESIAN_POINT ( 'NONE',  ( 11.18358067844100034, 1422.622611808279999, 203.3483468631889934 ) ) ;
#101868=CARTESIAN_POINT ( 'NONE',  ( -10.13020485171709950, 1461.692418066599885, 209.8925213690289979 ) ) ;
#101871=CARTESIAN_POINT ( 'NONE',  ( 9.501937463079149992, 1425.198055971670101, 196.1347459188490063 ) ) ;
#101872=CARTESIAN_POINT ( 'NONE',  ( 8.798972287939317738, 1464.673512069870185, 213.6296587821800017 ) ) ;
#101876=CARTESIAN_POINT ( 'NONE',  ( -7.871069549766747109, 1426.247912565474508, 206.9070274792266559 ) ) ;
#101877=B_SPLINE_CURVE_WITH_KNOTS ( 'NONE', 5,
 ( #38856, #73035, #107174, #30466, #64652, #56230 ),
 .UNSPECIFIED., .F., .F.,
 ( 6, 6 ),
 ( -1.999999954793280077, 0.000000000000000000 ),
 .UNSPECIFIED. ) ;
#101878=CARTESIAN_POINT ( 'NONE',  ( 4.687651746879999415, 1478.378160227390254, 228.9010599218989910 ) ) ;
#101880=CARTESIAN_POINT ( 'NONE',  ( 3.374302901398949839, 1508.029867056955027, 220.2219692825980530 ) ) ;
#101882=CARTESIAN_POINT ( 'NONE',  ( -20.43379411225540210, 1466.940147600540058, 211.2182735651869905 ) ) ;
#101884=CARTESIAN_POINT ( 'NONE',  ( -19.70057179385869972, 1418.794758439270026, 207.3135327979470048 ) ) ;
#101894=CARTESIAN_POINT ( 'NONE',  ( -10.18171327880000021, 1472.619598059789951, 209.5761564533819978 ) ) ;
#101897=CARTESIAN_POINT ( 'NONE',  ( 7.389795930078929764, 1504.900412948340090, 213.9846519657809836 ) ) ;
#101898=CARTESIAN_POINT ( 'NONE',  ( -9.564290896847950307, 1437.870856459579954, 211.8468459910199897 ) ) ;
#101906=CARTESIAN_POINT ( 'NONE',  ( 11.63491105067470066, 1421.973764464760052, 207.9107772468980215 ) ) ;
#101910=CARTESIAN_POINT ( 'NONE',  ( 0.3947013525697100622, 1437.804170063959873, 227.6754659744219680 ) ) ;
#101912=CARTESIAN_POINT ( 'NONE',  ( 2.366934492629999998, 1474.701470341489994, 220.3007639910990179 ) ) ;
#101913=ADVANCED_FACE ( 'NONE', ( #75919 ), #8760, .T. ) ;
#101915=CARTESIAN_POINT ( 'NONE',  ( 12.51045652733512803, 1415.677402202029953, 211.4999743317719663 ) ) ;
#101918=CARTESIAN_POINT ( 'NONE',  ( -8.955241798779999485, 1494.044665287490034, 202.1005013471790335 ) ) ;
#101920=ADVANCED_FACE ( 'NONE', ( #31511 ), #40902, .T. ) ;
#101923=EDGE_CURVE ( 'NONE', #10343, #109438, #30203, .T. ) ;
#101926=CARTESIAN_POINT ( 'NONE',  ( 8.526934319540000473, 1449.624708711990024, 204.5462524797590049 ) ) ;
#101933=CARTESIAN_POINT ( 'NONE',  ( -2.490606800900000195, 1496.797481259589858, 198.0109085349990039 ) ) ;
#101944=VECTOR ( 'NONE', #73219, 1000.000000000000000 ) ;
#101949=CARTESIAN_POINT ( 'NONE',  ( 12.68260786739960011, 1500.745025545950057, 209.9285465654390066 ) ) ;
#101951=CARTESIAN_POINT ( 'NONE',  ( 4.580254622799669662, 1508.551704408389924, 212.9784530087700318 ) ) ;
#101955=CARTESIAN_POINT ( 'NONE',  ( 9.369980246745740260, 1462.099920443929932, 206.4857951425539966 ) ) ;
#101961=CARTESIAN_POINT ( 'NONE',  ( 10.53440680805939955, 1452.831114188890069, 210.2190104787899827 ) ) ;
#101962=CARTESIAN_POINT ( 'NONE',  ( -2.487935121788300119, 1509.038615937200120, 204.6345961869410246 ) ) ;
#101963=CARTESIAN_POINT ( 'NONE',  ( -11.81019069571562774, 1417.596857770419547, 199.2280744327704838 ) ) ;
#101965=CARTESIAN_POINT ( 'NONE',  ( 4.326992699989999913, 1515.158586642790169, 209.1218459614979963 ) ) ;
#101966=CARTESIAN_POINT ( 'NONE',  ( -6.843521712735489260, 1453.772848492380035, 202.7227712865530123 ) ) ;
#101970=DIRECTION ( 'NONE',  ( 4.465978680329379737E-17, 1.000000000000000000, -2.349386720892264891E-16 ) ) ;
#101976=CARTESIAN_POINT ( 'NONE',  ( 19.25089118869999893, 1455.005958191190075, 207.2694656823390176 ) ) ;
#101977=B_SPLINE_CURVE_WITH_KNOTS ( 'NONE', 3,
 ( #16733, #109731, #92922, #16195, #67747, #8356, #42520, #50396, #84524, #7813, #33550, #110828, #51482, #78908, #88395, #87863, #79450, #1652, #2762, #102963, #20075, #69416, #45314, #69971, #70524, #52047, #36881, #71076, #19520, #34673, #35787, #86183, #2215, #105200 ),
 .UNSPECIFIED., .F., .F.,
 ( 4, 3, 3, 3, 3, 3, 3, 3, 3, 3, 3, 4 ),
 ( -26.06149361980000023, -24.76029548010210135, -23.45909734040419892, -22.14719351067359909, -21.39637773376540153, -20.04300759126989817, -18.69429331602630029, -17.34897622602300160, -16.01021078912490125, -14.67612915947669983, -13.34696737019829982, -12.02292824550000105 ),
 .UNSPECIFIED. ) ;
#101982=CARTESIAN_POINT ( 'NONE',  ( 5.415590649712958893, 1429.910603248089956, 216.9138056063569877 ) ) ;
#101983=CARTESIAN_POINT ( 'NONE',  ( -16.65376764594610037, 1508.454796205149933, 213.7212175226700026 ) ) ;
#101984=CARTESIAN_POINT ( 'NONE',  ( -10.21381549268537725, 1491.160059455200326, 213.2743110981627126 ) ) ;
#101987=DIRECTION ( 'NONE',  ( -1.000000000000000000, -2.249639673992789970E-32, -1.224646799147350002E-16 ) ) ;
#101988=CARTESIAN_POINT ( 'NONE',  ( 5.312679136500000787, 1493.059131431590231, 218.8466398904690209 ) ) ;
#101992=CARTESIAN_POINT ( 'NONE',  ( 2.487935098288932778, 1508.551704408389924, 213.9544627682086286 ) ) ;
#101994=B_SPLINE_SURFACE_WITH_KNOTS ( 'NONE', 5, 5, ( 
 ( #39747, #65519, #83946, #49816, #99077, #38634 ),
 ( #30227, #64417, #73354, #30784, #22358, #99626 ),
 ( #57121, #91246, #14527, #48717, #74473, #108601 ),
 ( #31889, #66075, #68287, #93439, #76653, #16708 ),
 ( #9450, #110803, #35201, #43615, #52017, #85586 ),
 ( #17262, #51454, #8882, #69388, #58757, #102935 ) ),
 .UNSPECIFIED., .F., .F., .F.,
 ( 6, 6 ),
 ( 6, 6 ),
 ( 28.72930409989999845, 41.05058650750000027 ),
 ( 0.000000000000000000, 2.000000000000000000 ),
 .UNSPECIFIED. ) ;
#101996=ORIENTED_EDGE ( 'NONE', *, *, #48902, .T. ) ;
#102001=CARTESIAN_POINT ( 'NONE',  ( -11.30420028228749985, 1500.584958202139887, 210.9988023051070059 ) ) ;
#102004=AXIS2_PLACEMENT_3D ( 'NONE', #69983, #78354, #27390 ) ;
#102005=CARTESIAN_POINT ( 'NONE',  ( 0.7637831719629990523, 1508.279675140790005, 220.7126945919989964 ) ) ;
#102007=CARTESIAN_POINT ( 'NONE',  ( 1.859161530581180166, 1431.069669433720037, 199.8328166829190025 ) ) ;
#102008=CARTESIAN_POINT ( 'NONE',  ( -10.80279757036180044, 1461.800106919070004, 211.1805521804130024 ) ) ;
#102014=CARTESIAN_POINT ( 'NONE',  ( -9.902328854349999432, 1479.355524923690155, 213.2350952645890061 ) ) ;
#102022=CARTESIAN_POINT ( 'NONE',  ( 4.492546581380000958, 1453.878649273890005, 217.3453973181289882 ) ) ;
#102027=CARTESIAN_POINT ( 'NONE',  ( -14.98285036589999919, 1415.729638096350072, 205.4713522697590236 ) ) ;
#102029=CARTESIAN_POINT ( 'NONE',  ( -5.664944777449460567, 1484.831651990110004, 198.6533526945029848 ) ) ;
#102031=CARTESIAN_POINT ( 'NONE',  ( -5.245637547039999404, 1497.146055658990008, 219.2578757579989883 ) ) ;
#102033=CARTESIAN_POINT ( 'NONE',  ( -1.450592998049999860, 1477.402861163290027, 201.6210515953190168 ) ) ;
#102038=CARTESIAN_POINT ( 'NONE',  ( -18.65075743919999951, 1443.653128712389844, 211.8055058365289938 ) ) ;
#102054=CARTESIAN_POINT ( 'NONE',  ( 5.170554601400000116, 1484.055082523290139, 219.7711189574989703 ) ) ;
#102055=CARTESIAN_POINT ( 'NONE',  ( 10.24103526349649940, 1480.245554142349874, 206.6866148605930107 ) ) ;
#102058=ADVANCED_FACE ( 'NONE', ( #56258 ), #31967, .T. ) ;
#102059=CARTESIAN_POINT ( 'NONE',  ( -17.52911390707280148, 1441.908568393189853, 219.1841137618270068 ) ) ;
#102068=ADVANCED_FACE ( 'NONE', ( #98799 ), #35494, .T. ) ;
#102085=CARTESIAN_POINT ( 'NONE',  ( 3.829222816048220235, 1515.551704203360032, 206.3208014481249961 ) ) ;
#102088=LINE ( 'NONE', #20289, #102613 ) ;
#102092=CARTESIAN_POINT ( 'NONE',  ( 1.882487193640000056, 1467.451596611890182, 219.3027413508989980 ) ) ;
#102094=PRESENTATION_STYLE_ASSIGNMENT (( #50610 ) ) ;
#102099=B_SPLINE_CURVE_WITH_KNOTS ( 'NONE', 3,
 ( #48128, #74441, #30754, #100704, #108569, #90657, #82267, #108009, #64388, #39147, #81696, #91760, #98507, #107459, #64935, #49236, #99048, #13940, #32421, #31858, #31304, #13384, #39717, #47571, #74989, #92309, #5566, #56528, #73323, #40260, #40812, #82811, #49782, #15036, #73881, #83359, #21775, #14495, #15580, #55976, #65488, #66044, #66600, #99598, #23986, #22881, #48687, #57090, #83914, #91215, #100169, #6104, #23452, #57647, #6658, #109140, #58182, #7220, #41377, #75542, #30193, #18352, #51427, #69356, #35172, #43586, #77193, #9423, #60394, #103465, #77735, #8853, #26772, #34621, #60960, #86676, #16682, #43037, #110220, #95085, #496, #1048, #41925, #93966, #25651, #76624, #68805, #102907, #26205, #8304, #76081, #7759, #94514, #52544, #9973, #51989, #84472, #17788, #58728, #110776, #42466, #44143, #34068, #109677, #33494, #101803, #67695, #25095, #32953, #68259, #67143, #102368, #101240, #85557, #24540, #92863, #86129, #50879, #16143, #85010, #50346, #59300, #93415, #59842, #17230, #53100, #71590, #70467, #28435, #18904 ),
 .UNSPECIFIED., .F., .F.,
 ( 4, 3, 3, 3, 3, 3, 3, 3, 3, 3, 3, 3, 3, 3, 3, 3, 3, 3, 3, 3, 3, 3, 3, 3, 3, 3, 3, 3, 3, 3, 3, 3, 3, 3, 3, 3, 3, 3, 3, 3, 3, 3, 3, 4 ),
 ( 0.000000000000000000, 0.4989958285304099683, 0.8732426999282179025, 1.187904378483179979, 1.485459211540649971, 1.764154662664569884, 1.995983314121640095, 2.218900690584800106, 2.411230156830109994, 2.588723306273699620, 2.751770446255200397, 2.887652819974260154, 3.035486073829570142, 3.141664737081030445, 3.183319327684869915, 3.276504077055930164, 3.377348710061859993, 3.470358065450380280, 3.556407254322629719, 3.641400281485230206, 3.717201824902540253, 3.726393308647829805, 3.795380765736819928, 3.871873908516200391, 3.948738929127949771, 4.018859912850369476, 4.077147876327860132, 4.166923348113540371, 4.261100944480360475, 4.361051690202209841, 4.473351797408369634, 4.591235991841460695, 4.702032100850900065, 4.748093182062699924, 4.895722542919810572, 5.060544476256770174, 5.242866039422230173, 5.511025200193289564, 5.770121536528019845, 6.041084857940309583, 6.328006033295999977, 6.655379715367800486, 7.044317073833579634, 7.372157449769999538 ),
 .UNSPECIFIED. ) ;
#102105=ORIENTED_EDGE ( 'NONE', *, *, #71943, .F. ) ;
#102130=CARTESIAN_POINT ( 'NONE',  ( 3.717177354979999571, 1462.278529190689824, 228.4137915130989995 ) ) ;
#102135=CARTESIAN_POINT ( 'NONE',  ( 9.512629190459559680, 1434.630476851629965, 206.8407525937180083 ) ) ;
#102155=CARTESIAN_POINT ( 'NONE',  ( -8.356095914484159337, 1508.431967280379922, 219.3425879849650073 ) ) ;
#102156=CARTESIAN_POINT ( 'NONE',  ( -1.551161424019060098, 1463.265709907049995, 199.4650991780359846 ) ) ;
#102158=CARTESIAN_POINT ( 'NONE',  ( 10.92857032808210072, 1460.888924644350027, 208.5047758900509791 ) ) ;
#102160=CARTESIAN_POINT ( 'NONE',  ( 3.919632032540000477, 1466.374841473789729, 219.0280172745789855 ) ) ;
#102161=CARTESIAN_POINT ( 'NONE',  ( 1.367745396099944832, 1468.963081466252106, 219.0596951095364773 ) ) ;
#102167=CARTESIAN_POINT ( 'NONE',  ( -2.847678236620000192, 1430.845636562190066, 201.2564352188489920 ) ) ;
#102171=( BOUNDED_CURVE ( )  B_SPLINE_CURVE ( 3, ( #12090, #88259, #88807, #63100 ),
 .UNSPECIFIED., .F., .T. ) 
 B_SPLINE_CURVE_WITH_KNOTS ( ( 4, 4 ),
 ( 4.151398476256234815, 5.273379648758210081 ),
 .UNSPECIFIED. ) 
 CURVE ( )  GEOMETRIC_REPRESENTATION_ITEM ( )  RATIONAL_B_SPLINE_CURVE ( ( 1.000000000000000000, 0.8978190064439198759, 0.8978190064439198759, 1.000000000000000000 ) ) 
 REPRESENTATION_ITEM ( '' )  );
#102173=ORIENTED_EDGE ( 'NONE', *, *, #39061, .T. ) ;
#102174=CARTESIAN_POINT ( 'NONE',  ( -4.675540975309999681, 1462.620895424390028, 200.5633310686890241 ) ) ;
#102180=CARTESIAN_POINT ( 'NONE',  ( 11.59305468459999844, 1501.418989384490033, 208.8071487272210049 ) ) ;
#102183=CARTESIAN_POINT ( 'NONE',  ( 7.793367779400000472, 1427.553872258489946, 212.4452625024690064 ) ) ;
#102184=CARTESIAN_POINT ( 'NONE',  ( -2.329939107268110376, 1515.551844914359890, 213.1055637611929967 ) ) ;
#102194=EDGE_CURVE ( 'NONE', #35904, #93500, #12857, .T. ) ;
#102198=CARTESIAN_POINT ( 'NONE',  ( -0.2129047818200029696, 1500.069404719889917, 230.4573127901989835 ) ) ;
#102199=CARTESIAN_POINT ( 'NONE',  ( -15.52168468949967384, 1415.982095105879580, 207.6414872824098836 ) ) ;
#102202=FACE_OUTER_BOUND ( 'NONE', #41697, .T. ) ;
#102219=CARTESIAN_POINT ( 'NONE',  ( 1.145290945507940084, 1458.110487998910003, 199.6352770989870180 ) ) ;
#102221=CARTESIAN_POINT ( 'NONE',  ( 10.24652809674144649, 1501.212611039424701, 203.9352555582063928 ) ) ;
#102224=CARTESIAN_POINT ( 'NONE',  ( -1.138407481869679883, 1475.515787706559877, 197.7305842908260161 ) ) ;
#102228=CARTESIAN_POINT ( 'NONE',  ( -10.33301352385990057, 1447.717428273800124, 209.8082491242700200 ) ) ;
#102232=CARTESIAN_POINT ( 'NONE',  ( -4.327871496238200777, 1515.125026768160069, 209.9123818876519749 ) ) ;
#102236=ORIENTED_EDGE ( 'NONE', *, *, #4394, .F. ) ;
#102237=B_SPLINE_CURVE_WITH_KNOTS ( 'NONE', 5,
 ( #10594, #2768, #44204, #54815, #20082, #1106 ),
 .UNSPECIFIED., .F., .F.,
 ( 6, 6 ),
 ( 0.000000000000000000, 1.000000000000000000 ),
 .UNSPECIFIED. ) ;
#102240=ADVANCED_FACE ( 'NONE', ( #97422 ), #63846, .F. ) ;
#102244=ORIENTED_EDGE ( 'NONE', *, *, #69646, .T. ) ;
#102252=CARTESIAN_POINT ( 'NONE',  ( -10.94922716044850119, 1470.861560421989907, 209.5255082995269902 ) ) ;
#102262=CARTESIAN_POINT ( 'NONE',  ( -18.83642247210000065, 1444.248298674089938, 209.1218459616989946 ) ) ;
#102265=ORIENTED_EDGE ( 'NONE', *, *, #11862, .F. ) ;
#102270=VERTEX_POINT ( 'NONE', #38069 ) ;
#102272=CARTESIAN_POINT ( 'NONE',  ( -11.02166737461350010, 1492.206447049650023, 203.6901558032419928 ) ) ;
#102275=CARTESIAN_POINT ( 'NONE',  ( -14.81511931610000055, 1416.828882134419928, 206.5603892752189950 ) ) ;
#102277=CARTESIAN_POINT ( 'NONE',  ( 4.021865650940000592, 1487.198045919489914, 198.2747322527989979 ) ) ;
#102278=CARTESIAN_POINT ( 'NONE',  ( 2.010167598323350013, 1431.137515179070078, 218.3977979629700030 ) ) ;
#102281=CARTESIAN_POINT ( 'NONE',  ( -1.842963446620164092, 1515.320037145748756, 204.8511296326253159 ) ) ;
#102288=CARTESIAN_POINT ( 'NONE',  ( -16.57873794416559932, 1508.551704408389924, 213.1306309380350115 ) ) ;
#102290=CARTESIAN_POINT ( 'NONE',  ( -21.26826130359999922, 1504.995118174490017, 212.3995629039989979 ) ) ;
#102291=CARTESIAN_POINT ( 'NONE',  ( -11.40436649515589984, 1470.754293980279954, 209.1665043884289901 ) ) ;
#102294=CARTESIAN_POINT ( 'NONE',  ( 5.467155153583750149, 1493.854051205442147, 218.8016796649062883 ) ) ;
#102297=CARTESIAN_POINT ( 'NONE',  ( -2.265088008643420192, 1421.884433507809945, 193.4623903222540093 ) ) ;
#102303=CARTESIAN_POINT ( 'NONE',  ( -4.138993644310000164, 1515.551749209589843, 209.1218459616989946 ) ) ;
#102309=B_SPLINE_CURVE_WITH_KNOTS ( 'NONE', 5,
 ( #57279, #34243, #91407, #57819, #83535, #58909 ),
 .UNSPECIFIED., .F., .F.,
 ( 6, 6 ),
 ( 0.000000000000000000, 1.000000000000000000 ),
 .UNSPECIFIED. ) ;
#102310=CARTESIAN_POINT ( 'NONE',  ( 14.17511973000000047, 1428.761297070790079, 195.0897165316990254 ) ) ;
#102314=CARTESIAN_POINT ( 'NONE',  ( 1.875671004969999833, 1456.514200624189925, 219.5762891113990065 ) ) ;
#102315=VERTEX_POINT ( 'NONE', #67701 ) ;
#102327=CARTESIAN_POINT ( 'NONE',  ( -4.329448776275169664, 1515.064792882719985, 206.7917118343879963 ) ) ;
#102329=CARTESIAN_POINT ( 'NONE',  ( 11.56580875524219998, 1480.193683599319911, 211.4103531732560270 ) ) ;
#102336=CARTESIAN_POINT ( 'NONE',  ( -0.9166357444073550687, 1485.892889838330120, 197.2561232801839992 ) ) ;
#102345=B_SPLINE_CURVE_WITH_KNOTS ( 'NONE', 5,
 ( #97115, #104408, #52919, #96004, #3631, #63008 ),
 .UNSPECIFIED., .F., .F.,
 ( 6, 6 ),
 ( 0.000000000000000000, 1.000000000000000000 ),
 .UNSPECIFIED. ) ;
#102346=CARTESIAN_POINT ( 'NONE',  ( -4.495215926552520003, 1481.166686022519798, 231.0476533587359995 ) ) ;
#102348=DIRECTION ( 'NONE',  ( -0.3083968794178160722, -0.4480171631737070448, 0.8391495613221381378 ) ) ;
#102350=CARTESIAN_POINT ( 'NONE',  ( -17.94925291060000205, 1468.366100212389938, 200.1415149508490003 ) ) ;
#102355=CARTESIAN_POINT ( 'NONE',  ( -2.642331102980000068, 1475.301074652890065, 198.3937767294989953 ) ) ;
#102361=FACE_OUTER_BOUND ( 'NONE', #46692, .T. ) ;
#102368=CARTESIAN_POINT ( 'NONE',  ( 7.392999751807240116, 1426.269867617909995, 212.5881189270220091 ) ) ;
#102370=ORIENTED_EDGE ( 'NONE', *, *, #15100, .T. ) ;
#102372=CARTESIAN_POINT ( 'NONE',  ( -11.11407518912900017, 1492.021456573850173, 207.0665889738719727 ) ) ;
#102374=ADVANCED_FACE ( 'NONE', ( #8312 ), #1686, .T. ) ;
#102377=CARTESIAN_POINT ( 'NONE',  ( 8.075468704329999525, 1426.465554857850066, 211.6438910379590084 ) ) ;
#102399=CARTESIAN_POINT ( 'NONE',  ( 1.022675170609709916, 1445.282598627109792, 199.0986583360879933 ) ) ;
#102405=CARTESIAN_POINT ( 'NONE',  ( -4.836838691967080273, 1508.551704408389924, 212.4671294835000310 ) ) ;
#102407=CARTESIAN_POINT ( 'NONE',  ( 8.190748369970000553, 1421.378881458010255, 196.0919654739990108 ) ) ;
#102408=CARTESIAN_POINT ( 'NONE',  ( -0.5009090896308688867, 1432.030616873689951, 218.6088325375140187 ) ) ;
#102409=CARTESIAN_POINT ( 'NONE',  ( -3.591208274099999986, 1495.697152948690018, 197.7417738467989921 ) ) ;
#102422=CARTESIAN_POINT ( 'NONE',  ( 9.255168820965479881, 1422.794170407699994, 212.0163054975980117 ) ) ;
#102424=CARTESIAN_POINT ( 'NONE',  ( -11.00021946413910001, 1462.586022203469838, 208.1031543993230173 ) ) ;
#102429=CARTESIAN_POINT ( 'NONE',  ( -10.58089751883319884, 1462.237251693409917, 208.9718616002229794 ) ) ;
#102430=CARTESIAN_POINT ( 'NONE',  ( -9.526209128037958607, 1423.233055757800230, 192.3205453756600036 ) ) ;
#102431=CARTESIAN_POINT ( 'NONE',  ( 8.547027738309338929, 1419.998520249890134, 194.9826476886919977 ) ) ;
#102432=CARTESIAN_POINT ( 'NONE',  ( 5.445195913439840218, 1467.322352123520204, 217.4938090916859892 ) ) ;
#102436=CARTESIAN_POINT ( 'NONE',  ( -8.003970385414945099, 1425.916565961161268, 207.5703587753713748 ) ) ;
#102437=CARTESIAN_POINT ( 'NONE',  ( -2.525349509968036088, 1476.996657561013308, 199.0229261902041173 ) ) ;
#102439=CARTESIAN_POINT ( 'NONE',  ( -1.842963895390000273, 1515.551704166990021, 205.1377641647089831 ) ) ;
#102440=CARTESIAN_POINT ( 'NONE',  ( 4.873735476160000246, 1472.089320948289924, 218.0431589096889695 ) ) ;
#102441=CARTESIAN_POINT ( 'NONE',  ( 20.33643746716989753, 1475.138452556609991, 218.0161092331550208 ) ) ;
#102443=CARTESIAN_POINT ( 'NONE',  ( -17.10099446617070029, 1420.024199383779887, 206.1776963727390068 ) ) ;
#102451=CARTESIAN_POINT ( 'NONE',  ( -7.649966233313090669, 1508.551704408389924, 219.0282755267929815 ) ) ;
#102453=CARTESIAN_POINT ( 'NONE',  ( -11.40675845049999992, 1470.736590895890004, 209.2409589557610161 ) ) ;
#102455=CARTESIAN_POINT ( 'NONE',  ( 7.294530591305462330, 1447.438264182228068, 203.6988537847500709 ) ) ;
#102457=CARTESIAN_POINT ( 'NONE',  ( -3.982766651553749870, 1432.979116022980179, 216.7759890233299984 ) ) ;
#102459=CARTESIAN_POINT ( 'NONE',  ( -14.99634941789999942, 1415.350563318459990, 212.7117730710989747 ) ) ;
#102464=CARTESIAN_POINT ( 'NONE',  ( 10.46793285443070154, 1425.962962126699949, 207.8293122372670041 ) ) ;
#102469=CARTESIAN_POINT ( 'NONE',  ( 4.229167303610000594, 1436.983388288790138, 227.1518914930990150 ) ) ;
#102471=CARTESIAN_POINT ( 'NONE',  ( 4.727292513470000124, 1474.107684878189957, 219.5305710966990205 ) ) ;
#102472=CARTESIAN_POINT ( 'NONE',  ( 1.842962214803819831, 1515.372048948338943, 204.8601094092262542 ) ) ;
#102474=CARTESIAN_POINT ( 'NONE',  ( -7.000192180139999998, 1494.404549418689840, 199.4211192133089980 ) ) ;
#102475=EDGE_CURVE ( 'NONE', #25053, #67299, #59590, .T. ) ;
#102479=CARTESIAN_POINT ( 'NONE',  ( 10887.13479812350670, -2340.220200558883789, -7120.152215564383368 ) ) ;
#102480=CARTESIAN_POINT ( 'NONE',  ( 9.326190216649999698, 1450.430212708290128, 205.2552756270490022 ) ) ;
#102502=CARTESIAN_POINT ( 'NONE',  ( -5.081549875360000357, 1391.866816797490173, 214.6180254208989879 ) ) ;
#102504=VERTEX_POINT ( 'NONE', #62072 ) ;
#102506=CARTESIAN_POINT ( 'NONE',  ( -19.15298488520000220, 1464.559837765089924, 213.8319524061190009 ) ) ;
#102511=CARTESIAN_POINT ( 'NONE',  ( 8.380162515710001259, 1425.070964763900065, 194.6834137014990063 ) ) ;
#102513=CARTESIAN_POINT ( 'NONE',  ( -12.19226287358214833, 1417.436307414769544, 199.7077872052550731 ) ) ;
#102514=CARTESIAN_POINT ( 'NONE',  ( 4.091836660730000297, 1515.531866980889845, 210.2412738621790140 ) ) ;
#102515=CARTESIAN_POINT ( 'NONE',  ( -4.591899558935420345, 1455.336696413800155, 200.8800319518429944 ) ) ;
#102518=CARTESIAN_POINT ( 'NONE',  ( 9.707000155197439639, 1452.234455235359974, 209.8042379339860020 ) ) ;
#102524=CARTESIAN_POINT ( 'NONE',  ( 19.13172296059999766, 1454.817774558389829, 206.3490106532590005 ) ) ;
#102526=ORIENTED_EDGE ( 'NONE', *, *, #21997, .T. ) ;
#102529=CARTESIAN_POINT ( 'NONE',  ( -3.430374836980000008, 1431.708658569990121, 216.7924588047190184 ) ) ;
#102530=CARTESIAN_POINT ( 'NONE',  ( -4.368232472647803455, 1488.977261507675621, 219.1147625199656375 ) ) ;
#102532=CARTESIAN_POINT ( 'NONE',  ( 10.87756687473890160, 1470.161469495209985, 206.9927029381979935 ) ) ;
#102533=CARTESIAN_POINT ( 'NONE',  ( -9.218333506580000503, 1473.255740393489759, 204.2345550927689999 ) ) ;
#102534=CARTESIAN_POINT ( 'NONE',  ( 7.031363022279999875, 1494.605019377190047, 219.3119659920989761 ) ) ;
#102538=CARTESIAN_POINT ( 'NONE',  ( -21.68299751200000003, 1505.523879562090087, 209.6298452977370061 ) ) ;
#102547=CARTESIAN_POINT ( 'NONE',  ( 0.08387812437511810160, 1515.158224561690076, 204.7948437802780006 ) ) ;
#102553=CARTESIAN_POINT ( 'NONE',  ( 2.392804902923610033, 1445.901086195959806, 199.3053874824840079 ) ) ;
#102555=CARTESIAN_POINT ( 'NONE',  ( -7.027669101106630123, 1426.313406588260023, 202.9938954506890241 ) ) ;
#102560=CARTESIAN_POINT ( 'NONE',  ( -10.99409911865420142, 1481.669864629989888, 208.2822106822179933 ) ) ;
#102571=CARTESIAN_POINT ( 'NONE',  ( -16.02532890700000223, 1417.348757203270225, 206.0160147869889897 ) ) ;
#102573=CARTESIAN_POINT ( 'NONE',  ( -2.170627987649289992, 1485.611815795640041, 197.4219879416550327 ) ) ;
#102579=CARTESIAN_POINT ( 'NONE',  ( -11.84975450817150033, 1508.199963107450003, 208.6376032033030015 ) ) ;
#102580=CARTESIAN_POINT ( 'NONE',  ( 3.829620113550000315, 1515.051704408389924, 209.0973262533439936 ) ) ;
#102593=CARTESIAN_POINT ( 'NONE',  ( 4.798101961140000427, 1484.634215563789894, 219.1327562436990206 ) ) ;
#102594=CARTESIAN_POINT ( 'NONE',  ( 4.416167311050000599, 1423.572941315969956, 193.9044136913989860 ) ) ;
#102596=CARTESIAN_POINT ( 'NONE',  ( 11.44399576807470176, 1434.340548105539938, 225.7446294064320114 ) ) ;
#102604=CARTESIAN_POINT ( 'NONE',  ( 5.749238445798059871, 1447.708474149499807, 200.6605380239639942 ) ) ;
#102612=CARTESIAN_POINT ( 'NONE',  ( 5.476215863316349797, 1506.245585586920015, 219.4133328000820029 ) ) ;
#102613=VECTOR ( 'NONE', #54495, 1000.000000000000000 ) ;
#102621=CARTESIAN_POINT ( 'NONE',  ( -10.36068074410219886, 1448.206033820939865, 208.6438493282829825 ) ) ;
#102622=DIRECTION ( 'NONE',  ( 0.02616798426500960631, 0.9993150019883682011, 0.02616798426500950570 ) ) ;
#102642=CARTESIAN_POINT ( 'NONE',  ( -8.351543752122086772, 1474.679204586614105, 203.1296262194932467 ) ) ;
#102645=STYLED_ITEM ( 'NONE', ( #22205 ), #9778 ) ;
#102658=VERTEX_POINT ( 'NONE', #61515 ) ;
#102660=CARTESIAN_POINT ( 'NONE',  ( -13.70184035893560015, 1508.551704408389924, 210.3434241671160123 ) ) ;
#102664=B_SPLINE_SURFACE_WITH_KNOTS ( 'NONE', 5, 1, ( 
 ( #4087, #12995 ),
 ( #29267, #90258 ),
 ( #71318, #47178 ),
 ( #13541, #64000 ),
 ( #28166, #98111 ),
 ( #88093, #38211 ),
 ( #81859, #21386 ),
 ( #47726, #63459 ),
 ( #73489, #4623 ),
 ( #5160, #11380 ),
 ( #55595, #45552 ),
 ( #72932, #62354 ),
 ( #79692, #2997 ),
 ( #37118, #107072 ),
 ( #105432, #105991 ),
 ( #20849, #28721 ),
 ( #89718, #62927 ),
 ( #54505, #20301 ),
 ( #11918, #46096 ),
 ( #80227, #37670 ),
 ( #97578, #55045 ),
 ( #89172, #12463 ),
 ( #58331, #67297 ),
 ( #6801, #101389 ),
 ( #24684, #84612 ),
 ( #40961, #108167 ),
 ( #75140, #49380 ),
 ( #33108, #41528 ),
 ( #15727, #109288 ),
 ( #39869, #82968 ),
 ( #22479, #65086 ),
 ( #32573, #31458 ),
 ( #66748, #57251 ),
 ( #74587, #30908 ),
 ( #48286, #92456 ),
 ( #74035, #65638 ),
 ( #66202, #49928 ),
 ( #84065, #14097 ),
 ( #7905, #99754 ),
 ( #99200, #100851 ),
 ( #107625, #23044 ),
 ( #91378, #93012 ),
 ( #56679, #100322 ),
 ( #83507, #109827 ),
 ( #24141, #48845 ),
 ( #6262, #7363 ),
 ( #40410, #90815 ),
 ( #82430, #75686 ),
 ( #5726, #14657 ),
 ( #108723, #32013 ),
 ( #23606, #57794 ) ),
 .UNSPECIFIED., .F., .F., .F.,
 ( 6, 3, 3, 3, 3, 3, 3, 3, 3, 3, 3, 3, 3, 3, 3, 3, 6 ),
 ( 2, 2 ),
 ( 0.000000000000000000, 28.69702819429999963, 61.04778752440000034, 93.62768910810000023, 123.7336603250000024, 156.1762685979999787, 187.3272846180000215, 220.4669312460000015, 237.3878297990000021, 254.2938300590000154, 289.2398204710000300, 325.3030936050000150, 360.8626869010000178, 395.8828220460000011, 432.6128460950000090, 468.8934854820000169, 502.1482307969999965 ),
 ( -1.776356839400000001E-15, 2.001751835784610023 ),
 .UNSPECIFIED. ) ;
#102666=CARTESIAN_POINT ( 'NONE',  ( -3.247779998094530107, 1428.782300086839996, 200.3378027425290213 ) ) ;
#102671=EDGE_CURVE ( 'NONE', #2310, #23969, #43518, .T. ) ;
#102682=CARTESIAN_POINT ( 'NONE',  ( -2.409034624560000282, 1511.999350511789999, 206.7128113371389873 ) ) ;
#102688=CARTESIAN_POINT ( 'NONE',  ( -9.936111480414750119, 1448.113236486630058, 209.3298349216750012 ) ) ;
#102696=CARTESIAN_POINT ( 'NONE',  ( -13.59512407998240135, 1507.703338069740084, 209.3532897553030239 ) ) ;
#102698=CARTESIAN_POINT ( 'NONE',  ( 3.409085372019999838, 1467.742650992889821, 218.4995240695689915 ) ) ;
#102699=CARTESIAN_POINT ( 'NONE',  ( -1.431952011063330366, 1469.731770489434439, 219.0844453393653168 ) ) ;
#102703=CARTESIAN_POINT ( 'NONE',  ( -1.785930250549999876, 1430.082233120889896, 200.6040445722289860 ) ) ;
#102707=CARTESIAN_POINT ( 'NONE',  ( -1.892509460324644843, 1445.288012513316517, 217.9545851404853352 ) ) ;
#102715=CARTESIAN_POINT ( 'NONE',  ( 5.662343758720000508, 1504.894618425089902, 220.5557215505990314 ) ) ;
#102719=CARTESIAN_POINT ( 'NONE',  ( 7.786809421259999198, 1425.366053415200213, 211.4289136434089755 ) ) ;
#102723=CARTESIAN_POINT ( 'NONE',  ( -6.356619906689999766, 1483.629449051089978, 200.3071127286890203 ) ) ;
#102726=ORIENTED_EDGE ( 'NONE', *, *, #25079, .F. ) ;
#102732=DIRECTION ( 'NONE',  ( 1.149679124779773953E-17, 1.000000000000000000, -1.829746454213089849E-16 ) ) ;
#102733=CARTESIAN_POINT ( 'NONE',  ( -15.24330594657070748, 1416.048311171039131, 206.3693755384788062 ) ) ;
#102735=CARTESIAN_POINT ( 'NONE',  ( -3.179033943583710276, 1457.997354099609993, 219.3203918230290128 ) ) ;
#102739=CARTESIAN_POINT ( 'NONE',  ( 7.901854723500001398, 1423.732064818020035, 212.4548200391890020 ) ) ;
#102740=CARTESIAN_POINT ( 'NONE',  ( 20.81805062950000362, 1457.016307409189949, 206.8942079858889826 ) ) ;
#102763=CARTESIAN_POINT ( 'NONE',  ( 3.074703527060000052, 1441.333178254290033, 218.5515148082390056 ) ) ;
#102769=ADVANCED_FACE ( 'NONE', ( #52183 ), #86585, .T. ) ;
#102777=B_SPLINE_SURFACE_WITH_KNOTS ( 'NONE', 5, 5, ( 
 ( #57055, #108534, #91181, #57611, #74409, #41339 ),
 ( #4966, #14461, #66012, #58149, #81660, #82228 ),
 ( #32917, #100671, #82780, #73289, #23953, #67108 ),
 ( #30721, #48654, #56494, #109104, #39683, #6073 ),
 ( #99014, #90623, #73850, #40226, #83878, #7182 ),
 ( #109642, #107425, #31824, #100133, #64906, #23418 ) ),
 .UNSPECIFIED., .F., .F., .F.,
 ( 6, 6 ),
 ( 6, 6 ),
 ( 5.893388375696040349, 9.819929736123960140 ),
 ( 0.000000000000000000, 0.5002947206939659663 ),
 .UNSPECIFIED. ) ;
#102784=B_SPLINE_SURFACE_WITH_KNOTS ( 'NONE', 5, 5, ( 
 ( #74549, #6762, #75102, #59408, #33069, #31972 ),
 ( #100285, #51539, #67258, #15688, #34178, #83467 ),
 ( #109790, #101351, #57759, #68364, #85674, #49341 ),
 ( #7327, #40368, #24642, #66164, #91878, #102471 ),
 ( #41491, #109250, #40923, #92975, #23565, #58840 ),
 ( #32534, #85124, #108682, #16249, #67803, #100814 ),
 ( #49894, #50452, #8412, #17344, #84027, #93519 ),
 ( #76736, #76187, #110335, #75651, #7869, #101912 ),
 ( #42036, #25204, #16790, #50994, #42584, #25760 ) ),
 .UNSPECIFIED., .F., .F., .F.,
 ( 6, 3, 6 ),
 ( 6, 6 ),
 ( 0.000000000000000000, 3.343413285960000092, 6.686826571920000184 ),
 ( 0.000000000000000000, 2.000000000000000000 ),
 .UNSPECIFIED. ) ;
#102802=ORIENTED_EDGE ( 'NONE', *, *, #61954, .F. ) ;
#102809=CARTESIAN_POINT ( 'NONE',  ( -3.600510465689999773, 1428.725171273389833, 200.8945958432190082 ) ) ;
#102832=CARTESIAN_POINT ( 'NONE',  ( 3.279449832749999683, 1443.043429850790062, 217.3931667607889722 ) ) ;
#102834=CARTESIAN_POINT ( 'NONE',  ( 762.4595027433168752, -8387.357407334287927, 2038.119698773175060 ) ) ;
#102836=CARTESIAN_POINT ( 'NONE',  ( 11.59735442540000072, 1491.204275857490074, 206.7872505231089804 ) ) ;
#102837=CARTESIAN_POINT ( 'NONE',  ( 9.990308914500090509, 1460.215773286300191, 206.0069800743260089 ) ) ;
#102840=CARTESIAN_POINT ( 'NONE',  ( -13.82563399418980055, 1416.641875147470046, 202.2508794157299974 ) ) ;
#102844=CARTESIAN_POINT ( 'NONE',  ( -7.716404340140000429, 1508.514490008389885, 219.3175259690989947 ) ) ;
#102849=CARTESIAN_POINT ( 'NONE',  ( 762.4595027417112760, -8387.357407334286108, 2038.119698773842174 ) ) ;
#102853=CARTESIAN_POINT ( 'NONE',  ( -3.139465476176170000, 1486.898214819829946, 220.2800545222459903 ) ) ;
#102854=CARTESIAN_POINT ( 'NONE',  ( -19.04699134789089854, 1444.155793973100117, 199.5979840530640104 ) ) ;
#102858=CARTESIAN_POINT ( 'NONE',  ( -9.037727763111515600, 1438.144578922800520, 210.5737952941265689 ) ) ;
#102864=CARTESIAN_POINT ( 'NONE',  ( 8.402537688823850104, 1436.678101434069958, 207.1924150616570159 ) ) ;
#102868=CARTESIAN_POINT ( 'NONE',  ( -8.895525269423981030, 1462.225683208909913, 227.1187923881540200 ) ) ;
#102872=CARTESIAN_POINT ( 'NONE',  ( 9.788533930052889076, 1435.243776026920159, 208.4605043225519694 ) ) ;
#102877=CARTESIAN_POINT ( 'NONE',  ( 1.792759577082169820, 1486.608927711839897, 197.3295603274380028 ) ) ;
#102879=CARTESIAN_POINT ( 'NONE',  ( 8.534303549887848561, 1434.919570507270009, 206.3689778209339920 ) ) ;
#102880=CARTESIAN_POINT ( 'NONE',  ( -12.88231326090629913, 1422.424595942170072, 203.9020998089539773 ) ) ;
#102885=CARTESIAN_POINT ( 'NONE',  ( -4.705754339071280157, 1479.984670612119771, 230.9466448169910109 ) ) ;
#102891=CARTESIAN_POINT ( 'NONE',  ( -12.78956172709999883, 1502.763085786289821, 208.8827437375920226 ) ) ;
#102894=CARTESIAN_POINT ( 'NONE',  ( 0.3230418169460009814, 1476.414103484889893, 198.3680131446989776 ) ) ;
#102906=CARTESIAN_POINT ( 'NONE',  ( -2.496647090823195470, 1469.968832673554289, 218.9194591004516042 ) ) ;
#102907=CARTESIAN_POINT ( 'NONE',  ( 7.525900132721149660, 1425.843575467760047, 212.2409298998749989 ) ) ;
#102916=CARTESIAN_POINT ( 'NONE',  ( -2.919023784219999751, 1461.299471294090154, 228.5190642125989768 ) ) ;
#102917=FACE_OUTER_BOUND ( 'NONE', #18841, .T. ) ;
#102918=ORIENTED_EDGE ( 'NONE', *, *, #11862, .T. ) ;
#102922=CARTESIAN_POINT ( 'NONE',  ( 8.159145002205340447, 1435.857859259829866, 206.4447587482620179 ) ) ;
#102935=CARTESIAN_POINT ( 'NONE',  ( -3.812371265849999968, 1428.459941732490051, 200.5740418003289847 ) ) ;
#102945=CARTESIAN_POINT ( 'NONE',  ( -4.271224532677689645, 1508.551704408389924, 213.3620110914459929 ) ) ;
#102950=LINE ( 'NONE', #35215, #93083 ) ;
#102963=CARTESIAN_POINT ( 'NONE',  ( -9.052602208344991297, 1483.887799354419940, 201.3830137227830051 ) ) ;
#102965=AXIS2_PLACEMENT_3D ( 'NONE', #31015, #84721, #42187 ) ;
#102967=CARTESIAN_POINT ( 'NONE',  ( 8.904193304007050003, 1426.574205491320299, 210.6754700860900016 ) ) ;
#102968=CARTESIAN_POINT ( 'NONE',  ( 1.208874843759933038, 1421.371554683040586, 193.7626136730214625 ) ) ;
#102969=CARTESIAN_POINT ( 'NONE',  ( -4.327725855061320459, 1515.130588580269887, 208.4066028149230192 ) ) ;
#102976=CARTESIAN_POINT ( 'NONE',  ( 18.38166525818579800, 1428.164269971480053, 201.4944236828210080 ) ) ;
#102977=CARTESIAN_POINT ( 'NONE',  ( 10.23386993751040031, 1423.173846909970280, 200.2029385363399854 ) ) ;
#102983=CARTESIAN_POINT ( 'NONE',  ( -8.092407232544459816, 1425.062004142523392, 209.6995862100099828 ) ) ;
#102986=CARTESIAN_POINT ( 'NONE',  ( -1.460285906039999970, 1515.203804957989860, 204.7960373641490150 ) ) ;
#102989=CARTESIAN_POINT ( 'NONE',  ( 20.81805065521579934, 1457.016308257720084, 206.8942077970259845 ) ) ;
#102992=CARTESIAN_POINT ( 'NONE',  ( -20.36506032882270034, 1418.448525618100120, 208.7072595077149799 ) ) ;
#102994=CARTESIAN_POINT ( 'NONE',  ( 4.987363902569999397, 1436.241616658689964, 206.8881657827189997 ) ) ;
#103000=CARTESIAN_POINT ( 'NONE',  ( -17.51542736287469992, 1417.552205557379921, 206.7802911192910358 ) ) ;
#103002=CARTESIAN_POINT ( 'NONE',  ( -10.19876720080000077, 1472.745415185489946, 209.0901046235979948 ) ) ;
#103004=CARTESIAN_POINT ( 'NONE',  ( 6.037737136446180486, 1446.437918506160258, 202.3744026597657069 ) ) ;
#103006=CARTESIAN_POINT ( 'NONE',  ( -3.220366543789920488, 1433.265472343769943, 218.1215055313249991 ) ) ;
#103019=CARTESIAN_POINT ( 'NONE',  ( 6.595526062923129373, 1466.717679795370032, 216.5467274825269897 ) ) ;
#103023=CARTESIAN_POINT ( 'NONE',  ( -6.349572003580000512, 1494.536298393890092, 198.5213465523989953 ) ) ;
#103027=CARTESIAN_POINT ( 'NONE',  ( 2.220446049249999755E-16, 1516.051704408390151, 209.1218459616989946 ) ) ;
#103040=ORIENTED_EDGE ( 'NONE', *, *, #50748, .F. ) ;
#103052=CARTESIAN_POINT ( 'NONE',  ( 4.822058355276690023, 1508.551704408389924, 212.5065985955260146 ) ) ;
#103057=CARTESIAN_POINT ( 'NONE',  ( 10.07185917612419956, 1460.294335048200082, 206.2511351615570163 ) ) ;
#103066=CARTESIAN_POINT ( 'NONE',  ( -9.958774778861073429, 1418.280608540457479, 197.3728175944318082 ) ) ;
#103070=CARTESIAN_POINT ( 'NONE',  ( 10.12770055993100016, 1452.320269254320010, 209.2677959960770124 ) ) ;
#103082=CARTESIAN_POINT ( 'NONE',  ( -5.938778458005980809, 1508.471255113249981, 219.9128644399360155 ) ) ;
#103084=FACE_OUTER_BOUND ( 'NONE', #7948, .T. ) ;
#103093=CARTESIAN_POINT ( 'NONE',  ( 8.986732482983370573, 1468.575268126999845, 202.3908276555110035 ) ) ;
#103096=CARTESIAN_POINT ( 'NONE',  ( -2.975022846544269850, 1495.689959026299903, 216.9727101957990101 ) ) ;
#103097=EDGE_LOOP ( 'NONE', ( #3161, #26648, #20177, #57851 ) ) ;
#103103=CARTESIAN_POINT ( 'NONE',  ( -14.93718008229999938, 1416.181292664740113, 212.9156384192889959 ) ) ;
#103104=CARTESIAN_POINT ( 'NONE',  ( -0.05006135368913040146, 1515.158685764440179, 204.7948558572980176 ) ) ;
#103106=B_SPLINE_CURVE_WITH_KNOTS ( 'NONE', 5,
 ( #68142, #102252, #94970, #44023, #59181, #35604 ),
 .UNSPECIFIED., .F., .F.,
 ( 6, 6 ),
 ( -1.999999977866010026, 0.000000000000000000 ),
 .UNSPECIFIED. ) ;
#103111=CARTESIAN_POINT ( 'NONE',  ( -11.03761941066989927, 1462.381893958199953, 208.9991076938630101 ) ) ;
#103112=CARTESIAN_POINT ( 'NONE',  ( -4.992349863779999453, 1391.620913471789891, 203.8075142969990168 ) ) ;
#103113=CARTESIAN_POINT ( 'NONE',  ( -1.073363620209200085E-15, 1380.371560387289946, 209.1218459616989946 ) ) ;
#103115=FACE_OUTER_BOUND ( 'NONE', #258, .T. ) ;
#103117=CARTESIAN_POINT ( 'NONE',  ( -10.97550978995469961, 1481.752618510480033, 208.0127154857229925 ) ) ;
#103125=CARTESIAN_POINT ( 'NONE',  ( -11.42085373761049993, 1500.664288095930033, 209.5050427075310040 ) ) ;
#103129=CARTESIAN_POINT ( 'NONE',  ( -15.89469460119999766, 1416.172609518619993, 209.1989024842829963 ) ) ;
#103133=CARTESIAN_POINT ( 'NONE',  ( -3.619842073959999684, 1497.142537609690180, 220.5541519757989875 ) ) ;
#103139=AXIS2_PLACEMENT_3D ( 'NONE', #37717, #104925, #46148 ) ;
#103141=CARTESIAN_POINT ( 'NONE',  ( -18.48166340339999891, 1443.454462795790050, 212.6921494033990143 ) ) ;
#103153=CARTESIAN_POINT ( 'NONE',  ( 4.566741015489999889, 1485.595084333989917, 218.8629924376189990 ) ) ;
#103157=CARTESIAN_POINT ( 'NONE',  ( -17.63206642429129900, 1440.541090996499861, 218.8715579270100022 ) ) ;
#103159=CARTESIAN_POINT ( 'NONE',  ( 13.84584237522359906, 1499.900173460709766, 227.7510556141490099 ) ) ;
#103163=CARTESIAN_POINT ( 'NONE',  ( 9.821586882074960556, 1435.575910505290040, 209.2747408604490147 ) ) ;
#103164=CARTESIAN_POINT ( 'NONE',  ( -11.06280732299999947, 1490.126969804790178, 211.8519967247989939 ) ) ;
#103165=CARTESIAN_POINT ( 'NONE',  ( 8.748194321763609338, 1449.742677337359737, 203.5399419409159805 ) ) ;
#103168=CARTESIAN_POINT ( 'NONE',  ( 5.009886284249999377, 1430.069699660889910, 217.1776678749689893 ) ) ;
#103181=CARTESIAN_POINT ( 'NONE',  ( -10.36694999858590016, 1448.084678120760145, 208.9249857694410082 ) ) ;
#103187=CARTESIAN_POINT ( 'NONE',  ( 2.727465513059999846, 1467.148923109990164, 219.0926697488289960 ) ) ;
#103188=LINE ( 'NONE', #43323, #59071 ) ;
#103195=CARTESIAN_POINT ( 'NONE',  ( -0.4182119524568259639, 1432.129988308659904, 200.7098003538619935 ) ) ;
#103196=EDGE_LOOP ( 'NONE', ( #56678, #28516, #101666, #28988 ) ) ;
#103203=CARTESIAN_POINT ( 'NONE',  ( 1.846216073831150162, 1465.868771192480153, 198.2512937515799933 ) ) ;
#103204=CARTESIAN_POINT ( 'NONE',  ( 11.79334844382369951, 1421.931009736009855, 209.2876916042509947 ) ) ;
#103206=CARTESIAN_POINT ( 'NONE',  ( 2.435277524900000046, 1464.768429074390042, 199.5670726285990213 ) ) ;
#103217=VERTEX_POINT ( 'NONE', #30934 ) ;
#103219=CARTESIAN_POINT ( 'NONE',  ( -16.45376569770029818, 1508.551704408389924, 210.3850702157819796 ) ) ;
#103220=CARTESIAN_POINT ( 'NONE',  ( 5.597778194180000888, 1506.679269386989972, 219.3685102149989916 ) ) ;
#103224=AXIS2_PLACEMENT_3D ( 'NONE', #81509, #72590, #13197 ) ;
#103226=CARTESIAN_POINT ( 'NONE',  ( 2.782344708190000127, 1462.431012131489751, 228.5889832501989929 ) ) ;
#103231=CARTESIAN_POINT ( 'NONE',  ( -11.87206752526750009, 1482.026096006810121, 208.5610132530620149 ) ) ;
#103234=ORIENTED_EDGE ( 'NONE', *, *, #24188, .T. ) ;
#103238=CYLINDRICAL_SURFACE ( 'NONE', #21735, 2.000000000000007550 ) ;
#103240=CARTESIAN_POINT ( 'NONE',  ( 7.311826422820000282, 1422.546741514869836, 195.5507102769989842 ) ) ;
#103251=FACE_OUTER_BOUND ( 'NONE', #69394, .T. ) ;
#103253=CARTESIAN_POINT ( 'NONE',  ( 3.266177458080000040, 1467.802312483090191, 218.5517732847689842 ) ) ;
#103254=CARTESIAN_POINT ( 'NONE',  ( 0.08449630495836644994, 1469.347514019179016, 219.1765324506605452 ) ) ;
#103259=CARTESIAN_POINT ( 'NONE',  ( 8.381577504150859781, 1438.875682636792817, 211.6325970076460976 ) ) ;
#103262=VERTEX_POINT ( 'NONE', #63484 ) ;
#103264=CARTESIAN_POINT ( 'NONE',  ( 3.860559482726539926, 1456.030320310470188, 219.0185799711049981 ) ) ;
#103268=CARTESIAN_POINT ( 'NONE',  ( 12.25846076559999887, 1500.678402377489874, 208.9469212626399894 ) ) ;
#103272=CARTESIAN_POINT ( 'NONE',  ( 8.911818219449999745, 1428.279464179490105, 213.0373091593789923 ) ) ;
#103275=B_SPLINE_CURVE_WITH_KNOTS ( 'NONE', 3,
 ( #7725, #8267, #76590, #102329, #16647, #110741, #100674, #68223, #92832, #110188, #58152, #25615, #75511, #16108, #51390, #109645, #59807, #23957, #41886, #76044, #93926, #57614, #85522, #462, #8817 ),
 .UNSPECIFIED., .F., .F.,
 ( 4, 3, 3, 3, 3, 3, 3, 3, 4 ),
 ( -7.690123547477719868, -7.578754016464039900, -6.856148510135199992, -6.131423372794370330, -5.422190055320710300, -5.213236018046780273, -4.581108567758639616, -3.740027080196560050, -3.154256035599999564 ),
 .UNSPECIFIED. ) ;
#103278=CARTESIAN_POINT ( 'NONE',  ( -8.719918377449999980, 1483.750365165289850, 201.5181060481390034 ) ) ;
#103289=CARTESIAN_POINT ( 'NONE',  ( -0.8560893484002659592, 1457.237409688020080, 219.7250069795780121 ) ) ;
#103294=CARTESIAN_POINT ( 'NONE',  ( 7.944350852719999523, 1425.480812533560083, 211.5441705370589887 ) ) ;
#103295=CARTESIAN_POINT ( 'NONE',  ( -9.104803454449999833, 1421.479062531979935, 192.1853131694989827 ) ) ;
#103309=DIRECTION ( 'NONE',  ( -1.000000000000000000, -2.249639673992789970E-32, -1.224646799147350002E-16 ) ) ;
#103311=CARTESIAN_POINT ( 'NONE',  ( -1.474640905272780023, 1475.430171080190121, 197.7716959656699771 ) ) ;
#103330=B_SPLINE_SURFACE_WITH_KNOTS ( 'NONE', 5, 5, ( 
 ( #32583, #100859, #24150, #110381, #58340, #33660 ),
 ( #8459, #49936, #92464, #42633, #7373, #84075 ),
 ( #41537, #67305, #25805, #24693, #102514, #91389 ),
 ( #48855, #66213, #50498, #58888, #85174, #93564 ),
 ( #84620, #7914, #76784, #68410, #42086, #67852 ),
 ( #101965, #102, #82979, #25251, #16838, #59454 ) ),
 .UNSPECIFIED., .F., .F., .F.,
 ( 6, 6 ),
 ( 6, 6 ),
 ( 2.324858856890000158, 4.991117563570000470 ),
 ( 0.000000000000000000, 0.5000000000000000000 ),
 .UNSPECIFIED. ) ;
#103341=ADVANCED_FACE ( 'NONE', ( #60017 ), #46389, .F. ) ;
#103349=CARTESIAN_POINT ( 'NONE',  ( 10.67217592544739979, 1460.316194025420145, 206.8193158878239899 ) ) ;
#103351=VECTOR ( 'NONE', #17453, 1000.000000000000114 ) ;
#103354=CARTESIAN_POINT ( 'NONE',  ( -18.79700370569999635, 1444.661305230889866, 207.2600034499489823 ) ) ;
#103361=ORIENTED_EDGE ( 'NONE', *, *, #94752, .T. ) ;
#103369=CARTESIAN_POINT ( 'NONE',  ( 4.414758600232289609, 1430.295245474100057, 217.5194609254549789 ) ) ;
#103372=CARTESIAN_POINT ( 'NONE',  ( 11.13187122630000125, 1480.405616529990084, 211.3597187323589992 ) ) ;
#103383=CARTESIAN_POINT ( 'NONE',  ( 2.839373935849999864, 1442.324148150689780, 217.6523810350290091 ) ) ;
#103387=CARTESIAN_POINT ( 'NONE',  ( 10.79356334649999916, 1490.085259999289974, 207.2636451086090119 ) ) ;
#103388=CARTESIAN_POINT ( 'NONE',  ( 10.04317694198510047, 1459.686705811340062, 204.8127587182970046 ) ) ;
#103391=CARTESIAN_POINT ( 'NONE',  ( -2.472534047699199711, 1422.360495435749954, 192.6709246226909613 ) ) ;
#103403=CARTESIAN_POINT ( 'NONE',  ( -10.45767044947240088, 1479.639629119470101, 210.0294207369939841 ) ) ;
#103405=CARTESIAN_POINT ( 'NONE',  ( -11.11783079367559957, 1470.257259110569976, 211.5455878590279895 ) ) ;
#103407=CARTESIAN_POINT ( 'NONE',  ( -2.193888375216459963, 1486.670272915489932, 220.4458273536270099 ) ) ;
#103415=ORIENTED_EDGE ( 'NONE', *, *, #7683, .F. ) ;
#103427=CARTESIAN_POINT ( 'NONE',  ( 9.808562800256929393, 1435.340065754910029, 208.7021925875509964 ) ) ;
#103440=ORIENTED_EDGE ( 'NONE', *, *, #15331, .T. ) ;
#103441=CARTESIAN_POINT ( 'NONE',  ( -11.59117397610000033, 1507.247540214189939, 207.5195457387889917 ) ) ;
#103443=CARTESIAN_POINT ( 'NONE',  ( 10.95119923923629912, 1479.297566038250125, 229.8393126471409857 ) ) ;
#103451=CARTESIAN_POINT ( 'NONE',  ( -2.075457432642690225, 1421.202448102600101, 193.7464090391210334 ) ) ;
#103459=CARTESIAN_POINT ( 'NONE',  ( -8.218152191339997970, 1424.217405426100186, 209.2885718405189834 ) ) ;
#103465=CARTESIAN_POINT ( 'NONE',  ( 7.536552308397739708, 1425.565060507700082, 212.1829400242899624 ) ) ;
#103474=CARTESIAN_POINT ( 'NONE',  ( -19.09919624993290199, 1508.457687219779928, 210.0040316747289921 ) ) ;
#103475=CARTESIAN_POINT ( 'NONE',  ( 0.004157115712379180240, 1455.132373369690185, 215.8075664961990014 ) ) ;
#103476=EDGE_CURVE ( 'NONE', #51303, #57781, #36762, .T. ) ;
#103477=CARTESIAN_POINT ( 'NONE',  ( -9.235583105570428941, 1440.105707546520080, 206.5655124634290303 ) ) ;
#103505=EDGE_LOOP ( 'NONE', ( #84488, #6553, #47361, #34198 ) ) ;
#103506=CARTESIAN_POINT ( 'NONE',  ( 4.833436873729850092, 1508.551704408090018, 205.8972860377909910 ) ) ;
#103508=CARTESIAN_POINT ( 'NONE',  ( -2.716551984532820097, 1508.551704408389924, 214.0984450385660125 ) ) ;
#103520=CARTESIAN_POINT ( 'NONE',  ( 5.277460848200000498, 1426.742654866309977, 191.8370381630989812 ) ) ;
#103527=ADVANCED_FACE ( 'NONE', ( #97457 ), #51723, .T. ) ;
#103530=B_SPLINE_CURVE_WITH_KNOTS ( 'NONE', 3,
 ( #93723, #103231, #17001, #25970, #59066, #33837, #86453, #60168, #68027, #35501, #69693, #17564, #26541, #60736, #18132, #9744, #61297, #51765, #95416, #52877, #87004, #10294, #16457, #8627, #44470, #51200, #42802, #70253, #27657, #55639, #11421, #45590, #104360, #45038, #54001, #80274, #36607, #106566, #71914, #64039 ),
 .UNSPECIFIED., .F., .F.,
 ( 4, 3, 3, 3, 3, 3, 3, 3, 3, 3, 3, 3, 3, 4 ),
 ( -7.724159284985280038, -7.528912261385430682, -7.285801190272390038, -7.022071646754660001, -6.736975261711270591, -6.407913920619930259, -6.017318246991619546, -5.710627735595419807, -5.447746533992479989, -5.114105914177909717, -4.732608650904720271, -4.279348212383050409, -3.608572623993069328, -3.171332707879999546 ),
 .UNSPECIFIED. ) ;
#103532=CARTESIAN_POINT ( 'NONE',  ( -4.327610416712750485, 1515.134996992939932, 208.4730697464140121 ) ) ;
#103538=CARTESIAN_POINT ( 'NONE',  ( -10.57409850134300022, 1462.298722268380061, 208.7176379312979861 ) ) ;
#103539=CARTESIAN_POINT ( 'NONE',  ( -14.46118808569999814, 1422.533245244620048, 196.3519510282989984 ) ) ;
#103540=B_SPLINE_CURVE_WITH_KNOTS ( 'NONE', 5,
 ( #68791, #33480, #102891, #17215, #58716, #101228, #23974, #101790, #67128 ),
 .UNSPECIFIED., .F., .F.,
 ( 6, 3, 6 ),
 ( 0.000000000000000000, 0.3910644012100996103, 1.000000000000000000 ),
 .UNSPECIFIED. ) ;
#103541=CARTESIAN_POINT ( 'NONE',  ( 11.73977902011290020, 1420.726571890000287, 199.9640281710840100 ) ) ;
#103551=CARTESIAN_POINT ( 'NONE',  ( -1.842963640640000067, 1515.372048646890107, 204.8601094037989867 ) ) ;
#103552=CARTESIAN_POINT ( 'NONE',  ( 13.84583159390490081, 1499.900107518399864, 227.7510596827030156 ) ) ;
#103554=CARTESIAN_POINT ( 'NONE',  ( -18.18415092269999889, 1419.305676067660215, 210.3674448266889954 ) ) ;
#103557=ORIENTED_EDGE ( 'NONE', *, *, #48711, .T. ) ;
#103560=EDGE_CURVE ( 'NONE', #88662, #23187, #64208, .T. ) ;
#103565=CARTESIAN_POINT ( 'NONE',  ( -6.670684733933529564, 1508.551704408180058, 219.2717039139770066 ) ) ;
#103572=ADVANCED_FACE ( 'NONE', ( #7795 ), #74897, .T. ) ;
#103573=CARTESIAN_POINT ( 'NONE',  ( 9.093901123017769095, 1470.494570018200193, 191.1297851741429952 ) ) ;
#103574=CARTESIAN_POINT ( 'NONE',  ( -2.608414268140000214, 1431.710115199490019, 217.1231005886490095 ) ) ;
#103575=CARTESIAN_POINT ( 'NONE',  ( -16.25511663789999872, 1421.255025725300129, 210.0327608240260133 ) ) ;
#103586=CARTESIAN_POINT ( 'NONE',  ( 7.653407898138279819, 1466.072686860559998, 215.4064835335099986 ) ) ;
#103588=ORIENTED_EDGE ( 'NONE', *, *, #13773, .F. ) ;
#103592=CARTESIAN_POINT ( 'NONE',  ( -9.624884241989999367, 1493.132688955090089, 201.2649490877390122 ) ) ;
#103602=CARTESIAN_POINT ( 'NONE',  ( 0.8541212061450009774, 1457.065338652990249, 199.5100658954889923 ) ) ;
#103603=EDGE_CURVE ( 'NONE', #3002, #19377, #98237, .T. ) ;
#103609=CARTESIAN_POINT ( 'NONE',  ( -2.897049938759999943, 1495.303674484390058, 219.9350255916990022 ) ) ;
#103625=CARTESIAN_POINT ( 'NONE',  ( -5.024579074340000062, 1391.800828779589892, 214.6319658655289970 ) ) ;
#103629=CARTESIAN_POINT ( 'NONE',  ( 10.14559180641809988, 1460.375376629410084, 206.4970471914819825 ) ) ;
#103634=CARTESIAN_POINT ( 'NONE',  ( -14.47420009890000081, 1416.181292664740113, 214.4142689833190047 ) ) ;
#103635=CARTESIAN_POINT ( 'NONE',  ( 9.228474993260000758, 1423.651513103620118, 196.7592343168990112 ) ) ;
#103638=CARTESIAN_POINT ( 'NONE',  ( -13.98359605274442785, 1416.534589811554270, 202.6245575613080803 ) ) ;
#103640=CARTESIAN_POINT ( 'NONE',  ( -2.664535259099999805E-15, 1424.786834349990158, 209.1218459616989946 ) ) ;
#103643=CARTESIAN_POINT ( 'NONE',  ( 9.549813427814630273, 1451.221866577720220, 207.5450308176739895 ) ) ;
#103660=CARTESIAN_POINT ( 'NONE',  ( 1.959285284397550120, 1474.800623515119923, 220.3715842348549927 ) ) ;
#103662=CARTESIAN_POINT ( 'NONE',  ( 11.86100295819999850, 1492.894947675889853, 212.5846962613990172 ) ) ;
#103664=CARTESIAN_POINT ( 'NONE',  ( 8.943454933915715444, 1425.008260442055644, 195.6459240983384973 ) ) ;
#103665=CARTESIAN_POINT ( 'NONE',  ( -21.20078141540000161, 1505.634983266090103, 209.1959435100580151 ) ) ;
#103666=CARTESIAN_POINT ( 'NONE',  ( 11.08318464053740016, 1470.184830858459918, 206.6635668760160058 ) ) ;
#103670=VERTEX_POINT ( 'NONE', #64854 ) ;
#103676=CARTESIAN_POINT ( 'NONE',  ( -14.10889964140000075, 1415.677402202029953, 213.9573798837890308 ) ) ;
#103677=CARTESIAN_POINT ( 'NONE',  ( 1.059358656784129993, 1515.104045403560121, 204.7934250490989996 ) ) ;
#103679=CARTESIAN_POINT ( 'NONE',  ( -15.87663024991563532, 1415.942772094044130, 209.7336067992691824 ) ) ;
#103680=CARTESIAN_POINT ( 'NONE',  ( 20.21057157959999984, 1475.708668719390062, 208.1550663298600057 ) ) ;
#103683=CARTESIAN_POINT ( 'NONE',  ( 3.375977085881459949, 1446.395221913229989, 199.5681764770490076 ) ) ;
#103688=CARTESIAN_POINT ( 'NONE',  ( -8.070165105480000989, 1477.963585978789752, 216.1585797569989893 ) ) ;
#103690=CIRCLE ( 'NONE', #82178, 14.91144628110000170 ) ;
#103697=CARTESIAN_POINT ( 'NONE',  ( -11.42922335629970121, 1500.819224854980121, 209.0445494102119994 ) ) ;
#103700=CARTESIAN_POINT ( 'NONE',  ( -16.80685858420000045, 1416.624127770589894, 209.3044896098560059 ) ) ;
#103701=VECTOR ( 'NONE', #55727, 1000.000000000000000 ) ;
#103705=DIRECTION ( 'NONE',  ( -0.4229618813980365877, 0.9061474752402244315, -4.354426617128452806E-10 ) ) ;
#103706=VERTEX_POINT ( 'NONE', #106276 ) ;
#103722=CARTESIAN_POINT ( 'NONE',  ( -10.94209231895430179, 1492.979988125699947, 207.3926202358989883 ) ) ;
#103723=CARTESIAN_POINT ( 'NONE',  ( 4.015743051850000356, 1515.588776726489868, 208.3686727890390102 ) ) ;
#103728=CARTESIAN_POINT ( 'NONE',  ( 4.875860680149999737, 1485.457236370389865, 218.7044629644089753 ) ) ;
#103730=CARTESIAN_POINT ( 'NONE',  ( 10.92993424403990055, 1479.841764369919929, 208.5741803220239774 ) ) ;
#103734=CARTESIAN_POINT ( 'NONE',  ( 18.92795655249999953, 1456.152682707289841, 200.2564363106190228 ) ) ;
#103735=CARTESIAN_POINT ( 'NONE',  ( -4.038582018629999659, 1515.598601288590089, 209.1218459616989946 ) ) ;
#103736=CARTESIAN_POINT ( 'NONE',  ( -13.90059962652860115, 1502.276548576450068, 227.4029734404369947 ) ) ;
#103738=CARTESIAN_POINT ( 'NONE',  ( -4.992622171949999910, 1391.631312501089951, 203.6357468861989730 ) ) ;
#103739=CARTESIAN_POINT ( 'NONE',  ( 9.806138588316610338, 1435.794735510610053, 209.7884860958980084 ) ) ;
#103741=CARTESIAN_POINT ( 'NONE',  ( -15.50017078884119925, 1420.382688314539791, 210.7385713550720254 ) ) ;
#103742=CARTESIAN_POINT ( 'NONE',  ( 4.250000000000000000, 1516.051704408390151, 209.1218459616989946 ) ) ;
#103747=CARTESIAN_POINT ( 'NONE',  ( 17.69622264849999738, 1430.679833671289771, 213.5595385020990022 ) ) ;
#103750=CARTESIAN_POINT ( 'NONE',  ( 8.117022692521160820, 1504.304627734529959, 218.0272414185070033 ) ) ;
#103755=VERTEX_POINT ( 'NONE', #21135 ) ;
#103759=CARTESIAN_POINT ( 'NONE',  ( -1.085993468421462049, 1457.203538262298252, 199.6660069001111140 ) ) ;
#103764=CARTESIAN_POINT ( 'NONE',  ( 18.87855043325079762, 1458.344546833890035, 213.8102210560949743 ) ) ;
#103765=B_SPLINE_CURVE_WITH_KNOTS ( 'NONE', 3,
 ( #9604, #52738, #43775, #70668, #35932, #68444, #69557, #60041, #70117, #28067, #69001, #53296, #52191, #103677, #104229, #104781, #76826, #140, #26976, #34262, #94719, #61166, #684, #94160, #53865, #77381, #60598, #10166, #102547, #51627, #19093, #103104, #86320, #78482, #27518, #26406, #77925, #85764, #1232, #25840, #35369, #34814, #9063, #95282, #43233, #86872, #19661, #44339, #1796, #61703, #44904, #95825, #87437, #10732, #79052, #2355, #96383, #62256, #36470, #88005, #42669 ),
 .UNSPECIFIED., .F., .F.,
 ( 4, 3, 3, 3, 3, 3, 3, 3, 3, 3, 3, 3, 3, 3, 3, 3, 3, 3, 3, 3, 4 ),
 ( 2.324858856900000159, 2.629298819338719895, 2.933834189079979726, 3.016888080820000262, 3.323211180994739777, 3.630193766017370205, 3.937176351040000188, 4.233214320261589947, 4.526002641850889852, 4.813615658591210433, 4.970096098089999970, 5.257590953320869787, 5.548112191959639894, 5.843468099502020507, 6.019659498230000239, 6.321166958536720060, 6.626011430711340466, 6.935803168168410693, 7.053491825980000129, 7.364378125943899178, 7.657659708029999734 ),
 .UNSPECIFIED. ) ;
#103767=CARTESIAN_POINT ( 'NONE',  ( 2.359087563130000120, 1467.696298592889889, 218.9570129866989987 ) ) ;
#103771=CARTESIAN_POINT ( 'NONE',  ( -8.684972823652898910, 1424.385334158459727, 206.2357065455580027 ) ) ;
#103775=CARTESIAN_POINT ( 'NONE',  ( -7.879428933958430470, 1439.609447256930025, 226.0913591242859866 ) ) ;
#103780=CARTESIAN_POINT ( 'NONE',  ( -14.45258105951289807, 1415.677402202029953, 212.7925583759839867 ) ) ;
#103784=CARTESIAN_POINT ( 'NONE',  ( -0.6005281695890769544, 1465.274001425240158, 198.1349723783799845 ) ) ;
#103785=EDGE_CURVE ( 'NONE', #1934, #52452, #26021, .T. ) ;
#103802=CARTESIAN_POINT ( 'NONE',  ( -0.1944809589943391759, 1455.245269478617274, 218.5524001425882261 ) ) ;
#103809=CARTESIAN_POINT ( 'NONE',  ( -3.071818229182819771, 1428.880991415399876, 200.2728629207279880 ) ) ;
#103825=CARTESIAN_POINT ( 'NONE',  ( -10.26351865721099799, 1448.707356115169887, 207.5368705317330011 ) ) ;
#103835=CARTESIAN_POINT ( 'NONE',  ( -0.8968889248344054099, 1469.603208379229500, 219.1395986089293331 ) ) ;
#103839=CARTESIAN_POINT ( 'NONE',  ( 1.401811570890000080, 1430.917890128589988, 199.7550729045790092 ) ) ;
#103840=CARTESIAN_POINT ( 'NONE',  ( 11.18378284279590140, 1480.307833489839823, 211.0917726453040189 ) ) ;
#103841=CARTESIAN_POINT ( 'NONE',  ( 1.894388308689999967, 1506.148290744889891, 221.7829938216989945 ) ) ;
#103846=CARTESIAN_POINT ( 'NONE',  ( 3.066664150160000268, 1486.999178531689950, 197.5625016150989950 ) ) ;
#103847=CARTESIAN_POINT ( 'NONE',  ( 9.145085911806999590, 1467.511344352970127, 205.0022163952010317 ) ) ;
#103850=CARTESIAN_POINT ( 'NONE',  ( 5.466273243599998999, 1504.965088730989919, 220.6538119101990105 ) ) ;
#103852=CARTESIAN_POINT ( 'NONE',  ( 8.177818021369999357, 1422.878296110979818, 213.9391550444189818 ) ) ;
#103855=CARTESIAN_POINT ( 'NONE',  ( -10.01326719289999900, 1481.014340515889899, 205.7823630344090020 ) ) ;
#103864=CARTESIAN_POINT ( 'NONE',  ( -2.975037811039999980, 1495.689967157589763, 216.9727041533189720 ) ) ;
#103867=CARTESIAN_POINT ( 'NONE',  ( -2.932381175664569906, 1457.907782490749923, 219.3878279419139972 ) ) ;
#103871=CARTESIAN_POINT ( 'NONE',  ( 7.594045040249999268, 1425.546108791900224, 212.0390539736889934 ) ) ;
#103872=CARTESIAN_POINT ( 'NONE',  ( 18.38166056949999927, 1428.164368492389940, 201.4944003551989908 ) ) ;
#103876=CARTESIAN_POINT ( 'NONE',  ( 4.758389699129999428, 1454.760432536389999, 217.3925755712789964 ) ) ;
#103877=ORIENTED_EDGE ( 'NONE', *, *, #7521, .F. ) ;
#103886=CARTESIAN_POINT ( 'NONE',  ( 2.268748340400060126, 1476.248048840699994, 197.8527876105920029 ) ) ;
#103898=ORIENTED_EDGE ( 'NONE', *, *, #83533, .F. ) ;
#103899=ORIENTED_EDGE ( 'NONE', *, *, #2239, .F. ) ;
#103900=CARTESIAN_POINT ( 'NONE',  ( -4.378216171020000047, 1453.707746106390005, 199.6107948432290016 ) ) ;
#103914=CARTESIAN_POINT ( 'NONE',  ( 10.46269364489999987, 1491.122602117189899, 212.5073291737689942 ) ) ;
#103915=AXIS2_PLACEMENT_3D ( 'NONE', #94880, #34964, #26562 ) ;
#103921=CARTESIAN_POINT ( 'NONE',  ( 10.52183747938889979, 1460.134765062619863, 206.2567342059500106 ) ) ;
#103923=VECTOR ( 'NONE', #90338, 1000.000000000000227 ) ;
#103926=CARTESIAN_POINT ( 'NONE',  ( 8.612130213264160616, 1437.494969288449965, 211.0257522034609963 ) ) ;
#103927=CARTESIAN_POINT ( 'NONE',  ( 5.172586535390000684, 1492.767659076290101, 188.8148697515989909 ) ) ;
#103928=CARTESIAN_POINT ( 'NONE',  ( -5.586178488784369733, 1491.246080089150155, 185.8699216472389821 ) ) ;
#103930=ORIENTED_EDGE ( 'NONE', *, *, #79453, .F. ) ;
#103937=CARTESIAN_POINT ( 'NONE',  ( -3.630422229999999750, 1429.843096179090026, 201.6307972852089847 ) ) ;
#103948=VERTEX_POINT ( 'NONE', #59201 ) ;
#103958=CARTESIAN_POINT ( 'NONE',  ( 2197.008826411130485, 11216.44053380570767, -1526.289979289628263 ) ) ;
#103964=CARTESIAN_POINT ( 'NONE',  ( 11.23851827549999882, 1490.487975447490044, 204.0492753133389954 ) ) ;
#103976=CARTESIAN_POINT ( 'NONE',  ( -10.46254913605810088, 1491.357146916849842, 212.5408882096329819 ) ) ;
#103977=CARTESIAN_POINT ( 'NONE',  ( -17.66148018635020378, 1440.150399676859934, 218.7822600330530065 ) ) ;
#103988=ORIENTED_EDGE ( 'NONE', *, *, #9346, .T. ) ;
#103990=CARTESIAN_POINT ( 'NONE',  ( -6.375527264914699010, 1460.280752625940067, 210.0337940185919763 ) ) ;
#103994=CARTESIAN_POINT ( 'NONE',  ( -4.598493981323799495, 1495.170853321719960, 197.6879014759489905 ) ) ;
#104002=CARTESIAN_POINT ( 'NONE',  ( 8.234565746623669469, 1434.603406620469741, 205.5025735347319937 ) ) ;
#104004=CARTESIAN_POINT ( 'NONE',  ( -11.79257184573279993, 1490.424927523380120, 209.6468054329459960 ) ) ;
#104007=CARTESIAN_POINT ( 'NONE',  ( -11.98355723010000062, 1507.902190792990041, 208.7310628602519955 ) ) ;
#104008=CARTESIAN_POINT ( 'NONE',  ( 20.42677715031149788, 1475.927527670890186, 217.8974877716310061 ) ) ;
#104016=CARTESIAN_POINT ( 'NONE',  ( -20.60448988230000111, 1484.737042837089803, 209.1218459616989946 ) ) ;
#104024=CARTESIAN_POINT ( 'NONE',  ( -9.255392140700001491, 1423.205578550119753, 209.4023171091370159 ) ) ;
#104025=ORIENTED_EDGE ( 'NONE', *, *, #35739, .T. ) ;
#104027=CARTESIAN_POINT ( 'NONE',  ( -7.437974795490000623, 1473.518143733989973, 200.3716835635890163 ) ) ;
#104028=CARTESIAN_POINT ( 'NONE',  ( -3.369085047521843457, 1470.161991784903194, 218.6691817296217835 ) ) ;
#104031=CARTESIAN_POINT ( 'NONE',  ( 2.204495346684369750, 1495.683245216109981, 221.2628089792190167 ) ) ;
#104032=VERTEX_POINT ( 'NONE', #92772 ) ;
#104039=CARTESIAN_POINT ( 'NONE',  ( 6.153332312239999879, 1471.680546255089894, 217.2442593896689971 ) ) ;
#104040=CARTESIAN_POINT ( 'NONE',  ( -9.490149457628850982, 1439.534074077459991, 207.9559815647490097 ) ) ;
#104045=LINE ( 'NONE', #1608, #91260 ) ;
#104065=CARTESIAN_POINT ( 'NONE',  ( 3.117394561335599779, 1508.880976916049804, 204.6292040151590186 ) ) ;
#104082=CARTESIAN_POINT ( 'NONE',  ( -17.42683798559999886, 1417.851019997039884, 207.0376866630389827 ) ) ;
#104088=CARTESIAN_POINT ( 'NONE',  ( 1.182417329582052812, 1421.364694982859646, 193.7605960035091925 ) ) ;
#104089=ADVANCED_FACE ( 'NONE', ( #7666 ), #33403, .T. ) ;
#104094=ADVANCED_FACE ( 'NONE', ( #83823 ), #16772, .T. ) ;
#104097=CARTESIAN_POINT ( 'NONE',  ( -9.991880054531121047, 1461.400997162919793, 210.8424979650880005 ) ) ;
#104099=CARTESIAN_POINT ( 'NONE',  ( -17.57139056652149733, 1418.330242804019917, 206.9610443431660087 ) ) ;
#104110=CARTESIAN_POINT ( 'NONE',  ( -13.90059966380340128, 1502.276548245260074, 227.4029733933120099 ) ) ;
#104113=CARTESIAN_POINT ( 'NONE',  ( -14.93837056410000130, 1416.023439710309958, 212.9159407817990086 ) ) ;
#104115=FACE_OUTER_BOUND ( 'NONE', #8971, .T. ) ;
#104117=CARTESIAN_POINT ( 'NONE',  ( 6.922360974429970794E-17, 1415.677402202029953, 209.1218459616989946 ) ) ;
#104119=CARTESIAN_POINT ( 'NONE',  ( -4.504196618690000875, 1474.524975280490025, 198.6118189482990033 ) ) ;
#104122=CARTESIAN_POINT ( 'NONE',  ( -5.156516201845800396, 1508.551704408389924, 219.6384978436439894 ) ) ;
#104129=CARTESIAN_POINT ( 'NONE',  ( 4.967684734197839624, 1469.890600053420030, 189.7939087450779994 ) ) ;
#104131=CARTESIAN_POINT ( 'NONE',  ( -11.06960323243380095, 1471.418000880429872, 206.7781049577790213 ) ) ;
#104137=VERTEX_POINT ( 'NONE', #43494 ) ;
#104139=CARTESIAN_POINT ( 'NONE',  ( 10.96545847595860046, 1490.902137392429950, 209.8197085273070002 ) ) ;
#104142=CARTESIAN_POINT ( 'NONE',  ( 8.833925975006069464, 1465.118606178020173, 213.5047465619319951 ) ) ;
#104157=B_SPLINE_CURVE_WITH_KNOTS ( 'NONE', 3,
 ( #43967, #94917, #877, #42302, #51823, #44521, #69181, #35002, #86507, #85962, #9802, #78108, #59128, #76455, #18733, #1410, #68631, #102733, #9262, #43421, #1985, #110609, #67529, #51255, #101629, #24918, #59671, #33891, #102199, #25478, #85388, #20940, #55692, #105530, #97668, #28820, #63017, #96576, #61896 ),
 .UNSPECIFIED., .F., .F.,
 ( 4, 2, 2, 1, 1, 1, 1, 2, 2, 2, 2, 1, 1, 1, 1, 2, 2, 2, 2, 1, 1, 1, 2, 2, 4 ),
 ( 0.000000000000000000, 0.1249999999992091604, 0.1874999999988137267, 0.2187499999986127763, 0.2343749999985210719, 0.2421874999984882926, 0.2460937499984814925, 0.2480468749984781063, 0.2499999999984747201, 0.3749999999988570254, 0.4374999999990452637, 0.4687499999991468491, 0.4843749999991899258, 0.4921874999992034705, 0.4960937499992135735, 0.4980468749992186805, 0.4999999999992237321, 0.6249999999993625099, 0.6874999999994277911, 0.7187499999994527711, 0.7343749999994535482, 0.7421874999994576561, 0.7460937499994595434, 0.7499999999994614308, 1.000000000000000000 ),
 .UNSPECIFIED. ) ;
#104161=CARTESIAN_POINT ( 'NONE',  ( -2.318462068020000100, 1495.571024868690074, 220.0861427028989965 ) ) ;
#104162=ORIENTED_EDGE ( 'NONE', *, *, #103476, .F. ) ;
#104176=CARTESIAN_POINT ( 'NONE',  ( -5.249808435119999395, 1391.918258567789962, 214.5638896842290251 ) ) ;
#104180=CARTESIAN_POINT ( 'NONE',  ( 9.611691241550468945, 1460.529588664869834, 206.0549884057099916 ) ) ;
#104182=ORIENTED_EDGE ( 'NONE', *, *, #99531, .T. ) ;
#104190=CARTESIAN_POINT ( 'NONE',  ( -5.924352395060029863, 1419.506400887321433, 194.9066959792404532 ) ) ;
#104192=CARTESIAN_POINT ( 'NONE',  ( 12.47681624269289280, 1420.546772247846320, 200.4723319259569791 ) ) ;
#104194=CARTESIAN_POINT ( 'NONE',  ( 10.40178565224220009, 1451.751389650100009, 207.5054792126090035 ) ) ;
#104195=CARTESIAN_POINT ( 'NONE',  ( -3.337824073649999779, 1502.591014432890006, 230.2741237628989950 ) ) ;
#104206=CARTESIAN_POINT ( 'NONE',  ( -7.144831657780449596, 1508.449369756350052, 219.6178892270350218 ) ) ;
#104208=CARTESIAN_POINT ( 'NONE',  ( -9.489078762094210973, 1470.877762335149782, 213.0725583738820035 ) ) ;
#104211=CARTESIAN_POINT ( 'NONE',  ( 9.146237114798470458, 1449.998848199699978, 208.1168068718100130 ) ) ;
#104213=CARTESIAN_POINT ( 'NONE',  ( -2.457346683533450094, 1422.331128196689860, 192.7387433577370075 ) ) ;
#104215=CARTESIAN_POINT ( 'NONE',  ( 8.332319144487495777, 1424.430118509189697, 195.7440745982989654 ) ) ;
#104216=CARTESIAN_POINT ( 'NONE',  ( -13.48450404919999990, 1503.201074756489788, 208.7146732095060031 ) ) ;
#104217=CARTESIAN_POINT ( 'NONE',  ( 9.887881744141459706, 1469.108246522290074, 203.7125116724459986 ) ) ;
#104221=CARTESIAN_POINT ( 'NONE',  ( -4.644703737721179060, 1496.617562890359977, 216.2902365695769902 ) ) ;
#104222=VERTEX_POINT ( 'NONE', #96086 ) ;
#104228=CARTESIAN_POINT ( 'NONE',  ( -14.37783120989999830, 1415.677402202029953, 213.0868688017489774 ) ) ;
#104229=CARTESIAN_POINT ( 'NONE',  ( 0.9886889294276358653, 1515.109643008290050, 204.7935716275389950 ) ) ;
#104230=ORIENTED_EDGE ( 'NONE', *, *, #120, .F. ) ;
#104242=EDGE_CURVE ( 'NONE', #104222, #9164, #29420, .T. ) ;
#104243=CARTESIAN_POINT ( 'NONE',  ( -10.89975107439999924, 1480.485161721690019, 212.5137882077189886 ) ) ;
#104254=CARTESIAN_POINT ( 'NONE',  ( -11.41402561306639996, 1500.969831351809944, 208.5831151434670119 ) ) ;
#104257=CARTESIAN_POINT ( 'NONE',  ( -16.31919663280000066, 1416.362649511440168, 209.6296053043620020 ) ) ;
#104280=DIRECTION ( 'NONE',  ( 0.4436356471204840890, 0.000000000000000000, 0.8962072375315819350 ) ) ;
#104285=CARTESIAN_POINT ( 'NONE',  ( 11.74549576979310039, 1479.261940693859970, 208.3477357056440269 ) ) ;
#104287=CARTESIAN_POINT ( 'NONE',  ( 10.60563969924810124, 1451.919000108789987, 190.2093396595549848 ) ) ;
#104293=CARTESIAN_POINT ( 'NONE',  ( -4.994701126379999856, 1391.710704567790117, 203.7548416175590091 ) ) ;
#104295=CARTESIAN_POINT ( 'NONE',  ( -11.37189650340000213, 1489.740153703190117, 212.1629306840389972 ) ) ;
#104319=CARTESIAN_POINT ( 'NONE',  ( -7.547148334389939706, 1424.043885779579796, 208.8816623809889848 ) ) ;
#104323=CARTESIAN_POINT ( 'NONE',  ( -6.312270842414640093, 1439.251699911259948, 226.7179307010800073 ) ) ;
#104332=CARTESIAN_POINT ( 'NONE',  ( 0.4668132112965759917, 1465.514551817379925, 198.1226951640539937 ) ) ;
#104340=EDGE_LOOP ( 'NONE', ( #56793, #110624, #84630, #6963 ) ) ;
#104342=EDGE_CURVE ( 'NONE', #73262, #58610, #8773, .T. ) ;
#104349=CARTESIAN_POINT ( 'NONE',  ( -3.955240613149759721, 1433.657955356159846, 217.8573778194910062 ) ) ;
#104354=CARTESIAN_POINT ( 'NONE',  ( 8.091207885150058843, 1435.785749346069906, 206.2618432467970138 ) ) ;
#104360=CARTESIAN_POINT ( 'NONE',  ( -11.61827763164220073, 1482.582230581700060, 206.5199852600759982 ) ) ;
#104372=EDGE_CURVE ( 'NONE', #38904, #57731, #101977, .T. ) ;
#104375=CARTESIAN_POINT ( 'NONE',  ( -8.931373544893890681, 1449.107262902880166, 211.1739995703599959 ) ) ;
#104379=CARTESIAN_POINT ( 'NONE',  ( -9.242820708772759630, 1508.434507021560194, 219.0621371396210009 ) ) ;
#104385=CARTESIAN_POINT ( 'NONE',  ( 17.70437741359999961, 1453.580057579390086, 200.5051001409389926 ) ) ;
#104386=B_SPLINE_CURVE_WITH_KNOTS ( 'NONE', 5,
 ( #98463, #54296, #38021, #97364, #82213, #71671 ),
 .UNSPECIFIED., .F., .F.,
 ( 6, 6 ),
 ( -1.999998997246040133, -9.600809889320771617E-07 ),
 .UNSPECIFIED. ) ;
#104390=B_SPLINE_CURVE_WITH_KNOTS ( 'NONE', 5,
 ( #13695, #91538, #30520, #109450, #74748, #21546, #32179, #83136, #47881 ),
 .UNSPECIFIED., .F., .F.,
 ( 6, 3, 6 ),
 ( 429.1212792279999917, 432.6128460950000090, 434.2407011939999961 ),
 .UNSPECIFIED. ) ;
#104391=CARTESIAN_POINT ( 'NONE',  ( -0.5241100996639990184, 1430.162173504289967, 199.7031367948490015 ) ) ;
#104394=CARTESIAN_POINT ( 'NONE',  ( -4.290508147089998836, 1515.379315998089851, 209.4884831641960261 ) ) ;
#104398=CARTESIAN_POINT ( 'NONE',  ( -0.1939829864129989923, 1486.063949427190209, 197.1933270691990003 ) ) ;
#104399=CARTESIAN_POINT ( 'NONE',  ( 3.238173812045069599, 1465.056324971090135, 199.8094274036559739 ) ) ;
#104401=CARTESIAN_POINT ( 'NONE',  ( 1.247882275640000094, 1499.086922831090078, 200.6750384717489908 ) ) ;
#104404=CARTESIAN_POINT ( 'NONE',  ( 8.719508408019999379, 1427.931009161789916, 212.3464450776189949 ) ) ;
#104408=CARTESIAN_POINT ( 'NONE',  ( 8.759801967190000482, 1450.891143041990063, 191.6269498783990173 ) ) ;
#104416=CARTESIAN_POINT ( 'NONE',  ( -13.58246093890570094, 1508.543141741580030, 210.2041360783450159 ) ) ;
#104419=CARTESIAN_POINT ( 'NONE',  ( -9.797288353148440265, 1438.442783550709919, 210.7140074991049801 ) ) ;
#104422=CARTESIAN_POINT ( 'NONE',  ( -9.467068884459999722, 1450.246902653889947, 204.4311477998990085 ) ) ;
#104424=CARTESIAN_POINT ( 'NONE',  ( 7.755601986420000316, 1424.473492849049990, 212.0082642979490117 ) ) ;
#104425=CARTESIAN_POINT ( 'NONE',  ( -19.34949465300000071, 1446.106505183189938, 200.0047805777890062 ) ) ;
#104426=B_SPLINE_CURVE_WITH_KNOTS ( 'NONE', 3,
 ( #102022, #93081, #85227, #75206, #24215, #100916, #16896, #41595, #57319, #83576, #91986, #7430, #33723, #58401, #58949, #32638, #66815, #68465, #49996, #92526, #51102, #67915 ),
 .UNSPECIFIED., .F., .F.,
 ( 4, 3, 3, 3, 3, 3, 3, 4 ),
 ( 6.826668448630000685E-15, 1.142757973758999901, 2.309653782353159990, 3.228996148453810111, 3.979625921832550262, 5.138688428070659953, 5.803026787480529691, 6.457992286039999641 ),
 .UNSPECIFIED. ) ;
#104431=FACE_OUTER_BOUND ( 'NONE', #71716, .T. ) ;
#104440=CARTESIAN_POINT ( 'NONE',  ( -2.509809942567690300, 1464.411809687589994, 199.2066022212569862 ) ) ;
#104457=CARTESIAN_POINT ( 'NONE',  ( 4.924481260220000323, 1423.601678417960102, 208.0358385729389852 ) ) ;
#104461=CARTESIAN_POINT ( 'NONE',  ( 10.46269364489999987, 1491.122602117189899, 212.5073291737689942 ) ) ;
#104470=CARTESIAN_POINT ( 'NONE',  ( 2.999854732238141697, 1441.831681250876045, 217.8331532270901221 ) ) ;
#104479=B_SPLINE_CURVE_WITH_KNOTS ( 'NONE', 3,
 ( #62067, #105712, #104031, #87810, #88893, #78280, #18905, #70469, #54762, #46368, #45813, #78852, #1592, #9974, #28995, #18353, #2711, #86678, #63181, #80505, #96192, #79947, #20024, #44703, #71026, #52546, #35730, #104589, #27884, #44145, #69918, #54219, #88345, #72129, #61508, #19467, #2162 ),
 .UNSPECIFIED., .F., .F.,
 ( 4, 3, 3, 3, 3, 3, 3, 3, 3, 3, 3, 3, 4 ),
 ( -13.74231060008099981, -13.66514189682659897, -12.92929132305900097, -12.11627204603709984, -11.30376823848880008, -10.44046530963600006, -9.415415393832899937, -8.316051554799299694, -7.441798631434849653, -6.496218934871920148, -5.648106363132958663, -4.910580565460959335, -4.218056259389999951 ),
 .UNSPECIFIED. ) ;
#104481=FACE_OUTER_BOUND ( 'NONE', #101292, .T. ) ;
#104484=VERTEX_POINT ( 'NONE', #72175 ) ;
#104490=CARTESIAN_POINT ( 'NONE',  ( -2.981671477319999930, 1430.762427285789954, 201.3088114122890033 ) ) ;
#104503=ORIENTED_EDGE ( 'NONE', *, *, #32448, .F. ) ;
#104506=ORIENTED_EDGE ( 'NONE', *, *, #97397, .F. ) ;
#104512=CARTESIAN_POINT ( 'NONE',  ( 2.801853610880000289, 1442.344586916589833, 217.6656895430990062 ) ) ;
#104514=CARTESIAN_POINT ( 'NONE',  ( -271.2574215431060338, 11216.44053380568585, -1816.021012422609601 ) ) ;
#104519=CARTESIAN_POINT ( 'NONE',  ( -5.534100668969379910, 1464.371862158079921, 199.5915835189479992 ) ) ;
#104521=CARTESIAN_POINT ( 'NONE',  ( 9.374206578739999074, 1489.420254891390186, 201.2494609442489946 ) ) ;
#104524=EDGE_LOOP ( 'NONE', ( #52923, #97391, #37530, #46450 ) ) ;
#104528=CARTESIAN_POINT ( 'NONE',  ( -2.454075143049999852, 1484.161599711790132, 198.7041245505990048 ) ) ;
#104530=CARTESIAN_POINT ( 'NONE',  ( -10.50583156713009991, 1480.154605857860133, 208.5861483567410062 ) ) ;
#104532=CARTESIAN_POINT ( 'NONE',  ( 7.500000000000000000, 1391.913060387289988, 209.1218459616989946 ) ) ;
#104534=CARTESIAN_POINT ( 'NONE',  ( -11.52230023899750044, 1489.339508248780248, 213.1482211750440001 ) ) ;
#104535=CARTESIAN_POINT ( 'NONE',  ( -16.61337778659050102, 1463.629532367329830, 220.4655059527940182 ) ) ;
#104540=ADVANCED_FACE ( 'NONE', ( #4400 ), #71508, .F. ) ;
#104554=CARTESIAN_POINT ( 'NONE',  ( -4.473177171425660070, 1495.214931084829914, 197.6378604175340001 ) ) ;
#104557=CARTESIAN_POINT ( 'NONE',  ( 18.81609481059999922, 1456.479165729590022, 204.5196734937790097 ) ) ;
#104563=CARTESIAN_POINT ( 'NONE',  ( -13.82453468407210018, 1421.936557082180116, 203.7229994192829849 ) ) ;
#104567=CARTESIAN_POINT ( 'NONE',  ( -4.240940644606780552, 1509.032041130069956, 212.8662740090449859 ) ) ;
#104568=CARTESIAN_POINT ( 'NONE',  ( 9.890535630430530745, 1492.213485579389953, 188.4030009006890225 ) ) ;
#104570=CARTESIAN_POINT ( 'NONE',  ( 7.503571368420000276, 1422.857534295030064, 195.6852864414989881 ) ) ;
#104578=CARTESIAN_POINT ( 'NONE',  ( -9.321551428969998554, 1460.110613089990011, 211.8159337765089845 ) ) ;
#104586=CARTESIAN_POINT ( 'NONE',  ( -10.06450494029999909, 1472.332863763290106, 203.5506889703189870 ) ) ;
#104589=CARTESIAN_POINT ( 'NONE',  ( -2.323079643848300346, 1496.857146867429947, 221.2763090542839848 ) ) ;
#104595=CARTESIAN_POINT ( 'NONE',  ( 2.764546554733247508, 1486.833185097884325, 219.5825234514556712 ) ) ;
#104596=CARTESIAN_POINT ( 'NONE',  ( -16.59330332571189714, 1508.551704408389924, 213.1175702257220053 ) ) ;
#104598=CARTESIAN_POINT ( 'NONE',  ( -8.809230282280388735, 1438.685521035069996, 208.2566144035540106 ) ) ;
#104603=CARTESIAN_POINT ( 'NONE',  ( -0.9541980962059989357, 1483.985701800989773, 201.2944015401489821 ) ) ;
#104604=CARTESIAN_POINT ( 'NONE',  ( 9.205082684422309924, 1434.999538654240041, 207.3832038862170180 ) ) ;
#104606=ORIENTED_EDGE ( 'NONE', *, *, #101724, .T. ) ;
#104609=CARTESIAN_POINT ( 'NONE',  ( 2.870880155352820040, 1466.604627524899797, 219.7960964397389887 ) ) ;
#104621=ORIENTED_EDGE ( 'NONE', *, *, #84525, .F. ) ;
#104642=CIRCLE ( 'NONE', #63597, 7.500000000000000000 ) ;
#104643=CARTESIAN_POINT ( 'NONE',  ( 1.302691703616797758, 1421.395884623610755, 193.7699158457419344 ) ) ;
#104651=CARTESIAN_POINT ( 'NONE',  ( -17.08916621680459969, 1420.636132269700056, 201.6183731251909990 ) ) ;
#104656=CARTESIAN_POINT ( 'NONE',  ( -1.333616551530000249, 1444.154719697190103, 199.5606640046889879 ) ) ;
#104659=CARTESIAN_POINT ( 'NONE',  ( -16.75463440289568950, 1420.038624242013157, 208.1824980296739227 ) ) ;
#104663=CARTESIAN_POINT ( 'NONE',  ( -3.224548122823300389, 1508.551704408489968, 204.2884089881570162 ) ) ;
#104672=CARTESIAN_POINT ( 'NONE',  ( -4.132631535169999815, 1476.440258689390021, 199.6218979630789931 ) ) ;
#104675=CARTESIAN_POINT ( 'NONE',  ( -5.717689142141139769, 1508.551704408389924, 219.5099898771389917 ) ) ;
#104681=CARTESIAN_POINT ( 'NONE',  ( -0.4792132924880010414, 1431.125656909089912, 217.6287611528490231 ) ) ;
#104695=CARTESIAN_POINT ( 'NONE',  ( -5.301602273869999493, 1495.069292928890036, 198.4488064414990163 ) ) ;
#104707=CARTESIAN_POINT ( 'NONE',  ( 2.371343438090000255, 1497.319062567490164, 197.3529125933990258 ) ) ;
#104708=CARTESIAN_POINT ( 'NONE',  ( -0.2209949390820010184, 1494.455004241089910, 220.2892042338989995 ) ) ;
#104719=CARTESIAN_POINT ( 'NONE',  ( 11.78230151170000006, 1435.286215961589960, 224.1839025558989817 ) ) ;
#104725=EDGE_CURVE ( 'NONE', #92866, #46415, #76608, .T. ) ;
#104726=LINE ( 'NONE', #63307, #44484 ) ;
#104735=CARTESIAN_POINT ( 'NONE',  ( 8.857752970044110441, 1451.634138792180011, 211.8773160595700062 ) ) ;
#104736=CARTESIAN_POINT ( 'NONE',  ( 7.991060968840001166, 1423.743734712820014, 195.9120172666990243 ) ) ;
#104737=ORIENTED_EDGE ( 'NONE', *, *, #17976, .F. ) ;
#104739=CARTESIAN_POINT ( 'NONE',  ( -6.042023989919642624, 1419.473644842602880, 194.9560967347969722 ) ) ;
#104744=CARTESIAN_POINT ( 'NONE',  ( 10.11442602625619891, 1452.508834773780109, 209.7499184922420170 ) ) ;
#104752=CARTESIAN_POINT ( 'NONE',  ( -10.61999372029469946, 1462.990852176999852, 206.0510140530389833 ) ) ;
#104755=CARTESIAN_POINT ( 'NONE',  ( -1.569490127089286480, 1507.974949272165532, 221.0030736985697786 ) ) ;
#104756=CARTESIAN_POINT ( 'NONE',  ( -4.863838082751120062, 1508.339116710969847, 220.3751376775360029 ) ) ;
#104760=CARTESIAN_POINT ( 'NONE',  ( -6.941887704655929525, 1471.020790314250007, 216.5580302958940138 ) ) ;
#104766=CARTESIAN_POINT ( 'NONE',  ( 8.630513237909999802, 1492.548647927590082, 216.1639467023389898 ) ) ;
#104769=CARTESIAN_POINT ( 'NONE',  ( -18.20628436530000016, 1504.691793905290069, 209.0089166509420124 ) ) ;
#104770=CARTESIAN_POINT ( 'NONE',  ( 10.69207100893769891, 1469.742000000100006, 205.4164582955250182 ) ) ;
#104771=CARTESIAN_POINT ( 'NONE',  ( 11.02420060192179996, 1422.875103594119992, 206.9420604818759841 ) ) ;
#104772=CARTESIAN_POINT ( 'NONE',  ( -9.906853760125690300, 1439.767124081580050, 207.7335298351040080 ) ) ;
#104779=CARTESIAN_POINT ( 'NONE',  ( 3.561968053029999748, 1506.511571253490047, 220.3681567290990131 ) ) ;
#104780=CARTESIAN_POINT ( 'NONE',  ( -14.62125525909999979, 1415.677402202029953, 212.1284411519390289 ) ) ;
#104781=CARTESIAN_POINT ( 'NONE',  ( 0.9184306762236260635, 1515.115092018379983, 204.7937143148920143 ) ) ;
#104783=CARTESIAN_POINT ( 'NONE',  ( -15.74969544120698117, 1415.781883517263168, 209.6858483997482665 ) ) ;
#104785=CARTESIAN_POINT ( 'NONE',  ( -10.23213401892603436, 1472.778035024365408, 208.9421871917756448 ) ) ;
#104787=CARTESIAN_POINT ( 'NONE',  ( 9.561942892529945226, 1436.616837100986459, 211.5588262537796709 ) ) ;
#104794=CARTESIAN_POINT ( 'NONE',  ( -19.15298488520000220, 1464.559837765089924, 213.8319524061190009 ) ) ;
#104804=CARTESIAN_POINT ( 'NONE',  ( -15.33452496817989896, 1418.116965089579935, 203.1099089491380028 ) ) ;
#104811=CARTESIAN_POINT ( 'NONE',  ( 1.713123635352999941, 1431.453930620565643, 200.4877085583662790 ) ) ;
#104816=CARTESIAN_POINT ( 'NONE',  ( -13.58886547874749873, 1508.451091720879958, 209.7742548574910302 ) ) ;
#104820=CARTESIAN_POINT ( 'NONE',  ( -11.87772997576320044, 1481.884250532160195, 209.0415709480480189 ) ) ;
#104831=CARTESIAN_POINT ( 'NONE',  ( 3.906019471690000078, 1515.551703594190030, 207.6331533119790151 ) ) ;
#104837=CARTESIAN_POINT ( 'NONE',  ( 11.72230831049659905, 1479.187001874789985, 208.0687465664710203 ) ) ;
#104840=CARTESIAN_POINT ( 'NONE',  ( 8.241694428620000679, 1462.303391458189935, 228.8627610174989968 ) ) ;
#104845=CARTESIAN_POINT ( 'NONE',  ( -4.994708985280000846, 1391.711004686890192, 203.7017277140789986 ) ) ;
#104847=CARTESIAN_POINT ( 'NONE',  ( -11.00301372470000061, 1492.094802143589959, 210.0154403701209844 ) ) ;
#104851=ADVANCED_FACE ( 'NONE', ( #70949 ), #50780, .T. ) ;
#104853=CARTESIAN_POINT ( 'NONE',  ( 5.597770706110460459, 1506.679316021459954, 219.3685166263610142 ) ) ;
#104854=CARTESIAN_POINT ( 'NONE',  ( -12.72386900654892017, 1421.513396326319935, 210.6452810979295975 ) ) ;
#104873=CARTESIAN_POINT ( 'NONE',  ( -11.37749809445980098, 1422.109346327800040, 209.6141660988719764 ) ) ;
#104877=CARTESIAN_POINT ( 'NONE',  ( -17.84645756668390248, 1442.885565304640295, 215.1978005858999836 ) ) ;
#104878=ORIENTED_EDGE ( 'NONE', *, *, #24674, .F. ) ;
#104886=CARTESIAN_POINT ( 'NONE',  ( 10.92857027410000015, 1460.888924372889960, 208.5047761330480114 ) ) ;
#104887=EDGE_CURVE ( 'NONE', #95667, #94338, #37490, .T. ) ;
#104890=CARTESIAN_POINT ( 'NONE',  ( 2.768534767419999820, 1465.332393548289929, 199.5050815057789748 ) ) ;
#104893=EDGE_LOOP ( 'NONE', ( #25383, #65224, #3241, #33450 ) ) ;
#104898=VERTEX_POINT ( 'NONE', #106701 ) ;
#104909=CARTESIAN_POINT ( 'NONE',  ( -3.462099826290000237, 1507.707684683789921, 221.1489180092989955 ) ) ;
#104922=CARTESIAN_POINT ( 'NONE',  ( 18.81609481059999922, 1456.479165729590022, 204.5196734937790097 ) ) ;
#104925=DIRECTION ( 'NONE',  ( -9.138167445698339565E-47, 1.000000000000000000, -1.836970198721029688E-16 ) ) ;
#104928=CARTESIAN_POINT ( 'NONE',  ( -15.44036390149999960, 1415.706691406219988, 208.4181337457800112 ) ) ;
#104929=CARTESIAN_POINT ( 'NONE',  ( -12.48995958582669985, 1501.883328869510024, 211.6213070116990025 ) ) ;
#104938=CARTESIAN_POINT ( 'NONE',  ( -1.486478317020000217, 1515.456929490889934, 213.2968315210090111 ) ) ;
#104941=CARTESIAN_POINT ( 'NONE',  ( -19.83635568480000089, 1467.142385457190130, 209.5260977821610027 ) ) ;
#104944=CARTESIAN_POINT ( 'NONE',  ( 3.375977085881459949, 1446.395221913229989, 199.5681764770490076 ) ) ;
#104945=CARTESIAN_POINT ( 'NONE',  ( 1.662851635919999849, 1431.604427083889959, 200.5143776403489824 ) ) ;
#104946=CARTESIAN_POINT ( 'NONE',  ( -15.94166200583058490, 1416.020774055787342, 209.6543190501261620 ) ) ;
#104947=CARTESIAN_POINT ( 'NONE',  ( 3.554299344259999938, 1505.806595535689894, 220.9721874952989822 ) ) ;
#104949=ORIENTED_EDGE ( 'NONE', *, *, #55715, .F. ) ;
#104968=VERTEX_POINT ( 'NONE', #57980 ) ;
#104969=CARTESIAN_POINT ( 'NONE',  ( -11.40035806272144470, 1501.109170488654854, 208.2596098937023328 ) ) ;
#104970=CARTESIAN_POINT ( 'NONE',  ( -13.58909363943140036, 1508.363827828459989, 209.7584773189200007 ) ) ;
#104973=CARTESIAN_POINT ( 'NONE',  ( -9.978796886447030445, 1439.268830739550140, 208.9290397175849989 ) ) ;
#104978=CARTESIAN_POINT ( 'NONE',  ( 7.957350483939999108, 1425.611849966230011, 211.5358269577189958 ) ) ;
#104980=CARTESIAN_POINT ( 'NONE',  ( 14.17511973000000047, 1428.761297070790079, 195.0897165316990254 ) ) ;
#104985=CARTESIAN_POINT ( 'NONE',  ( 7.695178307639999993, 1454.153012403389994, 215.2868595619190160 ) ) ;
#104990=CARTESIAN_POINT ( 'NONE',  ( -1.213893508954652534, 1442.512427547091193, 200.3199665731655443 ) ) ;
#104996=CARTESIAN_POINT ( 'NONE',  ( -2.603434334352570101, 1463.518582721570056, 199.6736037120420235 ) ) ;
#105006=CARTESIAN_POINT ( 'NONE',  ( 3.919202604670000145, 1440.900018029090006, 218.2279973031590146 ) ) ;
#105009=ORIENTED_EDGE ( 'NONE', *, *, #100474, .T. ) ;
#105011=CARTESIAN_POINT ( 'NONE',  ( -3.264931758469999945, 1455.156802322290105, 200.1463041844289990 ) ) ;
#105018=CARTESIAN_POINT ( 'NONE',  ( 0.000000000000000000, 1420.584111001019892, 209.1218459616989946 ) ) ;
#105022=CARTESIAN_POINT ( 'NONE',  ( -12.22915601319570200, 1490.209347939349982, 209.7391394842479997 ) ) ;
#105029=LINE ( 'NONE', #87690, #110146 ) ;
#105041=CARTESIAN_POINT ( 'NONE',  ( 8.294124457724750599, 1425.422146639270068, 193.1250435841020021 ) ) ;
#105042=CARTESIAN_POINT ( 'NONE',  ( 19.12713426963480146, 1496.834684404690051, 222.0421991225989871 ) ) ;
#105050=CARTESIAN_POINT ( 'NONE',  ( -2.941234743340000346, 1429.809722365389916, 201.2044919420790166 ) ) ;
#105059=CARTESIAN_POINT ( 'NONE',  ( 9.905209297491678555, 1468.559939475269857, 207.6655895676410069 ) ) ;
#105064=ORIENTED_EDGE ( 'NONE', *, *, #49384, .F. ) ;
#105065=CARTESIAN_POINT ( 'NONE',  ( 7.654614188889650173, 1489.887865978259924, 207.9968767246130028 ) ) ;
#105068=CARTESIAN_POINT ( 'NONE',  ( 3.001614222390000197, 1441.369934486689999, 218.5760139890790299 ) ) ;
#105070=CARTESIAN_POINT ( 'NONE',  ( -1970.639179128770138, -8387.357407334289746, 1.374729025600770038 ) ) ;
#105077=CARTESIAN_POINT ( 'NONE',  ( 4.329200639848810539, 1515.074268821609849, 207.6257481534460112 ) ) ;
#105084=CARTESIAN_POINT ( 'NONE',  ( -5.301886427999999540, 1484.919761519890017, 198.4532048381990137 ) ) ;
#105090=CARTESIAN_POINT ( 'NONE',  ( -10.22907582296480200, 1490.127153888709927, 213.4824587814819665 ) ) ;
#105091=CARTESIAN_POINT ( 'NONE',  ( 10.99043244679999987, 1479.494642110589893, 229.8297439418990109 ) ) ;
#105096=CARTESIAN_POINT ( 'NONE',  ( 4.737752338079999959, 1428.052317588289952, 215.9265451789589747 ) ) ;
#105097=CARTESIAN_POINT ( 'NONE',  ( -18.82420833825850437, 1444.120425544869931, 209.6987789698510198 ) ) ;
#105098=ORIENTED_EDGE ( 'NONE', *, *, #29151, .F. ) ;
#105110=CARTESIAN_POINT ( 'NONE',  ( 9.014726288018540146, 1435.931555954980013, 208.8389660296269881 ) ) ;
#105113=CARTESIAN_POINT ( 'NONE',  ( 11.53661564504106174, 1502.557334605151937, 209.2924327149770534 ) ) ;
#105118=CARTESIAN_POINT ( 'NONE',  ( -9.103468112560660686, 1449.499701819690017, 210.3008494512589834 ) ) ;
#105119=DIRECTION ( 'NONE',  ( 0.2829264727638239885, 0.3709838398322150010, 0.8844905887530780664 ) ) ;
#105125=VERTEX_POINT ( 'NONE', #94877 ) ;
#105126=CARTESIAN_POINT ( 'NONE',  ( -3.788285567717010416, 1508.728291974460035, 213.4250882028100023 ) ) ;
#105127=CARTESIAN_POINT ( 'NONE',  ( -4.179417150059999919, 1482.939659495389833, 231.1991619290989775 ) ) ;
#105129=CARTESIAN_POINT ( 'NONE',  ( 11.16376535829999916, 1420.610325767149789, 198.7943618068990190 ) ) ;
#105134=CARTESIAN_POINT ( 'NONE',  ( 3.444951101639869950, 1484.732918568139894, 220.4578280794839884 ) ) ;
#105135=CARTESIAN_POINT ( 'NONE',  ( -9.649970257700001497, 1460.854139312389862, 213.4680788249189902 ) ) ;
#105139=CARTESIAN_POINT ( 'NONE',  ( -7.999790656699999225, 1424.877929483370053, 210.4221880905789988 ) ) ;
#105142=CARTESIAN_POINT ( 'NONE',  ( -9.828024340748898524, 1446.801136768030119, 212.2328356403849909 ) ) ;
#105144=CARTESIAN_POINT ( 'NONE',  ( -3.829619994797929916, 1515.551704292389786, 210.9648097401420159 ) ) ;
#105150=B_SPLINE_CURVE_WITH_KNOTS ( 'NONE', 3,
 ( #49608, #38426, #4823, #30584, #82081, #5385, #100537, #98335, #39542, #74809, #89933, #58009, #66421, #64213, #13210, #73716 ),
 .UNSPECIFIED., .F., .F.,
 ( 4, 3, 3, 3, 3, 4 ),
 ( -7.276681342242609318, -6.842771595400160223, -5.875983249300730016, -4.912620469295280401, -3.950810556825589792, -2.991101461899999592 ),
 .UNSPECIFIED. ) ;
#105153=CARTESIAN_POINT ( 'NONE',  ( 9.014562907850001139, 1470.471472073790210, 213.7600426553289878 ) ) ;
#105159=CARTESIAN_POINT ( 'NONE',  ( 8.977976324442520806, 1435.738830198290088, 208.3991943294609825 ) ) ;
#105163=B_SPLINE_CURVE_WITH_KNOTS ( 'NONE', 3,
 ( #64532, #21913, #56109, #90241, #13523, #19742 ),
 .UNSPECIFIED., .F., .F.,
 ( 4, 2, 4 ),
 ( 0.000000000000000000, 0.5000000000000000000, 1.000000000000000000 ),
 .UNSPECIFIED. ) ;
#105165=CARTESIAN_POINT ( 'NONE',  ( 1.657276590850500053, 1467.004937341380128, 220.0645755171550206 ) ) ;
#105168=CARTESIAN_POINT ( 'NONE',  ( 9.949026363403810080, 1472.637006744650307, 191.3883391339116997 ) ) ;
#105176=EDGE_CURVE ( 'NONE', #26525, #32787, #71308, .T. ) ;
#105192=CARTESIAN_POINT ( 'NONE',  ( 15.00046832902299876, 1429.237668425022093, 197.8089893366197884 ) ) ;
#105200=CARTESIAN_POINT ( 'NONE',  ( -6.025152189795589308, 1484.743689720570046, 198.8560543189699956 ) ) ;
#105205=CARTESIAN_POINT ( 'NONE',  ( -4.328687482160670008, 1515.093865522939950, 207.9272901344760101 ) ) ;
#105212=LINE ( 'NONE', #11698, #76056 ) ;
#105215=CARTESIAN_POINT ( 'NONE',  ( 10.01437067453739971, 1462.389803450230147, 210.8954083920299922 ) ) ;
#105217=CARTESIAN_POINT ( 'NONE',  ( -1.063750041850000105, 1443.513882422190136, 200.1423802087390129 ) ) ;
#105221=CARTESIAN_POINT ( 'NONE',  ( -16.00178234999744831, 1420.236353625467927, 209.6595671161338714 ) ) ;
#105224=CARTESIAN_POINT ( 'NONE',  ( -3.961741473678640268, 1508.551704408789874, 204.5769763901439831 ) ) ;
#105226=CARTESIAN_POINT ( 'NONE',  ( 2201.413669186790685, 11221.53578756870047, -1523.112345774690311 ) ) ;
#105228=CARTESIAN_POINT ( 'NONE',  ( -4.836530696830000586, 1489.194118352389751, 188.8927898524989928 ) ) ;
#105229=VERTEX_POINT ( 'NONE', #102156 ) ;
#105234=ORIENTED_EDGE ( 'NONE', *, *, #95918, .T. ) ;
#105235=CARTESIAN_POINT ( 'NONE',  ( -7.107506042044070327, 1508.551704404740121, 219.1601581955270035 ) ) ;
#105240=CARTESIAN_POINT ( 'NONE',  ( -0.2964941798090010017, 1431.756287522389812, 218.2392599841689957 ) ) ;
#105241=CARTESIAN_POINT ( 'NONE',  ( -11.16643434163729864, 1471.372555858320084, 206.7508257846899937 ) ) ;
#105247=CARTESIAN_POINT ( 'NONE',  ( 10.79340562696630101, 1490.084803914939812, 207.2635531919679863 ) ) ;
#105249=ORIENTED_EDGE ( 'NONE', *, *, #50885, .F. ) ;
#105252=CARTESIAN_POINT ( 'NONE',  ( 0.3222616711803319989, 1496.639296058219998, 196.7583996707039944 ) ) ;
#105254=CARTESIAN_POINT ( 'NONE',  ( 11.60812525217539992, 1427.544186611749865, 209.2289499687080081 ) ) ;
#105261=AXIS2_PLACEMENT_3D ( 'NONE', #32401, #65473, #99582 ) ;
#105264=CARTESIAN_POINT ( 'NONE',  ( -0.8045663272259990784, 1496.574851711289966, 197.1535040705990127 ) ) ;
#105268=ORIENTED_EDGE ( 'NONE', *, *, #23308, .F. ) ;
#105269=ADVANCED_FACE ( 'NONE', ( #20360 ), #34709, .T. ) ;
#105298=B_SPLINE_CURVE_WITH_KNOTS ( 'NONE', 3,
 ( #28708, #20285, #69636, #62913, #37102, #27600, #71302, #61784, #95908, #105416, #63445, #20836, #103759, #27060, #10243, #97024, #44419, #79129, #19169, #36552, #91900, #65627, #100308, #39302 ),
 .UNSPECIFIED., .F., .F.,
 ( 4, 2, 1, 1, 2, 2, 2, 2, 2, 1, 1, 2, 2, 4 ),
 ( 0.000000000000000000, 0.1249999999998059053, 0.1874999999996863065, 0.2187499999996492805, 0.2343749999996534994, 0.2499999999996577182, 0.3749999999996929123, 0.4999999999997282174, 0.6249999999997635225, 0.6874999999997812861, 0.7187499999997918332, 0.7343749999997692957, 0.7499999999997467581, 1.000000000000000000 ),
 .UNSPECIFIED. ) ;
#105299=CARTESIAN_POINT ( 'NONE',  ( 2.330134126090000368, 1515.064792882589927, 213.4512947377390049 ) ) ;
#105301=ORIENTED_EDGE ( 'NONE', *, *, #90717, .F. ) ;
#105310=CARTESIAN_POINT ( 'NONE',  ( 5.216739650425079589, 1497.653660005760230, 197.6765241825160047 ) ) ;
#105311=CARTESIAN_POINT ( 'NONE',  ( -4.275310502956699565, 1469.420104164370059, 218.4212499309419968 ) ) ;
#105315=CARTESIAN_POINT ( 'NONE',  ( -12.78813129401979864, 1502.651454227029944, 209.2144374427170135 ) ) ;
#105316=CARTESIAN_POINT ( 'NONE',  ( -2.369178030186009920, 1422.130784306599935, 193.0786739971210011 ) ) ;
#105319=CARTESIAN_POINT ( 'NONE',  ( -12.78085885379999986, 1502.746248514790068, 208.8788078008309981 ) ) ;
#105320=FACE_OUTER_BOUND ( 'NONE', #74733, .T. ) ;
#105324=ORIENTED_EDGE ( 'NONE', *, *, #17858, .F. ) ;
#105329=B_SPLINE_SURFACE_WITH_KNOTS ( 'NONE', 5, 5, ( 
 ( #109685, #93974, #92873, #50354, #84479, #36284 ),
 ( #70476, #1055, #22073, #29946, #56268, #104596 ),
 ( #11105, #53674, #78862, #2169, #27890, #9981 ),
 ( #35180, #21528, #90397, #69925, #38892, #44710 ),
 ( #89862, #55742, #106656, #62073, #64692, #81439 ),
 ( #30503, #87818, #96199, #77745, #19474, #45266 ),
 ( #79405, #86687, #107215, #4750, #52553, #47315 ),
 ( #69365, #2716, #95643, #73075, #98811, #36839 ),
 ( #103474, #10536, #43594, #13131, #26780, #72526 ) ),
 .UNSPECIFIED., .F., .F., .F.,
 ( 6, 3, 6 ),
 ( 6, 6 ),
 ( 4.387253917325519836, 7.393604636469999214, 10.39995535562450080 ),
 ( -0.001720784224481730022, 1.000000000000000000 ),
 .UNSPECIFIED. ) ;
#105331=CARTESIAN_POINT ( 'NONE',  ( 4.498501936019999370, 1505.761609765590038, 220.2758765865989972 ) ) ;
#105334=CARTESIAN_POINT ( 'NONE',  ( -16.76766723949620186, 1420.018926319380171, 208.3735033652980064 ) ) ;
#105336=CARTESIAN_POINT ( 'NONE',  ( -17.24222792867009701, 1417.941613371040148, 205.1746868673990036 ) ) ;
#105338=TOROIDAL_SURFACE ( 'NONE', #40983, 11.23850026409999892, 0.5000000000000000000 ) ;
#105339=VECTOR ( 'NONE', #109567, 1000.000000000000114 ) ;
#105341=CARTESIAN_POINT ( 'NONE',  ( -6.409211830000000276, 1460.447398049189815, 209.7327255955039789 ) ) ;
#105348=CARTESIAN_POINT ( 'NONE',  ( -5.594770757790000992, 1475.752789105589954, 217.8971188394789920 ) ) ;
#105363=CARTESIAN_POINT ( 'NONE',  ( -15.41720089870000088, 1415.311335408779769, 208.7885211753810211 ) ) ;
#105366=CARTESIAN_POINT ( 'NONE',  ( 4.563201210870380109, 1455.845590638939939, 218.7168878893969861 ) ) ;
#105373=CARTESIAN_POINT ( 'NONE',  ( -9.134867208606445743, 1469.981975463268327, 191.1356054705261158 ) ) ;
#105374=ORIENTED_EDGE ( 'NONE', *, *, #79593, .T. ) ;
#105375=CARTESIAN_POINT ( 'NONE',  ( -5.302697812188962523, 1464.205369536075750, 199.9536599677759057 ) ) ;
#105378=CARTESIAN_POINT ( 'NONE',  ( -11.67232828841030035, 1481.221314557019923, 211.0847665075339989 ) ) ;
#105387=CARTESIAN_POINT ( 'NONE',  ( -6.910348952263761113, 1496.006749978269909, 200.2510802398396379 ) ) ;
#105392=CARTESIAN_POINT ( 'NONE',  ( 1.773850233349999916, 1423.360122320810206, 192.5455093738989945 ) ) ;
#105396=CARTESIAN_POINT ( 'NONE',  ( 10.53029073209870070, 1452.309494521090073, 190.1435485275030146 ) ) ;
#105402=CARTESIAN_POINT ( 'NONE',  ( -1970.025574498409924, -8382.262153571269664, 5.165967170900809258 ) ) ;
#105408=CARTESIAN_POINT ( 'NONE',  ( -9.253356380629998768, 1423.298286757820051, 209.1001181959080100 ) ) ;
#105410=CARTESIAN_POINT ( 'NONE',  ( -10.77418843618166377, 1422.305283220386627, 210.6378112949979311 ) ) ;
#105415=EDGE_LOOP ( 'NONE', ( #65908, #18427, #64293, #46893 ) ) ;
#105416=CARTESIAN_POINT ( 'NONE',  ( -0.2829287784654356819, 1457.550022606329549, 199.5929807864239081 ) ) ;
#105429=CARTESIAN_POINT ( 'NONE',  ( -5.778791999094319287, 1426.204447263729890, 207.0106680037629872 ) ) ;
#105432=CARTESIAN_POINT ( 'NONE',  ( -9.299436816969999242, 1446.922293007090275, 190.6945112479990030 ) ) ;
#105434=CARTESIAN_POINT ( 'NONE',  ( -1.318899170704230128, 1431.696355161669999, 200.8232092877559865 ) ) ;
#105437=ORIENTED_EDGE ( 'NONE', *, *, #66749, .T. ) ;
#105442=CARTESIAN_POINT ( 'NONE',  ( 3.156336099161360043, 1466.261550192479945, 198.5320301967060175 ) ) ;
#105446=CARTESIAN_POINT ( 'NONE',  ( 3.153087606539999754, 1465.853416239390071, 199.3411100570189944 ) ) ;
#105457=CARTESIAN_POINT ( 'NONE',  ( 21.14415186440000127, 1497.093961449289964, 210.1561521351690089 ) ) ;
#105458=CARTESIAN_POINT ( 'NONE',  ( 19.52205342210000083, 1473.076230373790168, 204.3554439105789982 ) ) ;
#105459=CARTESIAN_POINT ( 'NONE',  ( -7.993033103293710084, 1436.236666033240226, 214.7384163211640100 ) ) ;
#105463=CARTESIAN_POINT ( 'NONE',  ( -6.814218036220000663, 1508.185726375689910, 220.1716981485990061 ) ) ;
#105466=CARTESIAN_POINT ( 'NONE',  ( 5.423836325560000837, 1437.243905350390150, 208.3828194269840139 ) ) ;
#105470=CARTESIAN_POINT ( 'NONE',  ( -1.975340820460000257, 1463.175830154689947, 228.7200063650990103 ) ) ;
#105481=CARTESIAN_POINT ( 'NONE',  ( -2.298816259811510054, 1486.462377102800019, 220.8289805423670202 ) ) ;
#105482=FACE_OUTER_BOUND ( 'NONE', #10897, .T. ) ;
#105487=CARTESIAN_POINT ( 'NONE',  ( -8.790791811524689692, 1448.890444021340045, 211.6766362075580048 ) ) ;
#105492=CARTESIAN_POINT ( 'NONE',  ( 1.094850995720000109, 1515.349842019790003, 213.4046786226089978 ) ) ;
#105493=EDGE_CURVE ( 'NONE', #92278, #55998, #87318, .T. ) ;
#105502=CARTESIAN_POINT ( 'NONE',  ( 0.5599827605490009796, 1431.620283137290016, 200.5991563158890187 ) ) ;
#105506=CARTESIAN_POINT ( 'NONE',  ( 3.628818058489999832, 1505.602008442089982, 221.3635114687990040 ) ) ;
#105507=CARTESIAN_POINT ( 'NONE',  ( -4.038582018749999669, 1515.598601288590089, 209.4984326820579952 ) ) ;
#105512=CARTESIAN_POINT ( 'NONE',  ( 9.473794194718619721, 1468.306494430019939, 205.7209031666899648 ) ) ;
#105516=LINE ( 'NONE', #71400, #32391 ) ;
#105524=B_SPLINE_CURVE_WITH_KNOTS ( 'NONE', 3,
 ( #48578, #82713, #50232, #91659, #40154, #108465, #14934, #74337, #31747, #65934, #67584, #50764, #390, #35059, #103349, #16568, #60850, #101690, #103921, #93306, #75964, #84899 ),
 .UNSPECIFIED., .F., .F.,
 ( 4, 3, 3, 3, 3, 3, 3, 4 ),
 ( -7.359819275554579932, -7.141305509537970053, -6.026261691904320372, -5.186741713040009749, -5.022423404310830009, -4.324046055999499316, -3.608772125771039896, -3.013663444789999701 ),
 .UNSPECIFIED. ) ;
#105529=CARTESIAN_POINT ( 'NONE',  ( -11.36125419377996515, 1501.596596453163556, 207.6628600452400804 ) ) ;
#105530=CARTESIAN_POINT ( 'NONE',  ( -15.59606447164447651, 1415.961119725337312, 208.0309741868692299 ) ) ;
#105537=CARTESIAN_POINT ( 'NONE',  ( -9.064953078289999411, 1451.258683735890145, 206.8358752714689786 ) ) ;
#105540=CARTESIAN_POINT ( 'NONE',  ( 7.699283328289999950, 1425.052167582540051, 211.8716563696589787 ) ) ;
#105547=CARTESIAN_POINT ( 'NONE',  ( 7.213645968120000695, 1453.321438162990034, 215.1620360656989988 ) ) ;
#105560=CARTESIAN_POINT ( 'NONE',  ( -2.130922739038390024, 1467.954349360780043, 220.0452206896550251 ) ) ;
#105580=EDGE_CURVE ( 'NONE', #54152, #35149, #93833, .T. ) ;
#105594=CARTESIAN_POINT ( 'NONE',  ( 3.007039660992123942, 1441.535621290770678, 218.1727171084023382 ) ) ;
#105602=CARTESIAN_POINT ( 'NONE',  ( 9.967911316253610821, 1425.849184522710175, 194.0881941884150024 ) ) ;
#105603=CARTESIAN_POINT ( 'NONE',  ( 19.38665828288160142, 1498.812007524589944, 221.8202318911040152 ) ) ;
#105609=ORIENTED_EDGE ( 'NONE', *, *, #93194, .T. ) ;
#105631=CARTESIAN_POINT ( 'NONE',  ( 0.07018038471609880369, 1442.854703621289900, 218.7250898028690074 ) ) ;
#105638=CARTESIAN_POINT ( 'NONE',  ( -4.890969413286970102, 1464.492716438699972, 199.2455826196770090 ) ) ;
#105642=CARTESIAN_POINT ( 'NONE',  ( -9.983709645732758986, 1472.259764172770019, 211.0763333463989966 ) ) ;
#105645=CARTESIAN_POINT ( 'NONE',  ( -14.53800271749999951, 1508.448877354789829, 216.0591006970490184 ) ) ;
#105652=DIRECTION ( 'NONE',  ( 0.3096375404471009563, -0.4473880807146179417, -0.8390283063045967937 ) ) ;
#105657=CARTESIAN_POINT ( 'NONE',  ( -8.181710101844450023, 1488.271543501559790, 217.5078058625639983 ) ) ;
#105658=CARTESIAN_POINT ( 'NONE',  ( -16.53114558859999761, 1465.611456236089907, 220.7423132190989747 ) ) ;
#105661=( BOUNDED_CURVE ( )  B_SPLINE_CURVE ( 3, ( #67657, #29753, #48790, #57193 ),
 .UNSPECIFIED., .F., .F. ) 
 B_SPLINE_CURVE_WITH_KNOTS ( ( 4, 4 ),
 ( 1.025211572815232008, 1.340431719809825895 ),
 .UNSPECIFIED. ) 
 CURVE ( )  GEOMETRIC_REPRESENTATION_ITEM ( )  RATIONAL_B_SPLINE_CURVE ( ( 1.000000000000000000, 0.9917368149478550388, 0.9917368149478550388, 1.000000000000000000 ) ) 
 REPRESENTATION_ITEM ( '' )  );
#105662=CARTESIAN_POINT ( 'NONE',  ( 8.051687730190000281, 1428.206419125489901, 213.2401846629289821 ) ) ;
#105663=CARTESIAN_POINT ( 'NONE',  ( 9.374720191569998917, 1498.531797635389921, 228.6938383677990316 ) ) ;
#105677=CARTESIAN_POINT ( 'NONE',  ( 2.087496205359999912, 1487.118434918990033, 216.9290059995090019 ) ) ;
#105681=CARTESIAN_POINT ( 'NONE',  ( -1.201530806679770080, 1515.093215458460008, 213.4505504663210047 ) ) ;
#105684=CARTESIAN_POINT ( 'NONE',  ( -4.329112086532120429, 1476.833686876630054, 219.7848579265929914 ) ) ;
#105688=CARTESIAN_POINT ( 'NONE',  ( 1.959285284397550120, 1474.800623515119923, 220.3715842348549927 ) ) ;
#105689=ORIENTED_EDGE ( 'NONE', *, *, #90299, .F. ) ;
#105691=CARTESIAN_POINT ( 'NONE',  ( -13.54199508319999978, 1506.857021832190185, 209.2226570286780145 ) ) ;
#105692=CARTESIAN_POINT ( 'NONE',  ( 9.839796275310359164, 1492.609014552419922, 188.3573332966260239 ) ) ;
#105698=CARTESIAN_POINT ( 'NONE',  ( 4.328264056533019932, 1515.110035495290049, 210.1077469519609906 ) ) ;
#105699=CARTESIAN_POINT ( 'NONE',  ( 3.824257248145499943, 1484.587375475480030, 220.3370414412930245 ) ) ;
#105701=CARTESIAN_POINT ( 'NONE',  ( -10.48877660729999839, 1461.381695361490074, 212.5316338973990185 ) ) ;
#105704=ORIENTED_EDGE ( 'NONE', *, *, #28969, .F. ) ;
#105712=CARTESIAN_POINT ( 'NONE',  ( 2.220665158331510014, 1495.679845400359909, 221.2599143071639958 ) ) ;
#105715=B_SPLINE_CURVE_WITH_KNOTS ( 'NONE', 5,
 ( #83075, #33212, #24254, #92026, #76329, #58989 ),
 .UNSPECIFIED., .F., .F.,
 ( 6, 6 ),
 ( 0.000000000000000000, 1.000000000000000000 ),
 .UNSPECIFIED. ) ;
#105717=TOROIDAL_SURFACE ( 'NONE', #82451, 8.800000000000000711, 1.000000000000000000 ) ;
#105718=DIRECTION ( 'NONE',  ( 2.041467857569999829E-16, -1.000000000000000000, 5.573852046271030309E-16 ) ) ;
#105719=CARTESIAN_POINT ( 'NONE',  ( -9.934732886592909651, 1439.684679282129991, 207.9389421599310026 ) ) ;
#105720=ORIENTED_EDGE ( 'NONE', *, *, #97304, .F. ) ;
#105726=VERTEX_POINT ( 'NONE', #45751 ) ;
#105729=CARTESIAN_POINT ( 'NONE',  ( -1.565479927690150097, 1467.839058700010128, 220.1279929306939778 ) ) ;
#105733=DIRECTION ( 'NONE',  ( 0.4436356471204865315, 1.250495761681361773E-32, 0.8962072375315807138 ) ) ;
#105740=CARTESIAN_POINT ( 'NONE',  ( -2.918137311410000212, 1438.508781642889971, 227.5106010738990108 ) ) ;
#105752=CARTESIAN_POINT ( 'NONE',  ( 10.27511161340000001, 1489.668981243689814, 204.7180042823989936 ) ) ;
#105758=CARTESIAN_POINT ( 'NONE',  ( -17.09418616900000032, 1417.376006423840181, 206.9664283537690039 ) ) ;
#105768=ADVANCED_FACE ( 'NONE', ( #28369 ), #91857, .F. ) ;
#105769=DIRECTION ( 'NONE',  ( 0.000000000000000000, 0.000000000000000000, 1.000000000000000000 ) ) ;
#105770=CARTESIAN_POINT ( 'NONE',  ( -9.519777939162850089, 1460.017017711900053, 210.6312322783699926 ) ) ;
#105786=CARTESIAN_POINT ( 'NONE',  ( -2.487920634212330118, 1508.551704408389924, 204.1347675177020164 ) ) ;
#105793=VECTOR ( 'NONE', #85893, 1000.000000000000000 ) ;
#105797=ORIENTED_EDGE ( 'NONE', *, *, #42568, .T. ) ;
#105798=CARTESIAN_POINT ( 'NONE',  ( 10.99044919668839881, 1479.494726248550023, 229.8297398567180210 ) ) ;
#105800=( BOUNDED_CURVE ( )  B_SPLINE_CURVE ( 3, ( #18571, #104811, #52766, #86905 ),
 .UNSPECIFIED., .F., .T. ) 
 B_SPLINE_CURVE_WITH_KNOTS ( ( 4, 4 ),
 ( 1.021828243325141994, 2.119764315462445037 ),
 .UNSPECIFIED. ) 
 CURVE ( )  GEOMETRIC_REPRESENTATION_ITEM ( )  RATIONAL_B_SPLINE_CURVE ( ( 1.000000000000000000, 0.9020423082557569305, 0.9020423082557569305, 1.000000000000000000 ) ) 
 REPRESENTATION_ITEM ( '' )  );
#105805=CARTESIAN_POINT ( 'NONE',  ( -1.233464473149999963, 1431.858984285389852, 217.8324935667789930 ) ) ;
#105806=CARTESIAN_POINT ( 'NONE',  ( -10.21667613351959858, 1472.322293331309993, 207.1512473758539841 ) ) ;
#105814=CARTESIAN_POINT ( 'NONE',  ( 11.88070671566089942, 1491.927040624079837, 209.1634875332829893 ) ) ;
#105815=ORIENTED_EDGE ( 'NONE', *, *, #92146, .T. ) ;
#105819=CARTESIAN_POINT ( 'NONE',  ( 2.350390795498939589, 1497.086630012390287, 196.9446188252720162 ) ) ;
#105831=CARTESIAN_POINT ( 'NONE',  ( 2.144608228480000101, 1498.044160227690099, 197.8976463139989903 ) ) ;
#105835=CARTESIAN_POINT ( 'NONE',  ( 7.571416212307459759, 1423.019345442000031, 195.7264161909869813 ) ) ;
#105851=CARTESIAN_POINT ( 'NONE',  ( 4.997202291739998969, 1423.732852402740264, 194.0938664950990074 ) ) ;
#105852=VERTEX_POINT ( 'NONE', #30851 ) ;
#105853=AXIS2_PLACEMENT_3D ( 'NONE', #110481, #68504, #67956 ) ;
#105855=CARTESIAN_POINT ( 'NONE',  ( -5.812939435032099311, 1419.537318060671623, 194.8608174217619649 ) ) ;
#105863=ORIENTED_EDGE ( 'NONE', *, *, #44902, .T. ) ;
#105872=FACE_OUTER_BOUND ( 'NONE', #4326, .T. ) ;
#105873=CARTESIAN_POINT ( 'NONE',  ( -8.603211701180001114, 1469.317673379189955, 216.5015782100589945 ) ) ;
#105880=CARTESIAN_POINT ( 'NONE',  ( -13.39453303099999992, 1503.483788606090002, 208.7029727493389828 ) ) ;
#105882=CARTESIAN_POINT ( 'NONE',  ( 11.70359515955249918, 1422.053249383299999, 207.2442419415079655 ) ) ;
#105893=CARTESIAN_POINT ( 'NONE',  ( -14.77171694839999994, 1415.677402209299999, 212.1703745851490055 ) ) ;
#105895=CARTESIAN_POINT ( 'NONE',  ( -15.77795547941580168, 1420.228508977689899, 210.6635392844780199 ) ) ;
#105896=VERTEX_POINT ( 'NONE', #64492 ) ;
#105897=CARTESIAN_POINT ( 'NONE',  ( -15.88245123595834585, 1415.955066226697454, 209.7358280198473039 ) ) ;
#105900=CARTESIAN_POINT ( 'NONE',  ( 1.069043333538070017, 1430.790655322590055, 199.7345386470830135 ) ) ;
#105905=CARTESIAN_POINT ( 'NONE',  ( 7.914828484685850540, 1459.913996726710138, 203.2501674748179994 ) ) ;
#105908=CARTESIAN_POINT ( 'NONE',  ( -5.463886630600000238, 1476.963513525689905, 218.4976191159190080 ) ) ;
#105935=CARTESIAN_POINT ( 'NONE',  ( -13.59236974158869948, 1508.248953138170009, 209.5387658739280141 ) ) ;
#105952=DIRECTION ( 'NONE',  ( 0.1425040565888799349, 0.3680151204241798868, -0.9188348409779036885 ) ) ;
#105957=CARTESIAN_POINT ( 'NONE',  ( 19.11847670520000264, 1460.287704656489950, 220.2677159749989926 ) ) ;
#105970=CARTESIAN_POINT ( 'NONE',  ( -8.316672828268760753, 1425.055149638239982, 204.9623390585310005 ) ) ;
#105974=ORIENTED_EDGE ( 'NONE', *, *, #79453, .T. ) ;
#105976=ORIENTED_EDGE ( 'NONE', *, *, #50233, .T. ) ;
#105986=CARTESIAN_POINT ( 'NONE',  ( 12.54808185004130117, 1501.100271328960162, 211.1771682979919831 ) ) ;
#105991=CARTESIAN_POINT ( 'NONE',  ( -9.771935530151019123, 1448.872218581839888, 190.8346833224969998 ) ) ;
#106000=CARTESIAN_POINT ( 'NONE',  ( 9.855320986769999791, 1462.478457361989967, 210.0130851932640041 ) ) ;
#106003=CARTESIAN_POINT ( 'NONE',  ( -0.4967503101659990206, 1463.947305906790007, 199.2992579264090125 ) ) ;
#106014=CARTESIAN_POINT ( 'NONE',  ( -17.47298132753811117, 1508.456142919008016, 212.6551300565776899 ) ) ;
#106016=DIRECTION ( 'NONE',  ( -1.000000000000000000, -2.249639673992789970E-32, -1.224646799147350002E-16 ) ) ;
#106017=CARTESIAN_POINT ( 'NONE',  ( -6.052777691587611031, 1434.867522108110052, 216.6696794239180122 ) ) ;
#106021=CARTESIAN_POINT ( 'NONE',  ( -7.239307611560000133, 1509.020652858989934, 218.9550108994890252 ) ) ;
#106023=CARTESIAN_POINT ( 'NONE',  ( 18.14949073579999705, 1432.344282874789997, 211.8258969992290019 ) ) ;
#106027=CARTESIAN_POINT ( 'NONE',  ( 3.101757698284638209, 1466.831514544163610, 219.0062985612876503 ) ) ;
#106031=CARTESIAN_POINT ( 'NONE',  ( -2.218918642439999811, 1431.115532562089811, 203.8893404030790180 ) ) ;
#106036=CARTESIAN_POINT ( 'NONE',  ( -14.61826233789999918, 1415.850734755279973, 204.4424076310489795 ) ) ;
#106041=CARTESIAN_POINT ( 'NONE',  ( -10.29850490222790071, 1448.590037845560119, 207.7852207394710149 ) ) ;
#106043=VERTEX_POINT ( 'NONE', #74536 ) ;
#106046=CARTESIAN_POINT ( 'NONE',  ( 1.118758552039999854, 1515.569725561690120, 213.0929468739089714 ) ) ;
#106048=CARTESIAN_POINT ( 'NONE',  ( -0.8391973868109434687, 1463.415940303041452, 199.3702334271763164 ) ) ;
#106050=CARTESIAN_POINT ( 'NONE',  ( -9.996566840449769842, 1446.992630724909986, 211.6934593223399759 ) ) ;
#106051=CARTESIAN_POINT ( 'NONE',  ( -3.220674670777950332, 1433.265635011049881, 218.1214075741529825 ) ) ;
#106052=CARTESIAN_POINT ( 'NONE',  ( 0.3109538050990010016, 1430.738335933489907, 200.0544679982990033 ) ) ;
#106056=VERTEX_POINT ( 'NONE', #63940 ) ;
#106058=CARTESIAN_POINT ( 'NONE',  ( 11.13982123801030077, 1470.272549761619985, 206.9150573627110248 ) ) ;
#106064=CARTESIAN_POINT ( 'NONE',  ( 12.15645370196850017, 1491.542819424739946, 207.2681566586209954 ) ) ;
#106065=CARTESIAN_POINT ( 'NONE',  ( -10.12198797759999991, 1482.055157405490036, 205.4868429776790038 ) ) ;
#106071=CARTESIAN_POINT ( 'NONE',  ( -11.40679451554845336, 1501.041746466157065, 208.3891828855351491 ) ) ;
#106073=CARTESIAN_POINT ( 'NONE',  ( -5.144873395449999443, 1502.885538352589947, 229.8910404859989853 ) ) ;
#106079=ADVANCED_FACE ( 'NONE', ( #108667 ), #94609, .T. ) ;
#106081=CARTESIAN_POINT ( 'NONE',  ( 7.490627823309999656, 1426.027613909420097, 212.3458724979089709 ) ) ;
#106082=CARTESIAN_POINT ( 'NONE',  ( 13.84583145400000070, 1499.900106662689723, 227.7510597354990125 ) ) ;
#106088=CARTESIAN_POINT ( 'NONE',  ( 3.313501335607582643, 1397.551704408390151, 215.1871694724064810 ) ) ;
#106090=ORIENTED_EDGE ( 'NONE', *, *, #51843, .F. ) ;
#106096=CARTESIAN_POINT ( 'NONE',  ( -21.50860586580829903, 1505.511036766189818, 209.4816256532819807 ) ) ;
#106106=EDGE_LOOP ( 'NONE', ( #30755, #92732, #35035, #58865, #58016 ) ) ;
#106115=B_SPLINE_SURFACE_WITH_KNOTS ( 'NONE', 5, 5, ( 
 ( #53870, #53300, #46552, #79600, #36474, #70672 ),
 ( #80687, #44343, #62833, #3998, #26982, #96947 ),
 ( #61171, #95286, #18548, #10170, #78486, #1800 ),
 ( #35937, #95829, #5068, #72305, #81219, #31369 ),
 ( #22390, #90724, #57158, #64995, #13446, #29720 ),
 ( #74505, #30818, #47637, #90165, #82334, #108634 ) ),
 .UNSPECIFIED., .F., .F., .F.,
 ( 6, 6 ),
 ( 6, 6 ),
 ( 10.65476131940000037, 18.78936860560000000 ),
 ( 0.000000000000000000, 0.5000000000000000000 ),
 .UNSPECIFIED. ) ;
#106119=ADVANCED_FACE ( 'NONE', ( #65026 ), #14950, .T. ) ;
#106120=EDGE_CURVE ( 'NONE', #53131, #100441, #32501, .T. ) ;
#106121=ADVANCED_FACE ( 'NONE', ( #66693 ), #93682, .T. ) ;
#106124=CARTESIAN_POINT ( 'NONE',  ( -12.18560036526529977, 1490.059793347699951, 210.2795501257769786 ) ) ;
#106125=EDGE_CURVE ( 'NONE', #79128, #103755, #20117, .T. ) ;
#106130=ORIENTED_EDGE ( 'NONE', *, *, #94794, .F. ) ;
#106134=CARTESIAN_POINT ( 'NONE',  ( 18.51068734469999910, 1475.362681785890118, 218.3399159096489939 ) ) ;
#106140=CARTESIAN_POINT ( 'NONE',  ( 14.99555783611850046, 1427.394895963429917, 198.9768735146830068 ) ) ;
#106141=CARTESIAN_POINT ( 'NONE',  ( -18.80013642706989785, 1505.319320522869930, 222.5373253066319990 ) ) ;
#106148=ORIENTED_EDGE ( 'NONE', *, *, #23577, .T. ) ;
#106150=CARTESIAN_POINT ( 'NONE',  ( -2.634252018550000241, 1429.123518628689908, 200.1269094519890075 ) ) ;
#106153=CARTESIAN_POINT ( 'NONE',  ( -3.562576982599999997, 1500.604443063090002, 230.1476615162989958 ) ) ;
#106155=CARTESIAN_POINT ( 'NONE',  ( 20.21728935790000037, 1475.862786327189951, 209.1218459616989946 ) ) ;
#106159=CARTESIAN_POINT ( 'NONE',  ( -16.43661047864564040, 1416.852979121301360, 207.9780681923153338 ) ) ;
#106161=CARTESIAN_POINT ( 'NONE',  ( 9.923128685616420697, 1469.055232010309965, 207.6288126312279871 ) ) ;
#106164=CARTESIAN_POINT ( 'NONE',  ( 10.40804279477580074, 1480.934692010039953, 207.3742714289850255 ) ) ;
#106168=CARTESIAN_POINT ( 'NONE',  ( 8.179170872261016356, 1424.126445343982823, 195.8532290842973680 ) ) ;
#106169=CARTESIAN_POINT ( 'NONE',  ( -0.5923098205000010275, 1443.101676972689802, 218.7159598536189833 ) ) ;
#106174=CARTESIAN_POINT ( 'NONE',  ( -19.58905257500000019, 1465.550414696789858, 206.2240342260589898 ) ) ;
#106176=CARTESIAN_POINT ( 'NONE',  ( 7.407046107680000269, 1488.581653516390134, 199.5623810922690211 ) ) ;
#106180=CARTESIAN_POINT ( 'NONE',  ( -9.103468112560660686, 1449.499701819690017, 210.3008494512589834 ) ) ;
#106183=CARTESIAN_POINT ( 'NONE',  ( 11.24351695115020000, 1470.448214870340053, 207.4320293865459917 ) ) ;
#106184=CARTESIAN_POINT ( 'NONE',  ( -2.812370349340000519, 1484.074845783890169, 198.7990170648990045 ) ) ;
#106185=CARTESIAN_POINT ( 'NONE',  ( -15.77133272873888714, 1418.153095964348040, 203.3734822495675019 ) ) ;
#106189=CARTESIAN_POINT ( 'NONE',  ( 5.063479484552349419, 1494.517360836430043, 219.5241837424580353 ) ) ;
#106190=CARTESIAN_POINT ( 'NONE',  ( -10.25580389252270130, 1489.562374261269724, 214.0502075833479978 ) ) ;
#106191=CARTESIAN_POINT ( 'NONE',  ( -20.43379408400000230, 1466.940146741789931, 211.2182734472289951 ) ) ;
#106194=CARTESIAN_POINT ( 'NONE',  ( 6.200611228269999664, 1427.799628982990043, 214.6497469830689795 ) ) ;
#106195=CARTESIAN_POINT ( 'NONE',  ( 1.026847439679999807, 1494.050500615490137, 217.3813169612789977 ) ) ;
#106206=CARTESIAN_POINT ( 'NONE',  ( 9.273082254300890170, 1436.468110177680273, 210.7387439683169816 ) ) ;
#106211=CARTESIAN_POINT ( 'NONE',  ( 7.147354835452560451, 1466.396680852790041, 215.9969464199629954 ) ) ;
#106215=CARTESIAN_POINT ( 'NONE',  ( 1.351910739691850161, 1515.082829241050149, 213.4508224384909738 ) ) ;
#106217=CARTESIAN_POINT ( 'NONE',  ( -9.137858907971150302, 1479.061965924570131, 216.3904244229409812 ) ) ;
#106223=CARTESIAN_POINT ( 'NONE',  ( -17.72465096253550243, 1488.214251129269996, 195.0958863970620030 ) ) ;
#106227=DIRECTION ( 'NONE',  ( 1.224646799147350002E-16, -1.836970198721029688E-16, -1.000000000000000000 ) ) ;
#106241=CARTESIAN_POINT ( 'NONE',  ( -9.413255646274679478, 1447.050163675619842, 212.1529317657590070 ) ) ;
#106246=B_SPLINE_SURFACE_WITH_KNOTS ( 'NONE', 5, 5, ( 
 ( #7682, #6588, #24466, #8771, #33417, #84395 ),
 ( #67065, #41839, #93881, #85473, #23913, #32345 ),
 ( #25015, #67613, #42953, #75994, #101171, #15511 ),
 ( #101725, #77113, #16063, #74912, #58108, #51339 ),
 ( #58655, #32876, #110144, #420, #8220, #50266 ),
 ( #68179, #68722, #26119, #50796, #59216, #42386 ) ),
 .UNSPECIFIED., .F., .F., .F.,
 ( 6, 6 ),
 ( 6, 6 ),
 ( 28.60746992390000187, 29.16358567150000169 ),
 ( 106.3256099500000005, 116.2484248749999978 ),
 .UNSPECIFIED. ) ;
#106247=ORIENTED_EDGE ( 'NONE', *, *, #106934, .F. ) ;
#106262=CARTESIAN_POINT ( 'NONE',  ( 11.32255167084790060, 1471.391268690820198, 210.6326086776350053 ) ) ;
#106266=CARTESIAN_POINT ( 'NONE',  ( -3.750000000000000000, 1512.051704408390151, 209.1218459616989946 ) ) ;
#106272=VERTEX_POINT ( 'NONE', #63804 ) ;
#106276=CARTESIAN_POINT ( 'NONE',  ( 0.7162863658319988946, 1429.709265593189912, 217.4063670190490143 ) ) ;
#106284=EDGE_CURVE ( 'NONE', #55990, #15017, #68618, .T. ) ;
#106288=ADVANCED_FACE ( 'NONE', ( #48092 ), #49874, .T. ) ;
#106304=CYLINDRICAL_SURFACE ( 'NONE', #19765, 0.4999999999999909517 ) ;
#106305=CARTESIAN_POINT ( 'NONE',  ( 10.52399048938390003, 1498.970143501030179, 202.0357175427869834 ) ) ;
#106311=CARTESIAN_POINT ( 'NONE',  ( 11.96299724475220039, 1501.580462394789947, 211.5588274086130127 ) ) ;
#106317=CARTESIAN_POINT ( 'NONE',  ( -2.487923244941209866, 1508.731373123109961, 204.5668975639180189 ) ) ;
#106319=B_SPLINE_CURVE_WITH_KNOTS ( 'NONE', 3,
 ( #42720, #17476, #9112, #7453, #25332, #101487, #42164, #24774 ),
 .UNSPECIFIED., .F., .F.,
 ( 4, 2, 2, 4 ),
 ( 0.000000000000000000, 0.5000000000000000000, 0.7500000000000000000, 1.000000000000000000 ),
 .UNSPECIFIED. ) ;
#106322=CARTESIAN_POINT ( 'NONE',  ( -4.840660725190000235, 1489.193457555089935, 188.8938074394989997 ) ) ;
#106325=B_SPLINE_CURVE_WITH_KNOTS ( 'NONE', 5,
 ( #13583, #47769, #39362, #107672, #22522, #30957 ),
 .UNSPECIFIED., .F., .F.,
 ( 6, 6 ),
 ( 0.000000000000000000, 1.000000000000000000 ),
 .UNSPECIFIED. ) ;
#106327=CARTESIAN_POINT ( 'NONE',  ( -3.072929113039999827, 1475.870006633390176, 199.1238679828490206 ) ) ;
#106329=ORIENTED_EDGE ( 'NONE', *, *, #94114, .T. ) ;
#106330=CARTESIAN_POINT ( 'NONE',  ( 20.75864866223560057, 1455.056248125270031, 207.3304711268599760 ) ) ;
#106333=CARTESIAN_POINT ( 'NONE',  ( -4.848919996459999382, 1489.192135936889827, 188.8958457811990002 ) ) ;
#106335=EDGE_CURVE ( 'NONE', #27879, #53764, #103275, .T. ) ;
#106336=CARTESIAN_POINT ( 'NONE',  ( 4.025649270539999769, 1466.171376325889923, 219.4115622680990043 ) ) ;
#106343=CARTESIAN_POINT ( 'NONE',  ( 11.46179980149750044, 1491.526194067609822, 208.8062879593289836 ) ) ;
#106349=CARTESIAN_POINT ( 'NONE',  ( 2.041914512376249657, 1497.024681018629963, 196.8943108031110114 ) ) ;
#106350=EDGE_CURVE ( 'NONE', #104484, #83093, #95253, .T. ) ;
#106364=B_SPLINE_SURFACE_WITH_KNOTS ( 'NONE', 5, 5, ( 
 ( #109502, #7581, #8670, #83194, #102184, #68073 ),
 ( #58005, #51242, #84823, #32778, #108394, #101617 ),
 ( #31675, #65856, #66962, #99975, #92141, #108948 ),
 ( #16503, #91591, #59113, #85376, #15414, #101071 ),
 ( #41736, #50161, #50692, #49605, #24369, #58555 ),
 ( #8124, #14866, #15958, #49058, #75895, #110047 ) ),
 .UNSPECIFIED., .F., .F., .F.,
 ( 6, 6 ),
 ( 6, 6 ),
 ( 5.893388375705330695, 9.819929736144670684 ),
 ( 0.000000000000000000, 0.5002947206946709580 ),
 .UNSPECIFIED. ) ;
#106366=CARTESIAN_POINT ( 'NONE',  ( 1.707874834880000137, 1497.186644415389765, 197.2309891130989854 ) ) ;
#106368=VERTEX_POINT ( 'NONE', #54181 ) ;
#106375=CARTESIAN_POINT ( 'NONE',  ( 0.8991927417389989907, 1486.143869282489959, 220.2726218139989953 ) ) ;
#106377=CARTESIAN_POINT ( 'NONE',  ( 20.12874795999999833, 1473.837606016890049, 209.1218459616989946 ) ) ;
#106389=ADVANCED_FACE ( 'NONE', ( #69879 ), #76716, .T. ) ;
#106390=VERTEX_POINT ( 'NONE', #65328 ) ;
#106391=CARTESIAN_POINT ( 'NONE',  ( -4.367915676912749845, 1447.898270802109892, 190.6350657527499948 ) ) ;
#106397=ORIENTED_EDGE ( 'NONE', *, *, #15824, .F. ) ;
#106401=ORIENTED_EDGE ( 'NONE', *, *, #72317, .F. ) ;
#106404=CARTESIAN_POINT ( 'NONE',  ( 10.96111033800959866, 1480.941108277019794, 213.4869506453160000 ) ) ;
#106405=CARTESIAN_POINT ( 'NONE',  ( 1.847634001515719993, 1478.089546411300262, 198.8590795898780073 ) ) ;
#106408=CARTESIAN_POINT ( 'NONE',  ( -11.87327837476540005, 1482.014171357300029, 208.6019633461839931 ) ) ;
#106411=CARTESIAN_POINT ( 'NONE',  ( -8.593317962150289091, 1470.520629101329860, 214.8006129900909968 ) ) ;
#106413=CARTESIAN_POINT ( 'NONE',  ( 8.725351515859999907, 1420.892103511989944, 196.4178243839989761 ) ) ;
#106415=CARTESIAN_POINT ( 'NONE',  ( -2.853004531550470180, 1476.255805782230254, 220.2301807339150059 ) ) ;
#106418=CARTESIAN_POINT ( 'NONE',  ( -12.63597620429999857, 1503.239529842989896, 208.6558503650219905 ) ) ;
#106422=ADVANCED_FACE ( 'NONE', ( #102202 ), #109770, .T. ) ;
#106424=ORIENTED_EDGE ( 'NONE', *, *, #106120, .F. ) ;
#106429=CARTESIAN_POINT ( 'NONE',  ( 5.328644995739999501, 1505.167604692990153, 220.2736030611989975 ) ) ;
#106431=CARTESIAN_POINT ( 'NONE',  ( -15.22121264530000140, 1415.857004583649996, 211.5998937619590095 ) ) ;
#106432=CARTESIAN_POINT ( 'NONE',  ( -17.33843278754439865, 1419.406148393270087, 207.7041131039349864 ) ) ;
#106437=CARTESIAN_POINT ( 'NONE',  ( 0.5650653572531030289, 1430.599530611739965, 199.7038102876320238 ) ) ;
#106439=DIRECTION ( 'NONE',  ( 0.000000000000000000, 1.000000000000000000, 0.000000000000000000 ) ) ;
#106453=CARTESIAN_POINT ( 'NONE',  ( -14.26437337564139973, 1416.738556469530067, 203.2135512967790021 ) ) ;
#106463=ORIENTED_EDGE ( 'NONE', *, *, #73425, .F. ) ;
#106464=CARTESIAN_POINT ( 'NONE',  ( 3.556995324409999881, 1476.475065048189890, 198.0947962222990100 ) ) ;
#106466=CARTESIAN_POINT ( 'NONE',  ( -11.29172267060000046, 1491.552985758590012, 207.2028609495190210 ) ) ;
#106467=CARTESIAN_POINT ( 'NONE',  ( 2.203005645500000220, 1464.498845408490070, 202.4205385530689796 ) ) ;
#106470=CARTESIAN_POINT ( 'NONE',  ( -11.85463470256620155, 1481.688684073870036, 209.6797579912160074 ) ) ;
#106475=CARTESIAN_POINT ( 'NONE',  ( -12.24102064520350019, 1490.576295553370073, 208.4712049614670093 ) ) ;
#106489=B_SPLINE_SURFACE_WITH_KNOTS ( 'NONE', 5, 5, ( 
 ( #34441, #51241, #76440, #26580, #27151, #69167, #36107, #1399, #52916 ),
 ( #70293, #861, #1971, #42289, #102719, #60777, #26013, #60209, #94902 ),
 ( #110595, #104404, #78095, #18176, #33879, #17606, #87048, #27698, #86492 ),
 ( #103272, #25463, #43953, #35538, #44508, #69733, #78655, #16502, #95455 ),
 ( #94328, #50691, #102183, #77010, #84822, #8123, #93766, #17045, #103852 ),
 ( #18720, #51806, #34987, #85375, #43406, #20927, #13071, #3079, #63004 ) ),
 .UNSPECIFIED., .F., .F., .F.,
 ( 6, 6 ),
 ( 6, 3, 6 ),
 ( 9.791992066980000686, 13.21653623010000089 ),
 ( 0.000000000000000000, 1.500000000000000000, 3.000000000000000000 ),
 .UNSPECIFIED. ) ;
#106491=CARTESIAN_POINT ( 'NONE',  ( -18.47517316556379896, 1466.235620594650072, 200.8822777731460008 ) ) ;
#106497=CARTESIAN_POINT ( 'NONE',  ( 1970.025574498409924, -8382.262153571269664, 413.0777247525010125 ) ) ;
#106502=CARTESIAN_POINT ( 'NONE',  ( -9.199049879260000395, 1422.949100153850168, 210.5804414222690184 ) ) ;
#106503=CARTESIAN_POINT ( 'NONE',  ( -12.08007700854662225, 1421.774748355924658, 210.6450025019371139 ) ) ;
#106506=EDGE_LOOP ( 'NONE', ( #62511, #109971, #97789, #59256 ) ) ;
#106510=VECTOR ( 'NONE', #85935, 1000.000000000000000 ) ;
#106518=CARTESIAN_POINT ( 'NONE',  ( 10.04235571396320026, 1481.895431969530136, 213.0073720138159956 ) ) ;
#106523=CARTESIAN_POINT ( 'NONE',  ( -7.229435970709999992, 1480.743738106489900, 207.9750912412490038 ) ) ;
#106526=CARTESIAN_POINT ( 'NONE',  ( -1.196549396492360140, 1431.757418655609854, 200.8025689291640106 ) ) ;
#106536=CARTESIAN_POINT ( 'NONE',  ( -0.5893430329309989890, 1464.381058777490125, 199.1585742529190100 ) ) ;
#106546=CARTESIAN_POINT ( 'NONE',  ( 11.63359383422730176, 1479.019660161769934, 207.4180740764660129 ) ) ;
#106552=CARTESIAN_POINT ( 'NONE',  ( -9.613420378160620672, 1438.053801520089792, 211.4783176813969874 ) ) ;
#106562=CARTESIAN_POINT ( 'NONE',  ( -8.320994297490690528, 1422.937291762939822, 213.3671062658739856 ) ) ;
#106566=CARTESIAN_POINT ( 'NONE',  ( -11.46886437749099841, 1482.732392890260144, 205.9150088758919708 ) ) ;
#106574=CARTESIAN_POINT ( 'NONE',  ( -20.65369855650610020, 1487.044956911440067, 207.4344914902700054 ) ) ;
#106577=CARTESIAN_POINT ( 'NONE',  ( -9.966727850805121136, 1439.480327375449860, 208.4309914983489875 ) ) ;
#106589=CARTESIAN_POINT ( 'NONE',  ( -6.916803064789941224, 1439.753322365320628, 203.7544753627797149 ) ) ;
#106590=CARTESIAN_POINT ( 'NONE',  ( -7.055457375169999601, 1459.495818635790101, 217.3326011958589845 ) ) ;
#106594=CARTESIAN_POINT ( 'NONE',  ( -4.123245670370000227, 1515.545044289889802, 209.8706601212949749 ) ) ;
#106601=DIRECTION ( 'NONE',  ( 1.224646799147350002E-16, -1.836970198721029688E-16, -1.000000000000000000 ) ) ;
#106608=CARTESIAN_POINT ( 'NONE',  ( -3.244847879459100248, 1508.551704408389924, 204.2522919139599935 ) ) ;
#106611=CARTESIAN_POINT ( 'NONE',  ( -2.207969477403779912, 1436.315141507179987, 227.4839793697360051 ) ) ;
#106612=CARTESIAN_POINT ( 'NONE',  ( -13.58088438526920072, 1508.551704407800116, 210.3100666414740090 ) ) ;
#106619=CARTESIAN_POINT ( 'NONE',  ( 7.635296396580000255, 1426.631419723420095, 212.2123003208889997 ) ) ;
#106620=CARTESIAN_POINT ( 'NONE',  ( -22.15968325629999924, 1485.573345355790025, 217.2083650093589995 ) ) ;
#106625=CARTESIAN_POINT ( 'NONE',  ( 9.906408661899998691, 1453.734930172990062, 213.0153772767789917 ) ) ;
#106635=CARTESIAN_POINT ( 'NONE',  ( -21.51614340397090075, 1505.638256348389859, 209.3196076299650201 ) ) ;
#106646=EDGE_LOOP ( 'NONE', ( #78800, #97482, #16424, #31859 ) ) ;
#106647=ORIENTED_EDGE ( 'NONE', *, *, #81068, .T. ) ;
#106648=CARTESIAN_POINT ( 'NONE',  ( -17.65532971150000208, 1419.497219977419945, 207.2321558962389929 ) ) ;
#106655=ORIENTED_EDGE ( 'NONE', *, *, #93262, .F. ) ;
#106656=CARTESIAN_POINT ( 'NONE',  ( -17.83734749800949970, 1508.522611025080096, 211.8629472681300001 ) ) ;
#106662=ORIENTED_EDGE ( 'NONE', *, *, #51476, .F. ) ;
#106673=CARTESIAN_POINT ( 'NONE',  ( 10.10526312269999849, 1471.402127165189995, 212.2219414490489839 ) ) ;
#106679=CARTESIAN_POINT ( 'NONE',  ( 6.179817242093199603, 1424.911203525419978, 192.2193043612860208 ) ) ;
#106689=CARTESIAN_POINT ( 'NONE',  ( -2.140641997699999965, 1508.551704408389924, 220.0635241299990241 ) ) ;
#106691=CARTESIAN_POINT ( 'NONE',  ( 11.24138533720000055, 1422.409861511610188, 204.1338940524489942 ) ) ;
#106695=CARTESIAN_POINT ( 'NONE',  ( 2.780672902370000088, 1460.407737242989924, 228.5579519583990020 ) ) ;
#106696=CARTESIAN_POINT ( 'NONE',  ( 11.37695908739150141, 1470.749029468129947, 208.3696375387830244 ) ) ;
#106700=EDGE_LOOP ( 'NONE', ( #107203, #15058, #10380, #19740 ) ) ;
#106701=CARTESIAN_POINT ( 'NONE',  ( 18.79226589730000185, 1456.307606824690083, 213.7887498653890077 ) ) ;
#106704=CARTESIAN_POINT ( 'NONE',  ( 4.706522373909999502, 1426.134490744389950, 210.8435422850390069 ) ) ;
#106705=CARTESIAN_POINT ( 'NONE',  ( 8.973660471278915196, 1425.007957488622651, 195.6894122325922467 ) ) ;
#106706=CARTESIAN_POINT ( 'NONE',  ( 1.531308761570000065, 1442.248940191690053, 218.5680284645490019 ) ) ;
#106710=CARTESIAN_POINT ( 'NONE',  ( -20.44161166330000157, 1485.241385972889930, 206.1012198832090121 ) ) ;
#106718=CARTESIAN_POINT ( 'NONE',  ( -16.65377040190000102, 1508.454794883789873, 213.7212185660889929 ) ) ;
#106720=CARTESIAN_POINT ( 'NONE',  ( 11.26363633646609941, 1470.487396938490065, 207.5510992998169968 ) ) ;
#106721=CARTESIAN_POINT ( 'NONE',  ( -3.378095328389999707, 1485.354467027690134, 197.6993834011990145 ) ) ;
#106724=AXIS2_PLACEMENT_3D ( 'NONE', #87566, #11948, #80259 ) ;
#106727=CARTESIAN_POINT ( 'NONE',  ( 4.730876151940029750, 1493.686648256609942, 219.2027333063510071 ) ) ;
#106728=CARTESIAN_POINT ( 'NONE',  ( -21.26809933518700291, 1485.919115173290038, 201.7808441828850050 ) ) ;
#106729=CARTESIAN_POINT ( 'NONE',  ( -15.45647355988487881, 1415.677402202029953, 209.5466896407415618 ) ) ;
#106732=CARTESIAN_POINT ( 'NONE',  ( 6.365104321110000463, 1429.227105708690033, 215.6823107352090005 ) ) ;
#106733=DIRECTION ( 'NONE',  ( 1.224646799147353207E-16, -1.836970198721029688E-16, -1.000000000000000000 ) ) ;
#106748=CARTESIAN_POINT ( 'NONE',  ( 0.000000000000000000, 1420.119835273649869, 209.1218459616989946 ) ) ;
#106751=CARTESIAN_POINT ( 'NONE',  ( 8.616434899906300515, 1465.329448497550175, 213.9433383265620137 ) ) ;
#106753=CARTESIAN_POINT ( 'NONE',  ( 0.3731951684343629561, 1515.150224411170029, 213.4490576343089856 ) ) ;
#106755=CARTESIAN_POINT ( 'NONE',  ( -11.02097544798480122, 1480.400473981879941, 213.2717396774600331 ) ) ;
#106762=CARTESIAN_POINT ( 'NONE',  ( -22.15338394760000185, 1485.967612886890038, 217.2877321619890267 ) ) ;
#106770=CARTESIAN_POINT ( 'NONE',  ( -6.384611937859999919, 1459.149684699189947, 217.3122905540589898 ) ) ;
#106773=ORIENTED_EDGE ( 'NONE', *, *, #2138, .F. ) ;
#106789=CARTESIAN_POINT ( 'NONE',  ( 9.600863931830000197, 1470.542903070589773, 212.2537315410889676 ) ) ;
#106793=CARTESIAN_POINT ( 'NONE',  ( 9.338308684742390398, 1435.342874469600019, 208.2407783485550112 ) ) ;
#106798=CARTESIAN_POINT ( 'NONE',  ( 10.95098205620359977, 1471.837422849929908, 212.3987392730099657 ) ) ;
#106799=CARTESIAN_POINT ( 'NONE',  ( -20.68580785760000040, 1486.599620265689964, 210.1129637272439936 ) ) ;
#106810=CARTESIAN_POINT ( 'NONE',  ( 4.487249772970000272, 1509.038615934189920, 209.1218459625970070 ) ) ;
#106829=CARTESIAN_POINT ( 'NONE',  ( -5.062212390315069754, 1474.342205398819942, 198.8731691453010058 ) ) ;
#106840=CARTESIAN_POINT ( 'NONE',  ( 11.74145575222949844, 1499.920360182230070, 205.7526641877259976 ) ) ;
#106847=EDGE_CURVE ( 'NONE', #18777, #53857, #75151, .T. ) ;
#106853=CARTESIAN_POINT ( 'NONE',  ( -4.410745965304349703, 1508.610338743689908, 205.2563625205500273 ) ) ;
#106862=EDGE_CURVE ( 'NONE', #50172, #32360, #91193, .T. ) ;
#106863=CARTESIAN_POINT ( 'NONE',  ( 2.487935123020000194, 1508.551704408389924, 204.1347675455010062 ) ) ;
#106866=CARTESIAN_POINT ( 'NONE',  ( 10.75634779605130120, 1451.137958617219965, 190.3409307970749751 ) ) ;
#106872=CARTESIAN_POINT ( 'NONE',  ( -4.885449122210000716, 1463.524425562389752, 200.4816631501890072 ) ) ;
#106878=CARTESIAN_POINT ( 'NONE',  ( 8.731332846349999954, 1459.404707344790040, 227.0651519182989944 ) ) ;
#106882=DIRECTION ( 'NONE',  ( -9.500021872036790217E-47, 1.000000000000000000, -1.836970198721029688E-16 ) ) ;
#106884=VERTEX_POINT ( 'NONE', #44128 ) ;
#106901=CARTESIAN_POINT ( 'NONE',  ( -9.033366821045200723, 1447.304030695519941, 212.0885462952919909 ) ) ;
#106905=CYLINDRICAL_SURFACE ( 'NONE', #31893, 0.4999999999999909517 ) ;
#106916=CARTESIAN_POINT ( 'NONE',  ( 1.969630537620000066, 1485.776228655490058, 220.0997983293990217 ) ) ;
#106917=CARTESIAN_POINT ( 'NONE',  ( -4.994701136659999818, 1391.710704960489920, 214.4888430591489907 ) ) ;
#106928=ORIENTED_EDGE ( 'NONE', *, *, #20324, .F. ) ;
#106931=VECTOR ( 'NONE', #89952, 1000.000000000000114 ) ;
#106934=EDGE_CURVE ( 'NONE', #102270, #79909, #29712, .T. ) ;
#106944=ORIENTED_EDGE ( 'NONE', *, *, #69262, .T. ) ;
#106945=CARTESIAN_POINT ( 'NONE',  ( 9.188387156589639559, 1482.188622616660041, 216.5467321156359901 ) ) ;
#106948=ORIENTED_EDGE ( 'NONE', *, *, #20631, .T. ) ;
#106949=CARTESIAN_POINT ( 'NONE',  ( -11.42598084535810088, 1481.698338076739901, 209.1408964386100138 ) ) ;
#106952=CARTESIAN_POINT ( 'NONE',  ( 1.968522348845569869, 1498.935384250119796, 197.9561377214020013 ) ) ;
#106955=CARTESIAN_POINT ( 'NONE',  ( 12.21937182940000000, 1420.343723557070007, 199.7692422141290081 ) ) ;
#106956=CARTESIAN_POINT ( 'NONE',  ( -2.552257842228009999, 1476.146710473380153, 220.2966558116410170 ) ) ;
#106957=CARTESIAN_POINT ( 'NONE',  ( -20.06562366400000030, 1485.934169092390221, 214.0282076738189971 ) ) ;
#106962=CARTESIAN_POINT ( 'NONE',  ( 12.38805570981969950, 1421.643760760719942, 207.4832281941469887 ) ) ;
#106967=ORIENTED_EDGE ( 'NONE', *, *, #17506, .F. ) ;
#106969=CARTESIAN_POINT ( 'NONE',  ( -16.70830179842720042, 1417.149226859160080, 207.3570905742490140 ) ) ;
#106972=CARTESIAN_POINT ( 'NONE',  ( -14.93837044589999863, 1416.023439725270009, 212.9159407297890141 ) ) ;
#106973=CARTESIAN_POINT ( 'NONE',  ( -17.59913612719639886, 1419.797432416249876, 206.6689813231369897 ) ) ;
#106978=CARTESIAN_POINT ( 'NONE',  ( -7.454153900785907894, 1476.755908734740842, 216.3333321094707173 ) ) ;
#106979=CARTESIAN_POINT ( 'NONE',  ( -19.38497611889999916, 1464.684217820690037, 212.9113686205490126 ) ) ;
#106988=CARTESIAN_POINT ( 'NONE',  ( 2.005628669607020242, 1474.789351304850015, 220.3635328066820023 ) ) ;
#107000=CARTESIAN_POINT ( 'NONE',  ( -4.329448776040000446, 1515.064792882589927, 207.6699913460390121 ) ) ;
#107002=CARTESIAN_POINT ( 'NONE',  ( 0.9841710845998976609, 1484.601693631961325, 198.4550311835998855 ) ) ;
#107008=CARTESIAN_POINT ( 'NONE',  ( 4.570408800500000090, 1476.902228035989992, 198.8607389952989877 ) ) ;
#107010=CARTESIAN_POINT ( 'NONE',  ( -11.42267527399999949, 1490.824039550989937, 209.4152927566280198 ) ) ;
#107016=CARTESIAN_POINT ( 'NONE',  ( 8.214112888310001637, 1423.929736291430117, 211.6354380387589913 ) ) ;
#107021=CARTESIAN_POINT ( 'NONE',  ( -12.07909423994960108, 1491.047902796329936, 206.9755603749529769 ) ) ;
#107022=CARTESIAN_POINT ( 'NONE',  ( -4.580619238605350141, 1508.551704408389924, 205.2658447893479945 ) ) ;
#107032=CARTESIAN_POINT ( 'NONE',  ( -11.25901873334290038, 1500.172003390719965, 210.8567363214919794 ) ) ;
#107034=CARTESIAN_POINT ( 'NONE',  ( -2.379192260459999986, 1422.184172195939937, 193.0946206466989850 ) ) ;
#107037=CARTESIAN_POINT ( 'NONE',  ( -20.46642572180000030, 1467.931903674690147, 211.3545004319090026 ) ) ;
#107050=EDGE_CURVE ( 'NONE', #25418, #11098, #60242, .T. ) ;
#107055=B_SPLINE_CURVE_WITH_KNOTS ( 'NONE', 5,
 ( #12174, #36832, #35726, #104027, #53663, #104586, #20556, #89441, #10526 ),
 .UNSPECIFIED., .F., .F.,
 ( 6, 3, 6 ),
 ( 0.000000000000000000, 0.4556035044110292587, 1.000000000000000000 ),
 .UNSPECIFIED. ) ;
#107060=CARTESIAN_POINT ( 'NONE',  ( 11.23408297830000002, 1500.787540975290085, 206.3532497413090141 ) ) ;
#107067=CARTESIAN_POINT ( 'NONE',  ( 7.161184789771309234, 1483.929743994920045, 217.3859321370360078 ) ) ;
#107072=CARTESIAN_POINT ( 'NONE',  ( -19.34950235940319985, 1446.106554878399947, 200.0047909411070179 ) ) ;
#107073=FACE_OUTER_BOUND ( 'NONE', #6403, .T. ) ;
#107077=CARTESIAN_POINT ( 'NONE',  ( 5.456719627610000067, 1455.595244131089885, 218.2350948550090095 ) ) ;
#107090=ORIENTED_EDGE ( 'NONE', *, *, #69154, .F. ) ;
#107097=CARTESIAN_POINT ( 'NONE',  ( 20.96806063649999885, 1497.404333632189946, 212.2179028469190030 ) ) ;
#107113=CARTESIAN_POINT ( 'NONE',  ( 2.329957330370219903, 1515.551704201149960, 212.9510108335710186 ) ) ;
#107114=CARTESIAN_POINT ( 'NONE',  ( -4.726544020967549997, 1483.113842110900123, 199.5813482372220165 ) ) ;
#107115=FACE_OUTER_BOUND ( 'NONE', #7230, .T. ) ;
#107120=CARTESIAN_POINT ( 'NONE',  ( -15.04100366369999975, 1416.091181750810165, 205.5542740844690002 ) ) ;
#107121=CARTESIAN_POINT ( 'NONE',  ( -7.497461585337410028, 1441.051475807649922, 203.6591753659959920 ) ) ;
#107132=CARTESIAN_POINT ( 'NONE',  ( -0.7420515760000009342, 1515.368784161290250, 213.4096358822789909 ) ) ;
#107149=CARTESIAN_POINT ( 'NONE',  ( 8.978224880359460869, 1452.688325515109909, 212.1105500328530127 ) ) ;
#107152=CARTESIAN_POINT ( 'NONE',  ( -5.005324004894529111, 1391.742413812679388, 214.7013071040425132 ) ) ;
#107156=B_SPLINE_SURFACE_WITH_KNOTS ( 'NONE', 5, 1, ( 
 ( #103990, #27288 ),
 ( #26731, #52507 ),
 ( #77154, #78802 ),
 ( #34580, #25610 ),
 ( #51949, #102868 ),
 ( #60919, #9931 ) ),
 .UNSPECIFIED., .F., .F., .F.,
 ( 6, 6 ),
 ( 2, 2 ),
 ( -7.538862163178030240E-05, 16.22318445422160238 ),
 ( 0.000000000000000000, 14.00007538862159961 ),
 .UNSPECIFIED. ) ;
#107157=CARTESIAN_POINT ( 'NONE',  ( 12.12990662800260111, 1491.497813992390093, 207.1218616752200035 ) ) ;
#107162=AXIS2_PLACEMENT_3D ( 'NONE', #87498, #56093, #56646 ) ;
#107166=CARTESIAN_POINT ( 'NONE',  ( -13.59502692214180009, 1507.745895393389901, 209.3598175520070015 ) ) ;
#107174=CARTESIAN_POINT ( 'NONE',  ( 11.85459481136119919, 1500.917689636769865, 208.6046480963290151 ) ) ;
#107175=CARTESIAN_POINT ( 'NONE',  ( 18.46110511450000047, 1471.786120934990095, 195.2229451476989937 ) ) ;
#107182=CARTESIAN_POINT ( 'NONE',  ( 9.085013217329999335, 1453.300037844490134, 212.7885071865789826 ) ) ;
#107183=ORIENTED_EDGE ( 'NONE', *, *, #46404, .T. ) ;
#107184=EDGE_LOOP ( 'NONE', ( #27197, #106397, #61347, #71654, #22022, #110, #90387, #4850, #101744, #48990, #16043, #14703 ) ) ;
#107191=FACE_OUTER_BOUND ( 'NONE', #9817, .T. ) ;
#107196=CARTESIAN_POINT ( 'NONE',  ( -3.983812761516020373, 1463.710686891660089, 200.0140896495050242 ) ) ;
#107203=ORIENTED_EDGE ( 'NONE', *, *, #43441, .T. ) ;
#107208=CARTESIAN_POINT ( 'NONE',  ( -17.57407502070000049, 1419.698630043679941, 206.3903661100590057 ) ) ;
#107215=CARTESIAN_POINT ( 'NONE',  ( -18.53384158972099982, 1508.522892864089954, 210.7233192446600185 ) ) ;
#107222=CARTESIAN_POINT ( 'NONE',  ( -8.946235101802798795, 1451.321446327319791, 206.7355029101660193 ) ) ;
#107226=ORIENTED_EDGE ( 'NONE', *, *, #23551, .T. ) ;
#107236=CARTESIAN_POINT ( 'NONE',  ( 15.82512562826290292, 1427.733577895149892, 200.2964982622260095 ) ) ;
#107250=CARTESIAN_POINT ( 'NONE',  ( 10.76697211809999999, 1423.735811814160115, 203.5994285750890072 ) ) ;
#107254=CARTESIAN_POINT ( 'NONE',  ( 8.631780704876279131, 1438.018275767699834, 210.0183142686710198 ) ) ;
#107257=CARTESIAN_POINT ( 'NONE',  ( 10.52024531799330020, 1481.173637506630030, 208.1780703194219768 ) ) ;
#107265=CARTESIAN_POINT ( 'NONE',  ( 2.159699301869999477, 1441.959095157789989, 218.4271172946090189 ) ) ;
#107267=CARTESIAN_POINT ( 'NONE',  ( 17.10950584751149961, 1472.077583655310036, 198.3318500205459998 ) ) ;
#107269=CARTESIAN_POINT ( 'NONE',  ( -20.55757218060000113, 1485.073878606189965, 207.1049163177690104 ) ) ;
#107275=ORIENTED_EDGE ( 'NONE', *, *, #36574, .T. ) ;
#107279=CYLINDRICAL_SURFACE ( 'NONE', #68226, 0.2999999999999669598 ) ;
#107285=B_SPLINE_SURFACE_WITH_KNOTS ( 'NONE', 5, 5, ( 
 ( #96692, #80984, #78781, #62572, #55251, #89383 ),
 ( #46310, #54157, #2095, #19962, #70409, #12675 ),
 ( #11027, #104528, #4290, #97226, #38417, #71528 ),
 ( #2648, #106184, #72593, #3754, #3205, #106721 ),
 ( #36776, #37332, #20497, #11577, #30012, #44639 ),
 ( #45196, #64202, #27825, #87179, #37886, #45754 ),
 ( #62005, #96125, #19399, #53603, #79337, #105084 ),
 ( #79891, #100530, #56893, #15410, #23809, #32232 ),
 ( #108944, #7028, #64765, #91024, #107833, #55808 ) ),
 .UNSPECIFIED., .F., .F., .F.,
 ( 6, 3, 6 ),
 ( 6, 6 ),
 ( 9.104900351529998659, 12.35991293620000064, 15.61492552089999997 ),
 ( 0.000000000000000000, 2.000000000000000000 ),
 .UNSPECIFIED. ) ;
#107292=CARTESIAN_POINT ( 'NONE',  ( 5.598416906409999783, 1429.565212975089935, 216.3190638356489899 ) ) ;
#107293=CARTESIAN_POINT ( 'NONE',  ( 20.45347777980000004, 1495.695647834889996, 214.2365953844490036 ) ) ;
#107295=VECTOR ( 'NONE', #53792, 1000.000000000000000 ) ;
#107306=CARTESIAN_POINT ( 'NONE',  ( 8.614620945600030666, 1437.484188997010051, 209.9974677346399972 ) ) ;
#107312=CARTESIAN_POINT ( 'NONE',  ( -0.8481724230074738635, 1515.120541028469916, 213.4498349211539789 ) ) ;
#107314=CARTESIAN_POINT ( 'NONE',  ( -8.346688520235490572, 1478.631378035029911, 217.2409271317110040 ) ) ;
#107321=CARTESIAN_POINT ( 'NONE',  ( -0.3862418810146379666, 1500.063169577209919, 233.1571753207470010 ) ) ;
#107330=CARTESIAN_POINT ( 'NONE',  ( -3.179033936840000241, 1457.997354091689886, 219.3203917952990025 ) ) ;
#107336=ORIENTED_EDGE ( 'NONE', *, *, #53536, .F. ) ;
#107341=CARTESIAN_POINT ( 'NONE',  ( -17.64585193930734519, 1419.365468075514855, 207.2015379587035682 ) ) ;
#107345=ORIENTED_EDGE ( 'NONE', *, *, #57592, .F. ) ;
#107352=CARTESIAN_POINT ( 'NONE',  ( -9.161428420492889302, 1488.487993194839873, 190.2768237055279883 ) ) ;
#107363=CARTESIAN_POINT ( 'NONE',  ( 6.888583400142420210, 1460.429153260329031, 202.3504153456137260 ) ) ;
#107364=CARTESIAN_POINT ( 'NONE',  ( 6.121126660120000729, 1455.402339941889750, 217.8370560331890147 ) ) ;
#107365=CARTESIAN_POINT ( 'NONE',  ( 7.611664470185079523, 1439.490851628699829, 213.6370682771540146 ) ) ;
#107370=DIRECTION ( 'NONE',  ( -1.224646799147350002E-16, 1.836970198721029688E-16, 1.000000000000000000 ) ) ;
#107373=CARTESIAN_POINT ( 'NONE',  ( -5.032977197542991554, 1391.805267110368050, 214.4361776410948721 ) ) ;
#107389=CARTESIAN_POINT ( 'NONE',  ( 0.6889265495279990326, 1475.123389914190057, 220.5466911795989802 ) ) ;
#107398=CARTESIAN_POINT ( 'NONE',  ( -10.50217937927759948, 1470.323102136789885, 212.1317377489009743 ) ) ;
#107402=CARTESIAN_POINT ( 'NONE',  ( 11.78140839543589991, 1479.499659610600020, 209.2033645326229703 ) ) ;
#107408=CARTESIAN_POINT ( 'NONE',  ( -2.092371031960829963, 1508.551704408389924, 220.0661208745100055 ) ) ;
#107418=CARTESIAN_POINT ( 'NONE',  ( -3.251166460929999946, 1475.808624674589737, 199.1811513380790188 ) ) ;
#107421=CARTESIAN_POINT ( 'NONE',  ( -13.05159921682169966, 1467.538567272380078, 191.8992743155650089 ) ) ;
#107425=CARTESIAN_POINT ( 'NONE',  ( -2.329898844065350083, 1515.219291385429869, 204.7964424083469908 ) ) ;
#107427=CARTESIAN_POINT ( 'NONE',  ( -5.487686449739999972, 1463.833492974589944, 200.5004408324890335 ) ) ;
#107428=CARTESIAN_POINT ( 'NONE',  ( -15.20114627789167550, 1420.043106467314828, 212.3145834610196800 ) ) ;
#107430=CARTESIAN_POINT ( 'NONE',  ( 21.04904418909999819, 1494.916427559390058, 209.1218459616989946 ) ) ;
#107433=CARTESIAN_POINT ( 'NONE',  ( 17.80745809460000117, 1457.129128898490080, 217.9030147174489969 ) ) ;
#107434=DIRECTION ( 'NONE',  ( 9.500914144214121536E-47, -1.000000000000000000, 1.836970198721029688E-16 ) ) ;
#107446=CARTESIAN_POINT ( 'NONE',  ( -15.06439020900000081, 1420.324155258209885, 212.5657008686889924 ) ) ;
#107454=CARTESIAN_POINT ( 'NONE',  ( -8.557097019430230489, 1448.618184358840153, 212.3365240749560030 ) ) ;
#107459=CARTESIAN_POINT ( 'NONE',  ( 7.164851019203979376, 1424.936393926430128, 212.9153315477099966 ) ) ;
#107462=CARTESIAN_POINT ( 'NONE',  ( -3.234068298869999580, 1415.020930770710038, 205.6238868179589758 ) ) ;
#107483=CARTESIAN_POINT ( 'NONE',  ( 0.7786186376918419194, 1443.353423969640062, 200.2227269049809877 ) ) ;
#107486=EDGE_CURVE ( 'NONE', #345, #54152, #104479, .T. ) ;
#107495=ADVANCED_FACE ( 'NONE', ( #87240 ), #48297, .T. ) ;
#107497=CARTESIAN_POINT ( 'NONE',  ( 6.195891505149140777, 1479.055035075845808, 200.6311094197622822 ) ) ;
#107500=CARTESIAN_POINT ( 'NONE',  ( -10.53750713949369988, 1480.572745636769923, 208.8422318348939939 ) ) ;
#107503=CARTESIAN_POINT ( 'NONE',  ( 4.672708027043240619, 1498.588723887579818, 198.5412103530289869 ) ) ;
#107506=CARTESIAN_POINT ( 'NONE',  ( 11.58059658486819998, 1502.144060851190034, 214.4076140139739834 ) ) ;
#107508=CARTESIAN_POINT ( 'NONE',  ( -0.8218185942339699679, 1475.571559382040050, 220.5270802406460007 ) ) ;
#107514=CARTESIAN_POINT ( 'NONE',  ( 11.02997679787949892, 1425.732792483290041, 206.4966215837540062 ) ) ;
#107516=CARTESIAN_POINT ( 'NONE',  ( -9.670994933606040789, 1440.251970265710042, 206.4953985460990111 ) ) ;
#107519=CARTESIAN_POINT ( 'NONE',  ( -4.772433264290000032, 1461.586210710390105, 228.1254610687989839 ) ) ;
#107522=CARTESIAN_POINT ( 'NONE',  ( 20.05523460210000053, 1476.340215940290136, 212.0965055883189905 ) ) ;
#107523=ADVANCED_FACE ( 'NONE', ( #31732 ), #109117, .T. ) ;
#107524=CARTESIAN_POINT ( 'NONE',  ( -15.68545621147730174, 1420.312772934420082, 210.6112538882230183 ) ) ;
#107525=ORIENTED_EDGE ( 'NONE', *, *, #77112, .T. ) ;
#107526=CARTESIAN_POINT ( 'NONE',  ( 3.249023004060000552, 1430.716676741390074, 218.0587861596190180 ) ) ;
#107540=LINE ( 'NONE', #73403, #71766 ) ;
#107547=CARTESIAN_POINT ( 'NONE',  ( -0.7147294630179988895, 1515.255091259190067, 204.7973799830389794 ) ) ;
#107548=CARTESIAN_POINT ( 'NONE',  ( 12.47690690837549887, 1427.073077267369854, 206.5591765600709948 ) ) ;
#107549=CARTESIAN_POINT ( 'NONE',  ( -2.515613211938379834, 1448.349718483709921, 188.5842421559209754 ) ) ;
#107563=CARTESIAN_POINT ( 'NONE',  ( -12.02051124189999953, 1491.153688314190049, 206.6632161944989718 ) ) ;
#107564=CARTESIAN_POINT ( 'NONE',  ( -0.1750448602389990116, 1463.552070523890052, 202.0965116382990061 ) ) ;
#107572=CARTESIAN_POINT ( 'NONE',  ( -12.25240435165759934, 1490.361895997039937, 209.2004140072839959 ) ) ;
#107573=CARTESIAN_POINT ( 'NONE',  ( -4.036901419354849807, 1508.551704408389924, 204.6714407391750115 ) ) ;
#107577=LINE ( 'NONE', #91329, #21572 ) ;
#107580=CARTESIAN_POINT ( 'NONE',  ( 9.901850170015880082, 1470.206455802750042, 211.0690064422630030 ) ) ;
#107587=CARTESIAN_POINT ( 'NONE',  ( -16.58048539533550070, 1464.422290153699805, 220.5762272166699915 ) ) ;
#107594=CARTESIAN_POINT ( 'NONE',  ( -21.10523119420000171, 1505.940419546890098, 209.1830678612959957 ) ) ;
#107600=ORIENTED_EDGE ( 'NONE', *, *, #72798, .F. ) ;
#107604=ORIENTED_EDGE ( 'NONE', *, *, #98663, .T. ) ;
#107608=CARTESIAN_POINT ( 'NONE',  ( -0.03631497420734799975, 1485.874503519110021, 221.0111561022920057 ) ) ;
#107619=CARTESIAN_POINT ( 'NONE',  ( 10.53166116164130095, 1481.128123199839820, 211.0446672586460011 ) ) ;
#107621=CARTESIAN_POINT ( 'NONE',  ( 4.869069343142859552, 1508.551704408389924, 212.3687905588049887 ) ) ;
#107625=CARTESIAN_POINT ( 'NONE',  ( -5.221955787189999754, 1489.269541098190075, 185.8916489435990229 ) ) ;
#107631=CARTESIAN_POINT ( 'NONE',  ( 12.26246110829129954, 1499.794402872200180, 205.9643549718410043 ) ) ;
#107637=CARTESIAN_POINT ( 'NONE',  ( -0.1906498135749990219, 1465.356101280390021, 198.0942218014990033 ) ) ;
#107644=CARTESIAN_POINT ( 'NONE',  ( 9.146299198640271300, 1461.861878385089767, 205.8341600298289791 ) ) ;
#107646=ORIENTED_EDGE ( 'NONE', *, *, #10056, .T. ) ;
#107649=ORIENTED_EDGE ( 'NONE', *, *, #13601, .T. ) ;
#107652=CARTESIAN_POINT ( 'NONE',  ( -17.96672434486609760, 1508.456899395794380, 211.9397210758587562 ) ) ;
#107672=CARTESIAN_POINT ( 'NONE',  ( -11.50563503569702029, 1508.158922853092690, 207.5673892822083531 ) ) ;
#107675=CARTESIAN_POINT ( 'NONE',  ( 2.317514236480000100, 1508.438296843690068, 220.2276651528989930 ) ) ;
#107678=CARTESIAN_POINT ( 'NONE',  ( -7.825739482554860516, 1440.186617985560133, 204.8166144522810157 ) ) ;
#107682=CARTESIAN_POINT ( 'NONE',  ( -8.588755447433969792, 1437.818850531529961, 207.9413692731380081 ) ) ;
#107689=EDGE_CURVE ( 'NONE', #36047, #75555, #53749, .T. ) ;
#107693=CARTESIAN_POINT ( 'NONE',  ( 2.137144914719688593, 1464.211915265456355, 199.5352916986041976 ) ) ;
#107696=CARTESIAN_POINT ( 'NONE',  ( -6.648038047673147766, 1439.929303981514749, 203.4146418879364830 ) ) ;
#107700=CARTESIAN_POINT ( 'NONE',  ( -1.754420609230000094, 1507.305123787589991, 221.4484239625990085 ) ) ;
#107718=CARTESIAN_POINT ( 'NONE',  ( 12.80045406827199983, 1421.352217623579918, 205.8583691802969895 ) ) ;
#107721=CARTESIAN_POINT ( 'NONE',  ( -19.83329619529999732, 1467.071755593990019, 210.0771979357010082 ) ) ;
#107722=CARTESIAN_POINT ( 'NONE',  ( 3.217370068945899941, 1424.184623523179880, 188.9579833762999783 ) ) ;
#107726=CARTESIAN_POINT ( 'NONE',  ( -6.923625731939999639, 1452.810235840890073, 202.5026240206190096 ) ) ;
#107727=EDGE_CURVE ( 'NONE', #1510, #2790, #39403, .T. ) ;
#107729=CARTESIAN_POINT ( 'NONE',  ( 8.061555088029999538, 1427.901936262589970, 212.7968812046490257 ) ) ;
#107730=CARTESIAN_POINT ( 'NONE',  ( -21.46486174369999844, 1504.440211354589792, 215.6677629392290214 ) ) ;
#107740=LINE ( 'NONE', #47289, #84240 ) ;
#107743=CARTESIAN_POINT ( 'NONE',  ( -15.54057306903361102, 1416.153203235703131, 210.7896593000916994 ) ) ;
#107744=CARTESIAN_POINT ( 'NONE',  ( 2.978012241769999680, 1445.410371645589976, 200.4888750985090269 ) ) ;
#107767=CARTESIAN_POINT ( 'NONE',  ( -12.33148714679999891, 1502.584565209489938, 208.9079283441639916 ) ) ;
#107774=CARTESIAN_POINT ( 'NONE',  ( -9.003774537682598833, 1451.190698364410082, 206.9733706270170046 ) ) ;
#107792=CARTESIAN_POINT ( 'NONE',  ( 12.13997568453070031, 1492.634789084120030, 211.4080700421230006 ) ) ;
#107803=CARTESIAN_POINT ( 'NONE',  ( 10.38136293079987027, 1472.225397094090113, 214.0145097960788689 ) ) ;
#107804=CARTESIAN_POINT ( 'NONE',  ( 12.92606856909999991, 1421.113610090889779, 204.2842550098989989 ) ) ;
#107805=CARTESIAN_POINT ( 'NONE',  ( -2.753739293390117471, 1497.642705930136572, 198.1704566312156999 ) ) ;
#107808=CARTESIAN_POINT ( 'NONE',  ( -1.027716997790000031, 1461.008287043790233, 228.8024499230989761 ) ) ;
#107809=CARTESIAN_POINT ( 'NONE',  ( 1.250333271336267371, 1515.565566433146614, 205.1761050331341494 ) ) ;
#107817=CARTESIAN_POINT ( 'NONE',  ( 10.94382554143900066, 1461.342062594439994, 209.7546787681809803 ) ) ;
#107818=EDGE_CURVE ( 'NONE', #76431, #19773, #93021, .T. ) ;
#107820=CARTESIAN_POINT ( 'NONE',  ( 2.657280408040000097, 1442.422209172990051, 217.7150463564190090 ) ) ;
#107833=CARTESIAN_POINT ( 'NONE',  ( -5.787667333660000857, 1484.577386382489976, 199.2118433045889958 ) ) ;
#107836=CARTESIAN_POINT ( 'NONE',  ( -8.616829302300699212, 1437.329206855350094, 209.9044458843100074 ) ) ;
#107839=CARTESIAN_POINT ( 'NONE',  ( -14.23978842837620107, 1415.677402202509938, 204.6746519906900232 ) ) ;
#107847=ORIENTED_EDGE ( 'NONE', *, *, #78321, .F. ) ;
#107850=CARTESIAN_POINT ( 'NONE',  ( 4.001542931430000394, 1454.513261907689866, 217.6365205154789919 ) ) ;
#107855=CARTESIAN_POINT ( 'NONE',  ( 9.067032342309868653, 1422.697473864469885, 213.1748852504530021 ) ) ;
#107856=CARTESIAN_POINT ( 'NONE',  ( 9.355425336389100011, 1464.485869949779953, 212.1516644132140073 ) ) ;
#107858=CARTESIAN_POINT ( 'NONE',  ( 0.8972167984987801104, 1515.116734647830071, 213.4499345946999824 ) ) ;
#107860=CARTESIAN_POINT ( 'NONE',  ( -4.063907090412950396, 1476.726422537800090, 219.8840548534849972 ) ) ;
#107868=CARTESIAN_POINT ( 'NONE',  ( -13.63402676890000009, 1504.645044512890081, 227.7399864453990119 ) ) ;
#107873=CARTESIAN_POINT ( 'NONE',  ( 4.327045307009350417, 1515.156577661779920, 209.3136710241140008 ) ) ;
#107875=CARTESIAN_POINT ( 'NONE',  ( 18.07842109055869884, 1431.201698177569824, 206.4737439103550116 ) ) ;
#107876=CARTESIAN_POINT ( 'NONE',  ( -3.840975779399999901, 1458.116743529589939, 218.6763403738689817 ) ) ;
#107881=ORIENTED_EDGE ( 'NONE', *, *, #70506, .F. ) ;
#107910=CARTESIAN_POINT ( 'NONE',  ( -18.26023438560000045, 1443.256148476890075, 213.5656046648789754 ) ) ;
#107911=CARTESIAN_POINT ( 'NONE',  ( 3.750000000000000000, 1524.051704408389924, 209.1218459616989946 ) ) ;
#107913=CARTESIAN_POINT ( 'NONE',  ( 4.093827366729640538, 1442.069873536569730, 216.9756443559270167 ) ) ;
#107918=CARTESIAN_POINT ( 'NONE',  ( -7.973546373915826990, 1425.245985973295547, 205.1887633420602413 ) ) ;
#107920=CARTESIAN_POINT ( 'NONE',  ( -10.03141724199999985, 1472.765117119090064, 207.2972502656089944 ) ) ;
#107922=ORIENTED_EDGE ( 'NONE', *, *, #80171, .F. ) ;
#107932=B_SPLINE_CURVE_WITH_KNOTS ( 'NONE', 3,
 ( #75146, #14662, #24689, #92461, #33114, #15732, #41533, #101961, #109293, #25247, #84071, #31463, #67849, #93018, #83512, #100327, #66754, #32578, #23612, #57799, #7911, #108728, #75691, #32018, #67301, #59450, #42082, #16834 ),
 .UNSPECIFIED., .F., .F.,
 ( 4, 3, 3, 3, 3, 3, 3, 3, 3, 4 ),
 ( -7.332849270026669863, -7.070672308253410421, -6.683016686340660151, -6.206605020891959867, -5.597668811241430120, -5.172869050969330473, -4.989338611940850043, -4.363064878034809801, -3.699273191951379935, -3.012888606410000669 ),
 .UNSPECIFIED. ) ;
#107936=LINE ( 'NONE', #65410, #12065 ) ;
#107938=VERTEX_POINT ( 'NONE', #33733 ) ;
#107939=CARTESIAN_POINT ( 'NONE',  ( -17.43675232709999889, 1417.688629781069949, 206.2161169699189713 ) ) ;
#107943=CARTESIAN_POINT ( 'NONE',  ( -1.062931043700000133, 1475.464638824089889, 220.1331094441989933 ) ) ;
#107948=CARTESIAN_POINT ( 'NONE',  ( -2.283851398302360280, 1454.773268660870144, 198.8765668124689796 ) ) ;
#107951=CARTESIAN_POINT ( 'NONE',  ( -10.12171546665249977, 1470.644541919200037, 212.0628956816030097 ) ) ;
#107958=CARTESIAN_POINT ( 'NONE',  ( 7.472831402659999789, 1423.077331640449984, 195.6326729942990141 ) ) ;
#107959=DIRECTION ( 'NONE',  ( 0.1867471702549220458, -2.391457216852619248E-16, -0.9824080081115885710 ) ) ;
#107961=CARTESIAN_POINT ( 'NONE',  ( -0.9649234502016059700, 1508.551704408389924, 220.0742041972960124 ) ) ;
#107971=CARTESIAN_POINT ( 'NONE',  ( 3.780333224634049749, 1508.551704408389924, 204.4954358679670179 ) ) ;
#107973=ORIENTED_EDGE ( 'NONE', *, *, #72032, .T. ) ;
#107974=CARTESIAN_POINT ( 'NONE',  ( -19.86622909784430036, 1443.388413634180097, 213.1207225405120198 ) ) ;
#107982=CARTESIAN_POINT ( 'NONE',  ( -10.16450165796499938, 1472.456210521550020, 207.1947926051400088 ) ) ;
#108004=CARTESIAN_POINT ( 'NONE',  ( -9.072363224181140495, 1449.404768024669920, 210.5087561342340052 ) ) ;
#108009=CARTESIAN_POINT ( 'NONE',  ( 7.041307337603809557, 1424.896087700059979, 213.1365174684090107 ) ) ;
#108017=CARTESIAN_POINT ( 'NONE',  ( -4.636716969933436516, 1378.031735257917717, 214.3255111405700575 ) ) ;
#108024=CARTESIAN_POINT ( 'NONE',  ( 9.760879523209998965, 1463.475536510490201, 209.9230695397520208 ) ) ;
#108035=EDGE_CURVE ( 'NONE', #39872, #3178, #36463, .T. ) ;
#108041=CARTESIAN_POINT ( 'NONE',  ( 5.952292128818620576, 1483.732806304819860, 219.3495610126499855 ) ) ;
#108046=CARTESIAN_POINT ( 'NONE',  ( -11.00988902727860008, 1481.333122227119929, 209.3333858298779830 ) ) ;
#108047=CARTESIAN_POINT ( 'NONE',  ( -2.654144332375780291, 1508.551704412109984, 220.2468185985560183 ) ) ;
#108048=ADVANCED_FACE ( 'NONE', ( #93630 ), #85652, .T. ) ;
#108051=CARTESIAN_POINT ( 'NONE',  ( 12.65754557789999879, 1420.238440408800216, 200.3470417333290072 ) ) ;
#108052=CARTESIAN_POINT ( 'NONE',  ( 18.79226589730000185, 1456.307606824690083, 213.7887498653890077 ) ) ;
#108054=CARTESIAN_POINT ( 'NONE',  ( 10.45814682399799977, 1479.299028883320034, 205.9955659561700259 ) ) ;
#108059=CARTESIAN_POINT ( 'NONE',  ( 10.66765284868029973, 1424.188739277350123, 206.6454873575900137 ) ) ;
#108060=CARTESIAN_POINT ( 'NONE',  ( -9.827361973644409332, 1439.976119166509989, 207.2092696800089868 ) ) ;
#108069=CARTESIAN_POINT ( 'NONE',  ( 10.62807384989510062, 1422.391294950000201, 210.1053146505880136 ) ) ;
#108070=CARTESIAN_POINT ( 'NONE',  ( 10.98461821322850085, 1423.291179694809898, 203.2749711373830337 ) ) ;
#108072=CARTESIAN_POINT ( 'NONE',  ( 3.975098305720000447, 1430.458171852989835, 217.7504258046890016 ) ) ;
#108077=B_SPLINE_SURFACE_WITH_KNOTS ( 'NONE', 5, 5, ( 
 ( #33969, #42371, #34524, #6147, #68165, #59743 ),
 ( #93864, #42939, #68705, #60866, #102809, #60294 ),
 ( #94412, #103937, #17689, #77638, #35076, #52454 ),
 ( #27235, #86583, #82857, #1492, #61415, #95538 ),
 ( #18811, #88251, #53006, #11544, #29978, #28897 ),
 ( #10430, #20463, #105050, #64170, #28339, #72035 ),
 ( #63091, #96087, #45163, #27783, #46277, #79303 ),
 ( #104490, #80404, #45719, #19363, #3717, #106150 ),
 ( #89346, #88800, #12082, #87140, #97189, #62534 ) ),
 .UNSPECIFIED., .F., .F., .F.,
 ( 6, 3, 6 ),
 ( 6, 6 ),
 ( 19.61749528909999896, 20.80534586139999931, 22.34240631349999973 ),
 ( 0.000000000000000000, 2.000000000000000000 ),
 .UNSPECIFIED. ) ;
#108078=CARTESIAN_POINT ( 'NONE',  ( 4.500000000000000000, 1508.551704408389924, 209.1218459616989946 ) ) ;
#108079=CARTESIAN_POINT ( 'NONE',  ( 3.429115760092809939, 1458.481892967550039, 200.0825522186730154 ) ) ;
#108090=CARTESIAN_POINT ( 'NONE',  ( 0.008286608639350531713, 1515.284302758789863, 204.7981455896689909 ) ) ;
#108104=CARTESIAN_POINT ( 'NONE',  ( 1.916663553690000077, 1477.644687611890049, 198.8912423807989853 ) ) ;
#108106=CARTESIAN_POINT ( 'NONE',  ( -11.79358356080000014, 1490.862585118089783, 208.2019470143079900 ) ) ;
#108114=CARTESIAN_POINT ( 'NONE',  ( -12.22815867699069869, 1490.645326540880205, 208.2429163971229968 ) ) ;
#108115=CARTESIAN_POINT ( 'NONE',  ( -4.987078426973329925, 1508.551704408389924, 206.6339106789369851 ) ) ;
#108116=ORIENTED_EDGE ( 'NONE', *, *, #36330, .F. ) ;
#108122=CARTESIAN_POINT ( 'NONE',  ( 10.89060804628219969, 1471.196313911609877, 210.4292383253470007 ) ) ;
#108124=CARTESIAN_POINT ( 'NONE',  ( 17.96908779310200188, 1430.390183715600187, 212.2284757796069812 ) ) ;
#108132=CARTESIAN_POINT ( 'NONE',  ( 1.012183099500000072, 1463.352738468689950, 230.5387435546990105 ) ) ;
#108139=CARTESIAN_POINT ( 'NONE',  ( -21.53565904410000087, 1506.077647802389947, 209.2113159668039941 ) ) ;
#108155=CARTESIAN_POINT ( 'NONE',  ( 11.40388019490000104, 1502.140095079889988, 207.7801577285290193 ) ) ;
#108159=EDGE_CURVE ( 'NONE', #88484, #42556, #80503, .T. ) ;
#108162=CARTESIAN_POINT ( 'NONE',  ( 12.47249016976989999, 1501.230039276080106, 211.6023161739269938 ) ) ;
#108164=EDGE_CURVE ( 'NONE', #77584, #26024, #55136, .T. ) ;
#108167=CARTESIAN_POINT ( 'NONE',  ( -20.43379574667769916, 1466.940197274710044, 211.2182803883939926 ) ) ;
#108173=CARTESIAN_POINT ( 'NONE',  ( -18.41923349776079633, 1508.551704408389924, 210.4158544684339915 ) ) ;
#108177=CARTESIAN_POINT ( 'NONE',  ( 1.946844730679999858, 1465.062448901589960, 199.3137936548990012 ) ) ;
#108194=CIRCLE ( 'NONE', #58172, 11.73843354579999954 ) ;
#108195=CARTESIAN_POINT ( 'NONE',  ( -10.17685046697009987, 1462.839848933360145, 206.1631249775429922 ) ) ;
#108204=B_SPLINE_SURFACE_WITH_KNOTS ( 'NONE', 5, 5, ( 
 ( #52804, #88065, #43295, #44965, #69063, #43840 ),
 ( #744, #95343, #25904, #9129, #104295, #11351 ),
 ( #18604, #203, #34875, #103164, #26465, #60660 ),
 ( #35432, #34326, #69619, #45522, #86935, #36537 ),
 ( #94785, #18062, #52256, #9668, #19153, #10226 ),
 ( #60102, #35995, #94218, #70185, #28134, #44404 ),
 ( #17493, #10795, #77986, #61767, #1292, #27582 ),
 ( #95893, #53360, #62325, #51691, #79113, #70734 ),
 ( #104847, #96450, #85832, #28695, #89144, #97009 ) ),
 .UNSPECIFIED., .F., .F., .F.,
 ( 6, 3, 6 ),
 ( 6, 6 ),
 ( 3.139241426659999945, 5.400505795499999984, 7.661770164330000021 ),
 ( 0.000000000000000000, 2.000000000000000000 ),
 .UNSPECIFIED. ) ;
#108207=CARTESIAN_POINT ( 'NONE',  ( -5.334733590569999073, 1453.182326120890139, 200.0999779489789887 ) ) ;
#108214=CARTESIAN_POINT ( 'NONE',  ( -11.82500768155940030, 1501.487207883790006, 211.3803078134539817 ) ) ;
#108217=FACE_OUTER_BOUND ( 'NONE', #110236, .T. ) ;
#108221=CARTESIAN_POINT ( 'NONE',  ( -18.80392059315889952, 1444.590799732510050, 207.5778593429040200 ) ) ;
#108222=CARTESIAN_POINT ( 'NONE',  ( 12.65728676410210163, 1420.119835224449844, 200.3472210950669989 ) ) ;
#108223=CARTESIAN_POINT ( 'NONE',  ( -5.560649665117820106, 1476.805467003079912, 214.4102409124259907 ) ) ;
#108226=CARTESIAN_POINT ( 'NONE',  ( -12.78943302956389871, 1502.708798875820094, 209.0180534851929792 ) ) ;
#108234=CARTESIAN_POINT ( 'NONE',  ( 10.86989410202379958, 1489.795966696680125, 207.8815529146370125 ) ) ;
#108239=CARTESIAN_POINT ( 'NONE',  ( -10.22015420455159962, 1447.362584368680018, 210.7051702221340008 ) ) ;
#108243=B_SPLINE_SURFACE_WITH_KNOTS ( 'NONE', 5, 5, ( 
 ( #52671, #44832, #26334, #95761, #52121, #96316 ),
 ( #85695, #19026, #10097, #34197, #70050, #35301 ),
 ( #103609, #44272, #36401, #43709, #70593, #78415 ),
 ( #2289, #104161, #94653, #616, #1170, #86249 ),
 ( #68936, #53229, #78986, #65, #87370, #9540 ),
 ( #104708, #85143, #8992, #77318, #1727, #43163 ),
 ( #26908, #77861, #61097, #34748, #28002, #95213 ),
 ( #27447, #8431, #42602, #35865, #76757, #68380 ),
 ( #25778, #59976, #94092, #17364, #19594, #62758 ) ),
 .UNSPECIFIED., .F., .F., .F.,
 ( 6, 3, 6 ),
 ( 6, 6 ),
 ( 4.218056259389999951, 8.316051950089999423, 13.74231060039999974 ),
 ( 0.000000000000000000, 2.000000000000000000 ),
 .UNSPECIFIED. ) ;
#108245=CARTESIAN_POINT ( 'NONE',  ( -10.29050077590000001, 1499.663130460889988, 214.7767004497089829 ) ) ;
#108246=CARTESIAN_POINT ( 'NONE',  ( -5.453001891610000484, 1437.869668061290213, 208.3330863909599771 ) ) ;
#108256=CARTESIAN_POINT ( 'NONE',  ( 4.240945049459830862, 1509.032014876047242, 212.8661584255399646 ) ) ;
#108265=CARTESIAN_POINT ( 'NONE',  ( 12.87612663444389938, 1421.246860338839952, 205.1732608065919976 ) ) ;
#108270=AXIS2_PLACEMENT_3D ( 'NONE', #31469, #72405, #47737 ) ;
#108271=CARTESIAN_POINT ( 'NONE',  ( -14.38097912129089906, 1422.143799352299993, 196.2925665020329973 ) ) ;
#108272=CARTESIAN_POINT ( 'NONE',  ( -16.49435349732149803, 1417.029099322570119, 208.6185211527730132 ) ) ;
#108273=DIRECTION ( 'NONE',  ( 1.000000000000000000, 2.249639673992789970E-32, 1.224646799147350002E-16 ) ) ;
#108274=DIRECTION ( 'NONE',  ( -1.000000000000000000, 0.000000000000000000, 0.000000000000000000 ) ) ;
#108275=CARTESIAN_POINT ( 'NONE',  ( -8.532458278280000030, 1445.788163739789979, 215.0754535007789912 ) ) ;
#108276=CARTESIAN_POINT ( 'NONE',  ( -4.863842518140000237, 1453.445020719190097, 199.8398594391789800 ) ) ;
#108279=CARTESIAN_POINT ( 'NONE',  ( 7.477834654460000507, 1427.293509551050192, 212.7723093538689909 ) ) ;
#108282=CARTESIAN_POINT ( 'NONE',  ( -15.71863267061869962, 1420.991171932389989, 203.3936535414759703 ) ) ;
#108286=CARTESIAN_POINT ( 'NONE',  ( 10.13545555999999870, 1453.511788975089985, 212.2748783715589980 ) ) ;
#108291=ORIENTED_EDGE ( 'NONE', *, *, #66749, .F. ) ;
#108295=CARTESIAN_POINT ( 'NONE',  ( 2.189499658180000363, 1445.800293503789817, 199.2521182821290040 ) ) ;
#108299=CARTESIAN_POINT ( 'NONE',  ( -4.534957494478200068, 1464.558362628190025, 199.0720338271949856 ) ) ;
#108300=CARTESIAN_POINT ( 'NONE',  ( 1.225455118299999979, 1418.194176457360072, 204.0816376824290046 ) ) ;
#108302=EDGE_CURVE ( 'NONE', #642, #53387, #107055, .T. ) ;
#108309=VERTEX_POINT ( 'NONE', #45259 ) ;
#108312=CARTESIAN_POINT ( 'NONE',  ( -5.010230551890000328, 1425.855359004169941, 208.5321073727319856 ) ) ;
#108319=CARTESIAN_POINT ( 'NONE',  ( -11.42889282249999994, 1501.636458983090051, 208.2613504466779943 ) ) ;
#108322=AXIS2_PLACEMENT_3D ( 'NONE', #99601, #82814, #90104 ) ;
#108337=B_SPLINE_CURVE_WITH_KNOTS ( 'NONE', 5,
 ( #34966, #10889, #8650, #19818, #26563, #69715, #36089, #104941, #42827 ),
 .UNSPECIFIED., .F., .F.,
 ( 6, 3, 6 ),
 ( 234.6130002419999983, 237.3878297990000021, 239.4206172199999969 ),
 .UNSPECIFIED. ) ;
#108343=CARTESIAN_POINT ( 'NONE',  ( 12.03563314606459933, 1492.750536582230097, 211.9176864492389996 ) ) ;
#108352=ORIENTED_EDGE ( 'NONE', *, *, #13931, .T. ) ;
#108359=CARTESIAN_POINT ( 'NONE',  ( 11.51329883360000039, 1422.113191770029971, 206.0591625496990105 ) ) ;
#108360=CARTESIAN_POINT ( 'NONE',  ( 1.155535764753627292, 1498.748878490413290, 197.8505271270100252 ) ) ;
#108364=CARTESIAN_POINT ( 'NONE',  ( 2.981764508932377655, 1456.749145576906358, 198.8578630351947538 ) ) ;
#108371=CARTESIAN_POINT ( 'NONE',  ( 2.326513265190000013, 1476.258183643389884, 197.8633931559990060 ) ) ;
#108373=CARTESIAN_POINT ( 'NONE',  ( 8.913965239475833968, 1424.958290419335526, 195.7060191906770399 ) ) ;
#108374=CARTESIAN_POINT ( 'NONE',  ( -1.349081561059999990, 1443.127676870989944, 219.0403161255090083 ) ) ;
#108379=CARTESIAN_POINT ( 'NONE',  ( 8.338382627507524347, 1487.567140753732701, 202.1928651156333956 ) ) ;
#108386=CARTESIAN_POINT ( 'NONE',  ( -9.526130908711980538, 1440.436523450050117, 205.9995045934610118 ) ) ;
#108394=CARTESIAN_POINT ( 'NONE',  ( -2.849562163009459859, 1515.551843419029865, 213.1048050409179950 ) ) ;
#108399=ORIENTED_EDGE ( 'NONE', *, *, #56286, .T. ) ;
#108400=DIRECTION ( 'NONE',  ( -1.000000000000000000, 0.000000000000000000, 0.000000000000000000 ) ) ;
#108401=EDGE_CURVE ( 'NONE', #38113, #1907, #46979, .T. ) ;
#108407=FACE_OUTER_BOUND ( 'NONE', #456, .T. ) ;
#108409=CARTESIAN_POINT ( 'NONE',  ( -1.795663807680000001, 1444.786284551390054, 217.9357666183690014 ) ) ;
#108426=CARTESIAN_POINT ( 'NONE',  ( -18.81286786266959865, 1505.121906714500028, 222.5033949973810081 ) ) ;
#108431=CARTESIAN_POINT ( 'NONE',  ( 4.327012391429460259, 1515.157834657049989, 209.2496350220929742 ) ) ;
#108434=CARTESIAN_POINT ( 'NONE',  ( -4.329448776275169664, 1515.064792882719985, 206.7917118343879963 ) ) ;
#108435=B_SPLINE_CURVE_WITH_KNOTS ( 'NONE', 3,
 ( #34691, #16753, #101876, #102436, #94588, #7290, #76149, #50417, #43108, #52066, #32499, #92942, #68881, #49857, #41454, #26281, #76696, #102983, #59922, #8375, #60470, #17868 ),
 .UNSPECIFIED., .F., .F.,
 ( 4, 2, 2, 1, 1, 1, 1, 2, 2, 2, 2, 2, 4 ),
 ( 0.000000000000000000, 0.2499999999991435740, 0.3749999999987154720, 0.4374999999985075827, 0.4687499999983973931, 0.4843749999983563703, 0.4921874999983420484, 0.4960937499983150145, 0.4999999999982880361, 0.6249999999986949328, 0.6874999999989206412, 0.7499999999991464605, 1.000000000000000000 ),
 .UNSPECIFIED. ) ;
#108439=CARTESIAN_POINT ( 'NONE',  ( -4.328570061217769549, 1515.098349647940040, 210.2573761392540064 ) ) ;
#108448=CARTESIAN_POINT ( 'NONE',  ( -17.64822974267435640, 1419.534037284996202, 207.1517795833794935 ) ) ;
#108465=CARTESIAN_POINT ( 'NONE',  ( 10.87353205008450097, 1460.686552688219990, 207.9238305753009683 ) ) ;
#108474=ORIENTED_EDGE ( 'NONE', *, *, #48835, .T. ) ;
#108478=CARTESIAN_POINT ( 'NONE',  ( -10.57604552250000118, 1471.371694624089741, 208.7882177754879933 ) ) ;
#108482=CARTESIAN_POINT ( 'NONE',  ( 20.21728935790000037, 1475.862786327189951, 209.1218459616989946 ) ) ;
#108485=CARTESIAN_POINT ( 'NONE',  ( -11.95964865010000011, 1416.297031888519996, 205.9046802826989904 ) ) ;
#108488=CARTESIAN_POINT ( 'NONE',  ( 7.407046107680000269, 1488.581653516390134, 199.5623810922690211 ) ) ;
#108495=CARTESIAN_POINT ( 'NONE',  ( -17.58082291759999904, 1417.836406065290021, 206.7640894888989749 ) ) ;
#108497=CARTESIAN_POINT ( 'NONE',  ( -17.45313156558830059, 1508.551704408389924, 211.9416870107529860 ) ) ;
#108501=CARTESIAN_POINT ( 'NONE',  ( -7.145324146093005702, 1508.387575007782061, 219.7168039286800081 ) ) ;
#108503=CARTESIAN_POINT ( 'NONE',  ( -1.791500013333100050, 1454.995498928959933, 198.7702412911150134 ) ) ;
#108506=CARTESIAN_POINT ( 'NONE',  ( -10.26287757781059895, 1470.737246754300031, 211.5706239509080149 ) ) ;
#108509=ORIENTED_EDGE ( 'NONE', *, *, #29151, .T. ) ;
#108514=CARTESIAN_POINT ( 'NONE',  ( 11.53450314954949896, 1502.145229493909937, 211.3292107343589805 ) ) ;
#108515=FACE_OUTER_BOUND ( 'NONE', #44720, .T. ) ;
#108518=CARTESIAN_POINT ( 'NONE',  ( 1.473600209469299926, 1508.551704408389924, 219.7879707489230157 ) ) ;
#108522=CARTESIAN_POINT ( 'NONE',  ( -12.01522815608920070, 1502.252156548509902, 208.9183199409420126 ) ) ;
#108523=CARTESIAN_POINT ( 'NONE',  ( 12.08872186521969994, 1492.701414612239887, 211.6956945743199867 ) ) ;
#108524=CARTESIAN_POINT ( 'NONE',  ( -2.525609700800000024, 1456.035086478289941, 218.2565648270789609 ) ) ;
#108530=CARTESIAN_POINT ( 'NONE',  ( 3.246944597107860098, 1508.551704408389924, 204.2527766185579878 ) ) ;
#108534=CARTESIAN_POINT ( 'NONE',  ( -4.325403553846939531, 1515.219291385629958, 206.7919471186340274 ) ) ;
#108536=CARTESIAN_POINT ( 'NONE',  ( -9.519812938348620079, 1460.017558366200092, 210.6311618255110147 ) ) ;
#108537=CARTESIAN_POINT ( 'NONE',  ( -5.452217511760000690, 1462.447772966889943, 201.0260644561890047 ) ) ;
#108541=CARTESIAN_POINT ( 'NONE',  ( -13.81128163186000002, 1508.551704408389924, 215.9575079269010018 ) ) ;
#108545=CARTESIAN_POINT ( 'NONE',  ( 8.562350050396240420, 1433.778962878430093, 204.3790883806010186 ) ) ;
#108569=CARTESIAN_POINT ( 'NONE',  ( 6.965382933308789326, 1424.882428658780100, 213.2657788462730082 ) ) ;
#108579=CARTESIAN_POINT ( 'NONE',  ( -5.080289282479999002, 1480.093209919690253, 228.8812397303989883 ) ) ;
#108581=B_SPLINE_CURVE_WITH_KNOTS ( 'NONE', 3,
 ( #11930, #95936, #36578, #89730, #53398, #88103, #4630, #62938 ),
 .UNSPECIFIED., .F., .F.,
 ( 4, 2, 2, 4 ),
 ( -0.08162639889109629676, -0.08079092939402009177, -0.04068425817429450336, 0.000000000000000000 ),
 .UNSPECIFIED. ) ;
#108587=CARTESIAN_POINT ( 'NONE',  ( 10.10980088610000038, 1462.073314986889955, 210.1684032625090026 ) ) ;
#108594=VECTOR ( 'NONE', #84401, 1000.000000000000114 ) ;
#108598=VERTEX_POINT ( 'NONE', #94953 ) ;
#108601=CARTESIAN_POINT ( 'NONE',  ( -6.992186432439999599, 1426.424829897749987, 202.7541583518589903 ) ) ;
#108608=CARTESIAN_POINT ( 'NONE',  ( 4.832611339330939337, 1508.551704408389924, 206.6339237841029899 ) ) ;
#108611=CARTESIAN_POINT ( 'NONE',  ( 6.454219559888790592, 1504.605177847159894, 220.1239436410009773 ) ) ;
#108613=CARTESIAN_POINT ( 'NONE',  ( 0.4691691604916909952, 1431.662181100700082, 218.6011377030980043 ) ) ;
#108614=CARTESIAN_POINT ( 'NONE',  ( -8.829505046341829200, 1493.480017849250089, 200.5570910297369949 ) ) ;
#108615=CARTESIAN_POINT ( 'NONE',  ( -4.677432903610000636, 1495.589319749489960, 198.5260162735989695 ) ) ;
#108616=CARTESIAN_POINT ( 'NONE',  ( 4.124127541549999165, 1440.791920158089852, 218.1322488136489994 ) ) ;
#108620=CARTESIAN_POINT ( 'NONE',  ( 10.82955669553860112, 1425.268927654319896, 206.5179382998420010 ) ) ;
#108630=CARTESIAN_POINT ( 'NONE',  ( 10.97092914054660007, 1423.389121826950031, 203.2629501824719966 ) ) ;
#108632=CARTESIAN_POINT ( 'NONE',  ( 1.188910551360000012, 1429.998391900489878, 217.3728214398389866 ) ) ;
#108634=CARTESIAN_POINT ( 'NONE',  ( -16.70830602919999919, 1417.149230822529944, 207.3570811876390110 ) ) ;
#108638=B_SPLINE_CURVE_WITH_KNOTS ( 'NONE', 5,
 ( #25273, #16860, #40992, #33138, #101424, #110404, #59474, #6832, #75171, #60026, #124, #109321 ),
 .UNSPECIFIED., .F., .F.,
 ( 6, 3, 3, 6 ),
 ( 0.000000000000000000, 0.2395393521504640966, 0.6197696760997779553, 1.000000000000000000 ),
 .UNSPECIFIED. ) ;
#108648=CARTESIAN_POINT ( 'NONE',  ( -4.125529553939999872, 1479.921875556590066, 229.1190508355989834 ) ) ;
#108650=CARTESIAN_POINT ( 'NONE',  ( 1.081422847559999845, 1515.099766759590011, 204.7933130088590019 ) ) ;
#108652=CARTESIAN_POINT ( 'NONE',  ( 4.677562527581470064, 1434.889072014880185, 228.7640133665269957 ) ) ;
#108658=CARTESIAN_POINT ( 'NONE',  ( -1.637258856660000150, 1483.893433971690001, 198.5669146070989939 ) ) ;
#108662=ORIENTED_EDGE ( 'NONE', *, *, #32981, .F. ) ;
#108667=FACE_OUTER_BOUND ( 'NONE', #14794, .T. ) ;
#108668=VECTOR ( 'NONE', #7304, 1000.000000000000114 ) ;
#108675=CARTESIAN_POINT ( 'NONE',  ( -4.363624498282149489, 1508.551704408389924, 204.9809794401540159 ) ) ;
#108676=ORIENTED_EDGE ( 'NONE', *, *, #48711, .F. ) ;
#108682=CARTESIAN_POINT ( 'NONE',  ( 2.720194589200000124, 1473.666501463190116, 219.1326999374989839 ) ) ;
#108683=CARTESIAN_POINT ( 'NONE',  ( 9.936615814174009742, 1469.595287704849852, 210.7004918180149957 ) ) ;
#108701=CARTESIAN_POINT ( 'NONE',  ( 3.127269064749419236, 1466.004634090720629, 199.2798694621438926 ) ) ;
#108709=CARTESIAN_POINT ( 'NONE',  ( -1.427070966906029970, 1486.249699017309922, 220.9490979875029950 ) ) ;
#108710=CARTESIAN_POINT ( 'NONE',  ( 11.57530258789999955, 1501.342160219190191, 208.5271145533289996 ) ) ;
#108717=CARTESIAN_POINT ( 'NONE',  ( 12.63405317313929821, 1500.911264070530024, 210.5278134812520250 ) ) ;
#108720=( BOUNDED_CURVE ( )  B_SPLINE_CURVE ( 3, ( #84357, #101687, #24978, #17675 ),
 .UNSPECIFIED., .F., .T. ) 
 B_SPLINE_CURVE_WITH_KNOTS ( ( 4, 4 ),
 ( 1.021750339367931915, 2.119842335967295099 ),
 .UNSPECIFIED. ) 
 CURVE ( )  GEOMETRIC_REPRESENTATION_ITEM ( )  RATIONAL_B_SPLINE_CURVE ( ( 1.000000000000000000, 0.9020151856930300749, 0.9020151856930300749, 1.000000000000000000 ) ) 
 REPRESENTATION_ITEM ( '' )  );
#108723=CARTESIAN_POINT ( 'NONE',  ( -21.46486174369999844, 1504.440211354589792, 215.6677629392290214 ) ) ;
#108726=VERTEX_POINT ( 'NONE', #53524 ) ;
#108727=CARTESIAN_POINT ( 'NONE',  ( -0.1267786306729990209, 1432.696254167089819, 203.3330887969689798 ) ) ;
#108728=CARTESIAN_POINT ( 'NONE',  ( 10.34090598038000053, 1453.264473920479759, 211.4883971156640143 ) ) ;
#108729=CARTESIAN_POINT ( 'NONE',  ( 12.58710147329349915, 1500.144068373949949, 207.5432606781910181 ) ) ;
#108731=CARTESIAN_POINT ( 'NONE',  ( -2.330134125103331844, 1515.320037165259464, 213.3925622817942553 ) ) ;
#108740=EDGE_LOOP ( 'NONE', ( #20174, #88347, #52652, #93798 ) ) ;
#108743=ORIENTED_EDGE ( 'NONE', *, *, #95662, .F. ) ;
#108747=CARTESIAN_POINT ( 'NONE',  ( -2.664535259099999805E-15, 1424.786834349990158, 209.1218459616989946 ) ) ;
#108750=CARTESIAN_POINT ( 'NONE',  ( -9.841064997534830994, 1462.508760387780057, 206.4810345683729906 ) ) ;
#108761=VERTEX_POINT ( 'NONE', #12049 ) ;
#108771=CARTESIAN_POINT ( 'NONE',  ( 2.876567151200000172, 1508.185761598690078, 220.3556610966990092 ) ) ;
#108773=CARTESIAN_POINT ( 'NONE',  ( -2.026117440780000223, 1436.275455653890049, 227.5319773123989933 ) ) ;
#108777=VECTOR ( 'NONE', #34001, 1000.000000000000227 ) ;
#108778=CARTESIAN_POINT ( 'NONE',  ( -4.285402615378519187, 1475.851751799939848, 215.4336415230879993 ) ) ;
#108779=B_SPLINE_CURVE_WITH_KNOTS ( 'NONE', 3,
 ( #73943, #65552, #55498, #82876, #89625, #106978, #40323, #31921, #30266, #21841, #23517, #66114, #12913, #91826, #49295, #47093, #56038, #555, #92929, #51490, #7819 ),
 .UNSPECIFIED., .F., .F.,
 ( 4, 2, 2, 2, 1, 1, 1, 1, 1, 2, 2, 2, 4 ),
 ( 0.000000000000000000, 0.2499999999978126386, 0.3749999999967190689, 0.4374999999961580177, 0.4687499999958776309, 0.4843749999957374097, 0.4921874999956772911, 0.4960937499956372121, 0.4980468749956170060, 0.4990234374956199481, 0.4999999999956228902, 0.7499999999978114174, 1.000000000000000000 ),
 .UNSPECIFIED. ) ;
#108796=CARTESIAN_POINT ( 'NONE',  ( -3.179033943583710276, 1457.997354099609993, 219.3203918230290128 ) ) ;
#108800=CARTESIAN_POINT ( 'NONE',  ( -4.287908595200000228, 1515.369371658090131, 209.8551202939650011 ) ) ;
#108801=CARTESIAN_POINT ( 'NONE',  ( -5.481756276210000500, 1437.661022548789788, 208.5938030632829907 ) ) ;
#108808=LINE ( 'NONE', #83056, #103923 ) ;
#108817=CARTESIAN_POINT ( 'NONE',  ( 10.84130981773069990, 1478.843033899609964, 205.9626931864170274 ) ) ;
#108819=ADVANCED_FACE ( 'NONE', ( #69782 ), #61594, .T. ) ;
#108821=CARTESIAN_POINT ( 'NONE',  ( -13.59157698562750127, 1508.214338131689829, 209.5916190095410059 ) ) ;
#108822=CARTESIAN_POINT ( 'NONE',  ( 18.38166056955379801, 1428.164368491259893, 201.4944003554669791 ) ) ;
#108823=CARTESIAN_POINT ( 'NONE',  ( -16.03814159374950066, 1416.346020389309842, 209.5174529804690167 ) ) ;
#108826=DIRECTION ( 'NONE',  ( -1.224646799147353947E-16, 1.836970198721029688E-16, 1.000000000000000000 ) ) ;
#108829=CARTESIAN_POINT ( 'NONE',  ( -4.848919996459999382, 1489.192135936889827, 188.8958457811990002 ) ) ;
#108836=ORIENTED_EDGE ( 'NONE', *, *, #15071, .F. ) ;
#108845=CARTESIAN_POINT ( 'NONE',  ( 0.7786077578810010058, 1443.353418816490148, 200.2227257021989715 ) ) ;
#108861=CARTESIAN_POINT ( 'NONE',  ( -4.924195455119999565, 1424.762629879490078, 209.7208662265510100 ) ) ;
#108868=B_SPLINE_CURVE_WITH_KNOTS ( 'NONE', 3,
 ( #22838, #100122, #91169, #47527, #31262, #57596, #40767, #55933, #14447, #64894, #13891, #66002, #40216, #108522, #83319, #74945, #81648, #13335, #91718, #5515, #38552, #14992, #29602, #99001, #39670, #97903, #89514, #4426, #4953, #39096, #73273, #30708, #22278, #73838 ),
 .UNSPECIFIED., .F., .F.,
 ( 4, 3, 3, 3, 3, 3, 3, 3, 3, 3, 3, 4 ),
 ( -2.000000000000000000, -1.856589768169299992, -1.673906318599919896, -1.488963774399080009, -1.302849350329150058, -1.115290844420000038, -0.9273284311027238935, -0.7394249586046770517, -0.5520371894422699821, -0.3663516837637139645, -0.1822529853692169688, 0.000000000000000000 ),
 .UNSPECIFIED. ) ;
#108869=ORIENTED_EDGE ( 'NONE', *, *, #60710, .T. ) ;
#108870=CARTESIAN_POINT ( 'NONE',  ( -12.86990655680000017, 1502.949917638090028, 208.7255105242149682 ) ) ;
#108882=VERTEX_POINT ( 'NONE', #54090 ) ;
#108892=CARTESIAN_POINT ( 'NONE',  ( 12.22337018873460046, 1492.513505122720062, 210.8907448166860092 ) ) ;
#108900=EDGE_CURVE ( 'NONE', #105726, #59860, #76315, .T. ) ;
#108907=EDGE_CURVE ( 'NONE', #31410, #104032, #68411, .T. ) ;
#108909=CARTESIAN_POINT ( 'NONE',  ( 9.986106302859869999, 1472.420748959189950, 214.7747459013789921 ) ) ;
#108910=CARTESIAN_POINT ( 'NONE',  ( 12.65362936969999907, 1421.491550492859915, 206.7389950482590280 ) ) ;
#108923=CARTESIAN_POINT ( 'NONE',  ( 10.82757510571090087, 1461.786499189259985, 210.8991486123640016 ) ) ;
#108927=CARTESIAN_POINT ( 'NONE',  ( 4.780307568339999591, 1467.625956517089890, 217.8721402715589761 ) ) ;
#108933=CARTESIAN_POINT ( 'NONE',  ( -20.61188484020000189, 1484.905759244990122, 208.1134661061090014 ) ) ;
#108937=ADVANCED_FACE ( 'NONE', ( #56814 ), #60689, .T. ) ;
#108944=CARTESIAN_POINT ( 'NONE',  ( -5.102344180470000268, 1483.010475857490064, 199.7820757393690201 ) ) ;
#108947=CARTESIAN_POINT ( 'NONE',  ( -8.651457448287009910, 1437.323783882450016, 208.9337525471009656 ) ) ;
#108948=CARTESIAN_POINT ( 'NONE',  ( -3.272146740928380204, 1515.551704204679936, 212.7661985179009889 ) ) ;
#108952=CARTESIAN_POINT ( 'NONE',  ( -15.28181346384849881, 1415.677402202079975, 208.7265255348459903 ) ) ;
#108955=CARTESIAN_POINT ( 'NONE',  ( -3.643503312559999596, 1432.730203132190127, 213.6018711577490024 ) ) ;
#108961=ORIENTED_EDGE ( 'NONE', *, *, #90559, .T. ) ;
#108965=CARTESIAN_POINT ( 'NONE',  ( 3.733372969449999967, 1456.065302378790193, 219.0848356464390179 ) ) ;
#108979=CARTESIAN_POINT ( 'NONE',  ( 6.225972109890000716, 1494.795958560490135, 219.7811165620990153 ) ) ;
#108984=CARTESIAN_POINT ( 'NONE',  ( 19.43854577420000140, 1499.207340252790118, 221.7758532508989902 ) ) ;
#108988=CARTESIAN_POINT ( 'NONE',  ( -14.65245215464970130, 1420.119839417710182, 213.8659310620899987 ) ) ;
#108993=CARTESIAN_POINT ( 'NONE',  ( -4.329341215434440393, 1515.068899831251429, 206.1636082373503598 ) ) ;
#108997=LINE ( 'NONE', #32283, #62766 ) ;
#109004=CARTESIAN_POINT ( 'NONE',  ( 5.838247866735959413, 1424.382028414360093, 193.5240377819480102 ) ) ;
#109020=CARTESIAN_POINT ( 'NONE',  ( -4.802552260849999755, 1482.676166849490073, 203.0569153438389947 ) ) ;
#109029=CARTESIAN_POINT ( 'NONE',  ( -1.925896724263820081, 1425.116320396220090, 191.2239611826650219 ) ) ;
#109038=ADVANCED_FACE ( 'NONE', ( #8455 ), #26668, .T. ) ;
#109040=ORIENTED_EDGE ( 'NONE', *, *, #79994, .T. ) ;
#109042=CARTESIAN_POINT ( 'NONE',  ( -8.630767090659189122, 1438.254930141910108, 208.1080191835690130 ) ) ;
#109045=CARTESIAN_POINT ( 'NONE',  ( 7.366459948930000223, 1481.681596261390041, 209.4342970301970013 ) ) ;
#109046=ADVANCED_FACE ( 'NONE', ( #49932 ), #64446, .F. ) ;
#109052=CARTESIAN_POINT ( 'NONE',  ( 5.634333898429999543, 1486.294848711289887, 199.9182129588890007 ) ) ;
#109057=CARTESIAN_POINT ( 'NONE',  ( -17.76922258761841888, 1445.720595802438993, 202.6296028318632523 ) ) ;
#109066=CARTESIAN_POINT ( 'NONE',  ( -1.176577584829999967, 1474.814957531289792, 219.4969863823990011 ) ) ;
#109068=CARTESIAN_POINT ( 'NONE',  ( -11.21541762013639953, 1471.302741629689990, 206.9949349079969920 ) ) ;
#109069=CARTESIAN_POINT ( 'NONE',  ( -5.719822330129272103, 1508.285359404909286, 220.2077194730133556 ) ) ;
#109072=CARTESIAN_POINT ( 'NONE',  ( -2.568069795494909879, 1454.639726342709992, 198.9496893171560146 ) ) ;
#109075=CARTESIAN_POINT ( 'NONE',  ( -10.14096832535920001, 1471.320523670169905, 210.8482381047599858 ) ) ;
#109076=CARTESIAN_POINT ( 'NONE',  ( 4.326992699989999913, 1515.158586642790169, 209.1218459614979963 ) ) ;
#109082=CARTESIAN_POINT ( 'NONE',  ( -2.044458700900000370, 1442.173530875790220, 200.4791613073190035 ) ) ;
#109084=CARTESIAN_POINT ( 'NONE',  ( 271.2574323654409909, 11216.44053380570040, 2234.264705616360061 ) ) ;
#109087=CARTESIAN_POINT ( 'NONE',  ( -1.253615010250130002, 1508.551704408389924, 220.0817883865630051 ) ) ;
#109090=CARTESIAN_POINT ( 'NONE',  ( -4.554948383327420025, 1508.731373119430145, 206.6339226617529903 ) ) ;
#109093=CARTESIAN_POINT ( 'NONE',  ( 10.51030381764329924, 1491.592991267690195, 212.4264936531670003 ) ) ;
#109094=CARTESIAN_POINT ( 'NONE',  ( -1.912679614370000003, 1457.559505151690018, 219.6146910743989906 ) ) ;
#109104=CARTESIAN_POINT ( 'NONE',  ( -3.465053098240730378, 1515.493282983300105, 205.2090698384729990 ) ) ;
#109108=CARTESIAN_POINT ( 'NONE',  ( -8.979645201780000363, 1461.875990298290162, 205.2600572402090222 ) ) ;
#109112=CARTESIAN_POINT ( 'NONE',  ( -9.924526517117328694, 1508.551704408389924, 218.3000131550199967 ) ) ;
#109117=CONICAL_SURFACE ( 'NONE', #8933, 6.911399307709998219, 0.04363323129990067523 ) ;
#109119=VERTEX_POINT ( 'NONE', #103634 ) ;
#109124=B_SPLINE_CURVE_WITH_KNOTS ( 'NONE', 5,
 ( #90753, #66143, #14032, #82364, #6197, #38694 ),
 .UNSPECIFIED., .F., .F.,
 ( 6, 6 ),
 ( 141.6155516059999968, 151.1003634729999874 ),
 .UNSPECIFIED. ) ;
#109126=CARTESIAN_POINT ( 'NONE',  ( 1.249673192637140273, 1515.565594798377106, 213.0676417522672637 ) ) ;
#109127=CARTESIAN_POINT ( 'NONE',  ( -14.86061390519999925, 1420.111516814780089, 213.2229217038190257 ) ) ;
#109133=CARTESIAN_POINT ( 'NONE',  ( -8.125957766200000876, 1425.045124160440082, 205.5278006110690114 ) ) ;
#109136=VECTOR ( 'NONE', #12259, 1000.000000000000227 ) ;
#109140=CARTESIAN_POINT ( 'NONE',  ( 7.513327647825819966, 1425.400186687669930, 212.2206837014999792 ) ) ;
#109143=CARTESIAN_POINT ( 'NONE',  ( -12.02051106306990036, 1491.153688555679992, 206.6632162730240054 ) ) ;
#109145=CARTESIAN_POINT ( 'NONE',  ( -19.41751478759999827, 1465.673884635790273, 205.2708586912889928 ) ) ;
#109155=CARTESIAN_POINT ( 'NONE',  ( 10.92766316885620093, 1501.618323021010156, 205.6861136770480130 ) ) ;
#109164=CARTESIAN_POINT ( 'NONE',  ( 4.833436809398059530, 1508.551704408489968, 212.3463955241550138 ) ) ;
#109165=ORIENTED_EDGE ( 'NONE', *, *, #74271, .T. ) ;
#109174=CARTESIAN_POINT ( 'NONE',  ( 17.22533712008139872, 1431.108080386279880, 215.5140119622810175 ) ) ;
#109176=CARTESIAN_POINT ( 'NONE',  ( -10.68155123028649989, 1480.766592174720017, 209.7229870821389852 ) ) ;
#109180=CARTESIAN_POINT ( 'NONE',  ( 9.991870921357078217, 1503.103680341759855, 217.0222761520359711 ) ) ;
#109181=ADVANCED_FACE ( 'NONE', ( #52144 ), #9697, .T. ) ;
#109182=CARTESIAN_POINT ( 'NONE',  ( 8.202111252990000878, 1421.417609776869767, 196.1188898363990063 ) ) ;
#109183=CARTESIAN_POINT ( 'NONE',  ( 0.8357676597613630243, 1431.531542961990226, 218.5749032632120077 ) ) ;
#109184=CARTESIAN_POINT ( 'NONE',  ( 10.02558921254980007, 1480.462737418800089, 205.8973177429729731 ) ) ;
#109188=CARTESIAN_POINT ( 'NONE',  ( 10.67226526208479775, 1424.091373414049940, 206.6618934297929968 ) ) ;
#109193=CARTESIAN_POINT ( 'NONE',  ( 0.7266811465689989591, 1473.184386732089934, 216.5181915634790073 ) ) ;
#109196=CARTESIAN_POINT ( 'NONE',  ( 3.552713678799999608E-15, 1415.677402202029953, 209.1218459616989946 ) ) ;
#109199=CARTESIAN_POINT ( 'NONE',  ( 10.96051199111599850, 1427.774010562269950, 210.4713807161799934 ) ) ;
#109200=CARTESIAN_POINT ( 'NONE',  ( 11.41161631220640160, 1425.396560188790090, 202.9572278001960228 ) ) ;
#109201=CARTESIAN_POINT ( 'NONE',  ( -10.95711598477149806, 1462.675152724350028, 207.6879324179139985 ) ) ;
#109210=CARTESIAN_POINT ( 'NONE',  ( 4.789658230336130806, 1465.867910918690086, 219.0701299224020033 ) ) ;
#109211=CARTESIAN_POINT ( 'NONE',  ( -10.25237617670000034, 1481.942191864189908, 205.9184019755789734 ) ) ;
#109213=CARTESIAN_POINT ( 'NONE',  ( 4.853172208638510732, 1474.073916305050034, 219.4636496197130100 ) ) ;
#109218=CARTESIAN_POINT ( 'NONE',  ( 0.7223987349950009573, 1515.137743094390089, 204.7943074541789770 ) ) ;
#109224=CARTESIAN_POINT ( 'NONE',  ( 9.905242068095489572, 1468.560492227489931, 207.6656469818879884 ) ) ;
#109233=CARTESIAN_POINT ( 'NONE',  ( -1.227669779950000040, 1484.909253711390193, 198.3212086688990041 ) ) ;
#109237=CARTESIAN_POINT ( 'NONE',  ( -7.817296349952290946, 1435.611607423119949, 212.8323433814960026 ) ) ;
#109239=CARTESIAN_POINT ( 'NONE',  ( -15.27521432969999893, 1416.121557574000008, 211.5121764755990057 ) ) ;
#109244=CARTESIAN_POINT ( 'NONE',  ( 10.80336067484410023, 1425.743873502309953, 206.7465275332850183 ) ) ;
#109245=ORIENTED_EDGE ( 'NONE', *, *, #25491, .F. ) ;
#109248=CARTESIAN_POINT ( 'NONE',  ( 1.494261883209599739, 1437.570713977159812, 227.6107760732709835 ) ) ;
#109249=ORIENTED_EDGE ( 'NONE', *, *, #48761, .F. ) ;
#109250=CARTESIAN_POINT ( 'NONE',  ( 3.296903354329999480, 1473.033302177089809, 218.8000070911390083 ) ) ;
#109251=CARTESIAN_POINT ( 'NONE',  ( 9.992887457760350145, 1469.445556547170099, 210.2216697196110147 ) ) ;
#109252=( BOUNDED_CURVE ( )  B_SPLINE_CURVE ( 3, ( #9677, #61236, #8570, #25911 ),
 .UNSPECIFIED., .F., .F. ) 
 B_SPLINE_CURVE_WITH_KNOTS ( ( 4, 4 ),
 ( 1.005056174319898021, 2.136536482083220001 ),
 .UNSPECIFIED. ) 
 CURVE ( )  GEOMETRIC_REPRESENTATION_ITEM ( )  RATIONAL_B_SPLINE_CURVE ( ( 1.000000000000000000, 0.8961280526803196977, 0.8961280526803196977, 1.000000000000000000 ) ) 
 REPRESENTATION_ITEM ( '' )  );
#109263=CARTESIAN_POINT ( 'NONE',  ( -0.2489806300479990020, 1456.626617263189928, 199.4885384397790062 ) ) ;
#109275=CARTESIAN_POINT ( 'NONE',  ( 12.17354065289999987, 1500.378712179390050, 207.7715712704689963 ) ) ;
#109288=CARTESIAN_POINT ( 'NONE',  ( -13.32684882476630150, 1469.522643478239843, 191.9925929742840083 ) ) ;
#109289=CARTESIAN_POINT ( 'NONE',  ( 4.487249775049700240, 1509.038615934839981, 206.6339108193819811 ) ) ;
#109291=EDGE_LOOP ( 'NONE', ( #22387, #26243, #60916, #90062 ) ) ;
#109293=CARTESIAN_POINT ( 'NONE',  ( 10.52582308400029909, 1452.864387279470066, 210.3124659236350169 ) ) ;
#109312=ORIENTED_EDGE ( 'NONE', *, *, #13962, .F. ) ;
#109318=CARTESIAN_POINT ( 'NONE',  ( -9.301208406426139774, 1461.161189386590195, 206.3998599881980169 ) ) ;
#109320=CARTESIAN_POINT ( 'NONE',  ( 9.916409037356570977, 1468.767901124550008, 207.5969806327450158 ) ) ;
#109321=CARTESIAN_POINT ( 'NONE',  ( -2.130922739038390024, 1467.954349360780043, 220.0452206896550251 ) ) ;
#109325=CARTESIAN_POINT ( 'NONE',  ( 2.487935141041626164, 1508.731359867455012, 213.6768079671783198 ) ) ;
#109334=CARTESIAN_POINT ( 'NONE',  ( 3.465053098240360008, 1515.493282983300105, 213.0346220849250187 ) ) ;
#109340=DIRECTION ( 'NONE',  ( 1.000000000000000000, 0.000000000000000000, 0.000000000000000000 ) ) ;
#109344=CARTESIAN_POINT ( 'NONE',  ( -5.494590086983840216, 1440.608783345210213, 202.1972241445429859 ) ) ;
#109346=CARTESIAN_POINT ( 'NONE',  ( -7.177114193734159819, 1426.187286780010027, 203.1778547286869809 ) ) ;
#109359=LINE ( 'NONE', #23675, #93310 ) ;
#109363=CARTESIAN_POINT ( 'NONE',  ( -15.13370552100000133, 1417.513322374810059, 204.2902361586989741 ) ) ;
#109365=DIRECTION ( 'NONE',  ( 0.9396491905462577288, 0.3023466567524009108, 0.1601433665701099407 ) ) ;
#109366=CARTESIAN_POINT ( 'NONE',  ( -8.645398683972508991, 1437.369593462749890, 208.8432647735320131 ) ) ;
#109368=CARTESIAN_POINT ( 'NONE',  ( 0.3811431543340009775, 1478.039055931090161, 201.4703185268089953 ) ) ;
#109381=CARTESIAN_POINT ( 'NONE',  ( 4.226426730299999157, 1515.477082009390188, 209.1218459616989946 ) ) ;
#109386=CARTESIAN_POINT ( 'NONE',  ( 10.17851409671319907, 1480.182533543850013, 206.4481411506540098 ) ) ;
#109387=ORIENTED_EDGE ( 'NONE', *, *, #14089, .T. ) ;
#109389=CARTESIAN_POINT ( 'NONE',  ( -19.86686180190000073, 1444.169376520590049, 213.3106045261990005 ) ) ;
#109391=CARTESIAN_POINT ( 'NONE',  ( 20.75865325816559803, 1455.056399775050068, 207.3304373731819794 ) ) ;
#109396=CARTESIAN_POINT ( 'NONE',  ( 3.829620113550000315, 1515.051704408389924, 209.0973262533439936 ) ) ;
#109397=CARTESIAN_POINT ( 'NONE',  ( -8.044397765300001168, 1452.253295118390042, 204.1782792353590139 ) ) ;
#109398=LINE ( 'NONE', #8564, #14437 ) ;
#109403=CARTESIAN_POINT ( 'NONE',  ( -17.55845490061370029, 1419.966211264809999, 204.6173968078139751 ) ) ;
#109415=CARTESIAN_POINT ( 'NONE',  ( 3.778540308873199915, 1515.551842517600107, 205.7532741663330000 ) ) ;
#109416=CARTESIAN_POINT ( 'NONE',  ( 3.601839739459999912, 1444.840594719589944, 200.9001243581789993 ) ) ;
#109419=CARTESIAN_POINT ( 'NONE',  ( -5.208614297041160413, 1464.433914205869996, 199.4042851730860093 ) ) ;
#109435=CARTESIAN_POINT ( 'NONE',  ( -12.20495830810000015, 1503.566102511789950, 208.5052324830940051 ) ) ;
#109438=VERTEX_POINT ( 'NONE', #13017 ) ;
#109440=VERTEX_POINT ( 'NONE', #48313 ) ;
#109442=CARTESIAN_POINT ( 'NONE',  ( -7.846715645779529069, 1452.866283417570003, 204.0807684293459943 ) ) ;
#109446=VERTEX_POINT ( 'NONE', #47203 ) ;
#109448=CARTESIAN_POINT ( 'NONE',  ( -5.311724842150000292, 1500.891271500089942, 229.7588813323989996 ) ) ;
#109450=CARTESIAN_POINT ( 'NONE',  ( 20.83491851400000172, 1494.467306230789973, 206.1460450736289829 ) ) ;
#109456=CARTESIAN_POINT ( 'NONE',  ( 12.07459970771560087, 1492.710845711899992, 211.7408674243640121 ) ) ;
#109474=CARTESIAN_POINT ( 'NONE',  ( -9.521726183726670456, 1448.210812606100035, 209.8762788027680131 ) ) ;
#109478=CIRCLE ( 'NONE', #93390, 12.38732017200242019 ) ;
#109483=CARTESIAN_POINT ( 'NONE',  ( 4.380514181050000566, 1467.321765115789958, 218.0672140897789859 ) ) ;
#109489=CARTESIAN_POINT ( 'NONE',  ( -1.441213829320000084, 1430.262570393590067, 200.5314639573489899 ) ) ;
#109493=ORIENTED_EDGE ( 'NONE', *, *, #63363, .T. ) ;
#109498=CARTESIAN_POINT ( 'NONE',  ( 11.12031993019763121, 1427.725797866641187, 210.2198567556694684 ) ) ;
#109502=CARTESIAN_POINT ( 'NONE',  ( -2.329898369990449858, 1515.064791341159889, 213.4512947646889813 ) ) ;
#109517=CARTESIAN_POINT ( 'NONE',  ( -4.989228071470000359, 1445.489057496590249, 216.9515723730989976 ) ) ;
#109520=CARTESIAN_POINT ( 'NONE',  ( 9.688259743311579797, 1463.788314065760233, 210.6196158358079913 ) ) ;
#109521=CARTESIAN_POINT ( 'NONE',  ( 7.089203542179999928, 1424.901038349889859, 213.0569889132190156 ) ) ;
#109531=EDGE_CURVE ( 'NONE', #46077, #53580, #74938, .T. ) ;
#109533=CARTESIAN_POINT ( 'NONE',  ( -13.61181236409999862, 1504.842419174190127, 227.7680708624989734 ) ) ;
#109540=CARTESIAN_POINT ( 'NONE',  ( -7.300564999359999696, 1480.050509870389988, 209.3673580074350014 ) ) ;
#109543=CARTESIAN_POINT ( 'NONE',  ( -10.37617513879240150, 1479.403831811299824, 210.6295454707710064 ) ) ;
#109548=CARTESIAN_POINT ( 'NONE',  ( -4.327741874859570181, 1515.129976808890206, 209.8453366680959959 ) ) ;
#109550=ORIENTED_EDGE ( 'NONE', *, *, #77112, .F. ) ;
#109553=CARTESIAN_POINT ( 'NONE',  ( 7.361390247576359513, 1424.789603017459967, 194.1635867254269954 ) ) ;
#109555=CARTESIAN_POINT ( 'NONE',  ( 0.9948947628070290428, 1432.734526706880160, 200.7323199818169996 ) ) ;
#109558=ORIENTED_EDGE ( 'NONE', *, *, #8261, .F. ) ;
#109567=DIRECTION ( 'NONE',  ( 0.1930015070322609605, 0.3681831545501960123, -0.9095007328137468816 ) ) ;
#109570=ADVANCED_FACE ( 'NONE', ( #62801 ), #52635, .T. ) ;
#109579=CARTESIAN_POINT ( 'NONE',  ( 8.231849866949039196, 1438.595873408519992, 212.0577543541930368 ) ) ;
#109584=CARTESIAN_POINT ( 'NONE',  ( -8.611763555213059362, 1437.722137921690091, 208.1397161665540239 ) ) ;
#109589=B_SPLINE_CURVE_WITH_KNOTS ( 'NONE', 3,
 ( #98953, #65938, #48583, #82717, #23349, #107363, #22776, #92214, #22226, #91113, #14389, #57540, #83265, #30659, #39039, #7113, #58081, #91663, #65389, #24440 ),
 .UNSPECIFIED., .F., .F.,
 ( 4, 2, 2, 2, 1, 1, 1, 1, 2, 2, 2, 4 ),
 ( 0.000000000000000000, 0.2500000000004283796, 0.3750000000006425971, 0.4375000000007521206, 0.4687500000008068546, 0.4843750000008363310, 0.4921875000008418821, 0.4960937500008518741, 0.4980468750008568146, 0.5000000000008617551, 0.7500000000004308776, 1.000000000000000000 ),
 .UNSPECIFIED. ) ;
#109594=CARTESIAN_POINT ( 'NONE',  ( 6.244159553780000316, 1487.029148873190024, 200.2607382902990025 ) ) ;
#109595=DIRECTION ( 'NONE',  ( 0.4794255386042031719, 0.000000000000000000, 0.8775825618903726477 ) ) ;
#109605=FACE_OUTER_BOUND ( 'NONE', #35304, .T. ) ;
#109608=CARTESIAN_POINT ( 'NONE',  ( -11.38457156623280220, 1470.946925340780126, 208.3536595213249996 ) ) ;
#109609=CARTESIAN_POINT ( 'NONE',  ( -6.245546245917391381, 1508.324562708814938, 220.0345331073419572 ) ) ;
#109614=CARTESIAN_POINT ( 'NONE',  ( -6.589996145302899677, 1420.351519938529918, 194.7646280328370096 ) ) ;
#109615=CARTESIAN_POINT ( 'NONE',  ( 4.328845283827350343, 1515.087839320550074, 207.8437208991539933 ) ) ;
#109622=CARTESIAN_POINT ( 'NONE',  ( 7.500754515229999697, 1423.062356241809766, 195.6521582632990146 ) ) ;
#109628=CARTESIAN_POINT ( 'NONE',  ( -4.324479010949999314, 1515.254596385190098, 208.3983727628749989 ) ) ;
#109632=CARTESIAN_POINT ( 'NONE',  ( 11.94675882516600041, 1492.833009754569957, 212.2903486444920134 ) ) ;
#109633=CARTESIAN_POINT ( 'NONE',  ( 1.326713953160000070, 1454.806608698389937, 218.4390644836289823 ) ) ;
#109638=CARTESIAN_POINT ( 'NONE',  ( -1.602167524609999782, 1430.706703968889997, 217.3531761583190018 ) ) ;
#109639=ORIENTED_EDGE ( 'NONE', *, *, #84388, .T. ) ;
#109641=CARTESIAN_POINT ( 'NONE',  ( -8.200736117659999991, 1501.216938893890074, 208.7100876187340077 ) ) ;
#109642=CARTESIAN_POINT ( 'NONE',  ( -2.329898367295349715, 1515.064791340959800, 204.7923971591859811 ) ) ;
#109644=CARTESIAN_POINT ( 'NONE',  ( -16.79355120555579717, 1420.470915846049820, 203.2250788671829866 ) ) ;
#109645=CARTESIAN_POINT ( 'NONE',  ( 11.75431539821480165, 1479.716031737669937, 209.9331422352859988 ) ) ;
#109647=CARTESIAN_POINT ( 'NONE',  ( 0.2017839417000019953, 1448.939945588189858, 190.0257811526990110 ) ) ;
#109649=CARTESIAN_POINT ( 'NONE',  ( -16.32163182381450284, 1508.551704408389924, 213.4489841974129831 ) ) ;
#109654=CARTESIAN_POINT ( 'NONE',  ( 8.177528389328550418, 1433.974668205089984, 204.5575942349009892 ) ) ;
#109663=FACE_OUTER_BOUND ( 'NONE', #47268, .T. ) ;
#109665=CARTESIAN_POINT ( 'NONE',  ( -0.6209246912237348370, 1515.589587247160352, 213.1417529444950105 ) ) ;
#109666=CARTESIAN_POINT ( 'NONE',  ( 2.008229287959999887, 1477.194275967190151, 198.7982270578989983 ) ) ;
#109672=CARTESIAN_POINT ( 'NONE',  ( -8.370248062009999046, 1424.386071264410020, 207.6999102099590004 ) ) ;
#109677=CARTESIAN_POINT ( 'NONE',  ( 7.467787984152029601, 1426.091549560359908, 212.4046628816660132 ) ) ;
#109685=CARTESIAN_POINT ( 'NONE',  ( -16.65350847794880451, 1508.454466938620271, 213.7226249311669903 ) ) ;
#109686=CARTESIAN_POINT ( 'NONE',  ( -4.633397096295920115, 1377.913060387289988, 213.8868415672910146 ) ) ;
#109694=EDGE_LOOP ( 'NONE', ( #13385, #33369, #45887, #98382 ) ) ;
#109695=EDGE_CURVE ( 'NONE', #3640, #5600, #69603, .T. ) ;
#109704=ORIENTED_EDGE ( 'NONE', *, *, #68530, .T. ) ;
#109709=ORIENTED_EDGE ( 'NONE', *, *, #13601, .F. ) ;
#109712=CARTESIAN_POINT ( 'NONE',  ( 0.6825862493659989871, 1429.440998290589960, 214.6621653640990246 ) ) ;
#109716=CARTESIAN_POINT ( 'NONE',  ( 0.000000000000000000, 1378.913060387289988, 209.1218459616989946 ) ) ;
#109717=CARTESIAN_POINT ( 'NONE',  ( 11.91507101810570113, 1501.870660809160199, 213.5943109225670185 ) ) ;
#109718=CARTESIAN_POINT ( 'NONE',  ( 8.157055013780000863, 1421.297622302039827, 196.0511713190989838 ) ) ;
#109719=CARTESIAN_POINT ( 'NONE',  ( -0.3337973666484369550, 1431.965207721749948, 218.6129415553859872 ) ) ;
#109720=CARTESIAN_POINT ( 'NONE',  ( -5.301603799309999587, 1495.069284652189936, 198.4487960541990219 ) ) ;
#109723=DIRECTION ( 'NONE',  ( -1.000000000000000000, 0.000000000000000000, -4.657385588302535823E-10 ) ) ;
#109724=CARTESIAN_POINT ( 'NONE',  ( 11.71723861691340041, 1426.603203500050085, 206.5361617024459804 ) ) ;
#109731=CARTESIAN_POINT ( 'NONE',  ( -11.33780467209640008, 1482.838548967459701, 205.4682982156419939 ) ) ;
#109733=FACE_OUTER_BOUND ( 'NONE', #58124, .T. ) ;
#109734=CARTESIAN_POINT ( 'NONE',  ( 11.31726009937499988, 1422.350445949510004, 203.3738828430369665 ) ) ;
#109740=CARTESIAN_POINT ( 'NONE',  ( -9.663432460078139385, 1460.495846937979877, 209.0938806983130007 ) ) ;
#109742=CARTESIAN_POINT ( 'NONE',  ( 7.733708448627369059, 1421.053201843950092, 195.5966628498169939 ) ) ;
#109744=CARTESIAN_POINT ( 'NONE',  ( 9.272480241026579861, 1463.528063730330132, 214.3122284173120136 ) ) ;
#109754=CARTESIAN_POINT ( 'NONE',  ( 9.549998149862538810, 1451.222071596379919, 207.5451647876320180 ) ) ;
#109758=CARTESIAN_POINT ( 'NONE',  ( -15.45163273801909831, 1421.121908474589873, 203.4374413400199728 ) ) ;
#109761=ORIENTED_EDGE ( 'NONE', *, *, #50292, .F. ) ;
#109770=B_SPLINE_SURFACE_WITH_KNOTS ( 'NONE', 5, 5, ( 
 ( #92699, #50177, #84305, #59674, #59131, #50708 ),
 ( #84839, #108409, #25482, #7050, #83754, #49621 ),
 ( #23285, #6498, #31691, #65874, #92157, #99994 ),
 ( #76458, #32254, #66977, #41208, #66434, #57481 ),
 ( #15430, #75378, #109517, #8139, #42305, #83209 ),
 ( #91606, #101088, #23830, #68090, #74821, #58570 ),
 ( #33337, #7596, #24387, #100550, #41751, #14883 ),
 ( #75910, #40098, #67532, #101632, #24921, #110612 ),
 ( #33894, #93253, #16518, #17061, #82662, #5953 ) ),
 .UNSPECIFIED., .F., .F., .F.,
 ( 6, 3, 6 ),
 ( 6, 6 ),
 ( 11.46419780020000090, 17.35795963829999877, 30.62292852850000102 ),
 ( 0.000000000000000000, 2.000000000000000000 ),
 .UNSPECIFIED. ) ;
#109771=CARTESIAN_POINT ( 'NONE',  ( -0.8557946027419990331, 1485.901655772089953, 197.2260526041989976 ) ) ;
#109772=CARTESIAN_POINT ( 'NONE',  ( -16.43158050010680071, 1420.644938884899830, 203.2808245233400157 ) ) ;
#109773=DIRECTION ( 'NONE',  ( 8.727810504445229884E-47, -1.000000000000000000, 1.836970198721029688E-16 ) ) ;
#109776=CARTESIAN_POINT ( 'NONE',  ( 6.520094218474939751, 1467.947603753620115, 206.8052153602889973 ) ) ;
#109784=CARTESIAN_POINT ( 'NONE',  ( 10.78065115729800105, 1422.571582845389912, 208.5037857000629913 ) ) ;
#109785=ORIENTED_EDGE ( 'NONE', *, *, #41772, .F. ) ;
#109790=CARTESIAN_POINT ( 'NONE',  ( 4.221033085759999359, 1472.290285735790121, 218.3905899716789918 ) ) ;
#109793=CARTESIAN_POINT ( 'NONE',  ( -5.215695275219999871, 1495.379823515289900, 198.7908128922989874 ) ) ;
#109798=CARTESIAN_POINT ( 'NONE',  ( 7329.274061526074547, -2340.220200558883789, 11096.25664408519697 ) ) ;
#109801=EDGE_CURVE ( 'NONE', #57731, #77826, #52998, .T. ) ;
#109802=DIRECTION ( 'NONE',  ( 0.9996573249755517088, -0.02617694830808747070, 0.000000000000000000 ) ) ;
#109803=CARTESIAN_POINT ( 'NONE',  ( -0.3879872414129990066, 1457.041586684089907, 199.5965184120390177 ) ) ;
#109827=CARTESIAN_POINT ( 'NONE',  ( 24.11200186056320049, 1496.633625139249943, 206.8275369771670000 ) ) ;
#109829=CARTESIAN_POINT ( 'NONE',  ( 3.313501335607582643, 1397.551704408390151, 215.1871694724064810 ) ) ;
#109835=CARTESIAN_POINT ( 'NONE',  ( -4.822785920201220655, 1507.731391114710050, 221.0789200719150074 ) ) ;
#109836=CARTESIAN_POINT ( 'NONE',  ( -14.15978805234909998, 1508.551704406640056, 210.0665490177079846 ) ) ;
#109838=CARTESIAN_POINT ( 'NONE',  ( 11.16717556649999921, 1414.661898229710005, 205.5169791222290030 ) ) ;
#109839=AXIS2_PLACEMENT_3D ( 'NONE', #24652, #48816, #109802 ) ;
#109841=CARTESIAN_POINT ( 'NONE',  ( -5.135284114272939959, 1454.993527858050129, 201.2217254690109769 ) ) ;
#109860=CARTESIAN_POINT ( 'NONE',  ( 10.69573263740039870, 1470.053339629819902, 207.0568841171169936 ) ) ;
#109866=CARTESIAN_POINT ( 'NONE',  ( 5.336874482553809251, 1467.014048226709974, 199.3769685164120062 ) ) ;
#109875=CARTESIAN_POINT ( 'NONE',  ( -11.59032152810750027, 1501.222894206809997, 211.2547116848260202 ) ) ;
#109878=CARTESIAN_POINT ( 'NONE',  ( -1.565724986139999997, 1508.487491088089882, 220.5488880004989767 ) ) ;
#109888=ORIENTED_EDGE ( 'NONE', *, *, #94937, .T. ) ;
#109896=( BOUNDED_CURVE ( )  B_SPLINE_CURVE ( 3, ( #34664, #540, #35217, #69403 ),
 .UNSPECIFIED., .F., .F. ) 
 B_SPLINE_CURVE_WITH_KNOTS ( ( 4, 4 ),
 ( 4.160324501940654507, 5.264453772624229977 ),
 .UNSPECIFIED. ) 
 CURVE ( )  GEOMETRIC_REPRESENTATION_ITEM ( )  RATIONAL_B_SPLINE_CURVE ( ( 1.000000000000000000, 0.9009623648433412457, 0.9009623648433412457, 1.000000000000000000 ) ) 
 REPRESENTATION_ITEM ( '' )  );
#109899=CARTESIAN_POINT ( 'NONE',  ( -14.46903053109999959, 1416.198242731890105, 203.7983957840089886 ) ) ;
#109901=CARTESIAN_POINT ( 'NONE',  ( -4.004834694394450167, 1485.215656302600109, 197.9145253210909914 ) ) ;
#109902=CARTESIAN_POINT ( 'NONE',  ( -16.22196899596580266, 1419.732669852162189, 209.9109564629500824 ) ) ;
#109903=CARTESIAN_POINT ( 'NONE',  ( -4.158099799109999495, 1497.082135898890101, 220.0114517002990056 ) ) ;
#109907=CARTESIAN_POINT ( 'NONE',  ( 10.57472631152969988, 1481.432876148939840, 209.0048588833070085 ) ) ;
#109925=CARTESIAN_POINT ( 'NONE',  ( 12.45034049356619832, 1421.619540909540092, 207.5029415923690124 ) ) ;
#109926=CARTESIAN_POINT ( 'NONE',  ( 10.46048277684489847, 1479.162378809809979, 206.0229427181779727 ) ) ;
#109928=B_SPLINE_SURFACE_WITH_KNOTS ( 'NONE', 5, 5, ( 
 ( #41308, #81634, #49171, #107951, #107398, #74925 ),
 ( #31243, #48624, #14427, #21716, #31793, #6598 ),
 ( #65427, #91151, #82755, #108506, #58120, #6047 ),
 ( #40198, #75481, #83852, #13316, #23387, #47511 ),
 ( #100106, #30694, #109075, #30134, #65984, #57577 ),
 ( #91703, #39080, #14976, #99534, #64325, #4936 ),
 ( #22261, #66535, #100640, #92254, #56462, #15524 ),
 ( #90595, #7152, #13872, #24481, #58667, #8233 ),
 ( #43524, #60894, #93348, #33430, #92803, #8787 ) ),
 .UNSPECIFIED., .F., .F., .F.,
 ( 6, 3, 6 ),
 ( 6, 6 ),
 ( 2.998553390235009886, 5.159116185979999436, 7.319678981714989874 ),
 ( -0.0004280697249928139899, 2.000000000000000000 ),
 .UNSPECIFIED. ) ;
#109930=CARTESIAN_POINT ( 'NONE',  ( -17.47028495609999865, 1442.689969983390029, 219.3627138812989870 ) ) ;
#109932=CARTESIAN_POINT ( 'NONE',  ( -16.53114280955439952, 1465.611523215409989, 220.7423225738290000 ) ) ;
#109933=CARTESIAN_POINT ( 'NONE',  ( -16.14867264346439768, 1416.534170367229990, 209.2886075942629986 ) ) ;
#109938=CARTESIAN_POINT ( 'NONE',  ( 7.543547206879660294, 1448.836622091779873, 202.0922639109040233 ) ) ;
#109949=EDGE_LOOP ( 'NONE', ( #26201, #818, #90987, #55394 ) ) ;
#109956=CARTESIAN_POINT ( 'NONE',  ( -4.987078442593329441, 1508.551704408389924, 211.6097810465890063 ) ) ;
#109957=CARTESIAN_POINT ( 'NONE',  ( 2.156155154889999981, 1445.629270856190033, 199.6471593918289784 ) ) ;
#109962=CARTESIAN_POINT ( 'NONE',  ( -2.795964621609999590, 1422.864594294989956, 191.4386244948990168 ) ) ;
#109971=ORIENTED_EDGE ( 'NONE', *, *, #69870, .F. ) ;
#109975=CARTESIAN_POINT ( 'NONE',  ( 21.08794113720000141, 1497.248615914389802, 211.1864905400789780 ) ) ;
#109979=CARTESIAN_POINT ( 'NONE',  ( -12.33321046680000066, 1502.561053867989813, 208.9929973234150111 ) ) ;
#109980=DIRECTION ( 'NONE',  ( -0.4544580288560248760, -1.636314548565651616E-16, -0.8907681516580486791 ) ) ;
#109996=DIRECTION ( 'NONE',  ( -0.9996573249755574819, 0.02617694830786557875, 0.000000000000000000 ) ) ;
#110002=CARTESIAN_POINT ( 'NONE',  ( 9.785296660211628250, 1435.228160504780135, 208.4213188007680060 ) ) ;
#110008=B_SPLINE_SURFACE_WITH_KNOTS ( 'NONE', 5, 1, ( 
 ( #28073, #10737 ),
 ( #20214, #71217 ),
 ( #36475, #80688 ),
 ( #28630, #30267 ),
 ( #105341, #106979 ),
 ( #53301, #62261 ) ),
 .UNSPECIFIED., .F., .F., .F.,
 ( 6, 6 ),
 ( 2, 2 ),
 ( 0.000000000000000000, 3.599196727790000327 ),
 ( 0.000000000000000000, 14.00000000000000000 ),
 .UNSPECIFIED. ) ;
#110017=CARTESIAN_POINT ( 'NONE',  ( -9.942029349575120634, 1448.220099355010007, 209.0865656338810084 ) ) ;
#110025=CARTESIAN_POINT ( 'NONE',  ( 4.216418746870000511, 1466.253355729990062, 218.9008380672689782 ) ) ;
#110043=CARTESIAN_POINT ( 'NONE',  ( 11.46977278200000150, 1502.214325488189843, 209.8002689844269923 ) ) ;
#110046=CARTESIAN_POINT ( 'NONE',  ( -9.872142711616779920, 1438.638380141409925, 210.3201327332649839 ) ) ;
#110047=CARTESIAN_POINT ( 'NONE',  ( -3.829164871871630016, 1515.551704201149960, 211.4518032920690018 ) ) ;
#110055=CARTESIAN_POINT ( 'NONE',  ( 2.907016575484743903, 1493.671177366619531, 219.9120732454466918 ) ) ;
#110058=CARTESIAN_POINT ( 'NONE',  ( 2.876961725570000183, 1499.580235354990009, 230.2170217437989947 ) ) ;
#110060=CARTESIAN_POINT ( 'NONE',  ( 3.899433454979999603, 1454.070828365190209, 217.6618255207390007 ) ) ;
#110066=CARTESIAN_POINT ( 'NONE',  ( 7.012556801809999740, 1423.949223476430006, 213.3686902051989875 ) ) ;
#110068=CARTESIAN_POINT ( 'NONE',  ( -3.932260160163730145, 1453.946481855800130, 199.4130354687199826 ) ) ;
#110071=CARTESIAN_POINT ( 'NONE',  ( -7.082378735300329353, 1478.706589098139830, 211.5813507964070084 ) ) ;
#110085=CARTESIAN_POINT ( 'NONE',  ( 0.000000000000000000, 0.000000000000000000, 0.000000000000000000 ) ) ;
#110093=VERTEX_POINT ( 'NONE', #69065 ) ;
#110101=DIRECTION ( 'NONE',  ( 1.000000000000000000, 0.000000000000000000, 0.000000000000000000 ) ) ;
#110116=CARTESIAN_POINT ( 'NONE',  ( -10.51083736151210068, 1480.296936587089931, 210.9545377047529939 ) ) ;
#110122=CARTESIAN_POINT ( 'NONE',  ( 8.927134929145720932, 1436.767706396419953, 210.5802712642290260 ) ) ;
#110127=CARTESIAN_POINT ( 'NONE',  ( -10.16145782839999967, 1473.012443313389895, 208.1237237223820387 ) ) ;
#110130=CARTESIAN_POINT ( 'NONE',  ( 20.05410099200000218, 1476.341259462790049, 212.1028602122389941 ) ) ;
#110133=CARTESIAN_POINT ( 'NONE',  ( -15.00213922130000022, 1416.331168602359867, 208.3054305177020069 ) ) ;
#110135=CARTESIAN_POINT ( 'NONE',  ( 4.127868055549999582, 1487.366509936789953, 197.8725145131990075 ) ) ;
#110136=DIRECTION ( 'NONE',  ( -1.156023075842281927E-31, 1.000000000000000000, -1.698192320643030073E-16 ) ) ;
#110144=CARTESIAN_POINT ( 'NONE',  ( -17.05626209599999754, 1420.313787275360028, 203.5730941281789796 ) ) ;
#110146=VECTOR ( 'NONE', #61955, 1000.000000000000114 ) ;
#110153=CARTESIAN_POINT ( 'NONE',  ( -5.137024739602960466, 1508.240697825915277, 220.3835027126725379 ) ) ;
#110156=CARTESIAN_POINT ( 'NONE',  ( 12.03449227190490056, 1491.353386486839781, 206.6667661091970274 ) ) ;
#110160=CARTESIAN_POINT ( 'NONE',  ( -13.37434658702809998, 1416.899496760530155, 201.3810223920989984 ) ) ;
#110165=FACE_OUTER_BOUND ( 'NONE', #25545, .T. ) ;
#110168=CARTESIAN_POINT ( 'NONE',  ( -740.1067050508938792, 11216.44053380570222, -1627.040744446347389 ) ) ;
#110172=CARTESIAN_POINT ( 'NONE',  ( -17.51543252019589758, 1417.552277257849937, 206.7803077767080140 ) ) ;
#110176=CARTESIAN_POINT ( 'NONE',  ( 11.57342425378350015, 1492.618401364529973, 211.9083419029999789 ) ) ;
#110181=CARTESIAN_POINT ( 'NONE',  ( 4.948068031341160022, 1508.551704408389924, 206.1941938154730281 ) ) ;
#110187=CARTESIAN_POINT ( 'NONE',  ( 4.967684365510000255, 1469.890599266690060, 189.7939106698990201 ) ) ;
#110188=CARTESIAN_POINT ( 'NONE',  ( 11.70397832847810093, 1479.895218179510039, 210.5107915740969986 ) ) ;
#110192=CARTESIAN_POINT ( 'NONE',  ( -14.83447489583599932, 1508.551704408389924, 215.0596454497180048 ) ) ;
#110195=CARTESIAN_POINT ( 'NONE',  ( 2.669590603778499993, 1486.875611465459997, 197.4822887014510115 ) ) ;
#110198=ORIENTED_EDGE ( 'NONE', *, *, #13773, .T. ) ;
#110200=CARTESIAN_POINT ( 'NONE',  ( 20.65265016900000106, 1477.900423433889955, 217.6009028526389955 ) ) ;
#110207=CARTESIAN_POINT ( 'NONE',  ( -2.149974513279420130, 1421.471342383219962, 193.6364440172239938 ) ) ;
#110210=CARTESIAN_POINT ( 'NONE',  ( -3.076049692719999840, 1475.159716291190080, 198.5224444241989943 ) ) ;
#110212=CARTESIAN_POINT ( 'NONE',  ( 10.01013843233299916, 1469.369181467840008, 209.9819040969830155 ) ) ;
#110216=CARTESIAN_POINT ( 'NONE',  ( -8.749325254410001307, 1423.947972453919874, 207.8877631365490117 ) ) ;
#110220=CARTESIAN_POINT ( 'NONE',  ( 7.538936308525870267, 1425.689389508179829, 212.1914861486659731 ) ) ;
#110224=CARTESIAN_POINT ( 'NONE',  ( -10.97486499478319999, 1492.422550449080063, 207.2127083187249923 ) ) ;
#110228=CARTESIAN_POINT ( 'NONE',  ( 17.24398683809999966, 1428.425037375490092, 203.1706303392290067 ) ) ;
#110231=ORIENTED_EDGE ( 'NONE', *, *, #64063, .T. ) ;
#110236=EDGE_LOOP ( 'NONE', ( #6212, #89736, #50115, #97562 ) ) ;
#110255=CARTESIAN_POINT ( 'NONE',  ( -11.38448554521469980, 1481.434469010069961, 209.9556807158220124 ) ) ;
#110257=CARTESIAN_POINT ( 'NONE',  ( -3.930410876235079787, 1508.551704408389924, 213.6518643025299866 ) ) ;
#110259=CARTESIAN_POINT ( 'NONE',  ( 7.447014729250000187, 1422.296623052599898, 195.6434364388990161 ) ) ;
#110260=CARTESIAN_POINT ( 'NONE',  ( -1.315863322207099895, 1432.366940000970089, 218.5411383834640162 ) ) ;
#110261=CARTESIAN_POINT ( 'NONE',  ( -4.858768762960000487, 1495.519531265289970, 198.6104072793989985 ) ) ;
#110264=CARTESIAN_POINT ( 'NONE',  ( 3.945738874322921141, 1515.565581977719148, 210.3719421152130167 ) ) ;
#110266=B_SPLINE_CURVE_WITH_KNOTS ( 'NONE', 3,
 ( #10777, #85813, #105387, #51676, #44949, #69604, #2405, #36522, #71267, #103722 ),
 .UNSPECIFIED., .F., .F.,
 ( 4, 2, 2, 2, 4 ),
 ( 0.000000000000000000, 0.2500000000000000000, 0.5000000000000000000, 0.7500000000000000000, 1.000000000000000000 ),
 .UNSPECIFIED. ) ;
#110271=DIRECTION ( 'NONE',  ( -0.9122148146285387060, -0.3835045346744238581, 0.1441818430190649758 ) ) ;
#110272=CARTESIAN_POINT ( 'NONE',  ( -12.00997496865170788, 1508.551704408370824, 210.3182342545297843 ) ) ;
#110273=EDGE_CURVE ( 'NONE', #102658, #19773, #109398, .T. ) ;
#110276=CARTESIAN_POINT ( 'NONE',  ( 8.933680575207208818, 1427.300831583419949, 211.2763433717070143 ) ) ;
#110278=CARTESIAN_POINT ( 'NONE',  ( 11.59968585941729913, 1421.929632843320178, 203.4071348278239952 ) ) ;
#110287=EDGE_CURVE ( 'NONE', #105125, #37624, #77507, .T. ) ;
#110289=CARTESIAN_POINT ( 'NONE',  ( 10.61677160567779943, 1423.423170255460036, 201.7579950878699719 ) ) ;
#110290=CARTESIAN_POINT ( 'NONE',  ( 9.472111571387470619, 1463.349806330050114, 213.0242536977909822 ) ) ;
#110291=EDGE_CURVE ( 'NONE', #39608, #106390, #64237, .T. ) ;
#110297=CARTESIAN_POINT ( 'NONE',  ( -1.682334239950061150, 1477.245458038868037, 198.8259265945336267 ) ) ;
#110299=CARTESIAN_POINT ( 'NONE',  ( 3.194122154841241290, 1508.524191963859948, 219.6292475936541564 ) ) ;
#110300=CARTESIAN_POINT ( 'NONE',  ( -5.138230509358902687, 1391.881841899301889, 203.8075142969990168 ) ) ;
#110301=CARTESIAN_POINT ( 'NONE',  ( -20.36853079741129946, 1464.956632542119905, 210.9458194320050097 ) ) ;
#110304=CARTESIAN_POINT ( 'NONE',  ( -16.74123569586150140, 1419.926558681200049, 209.1244132309280133 ) ) ;
#110316=CARTESIAN_POINT ( 'NONE',  ( 9.158757463789999775, 1480.005755715189935, 203.7772472770490140 ) ) ;
#110319=EDGE_CURVE ( 'NONE', #74404, #64216, #44490, .T. ) ;
#110320=CARTESIAN_POINT ( 'NONE',  ( -4.973371544095850361, 1432.678537253299965, 216.0289570334049927 ) ) ;
#110322=CARTESIAN_POINT ( 'NONE',  ( -16.86653121810000044, 1418.408574706249965, 208.1493301914530036 ) ) ;
#110328=CARTESIAN_POINT ( 'NONE',  ( 10.86989896834730018, 1426.593996385999844, 207.8838144468849976 ) ) ;
#110335=CARTESIAN_POINT ( 'NONE',  ( 1.988015751190000069, 1473.864677161789814, 219.3075819037990186 ) ) ;
#110336=CARTESIAN_POINT ( 'NONE',  ( 18.20258715539999983, 1429.723789929190161, 209.1218459616989946 ) ) ;
#110338=CARTESIAN_POINT ( 'NONE',  ( -8.944365594689999810, 1494.493485459390058, 202.2793638724489824 ) ) ;
#110350=FACE_OUTER_BOUND ( 'NONE', #19635, .T. ) ;
#110353=ADVANCED_FACE ( 'NONE', ( #100826 ), #70559, .T. ) ;
#110365=CARTESIAN_POINT ( 'NONE',  ( 12.69817581368640091, 1500.644936277410125, 209.5553692708770086 ) ) ;
#110367=CARTESIAN_POINT ( 'NONE',  ( 3.345283522277380239, 1508.551704408389924, 213.9586846534960216 ) ) ;
#110380=CARTESIAN_POINT ( 'NONE',  ( -11.47747972145789142, 1417.728687405828850, 198.8488469395149991 ) ) ;
#110381=CARTESIAN_POINT ( 'NONE',  ( 4.138543391159999807, 1515.492058413689847, 210.9648081929590262 ) ) ;
#110383=CARTESIAN_POINT ( 'NONE',  ( -6.466661620000779820, 1454.065070619989910, 202.3287932644439877 ) ) ;
#110392=ORIENTED_EDGE ( 'NONE', *, *, #82360, .T. ) ;
#110399=CARTESIAN_POINT ( 'NONE',  ( -6.065469208827907188, 1433.485399230374014, 215.0992432421768683 ) ) ;
#110400=CARTESIAN_POINT ( 'NONE',  ( -10.55208896769630122, 1462.421637114440045, 208.2011304212279867 ) ) ;
#110404=CARTESIAN_POINT ( 'NONE',  ( -8.603211701180001114, 1469.317673379189955, 216.5015782100589945 ) ) ;
#110405=CARTESIAN_POINT ( 'NONE',  ( -10.47439550540000042, 1490.889281562089991, 212.4388770995890070 ) ) ;
#110413=ORIENTED_EDGE ( 'NONE', *, *, #1488, .F. ) ;
#110420=CARTESIAN_POINT ( 'NONE',  ( -11.33943867567700003, 1500.720461424150017, 211.0488575539550027 ) ) ;
#110423=CARTESIAN_POINT ( 'NONE',  ( -2.188073835520000010, 1508.020975839189987, 220.9453034226989985 ) ) ;
#110427=CARTESIAN_POINT ( 'NONE',  ( -10.98402802510699949, 1462.124134087619950, 210.0291763056419825 ) ) ;
#110429=CARTESIAN_POINT ( 'NONE',  ( 3.750000000000000000, 1512.051704408390151, 209.1218459616989946 ) ) ;
#110433=CARTESIAN_POINT ( 'NONE',  ( -10.51083735039999922, 1480.296936571690139, 210.9545376977389992 ) ) ;
#110439=CARTESIAN_POINT ( 'NONE',  ( 1.701332460469982433, 1456.209741179828598, 218.8708370859535819 ) ) ;
#110447=CARTESIAN_POINT ( 'NONE',  ( -15.39508542709999794, 1416.424718227980065, 206.7259350337689909 ) ) ;
#110449=CARTESIAN_POINT ( 'NONE',  ( -5.418330280727370329, 1484.891209372279945, 198.5201634387589991 ) ) ;
#110450=CARTESIAN_POINT ( 'NONE',  ( -5.264763130462112528, 1496.215617598504195, 199.2138358744504103 ) ) ;
#110453=CARTESIAN_POINT ( 'NONE',  ( -5.502752162680000225, 1437.219209177789935, 209.1105472058980013 ) ) ;
#110464=CARTESIAN_POINT ( 'NONE',  ( -4.329448781177520189, 1515.064792686469900, 210.9648092169189795 ) ) ;
#110472=CARTESIAN_POINT ( 'NONE',  ( 4.800520365470000606, 1485.026014063289949, 218.8652762536089824 ) ) ;
#110473=CARTESIAN_POINT ( 'NONE',  ( 10.78014379640850073, 1479.477604915960001, 207.2887695641769881 ) ) ;
#110475=CARTESIAN_POINT ( 'NONE',  ( -8.149274592039999376, 1439.839152417889864, 228.6706535942990115 ) ) ;
#110481=CARTESIAN_POINT ( 'NONE',  ( 3.552713678799999608E-15, 1413.913060387330006, 209.1218459616989946 ) ) ;
#110490=CARTESIAN_POINT ( 'NONE',  ( 15.04135733889389925, 1432.105820058640120, 219.6911068266909979 ) ) ;
#110501=CARTESIAN_POINT ( 'NONE',  ( 4.020406191785269812, 1515.375307391110027, 205.5795572779110216 ) ) ;
#110516=VERTEX_POINT ( 'NONE', #91072 ) ;
#110520=CARTESIAN_POINT ( 'NONE',  ( -6.163969623551973420, 1475.687477306443270, 200.8053095011335927 ) ) ;
#110523=CARTESIAN_POINT ( 'NONE',  ( 11.30087886326580104, 1422.109560457819953, 210.2596498238989966 ) ) ;
#110526=ORIENTED_EDGE ( 'NONE', *, *, #72771, .F. ) ;
#110533=CARTESIAN_POINT ( 'NONE',  ( -1.940673996872300133, 1422.484488249149990, 192.6009970386809869 ) ) ;
#110534=ORIENTED_EDGE ( 'NONE', *, *, #43589, .F. ) ;
#110544=CARTESIAN_POINT ( 'NONE',  ( -3.325048289822069680, 1428.738726997929916, 200.3675363921470307 ) ) ;
#110549=CARTESIAN_POINT ( 'NONE',  ( 9.778038872353379318, 1435.196923564789813, 208.3424860689369780 ) ) ;
#110557=EDGE_CURVE ( 'NONE', #65578, #93757, #25303, .T. ) ;
#110559=CARTESIAN_POINT ( 'NONE',  ( 1.702416261868870073, 1493.957958506549858, 220.1113518634800243 ) ) ;
#110564=CARTESIAN_POINT ( 'NONE',  ( -9.208813132158530479, 1450.227655483129865, 208.7826788825430242 ) ) ;
#110574=CARTESIAN_POINT ( 'NONE',  ( -13.50530508558610165, 1506.272574391458193, 209.1324396371510659 ) ) ;
#110575=CARTESIAN_POINT ( 'NONE',  ( 3.887546720220000029, 1467.073181280790095, 218.4203203200989947 ) ) ;
#110580=CARTESIAN_POINT ( 'NONE',  ( -2.451814001629999851, 1429.700538548090208, 200.7967559036290197 ) ) ;
#110584=EDGE_LOOP ( 'NONE', ( #57508, #15730, #30251, #38624, #84751 ) ) ;
#110590=CARTESIAN_POINT ( 'NONE',  ( 11.47835457579999918, 1502.362092611190064, 208.5873688113690037 ) ) ;
#110591=CARTESIAN_POINT ( 'NONE',  ( -10.99273638689999899, 1491.630725208689910, 209.8916735729859795 ) ) ;
#110593=EDGE_CURVE ( 'NONE', #15508, #24424, #27905, .T. ) ;
#110595=CARTESIAN_POINT ( 'NONE',  ( 9.190770083770001264, 1428.225163806190039, 212.7760827912590003 ) ) ;
#110596=CARTESIAN_POINT ( 'NONE',  ( 1.702403487548299843, 1493.957943060129992, 220.1113531599900170 ) ) ;
#110597=FACE_OUTER_BOUND ( 'NONE', #72915, .T. ) ;
#110609=CARTESIAN_POINT ( 'NONE',  ( -15.30083054224856554, 1416.035659937719629, 206.6105554433750626 ) ) ;
#110612=CARTESIAN_POINT ( 'NONE',  ( -9.318458176530000969, 1446.292171852890078, 213.7041144372790313 ) ) ;
#110616=FACE_OUTER_BOUND ( 'NONE', #85421, .T. ) ;
#110623=LINE ( 'NONE', #50190, #21047 ) ;
#110624=ORIENTED_EDGE ( 'NONE', *, *, #26171, .T. ) ;
#110635=CARTESIAN_POINT ( 'NONE',  ( -9.352115965572330936, 1447.735190698479983, 210.9908785053780207 ) ) ;
#110644=CARTESIAN_POINT ( 'NONE',  ( 7.814348457125529279, 1424.914214976869971, 194.3898514750090101 ) ) ;
#110661=CARTESIAN_POINT ( 'NONE',  ( -9.526128307108560733, 1440.436522615020067, 205.9995050262249947 ) ) ;
#110677=CARTESIAN_POINT ( 'NONE',  ( -11.57883448593699782, 1491.718296208979837, 205.0404881661760044 ) ) ;
#110681=CARTESIAN_POINT ( 'NONE',  ( -15.03953889140000122, 1416.231637368560087, 208.6543985418939826 ) ) ;
#110683=CARTESIAN_POINT ( 'NONE',  ( 8.680261597580001265, 1487.719285257089950, 202.4559307200990190 ) ) ;
#110687=CARTESIAN_POINT ( 'NONE',  ( -18.31482527320000031, 1445.278739201789904, 204.5307550449689984 ) ) ;
#110696=EDGE_CURVE ( 'NONE', #75973, #59183, #30609, .T. ) ;
#110706=CARTESIAN_POINT ( 'NONE',  ( 10.41177509810879975, 1460.024667384750046, 205.9063203302740135 ) ) ;
#110710=CARTESIAN_POINT ( 'NONE',  ( -12.85636183069170002, 1417.155669274680122, 200.5510948150419779 ) ) ;
#110716=LINE ( 'NONE', #51361, #91384 ) ;
#110719=CARTESIAN_POINT ( 'NONE',  ( -10.49767250057509926, 1480.215366257469896, 208.4046347607720122 ) ) ;
#110723=CARTESIAN_POINT ( 'NONE',  ( -4.138993644619999301, 1515.551749209489799, 209.1218459617069811 ) ) ;
#110727=CARTESIAN_POINT ( 'NONE',  ( 11.45382141796380004, 1491.761286053230151, 209.6395483024749922 ) ) ;
#110734=EDGE_LOOP ( 'NONE', ( #30023, #14534, #89024, #30473, #74836, #48441, #32441, #32034, #1630, #31798 ) ) ;
#110741=CARTESIAN_POINT ( 'NONE',  ( 11.62073329257960097, 1480.091610248069856, 211.1128523392590068 ) ) ;
#110751=VECTOR ( 'NONE', #69683, 999.9999999999998863 ) ;
#110755=CARTESIAN_POINT ( 'NONE',  ( 20.38160163584860030, 1475.532940563729881, 217.9568059512479863 ) ) ;
#110765=CARTESIAN_POINT ( 'NONE',  ( -0.6851706257419990509, 1475.635431348089924, 197.6580713075989877 ) ) ;
#110775=CARTESIAN_POINT ( 'NONE',  ( -6.647957898892952855, 1470.949127383563791, 216.7466839929853677 ) ) ;
#110776=CARTESIAN_POINT ( 'NONE',  ( 7.490783964907898884, 1426.014963415389957, 212.3433401526569924 ) ) ;
#110779=ORIENTED_EDGE ( 'NONE', *, *, #68000, .T. ) ;
#110784=CARTESIAN_POINT ( 'NONE',  ( 7.894362808210001248, 1424.028044848189893, 212.1595859666189767 ) ) ;
#110785=CARTESIAN_POINT ( 'NONE',  ( 4.103915387205919529, 1467.926924930979794, 218.2234441087299786 ) ) ;
#110790=CARTESIAN_POINT ( 'NONE',  ( 8.379013882420577985, 1435.477853948120128, 206.7290831433529661 ) ) ;
#110791=ORIENTED_EDGE ( 'NONE', *, *, #53610, .T. ) ;
#110800=CARTESIAN_POINT ( 'NONE',  ( 4.679791025795809745, 1508.610720109290014, 212.2979026938089930 ) ) ;
#110803=CARTESIAN_POINT ( 'NONE',  ( -4.827292224569999846, 1429.041575181189955, 202.2878225452089964 ) ) ;
#110807=CARTESIAN_POINT ( 'NONE',  ( 1.636696423147410151, 1445.551428100869998, 199.1693562641009976 ) ) ;
#110810=CARTESIAN_POINT ( 'NONE',  ( -11.71878239930389931, 1481.302890658779916, 210.8565630715119994 ) ) ;
#110813=CARTESIAN_POINT ( 'NONE',  ( -3.856607047483139983, 1508.551704408389924, 213.7021005842219949 ) ) ;
#110815=CARTESIAN_POINT ( 'NONE',  ( 7.682163124739999738, 1421.658071144350060, 195.7645034974990210 ) ) ;
#110816=CARTESIAN_POINT ( 'NONE',  ( -3.220674668504990290, 1433.265634988960073, 218.1214075394389909 ) ) ;
#110817=B_SPLINE_SURFACE_WITH_KNOTS ( 'NONE', 5, 1, ( 
 ( #58674, #67635 ),
 ( #92809, #25035 ),
 ( #50286, #36642 ),
 ( #54576, #19825 ),
 ( #79212, #70838 ),
 ( #37746, #88711 ) ),
 .UNSPECIFIED., .F., .F., .F.,
 ( 6, 6 ),
 ( 2, 2 ),
 ( 0.000000000000000000, 3.542454554009999868 ),
 ( 0.000000000000000000, 14.00000000000000000 ),
 .UNSPECIFIED. ) ;
#110818=CARTESIAN_POINT ( 'NONE',  ( -3.617578910780000268, 1497.333807970789849, 198.4503654230989866 ) ) ;
#110825=ORIENTED_EDGE ( 'NONE', *, *, #17348, .F. ) ;
#110827=CARTESIAN_POINT ( 'NONE',  ( 4.930158634465010792, 1484.410507904570068, 219.1064042044509392 ) ) ;
#110828=CARTESIAN_POINT ( 'NONE',  ( -10.30348281067860050, 1483.409064405780100, 203.1509397556989995 ) ) ;
#110831=CARTESIAN_POINT ( 'NONE',  ( -10.15848451741849878, 1462.015496030800023, 208.6817910193179841 ) ) ;
ENDSEC;
END-ISO-10303-21;
